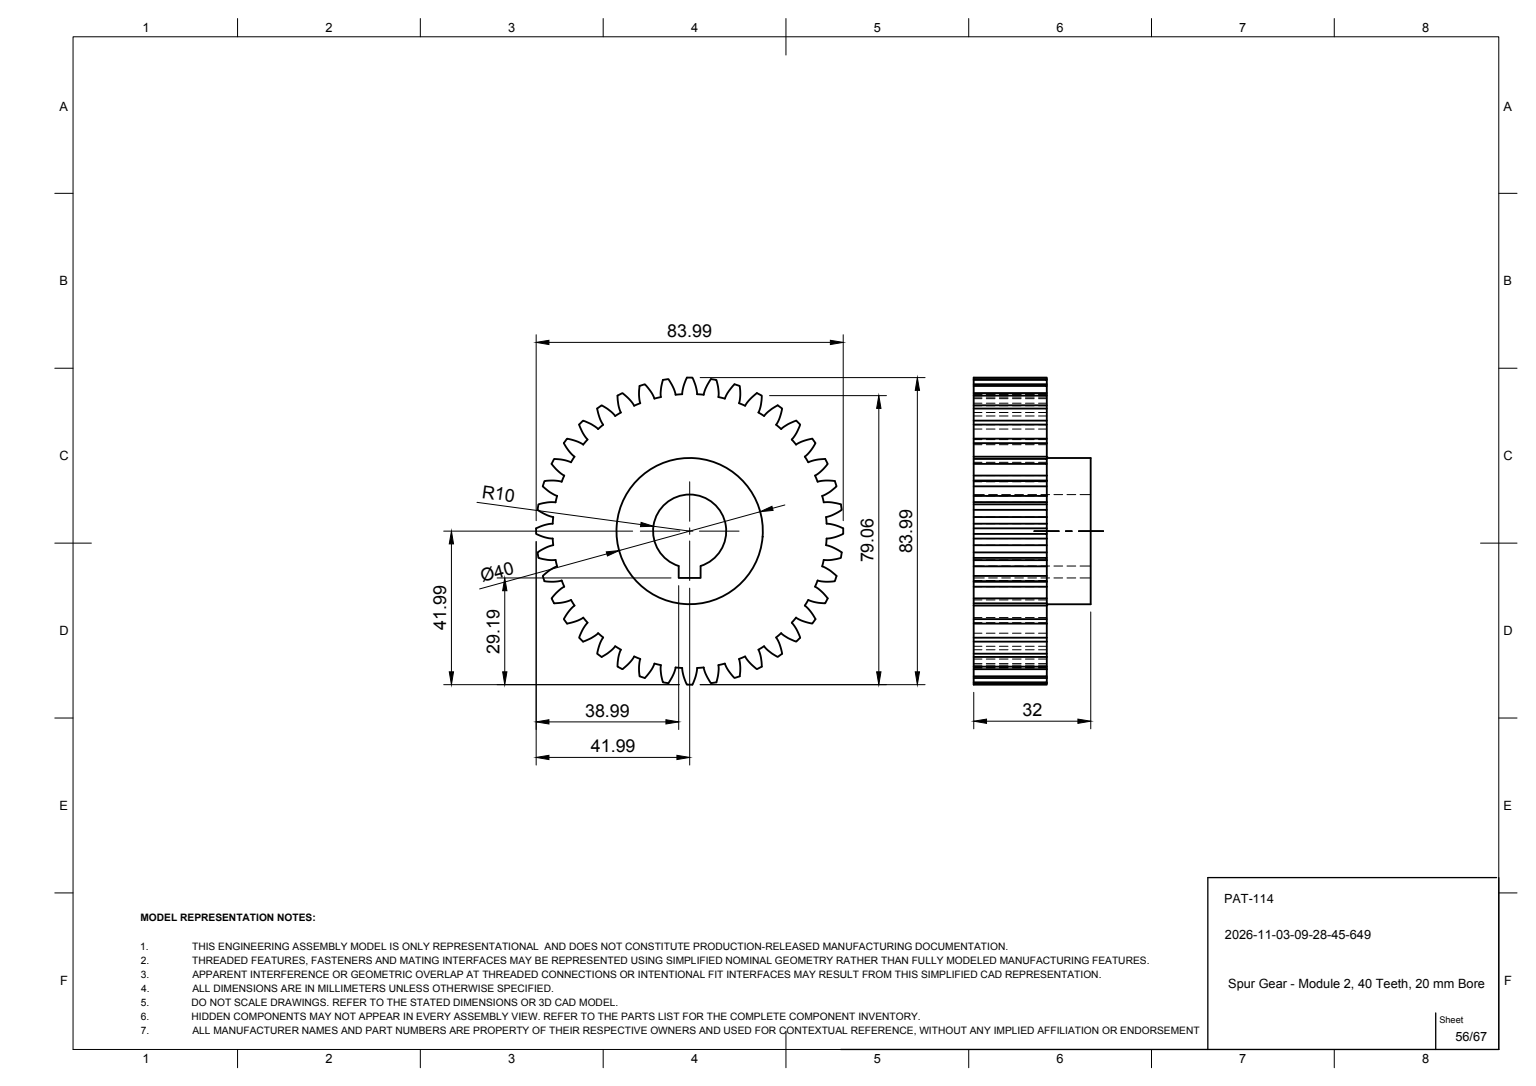
ISO-10303-21;
HEADER;
/* Generated by software containing ST-Developer
 * from STEP Tools, Inc. (www.steptools.com) 
 */

FILE_DESCRIPTION(
/* description */ ('Two-stage gear reducer in split housing'),
/* implementation_level */ '2;1');

FILE_NAME(
/* name */ 'Spur Gear - Module 2, 40 Teeth, 20 mm Bore.step',
/* time_stamp */ '2026-10-28T03:22:31-07:00',
/* author */ (''),
/* organization */ (''),
/* preprocessor_version */ 'ST-DEVELOPER v20.2',
/* originating_system */ 'Autodesk Translation Framework v15.17.0.0',
/* authorisation */ '');

FILE_SCHEMA (('AUTOMOTIVE_DESIGN { 1 0 10303 214 3 1 1 }'));
ENDSEC;

DATA;
#10=MECHANICAL_DESIGN_GEOMETRIC_PRESENTATION_REPRESENTATION('',(#1303),#73366);
#91=(
BOUNDED_SURFACE()
B_SPLINE_SURFACE(5,1,((#55478,#55479),(#55480,#55481),(#55482,#55483),(#55484,
#55485),(#55486,#55487),(#55488,#55489),(#55490,#55491),(#55492,#55493),
(#55494,#55495),(#55496,#55497),(#55498,#55499),(#55500,#55501),(#55502,
#55503),(#55504,#55505),(#55506,#55507),(#55508,#55509),(#55510,#55511),
(#55512,#55513),(#55514,#55515),(#55516,#55517),(#55518,#55519),(#55520,
#55521),(#55522,#55523),(#55524,#55525),(#55526,#55527),(#55528,#55529),
(#55530,#55531),(#55532,#55533),(#55534,#55535),(#55536,#55537),(#55538,
#55539),(#55540,#55541),(#55542,#55543),(#55544,#55545),(#55546,#55547),
(#55548,#55549),(#55550,#55551),(#55552,#55553),(#55554,#55555),(#55556,
#55557),(#55558,#55559),(#55560,#55561),(#55562,#55563),(#55564,#55565),
(#55566,#55567),(#55568,#55569),(#55570,#55571),(#55572,#55573),(#55574,
#55575),(#55576,#55577),(#55578,#55579),(#55580,#55581),(#55582,#55583),
(#55584,#55585),(#55586,#55587),(#55588,#55589),(#55590,#55591),(#55592,
#55593),(#55594,#55595),(#55596,#55597),(#55598,#55599),(#55600,#55601),
(#55602,#55603),(#55604,#55605),(#55606,#55607),(#55608,#55609),(#55610,
#55611),(#55612,#55613),(#55614,#55615),(#55616,#55617)),.UNSPECIFIED.,
 .F.,.F.,.F.)
B_SPLINE_SURFACE_WITH_KNOTS((6,1,1,1,1,1,1,1,1,1,1,1,1,1,1,1,1,1,1,1,1,
1,1,1,1,1,1,1,1,1,1,1,1,1,1,1,1,1,1,1,1,1,1,1,1,1,1,1,1,1,1,1,1,1,1,1,1,
1,1,1,1,1,1,1,1,6),(2,2),(-1.,-0.984615384615383,-0.969230769230768,-0.953846153846152,
-0.938461538461537,-0.923076923076922,-0.907692307692306,-0.892307692307691,
-0.876923076923076,-0.86153846153846,-0.846153846153845,-0.83076923076923,
-0.815384615384614,-0.799999999999999,-0.784615384615384,-0.769230769230768,
-0.753846153846153,-0.738461538461538,-0.723076923076922,-0.707692307692307,
-0.692307692307692,-0.676923076923076,-0.661538461538461,-0.646153846153846,
-0.63076923076923,-0.615384615384615,-0.6,-0.584615384615384,-0.569230769230769,
-0.553846153846154,-0.538461538461538,-0.523076923076923,-0.507692307692308,
-0.492307692307692,-0.476923076923077,-0.461538461538462,-0.446153846153846,
-0.430769230769231,-0.415384615384615,-0.4,-0.384615384615385,-0.369230769230769,
-0.353846153846154,-0.338461538461538,-0.323076923076923,-0.307692307692308,
-0.292307692307692,-0.276923076923077,-0.261538461538462,-0.246153846153846,
-0.230769230769231,-0.215384615384615,-0.2,-0.184615384615385,-0.169230769230769,
-0.153846153846154,-0.138461538461538,-0.123076923076923,-0.107692307692308,
-0.0923076923076923,-0.0769230769230769,-0.0615384615384615,-0.0461538461538462,
-0.0307692307692308,-0.0153846153846154,0.),(-1.,1.),.UNSPECIFIED.)
GEOMETRIC_REPRESENTATION_ITEM()
RATIONAL_B_SPLINE_SURFACE(((1.,1.),(1.,1.),(1.,1.),(1.,1.),(1.,1.),(1.,
1.),(1.,1.),(1.,1.),(1.,1.),(1.,1.),(1.,1.),(1.,1.),(1.,1.),(1.,1.),(1.,
1.),(1.,1.),(1.,1.),(1.,1.),(1.,1.),(1.,1.),(1.,1.),(1.,1.),(1.,1.),(1.,
1.),(1.,1.),(1.,1.),(1.,1.),(1.,1.),(1.,1.),(1.,1.),(1.,1.),(1.,1.),(1.,
1.),(1.,1.),(1.,1.),(1.,1.),(1.,1.),(1.,1.),(1.,1.),(1.,1.),(1.,1.),(1.,
1.),(1.,1.),(1.,1.),(1.,1.),(1.,1.),(1.,1.),(1.,1.),(1.,1.),(1.,1.),(1.,
1.),(1.,1.),(1.,1.),(1.,1.),(1.,1.),(1.,1.),(1.,1.),(1.,1.),(1.,1.),(1.,
1.),(1.,1.),(1.,1.),(1.,1.),(1.,1.),(1.,1.),(1.,1.),(1.,1.),(1.,1.),(1.,
1.),(1.,1.)))
REPRESENTATION_ITEM('')
SURFACE()
);
#92=(
BOUNDED_SURFACE()
B_SPLINE_SURFACE(5,1,((#55697,#55698),(#55699,#55700),(#55701,#55702),(#55703,
#55704),(#55705,#55706),(#55707,#55708),(#55709,#55710),(#55711,#55712),
(#55713,#55714),(#55715,#55716),(#55717,#55718),(#55719,#55720),(#55721,
#55722),(#55723,#55724),(#55725,#55726),(#55727,#55728),(#55729,#55730),
(#55731,#55732),(#55733,#55734),(#55735,#55736),(#55737,#55738),(#55739,
#55740),(#55741,#55742),(#55743,#55744),(#55745,#55746),(#55747,#55748),
(#55749,#55750),(#55751,#55752),(#55753,#55754),(#55755,#55756),(#55757,
#55758),(#55759,#55760),(#55761,#55762),(#55763,#55764),(#55765,#55766),
(#55767,#55768),(#55769,#55770),(#55771,#55772),(#55773,#55774),(#55775,
#55776),(#55777,#55778),(#55779,#55780),(#55781,#55782),(#55783,#55784),
(#55785,#55786),(#55787,#55788),(#55789,#55790),(#55791,#55792),(#55793,
#55794),(#55795,#55796),(#55797,#55798),(#55799,#55800),(#55801,#55802),
(#55803,#55804),(#55805,#55806),(#55807,#55808),(#55809,#55810),(#55811,
#55812),(#55813,#55814),(#55815,#55816),(#55817,#55818),(#55819,#55820),
(#55821,#55822),(#55823,#55824),(#55825,#55826),(#55827,#55828),(#55829,
#55830),(#55831,#55832),(#55833,#55834),(#55835,#55836)),.UNSPECIFIED.,
 .F.,.F.,.F.)
B_SPLINE_SURFACE_WITH_KNOTS((6,1,1,1,1,1,1,1,1,1,1,1,1,1,1,1,1,1,1,1,1,
1,1,1,1,1,1,1,1,1,1,1,1,1,1,1,1,1,1,1,1,1,1,1,1,1,1,1,1,1,1,1,1,1,1,1,1,
1,1,1,1,1,1,1,1,6),(2,2),(-1.,-0.984615384615383,-0.969230769230768,-0.953846153846152,
-0.938461538461537,-0.923076923076922,-0.907692307692306,-0.892307692307691,
-0.876923076923076,-0.86153846153846,-0.846153846153845,-0.83076923076923,
-0.815384615384614,-0.799999999999999,-0.784615384615384,-0.769230769230768,
-0.753846153846153,-0.738461538461538,-0.723076923076922,-0.707692307692307,
-0.692307692307692,-0.676923076923076,-0.661538461538461,-0.646153846153846,
-0.63076923076923,-0.615384615384615,-0.6,-0.584615384615384,-0.569230769230769,
-0.553846153846154,-0.538461538461538,-0.523076923076923,-0.507692307692308,
-0.492307692307692,-0.476923076923077,-0.461538461538462,-0.446153846153846,
-0.430769230769231,-0.415384615384615,-0.4,-0.384615384615385,-0.369230769230769,
-0.353846153846154,-0.338461538461538,-0.323076923076923,-0.307692307692308,
-0.292307692307692,-0.276923076923077,-0.261538461538462,-0.246153846153846,
-0.230769230769231,-0.215384615384615,-0.2,-0.184615384615385,-0.169230769230769,
-0.153846153846154,-0.138461538461538,-0.123076923076923,-0.107692307692308,
-0.0923076923076923,-0.0769230769230769,-0.0615384615384615,-0.0461538461538462,
-0.0307692307692308,-0.0153846153846154,0.),(-1.,1.),.UNSPECIFIED.)
GEOMETRIC_REPRESENTATION_ITEM()
RATIONAL_B_SPLINE_SURFACE(((1.,1.),(1.,1.),(1.,1.),(1.,1.),(1.,1.),(1.,
1.),(1.,1.),(1.,1.),(1.,1.),(1.,1.),(1.,1.),(1.,1.),(1.,1.),(1.,1.),(1.,
1.),(1.,1.),(1.,1.),(1.,1.),(1.,1.),(1.,1.),(1.,1.),(1.,1.),(1.,1.),(1.,
1.),(1.,1.),(1.,1.),(1.,1.),(1.,1.),(1.,1.),(1.,1.),(1.,1.),(1.,1.),(1.,
1.),(1.,1.),(1.,1.),(1.,1.),(1.,1.),(1.,1.),(1.,1.),(1.,1.),(1.,1.),(1.,
1.),(1.,1.),(1.,1.),(1.,1.),(1.,1.),(1.,1.),(1.,1.),(1.,1.),(1.,1.),(1.,
1.),(1.,1.),(1.,1.),(1.,1.),(1.,1.),(1.,1.),(1.,1.),(1.,1.),(1.,1.),(1.,
1.),(1.,1.),(1.,1.),(1.,1.),(1.,1.),(1.,1.),(1.,1.),(1.,1.),(1.,1.),(1.,
1.),(1.,1.)))
REPRESENTATION_ITEM('')
SURFACE()
);
#93=(
BOUNDED_SURFACE()
B_SPLINE_SURFACE(5,1,((#55927,#55928),(#55929,#55930),(#55931,#55932),(#55933,
#55934),(#55935,#55936),(#55937,#55938),(#55939,#55940),(#55941,#55942),
(#55943,#55944),(#55945,#55946),(#55947,#55948),(#55949,#55950),(#55951,
#55952),(#55953,#55954),(#55955,#55956),(#55957,#55958),(#55959,#55960),
(#55961,#55962),(#55963,#55964),(#55965,#55966),(#55967,#55968),(#55969,
#55970),(#55971,#55972),(#55973,#55974),(#55975,#55976),(#55977,#55978),
(#55979,#55980),(#55981,#55982),(#55983,#55984),(#55985,#55986),(#55987,
#55988),(#55989,#55990),(#55991,#55992),(#55993,#55994),(#55995,#55996),
(#55997,#55998),(#55999,#56000),(#56001,#56002),(#56003,#56004),(#56005,
#56006),(#56007,#56008),(#56009,#56010),(#56011,#56012),(#56013,#56014),
(#56015,#56016),(#56017,#56018),(#56019,#56020),(#56021,#56022),(#56023,
#56024),(#56025,#56026),(#56027,#56028),(#56029,#56030),(#56031,#56032),
(#56033,#56034),(#56035,#56036),(#56037,#56038),(#56039,#56040),(#56041,
#56042),(#56043,#56044),(#56045,#56046),(#56047,#56048),(#56049,#56050),
(#56051,#56052),(#56053,#56054),(#56055,#56056),(#56057,#56058),(#56059,
#56060),(#56061,#56062),(#56063,#56064),(#56065,#56066)),.UNSPECIFIED.,
 .F.,.F.,.F.)
B_SPLINE_SURFACE_WITH_KNOTS((6,1,1,1,1,1,1,1,1,1,1,1,1,1,1,1,1,1,1,1,1,
1,1,1,1,1,1,1,1,1,1,1,1,1,1,1,1,1,1,1,1,1,1,1,1,1,1,1,1,1,1,1,1,1,1,1,1,
1,1,1,1,1,1,1,1,6),(2,2),(-1.,-0.984615384615383,-0.969230769230768,-0.953846153846152,
-0.938461538461537,-0.923076923076922,-0.907692307692306,-0.892307692307691,
-0.876923076923076,-0.86153846153846,-0.846153846153845,-0.83076923076923,
-0.815384615384614,-0.799999999999999,-0.784615384615384,-0.769230769230768,
-0.753846153846153,-0.738461538461538,-0.723076923076922,-0.707692307692307,
-0.692307692307692,-0.676923076923076,-0.661538461538461,-0.646153846153846,
-0.63076923076923,-0.615384615384615,-0.6,-0.584615384615384,-0.569230769230769,
-0.553846153846154,-0.538461538461538,-0.523076923076923,-0.507692307692308,
-0.492307692307692,-0.476923076923077,-0.461538461538462,-0.446153846153846,
-0.430769230769231,-0.415384615384615,-0.4,-0.384615384615385,-0.369230769230769,
-0.353846153846154,-0.338461538461538,-0.323076923076923,-0.307692307692308,
-0.292307692307692,-0.276923076923077,-0.261538461538462,-0.246153846153846,
-0.230769230769231,-0.215384615384615,-0.2,-0.184615384615385,-0.169230769230769,
-0.153846153846154,-0.138461538461538,-0.123076923076923,-0.107692307692308,
-0.0923076923076923,-0.0769230769230769,-0.0615384615384615,-0.0461538461538462,
-0.0307692307692308,-0.0153846153846154,0.),(-1.,1.),.UNSPECIFIED.)
GEOMETRIC_REPRESENTATION_ITEM()
RATIONAL_B_SPLINE_SURFACE(((1.,1.),(1.,1.),(1.,1.),(1.,1.),(1.,1.),(1.,
1.),(1.,1.),(1.,1.),(1.,1.),(1.,1.),(1.,1.),(1.,1.),(1.,1.),(1.,1.),(1.,
1.),(1.,1.),(1.,1.),(1.,1.),(1.,1.),(1.,1.),(1.,1.),(1.,1.),(1.,1.),(1.,
1.),(1.,1.),(1.,1.),(1.,1.),(1.,1.),(1.,1.),(1.,1.),(1.,1.),(1.,1.),(1.,
1.),(1.,1.),(1.,1.),(1.,1.),(1.,1.),(1.,1.),(1.,1.),(1.,1.),(1.,1.),(1.,
1.),(1.,1.),(1.,1.),(1.,1.),(1.,1.),(1.,1.),(1.,1.),(1.,1.),(1.,1.),(1.,
1.),(1.,1.),(1.,1.),(1.,1.),(1.,1.),(1.,1.),(1.,1.),(1.,1.),(1.,1.),(1.,
1.),(1.,1.),(1.,1.),(1.,1.),(1.,1.),(1.,1.),(1.,1.),(1.,1.),(1.,1.),(1.,
1.),(1.,1.)))
REPRESENTATION_ITEM('')
SURFACE()
);
#94=(
BOUNDED_SURFACE()
B_SPLINE_SURFACE(5,1,((#56139,#56140),(#56141,#56142),(#56143,#56144),(#56145,
#56146),(#56147,#56148),(#56149,#56150),(#56151,#56152),(#56153,#56154),
(#56155,#56156),(#56157,#56158),(#56159,#56160),(#56161,#56162),(#56163,
#56164),(#56165,#56166),(#56167,#56168),(#56169,#56170),(#56171,#56172),
(#56173,#56174),(#56175,#56176),(#56177,#56178),(#56179,#56180),(#56181,
#56182),(#56183,#56184),(#56185,#56186),(#56187,#56188),(#56189,#56190),
(#56191,#56192),(#56193,#56194),(#56195,#56196),(#56197,#56198),(#56199,
#56200),(#56201,#56202),(#56203,#56204),(#56205,#56206),(#56207,#56208),
(#56209,#56210),(#56211,#56212),(#56213,#56214),(#56215,#56216),(#56217,
#56218),(#56219,#56220),(#56221,#56222),(#56223,#56224),(#56225,#56226),
(#56227,#56228),(#56229,#56230),(#56231,#56232),(#56233,#56234),(#56235,
#56236),(#56237,#56238),(#56239,#56240),(#56241,#56242),(#56243,#56244),
(#56245,#56246),(#56247,#56248),(#56249,#56250),(#56251,#56252),(#56253,
#56254),(#56255,#56256),(#56257,#56258),(#56259,#56260),(#56261,#56262),
(#56263,#56264),(#56265,#56266),(#56267,#56268),(#56269,#56270),(#56271,
#56272),(#56273,#56274),(#56275,#56276),(#56277,#56278)),.UNSPECIFIED.,
 .F.,.F.,.F.)
B_SPLINE_SURFACE_WITH_KNOTS((6,1,1,1,1,1,1,1,1,1,1,1,1,1,1,1,1,1,1,1,1,
1,1,1,1,1,1,1,1,1,1,1,1,1,1,1,1,1,1,1,1,1,1,1,1,1,1,1,1,1,1,1,1,1,1,1,1,
1,1,1,1,1,1,1,1,6),(2,2),(-1.,-0.984615384615383,-0.969230769230768,-0.953846153846152,
-0.938461538461537,-0.923076923076922,-0.907692307692306,-0.892307692307691,
-0.876923076923076,-0.86153846153846,-0.846153846153845,-0.83076923076923,
-0.815384615384614,-0.799999999999999,-0.784615384615384,-0.769230769230768,
-0.753846153846153,-0.738461538461538,-0.723076923076922,-0.707692307692307,
-0.692307692307692,-0.676923076923076,-0.661538461538461,-0.646153846153846,
-0.63076923076923,-0.615384615384615,-0.6,-0.584615384615384,-0.569230769230769,
-0.553846153846154,-0.538461538461538,-0.523076923076923,-0.507692307692308,
-0.492307692307692,-0.476923076923077,-0.461538461538462,-0.446153846153846,
-0.430769230769231,-0.415384615384615,-0.4,-0.384615384615385,-0.369230769230769,
-0.353846153846154,-0.338461538461538,-0.323076923076923,-0.307692307692308,
-0.292307692307692,-0.276923076923077,-0.261538461538462,-0.246153846153846,
-0.230769230769231,-0.215384615384615,-0.2,-0.184615384615385,-0.169230769230769,
-0.153846153846154,-0.138461538461538,-0.123076923076923,-0.107692307692308,
-0.0923076923076923,-0.0769230769230769,-0.0615384615384615,-0.0461538461538462,
-0.0307692307692308,-0.0153846153846154,0.),(-1.,1.),.UNSPECIFIED.)
GEOMETRIC_REPRESENTATION_ITEM()
RATIONAL_B_SPLINE_SURFACE(((1.,1.),(1.,1.),(1.,1.),(1.,1.),(1.,1.),(1.,
1.),(1.,1.),(1.,1.),(1.,1.),(1.,1.),(1.,1.),(1.,1.),(1.,1.),(1.,1.),(1.,
1.),(1.,1.),(1.,1.),(1.,1.),(1.,1.),(1.,1.),(1.,1.),(1.,1.),(1.,1.),(1.,
1.),(1.,1.),(1.,1.),(1.,1.),(1.,1.),(1.,1.),(1.,1.),(1.,1.),(1.,1.),(1.,
1.),(1.,1.),(1.,1.),(1.,1.),(1.,1.),(1.,1.),(1.,1.),(1.,1.),(1.,1.),(1.,
1.),(1.,1.),(1.,1.),(1.,1.),(1.,1.),(1.,1.),(1.,1.),(1.,1.),(1.,1.),(1.,
1.),(1.,1.),(1.,1.),(1.,1.),(1.,1.),(1.,1.),(1.,1.),(1.,1.),(1.,1.),(1.,
1.),(1.,1.),(1.,1.),(1.,1.),(1.,1.),(1.,1.),(1.,1.),(1.,1.),(1.,1.),(1.,
1.),(1.,1.)))
REPRESENTATION_ITEM('')
SURFACE()
);
#95=(
BOUNDED_SURFACE()
B_SPLINE_SURFACE(5,1,((#56369,#56370),(#56371,#56372),(#56373,#56374),(#56375,
#56376),(#56377,#56378),(#56379,#56380),(#56381,#56382),(#56383,#56384),
(#56385,#56386),(#56387,#56388),(#56389,#56390),(#56391,#56392),(#56393,
#56394),(#56395,#56396),(#56397,#56398),(#56399,#56400),(#56401,#56402),
(#56403,#56404),(#56405,#56406),(#56407,#56408),(#56409,#56410),(#56411,
#56412),(#56413,#56414),(#56415,#56416),(#56417,#56418),(#56419,#56420),
(#56421,#56422),(#56423,#56424),(#56425,#56426),(#56427,#56428),(#56429,
#56430),(#56431,#56432),(#56433,#56434),(#56435,#56436),(#56437,#56438),
(#56439,#56440),(#56441,#56442),(#56443,#56444),(#56445,#56446),(#56447,
#56448),(#56449,#56450),(#56451,#56452),(#56453,#56454),(#56455,#56456),
(#56457,#56458),(#56459,#56460),(#56461,#56462),(#56463,#56464),(#56465,
#56466),(#56467,#56468),(#56469,#56470),(#56471,#56472),(#56473,#56474),
(#56475,#56476),(#56477,#56478),(#56479,#56480),(#56481,#56482),(#56483,
#56484),(#56485,#56486),(#56487,#56488),(#56489,#56490),(#56491,#56492),
(#56493,#56494),(#56495,#56496),(#56497,#56498),(#56499,#56500),(#56501,
#56502),(#56503,#56504),(#56505,#56506),(#56507,#56508)),.UNSPECIFIED.,
 .F.,.F.,.F.)
B_SPLINE_SURFACE_WITH_KNOTS((6,1,1,1,1,1,1,1,1,1,1,1,1,1,1,1,1,1,1,1,1,
1,1,1,1,1,1,1,1,1,1,1,1,1,1,1,1,1,1,1,1,1,1,1,1,1,1,1,1,1,1,1,1,1,1,1,1,
1,1,1,1,1,1,1,1,6),(2,2),(-1.,-0.984615384615383,-0.969230769230768,-0.953846153846152,
-0.938461538461537,-0.923076923076922,-0.907692307692306,-0.892307692307691,
-0.876923076923076,-0.86153846153846,-0.846153846153845,-0.83076923076923,
-0.815384615384614,-0.799999999999999,-0.784615384615384,-0.769230769230768,
-0.753846153846153,-0.738461538461538,-0.723076923076922,-0.707692307692307,
-0.692307692307692,-0.676923076923076,-0.661538461538461,-0.646153846153846,
-0.63076923076923,-0.615384615384615,-0.6,-0.584615384615384,-0.569230769230769,
-0.553846153846154,-0.538461538461538,-0.523076923076923,-0.507692307692308,
-0.492307692307692,-0.476923076923077,-0.461538461538462,-0.446153846153846,
-0.430769230769231,-0.415384615384615,-0.4,-0.384615384615385,-0.369230769230769,
-0.353846153846154,-0.338461538461538,-0.323076923076923,-0.307692307692308,
-0.292307692307692,-0.276923076923077,-0.261538461538462,-0.246153846153846,
-0.230769230769231,-0.215384615384615,-0.2,-0.184615384615385,-0.169230769230769,
-0.153846153846154,-0.138461538461538,-0.123076923076923,-0.107692307692308,
-0.0923076923076923,-0.0769230769230769,-0.0615384615384615,-0.0461538461538462,
-0.0307692307692308,-0.0153846153846154,0.),(-1.,1.),.UNSPECIFIED.)
GEOMETRIC_REPRESENTATION_ITEM()
RATIONAL_B_SPLINE_SURFACE(((1.,1.),(1.,1.),(1.,1.),(1.,1.),(1.,1.),(1.,
1.),(1.,1.),(1.,1.),(1.,1.),(1.,1.),(1.,1.),(1.,1.),(1.,1.),(1.,1.),(1.,
1.),(1.,1.),(1.,1.),(1.,1.),(1.,1.),(1.,1.),(1.,1.),(1.,1.),(1.,1.),(1.,
1.),(1.,1.),(1.,1.),(1.,1.),(1.,1.),(1.,1.),(1.,1.),(1.,1.),(1.,1.),(1.,
1.),(1.,1.),(1.,1.),(1.,1.),(1.,1.),(1.,1.),(1.,1.),(1.,1.),(1.,1.),(1.,
1.),(1.,1.),(1.,1.),(1.,1.),(1.,1.),(1.,1.),(1.,1.),(1.,1.),(1.,1.),(1.,
1.),(1.,1.),(1.,1.),(1.,1.),(1.,1.),(1.,1.),(1.,1.),(1.,1.),(1.,1.),(1.,
1.),(1.,1.),(1.,1.),(1.,1.),(1.,1.),(1.,1.),(1.,1.),(1.,1.),(1.,1.),(1.,
1.),(1.,1.)))
REPRESENTATION_ITEM('')
SURFACE()
);
#96=(
BOUNDED_SURFACE()
B_SPLINE_SURFACE(5,1,((#56581,#56582),(#56583,#56584),(#56585,#56586),(#56587,
#56588),(#56589,#56590),(#56591,#56592),(#56593,#56594),(#56595,#56596),
(#56597,#56598),(#56599,#56600),(#56601,#56602),(#56603,#56604),(#56605,
#56606),(#56607,#56608),(#56609,#56610),(#56611,#56612),(#56613,#56614),
(#56615,#56616),(#56617,#56618),(#56619,#56620),(#56621,#56622),(#56623,
#56624),(#56625,#56626),(#56627,#56628),(#56629,#56630),(#56631,#56632),
(#56633,#56634),(#56635,#56636),(#56637,#56638),(#56639,#56640),(#56641,
#56642),(#56643,#56644),(#56645,#56646),(#56647,#56648),(#56649,#56650),
(#56651,#56652),(#56653,#56654),(#56655,#56656),(#56657,#56658),(#56659,
#56660),(#56661,#56662),(#56663,#56664),(#56665,#56666),(#56667,#56668),
(#56669,#56670),(#56671,#56672),(#56673,#56674),(#56675,#56676),(#56677,
#56678),(#56679,#56680),(#56681,#56682),(#56683,#56684),(#56685,#56686),
(#56687,#56688),(#56689,#56690),(#56691,#56692),(#56693,#56694),(#56695,
#56696),(#56697,#56698),(#56699,#56700),(#56701,#56702),(#56703,#56704),
(#56705,#56706),(#56707,#56708),(#56709,#56710),(#56711,#56712),(#56713,
#56714),(#56715,#56716),(#56717,#56718),(#56719,#56720)),.UNSPECIFIED.,
 .F.,.F.,.F.)
B_SPLINE_SURFACE_WITH_KNOTS((6,1,1,1,1,1,1,1,1,1,1,1,1,1,1,1,1,1,1,1,1,
1,1,1,1,1,1,1,1,1,1,1,1,1,1,1,1,1,1,1,1,1,1,1,1,1,1,1,1,1,1,1,1,1,1,1,1,
1,1,1,1,1,1,1,1,6),(2,2),(-1.,-0.984615384615383,-0.969230769230768,-0.953846153846152,
-0.938461538461537,-0.923076923076922,-0.907692307692306,-0.892307692307691,
-0.876923076923076,-0.86153846153846,-0.846153846153845,-0.83076923076923,
-0.815384615384614,-0.799999999999999,-0.784615384615384,-0.769230769230768,
-0.753846153846153,-0.738461538461538,-0.723076923076922,-0.707692307692307,
-0.692307692307692,-0.676923076923076,-0.661538461538461,-0.646153846153846,
-0.63076923076923,-0.615384615384615,-0.6,-0.584615384615384,-0.569230769230769,
-0.553846153846154,-0.538461538461538,-0.523076923076923,-0.507692307692308,
-0.492307692307692,-0.476923076923077,-0.461538461538462,-0.446153846153846,
-0.430769230769231,-0.415384615384615,-0.4,-0.384615384615385,-0.369230769230769,
-0.353846153846154,-0.338461538461538,-0.323076923076923,-0.307692307692308,
-0.292307692307692,-0.276923076923077,-0.261538461538462,-0.246153846153846,
-0.230769230769231,-0.215384615384615,-0.2,-0.184615384615385,-0.169230769230769,
-0.153846153846154,-0.138461538461538,-0.123076923076923,-0.107692307692308,
-0.0923076923076923,-0.0769230769230769,-0.0615384615384615,-0.0461538461538462,
-0.0307692307692308,-0.0153846153846154,0.),(-1.,1.),.UNSPECIFIED.)
GEOMETRIC_REPRESENTATION_ITEM()
RATIONAL_B_SPLINE_SURFACE(((1.,1.),(1.,1.),(1.,1.),(1.,1.),(1.,1.),(1.,
1.),(1.,1.),(1.,1.),(1.,1.),(1.,1.),(1.,1.),(1.,1.),(1.,1.),(1.,1.),(1.,
1.),(1.,1.),(1.,1.),(1.,1.),(1.,1.),(1.,1.),(1.,1.),(1.,1.),(1.,1.),(1.,
1.),(1.,1.),(1.,1.),(1.,1.),(1.,1.),(1.,1.),(1.,1.),(1.,1.),(1.,1.),(1.,
1.),(1.,1.),(1.,1.),(1.,1.),(1.,1.),(1.,1.),(1.,1.),(1.,1.),(1.,1.),(1.,
1.),(1.,1.),(1.,1.),(1.,1.),(1.,1.),(1.,1.),(1.,1.),(1.,1.),(1.,1.),(1.,
1.),(1.,1.),(1.,1.),(1.,1.),(1.,1.),(1.,1.),(1.,1.),(1.,1.),(1.,1.),(1.,
1.),(1.,1.),(1.,1.),(1.,1.),(1.,1.),(1.,1.),(1.,1.),(1.,1.),(1.,1.),(1.,
1.),(1.,1.)))
REPRESENTATION_ITEM('')
SURFACE()
);
#97=(
BOUNDED_SURFACE()
B_SPLINE_SURFACE(5,1,((#56811,#56812),(#56813,#56814),(#56815,#56816),(#56817,
#56818),(#56819,#56820),(#56821,#56822),(#56823,#56824),(#56825,#56826),
(#56827,#56828),(#56829,#56830),(#56831,#56832),(#56833,#56834),(#56835,
#56836),(#56837,#56838),(#56839,#56840),(#56841,#56842),(#56843,#56844),
(#56845,#56846),(#56847,#56848),(#56849,#56850),(#56851,#56852),(#56853,
#56854),(#56855,#56856),(#56857,#56858),(#56859,#56860),(#56861,#56862),
(#56863,#56864),(#56865,#56866),(#56867,#56868),(#56869,#56870),(#56871,
#56872),(#56873,#56874),(#56875,#56876),(#56877,#56878),(#56879,#56880),
(#56881,#56882),(#56883,#56884),(#56885,#56886),(#56887,#56888),(#56889,
#56890),(#56891,#56892),(#56893,#56894),(#56895,#56896),(#56897,#56898),
(#56899,#56900),(#56901,#56902),(#56903,#56904),(#56905,#56906),(#56907,
#56908),(#56909,#56910),(#56911,#56912),(#56913,#56914),(#56915,#56916),
(#56917,#56918),(#56919,#56920),(#56921,#56922),(#56923,#56924),(#56925,
#56926),(#56927,#56928),(#56929,#56930),(#56931,#56932),(#56933,#56934),
(#56935,#56936),(#56937,#56938),(#56939,#56940),(#56941,#56942),(#56943,
#56944),(#56945,#56946),(#56947,#56948),(#56949,#56950)),.UNSPECIFIED.,
 .F.,.F.,.F.)
B_SPLINE_SURFACE_WITH_KNOTS((6,1,1,1,1,1,1,1,1,1,1,1,1,1,1,1,1,1,1,1,1,
1,1,1,1,1,1,1,1,1,1,1,1,1,1,1,1,1,1,1,1,1,1,1,1,1,1,1,1,1,1,1,1,1,1,1,1,
1,1,1,1,1,1,1,1,6),(2,2),(-1.,-0.984615384615383,-0.969230769230768,-0.953846153846152,
-0.938461538461537,-0.923076923076922,-0.907692307692306,-0.892307692307691,
-0.876923076923076,-0.86153846153846,-0.846153846153845,-0.83076923076923,
-0.815384615384614,-0.799999999999999,-0.784615384615384,-0.769230769230768,
-0.753846153846153,-0.738461538461538,-0.723076923076922,-0.707692307692307,
-0.692307692307692,-0.676923076923076,-0.661538461538461,-0.646153846153846,
-0.63076923076923,-0.615384615384615,-0.6,-0.584615384615384,-0.569230769230769,
-0.553846153846154,-0.538461538461538,-0.523076923076923,-0.507692307692308,
-0.492307692307692,-0.476923076923077,-0.461538461538462,-0.446153846153846,
-0.430769230769231,-0.415384615384615,-0.4,-0.384615384615385,-0.369230769230769,
-0.353846153846154,-0.338461538461538,-0.323076923076923,-0.307692307692308,
-0.292307692307692,-0.276923076923077,-0.261538461538462,-0.246153846153846,
-0.230769230769231,-0.215384615384615,-0.2,-0.184615384615385,-0.169230769230769,
-0.153846153846154,-0.138461538461538,-0.123076923076923,-0.107692307692308,
-0.0923076923076923,-0.0769230769230769,-0.0615384615384615,-0.0461538461538462,
-0.0307692307692308,-0.0153846153846154,0.),(-1.,1.),.UNSPECIFIED.)
GEOMETRIC_REPRESENTATION_ITEM()
RATIONAL_B_SPLINE_SURFACE(((1.,1.),(1.,1.),(1.,1.),(1.,1.),(1.,1.),(1.,
1.),(1.,1.),(1.,1.),(1.,1.),(1.,1.),(1.,1.),(1.,1.),(1.,1.),(1.,1.),(1.,
1.),(1.,1.),(1.,1.),(1.,1.),(1.,1.),(1.,1.),(1.,1.),(1.,1.),(1.,1.),(1.,
1.),(1.,1.),(1.,1.),(1.,1.),(1.,1.),(1.,1.),(1.,1.),(1.,1.),(1.,1.),(1.,
1.),(1.,1.),(1.,1.),(1.,1.),(1.,1.),(1.,1.),(1.,1.),(1.,1.),(1.,1.),(1.,
1.),(1.,1.),(1.,1.),(1.,1.),(1.,1.),(1.,1.),(1.,1.),(1.,1.),(1.,1.),(1.,
1.),(1.,1.),(1.,1.),(1.,1.),(1.,1.),(1.,1.),(1.,1.),(1.,1.),(1.,1.),(1.,
1.),(1.,1.),(1.,1.),(1.,1.),(1.,1.),(1.,1.),(1.,1.),(1.,1.),(1.,1.),(1.,
1.),(1.,1.)))
REPRESENTATION_ITEM('')
SURFACE()
);
#98=(
BOUNDED_SURFACE()
B_SPLINE_SURFACE(5,1,((#57023,#57024),(#57025,#57026),(#57027,#57028),(#57029,
#57030),(#57031,#57032),(#57033,#57034),(#57035,#57036),(#57037,#57038),
(#57039,#57040),(#57041,#57042),(#57043,#57044),(#57045,#57046),(#57047,
#57048),(#57049,#57050),(#57051,#57052),(#57053,#57054),(#57055,#57056),
(#57057,#57058),(#57059,#57060),(#57061,#57062),(#57063,#57064),(#57065,
#57066),(#57067,#57068),(#57069,#57070),(#57071,#57072),(#57073,#57074),
(#57075,#57076),(#57077,#57078),(#57079,#57080),(#57081,#57082),(#57083,
#57084),(#57085,#57086),(#57087,#57088),(#57089,#57090),(#57091,#57092),
(#57093,#57094),(#57095,#57096),(#57097,#57098),(#57099,#57100),(#57101,
#57102),(#57103,#57104),(#57105,#57106),(#57107,#57108),(#57109,#57110),
(#57111,#57112),(#57113,#57114),(#57115,#57116),(#57117,#57118),(#57119,
#57120),(#57121,#57122),(#57123,#57124),(#57125,#57126),(#57127,#57128),
(#57129,#57130),(#57131,#57132),(#57133,#57134),(#57135,#57136),(#57137,
#57138),(#57139,#57140),(#57141,#57142),(#57143,#57144),(#57145,#57146),
(#57147,#57148),(#57149,#57150),(#57151,#57152),(#57153,#57154),(#57155,
#57156),(#57157,#57158),(#57159,#57160),(#57161,#57162)),.UNSPECIFIED.,
 .F.,.F.,.F.)
B_SPLINE_SURFACE_WITH_KNOTS((6,1,1,1,1,1,1,1,1,1,1,1,1,1,1,1,1,1,1,1,1,
1,1,1,1,1,1,1,1,1,1,1,1,1,1,1,1,1,1,1,1,1,1,1,1,1,1,1,1,1,1,1,1,1,1,1,1,
1,1,1,1,1,1,1,1,6),(2,2),(-1.,-0.984615384615383,-0.969230769230768,-0.953846153846152,
-0.938461538461537,-0.923076923076922,-0.907692307692306,-0.892307692307691,
-0.876923076923076,-0.86153846153846,-0.846153846153845,-0.83076923076923,
-0.815384615384614,-0.799999999999999,-0.784615384615384,-0.769230769230768,
-0.753846153846153,-0.738461538461538,-0.723076923076922,-0.707692307692307,
-0.692307692307692,-0.676923076923076,-0.661538461538461,-0.646153846153846,
-0.63076923076923,-0.615384615384615,-0.6,-0.584615384615384,-0.569230769230769,
-0.553846153846154,-0.538461538461538,-0.523076923076923,-0.507692307692308,
-0.492307692307692,-0.476923076923077,-0.461538461538462,-0.446153846153846,
-0.430769230769231,-0.415384615384615,-0.4,-0.384615384615385,-0.369230769230769,
-0.353846153846154,-0.338461538461538,-0.323076923076923,-0.307692307692308,
-0.292307692307692,-0.276923076923077,-0.261538461538462,-0.246153846153846,
-0.230769230769231,-0.215384615384615,-0.2,-0.184615384615385,-0.169230769230769,
-0.153846153846154,-0.138461538461538,-0.123076923076923,-0.107692307692308,
-0.0923076923076923,-0.0769230769230769,-0.0615384615384615,-0.0461538461538462,
-0.0307692307692308,-0.0153846153846154,0.),(-1.,1.),.UNSPECIFIED.)
GEOMETRIC_REPRESENTATION_ITEM()
RATIONAL_B_SPLINE_SURFACE(((1.,1.),(1.,1.),(1.,1.),(1.,1.),(1.,1.),(1.,
1.),(1.,1.),(1.,1.),(1.,1.),(1.,1.),(1.,1.),(1.,1.),(1.,1.),(1.,1.),(1.,
1.),(1.,1.),(1.,1.),(1.,1.),(1.,1.),(1.,1.),(1.,1.),(1.,1.),(1.,1.),(1.,
1.),(1.,1.),(1.,1.),(1.,1.),(1.,1.),(1.,1.),(1.,1.),(1.,1.),(1.,1.),(1.,
1.),(1.,1.),(1.,1.),(1.,1.),(1.,1.),(1.,1.),(1.,1.),(1.,1.),(1.,1.),(1.,
1.),(1.,1.),(1.,1.),(1.,1.),(1.,1.),(1.,1.),(1.,1.),(1.,1.),(1.,1.),(1.,
1.),(1.,1.),(1.,1.),(1.,1.),(1.,1.),(1.,1.),(1.,1.),(1.,1.),(1.,1.),(1.,
1.),(1.,1.),(1.,1.),(1.,1.),(1.,1.),(1.,1.),(1.,1.),(1.,1.),(1.,1.),(1.,
1.),(1.,1.)))
REPRESENTATION_ITEM('')
SURFACE()
);
#99=(
BOUNDED_SURFACE()
B_SPLINE_SURFACE(5,1,((#57253,#57254),(#57255,#57256),(#57257,#57258),(#57259,
#57260),(#57261,#57262),(#57263,#57264),(#57265,#57266),(#57267,#57268),
(#57269,#57270),(#57271,#57272),(#57273,#57274),(#57275,#57276),(#57277,
#57278),(#57279,#57280),(#57281,#57282),(#57283,#57284),(#57285,#57286),
(#57287,#57288),(#57289,#57290),(#57291,#57292),(#57293,#57294),(#57295,
#57296),(#57297,#57298),(#57299,#57300),(#57301,#57302),(#57303,#57304),
(#57305,#57306),(#57307,#57308),(#57309,#57310),(#57311,#57312),(#57313,
#57314),(#57315,#57316),(#57317,#57318),(#57319,#57320),(#57321,#57322),
(#57323,#57324),(#57325,#57326),(#57327,#57328),(#57329,#57330),(#57331,
#57332),(#57333,#57334),(#57335,#57336),(#57337,#57338),(#57339,#57340),
(#57341,#57342),(#57343,#57344),(#57345,#57346),(#57347,#57348),(#57349,
#57350),(#57351,#57352),(#57353,#57354),(#57355,#57356),(#57357,#57358),
(#57359,#57360),(#57361,#57362),(#57363,#57364),(#57365,#57366),(#57367,
#57368),(#57369,#57370),(#57371,#57372),(#57373,#57374),(#57375,#57376),
(#57377,#57378),(#57379,#57380),(#57381,#57382),(#57383,#57384),(#57385,
#57386),(#57387,#57388),(#57389,#57390),(#57391,#57392)),.UNSPECIFIED.,
 .F.,.F.,.F.)
B_SPLINE_SURFACE_WITH_KNOTS((6,1,1,1,1,1,1,1,1,1,1,1,1,1,1,1,1,1,1,1,1,
1,1,1,1,1,1,1,1,1,1,1,1,1,1,1,1,1,1,1,1,1,1,1,1,1,1,1,1,1,1,1,1,1,1,1,1,
1,1,1,1,1,1,1,1,6),(2,2),(-1.,-0.984615384615383,-0.969230769230768,-0.953846153846152,
-0.938461538461537,-0.923076923076922,-0.907692307692306,-0.892307692307691,
-0.876923076923076,-0.86153846153846,-0.846153846153845,-0.83076923076923,
-0.815384615384614,-0.799999999999999,-0.784615384615384,-0.769230769230768,
-0.753846153846153,-0.738461538461538,-0.723076923076922,-0.707692307692307,
-0.692307692307692,-0.676923076923076,-0.661538461538461,-0.646153846153846,
-0.63076923076923,-0.615384615384615,-0.6,-0.584615384615384,-0.569230769230769,
-0.553846153846154,-0.538461538461538,-0.523076923076923,-0.507692307692308,
-0.492307692307692,-0.476923076923077,-0.461538461538462,-0.446153846153846,
-0.430769230769231,-0.415384615384615,-0.4,-0.384615384615385,-0.369230769230769,
-0.353846153846154,-0.338461538461538,-0.323076923076923,-0.307692307692308,
-0.292307692307692,-0.276923076923077,-0.261538461538462,-0.246153846153846,
-0.230769230769231,-0.215384615384615,-0.2,-0.184615384615385,-0.169230769230769,
-0.153846153846154,-0.138461538461538,-0.123076923076923,-0.107692307692308,
-0.0923076923076923,-0.0769230769230769,-0.0615384615384615,-0.0461538461538462,
-0.0307692307692308,-0.0153846153846154,0.),(-1.,1.),.UNSPECIFIED.)
GEOMETRIC_REPRESENTATION_ITEM()
RATIONAL_B_SPLINE_SURFACE(((1.,1.),(1.,1.),(1.,1.),(1.,1.),(1.,1.),(1.,
1.),(1.,1.),(1.,1.),(1.,1.),(1.,1.),(1.,1.),(1.,1.),(1.,1.),(1.,1.),(1.,
1.),(1.,1.),(1.,1.),(1.,1.),(1.,1.),(1.,1.),(1.,1.),(1.,1.),(1.,1.),(1.,
1.),(1.,1.),(1.,1.),(1.,1.),(1.,1.),(1.,1.),(1.,1.),(1.,1.),(1.,1.),(1.,
1.),(1.,1.),(1.,1.),(1.,1.),(1.,1.),(1.,1.),(1.,1.),(1.,1.),(1.,1.),(1.,
1.),(1.,1.),(1.,1.),(1.,1.),(1.,1.),(1.,1.),(1.,1.),(1.,1.),(1.,1.),(1.,
1.),(1.,1.),(1.,1.),(1.,1.),(1.,1.),(1.,1.),(1.,1.),(1.,1.),(1.,1.),(1.,
1.),(1.,1.),(1.,1.),(1.,1.),(1.,1.),(1.,1.),(1.,1.),(1.,1.),(1.,1.),(1.,
1.),(1.,1.)))
REPRESENTATION_ITEM('')
SURFACE()
);
#100=(
BOUNDED_SURFACE()
B_SPLINE_SURFACE(5,1,((#57465,#57466),(#57467,#57468),(#57469,#57470),(#57471,
#57472),(#57473,#57474),(#57475,#57476),(#57477,#57478),(#57479,#57480),
(#57481,#57482),(#57483,#57484),(#57485,#57486),(#57487,#57488),(#57489,
#57490),(#57491,#57492),(#57493,#57494),(#57495,#57496),(#57497,#57498),
(#57499,#57500),(#57501,#57502),(#57503,#57504),(#57505,#57506),(#57507,
#57508),(#57509,#57510),(#57511,#57512),(#57513,#57514),(#57515,#57516),
(#57517,#57518),(#57519,#57520),(#57521,#57522),(#57523,#57524),(#57525,
#57526),(#57527,#57528),(#57529,#57530),(#57531,#57532),(#57533,#57534),
(#57535,#57536),(#57537,#57538),(#57539,#57540),(#57541,#57542),(#57543,
#57544),(#57545,#57546),(#57547,#57548),(#57549,#57550),(#57551,#57552),
(#57553,#57554),(#57555,#57556),(#57557,#57558),(#57559,#57560),(#57561,
#57562),(#57563,#57564),(#57565,#57566),(#57567,#57568),(#57569,#57570),
(#57571,#57572),(#57573,#57574),(#57575,#57576),(#57577,#57578),(#57579,
#57580),(#57581,#57582),(#57583,#57584),(#57585,#57586),(#57587,#57588),
(#57589,#57590),(#57591,#57592),(#57593,#57594),(#57595,#57596),(#57597,
#57598),(#57599,#57600),(#57601,#57602),(#57603,#57604)),.UNSPECIFIED.,
 .F.,.F.,.F.)
B_SPLINE_SURFACE_WITH_KNOTS((6,1,1,1,1,1,1,1,1,1,1,1,1,1,1,1,1,1,1,1,1,
1,1,1,1,1,1,1,1,1,1,1,1,1,1,1,1,1,1,1,1,1,1,1,1,1,1,1,1,1,1,1,1,1,1,1,1,
1,1,1,1,1,1,1,1,6),(2,2),(-1.,-0.984615384615383,-0.969230769230768,-0.953846153846152,
-0.938461538461537,-0.923076923076922,-0.907692307692306,-0.892307692307691,
-0.876923076923076,-0.86153846153846,-0.846153846153845,-0.83076923076923,
-0.815384615384614,-0.799999999999999,-0.784615384615384,-0.769230769230768,
-0.753846153846153,-0.738461538461538,-0.723076923076922,-0.707692307692307,
-0.692307692307692,-0.676923076923076,-0.661538461538461,-0.646153846153846,
-0.63076923076923,-0.615384615384615,-0.6,-0.584615384615384,-0.569230769230769,
-0.553846153846154,-0.538461538461538,-0.523076923076923,-0.507692307692308,
-0.492307692307692,-0.476923076923077,-0.461538461538462,-0.446153846153846,
-0.430769230769231,-0.415384615384615,-0.4,-0.384615384615385,-0.369230769230769,
-0.353846153846154,-0.338461538461538,-0.323076923076923,-0.307692307692308,
-0.292307692307692,-0.276923076923077,-0.261538461538462,-0.246153846153846,
-0.230769230769231,-0.215384615384615,-0.2,-0.184615384615385,-0.169230769230769,
-0.153846153846154,-0.138461538461538,-0.123076923076923,-0.107692307692308,
-0.0923076923076923,-0.0769230769230769,-0.0615384615384615,-0.0461538461538462,
-0.0307692307692308,-0.0153846153846154,0.),(-1.,1.),.UNSPECIFIED.)
GEOMETRIC_REPRESENTATION_ITEM()
RATIONAL_B_SPLINE_SURFACE(((1.,1.),(1.,1.),(1.,1.),(1.,1.),(1.,1.),(1.,
1.),(1.,1.),(1.,1.),(1.,1.),(1.,1.),(1.,1.),(1.,1.),(1.,1.),(1.,1.),(1.,
1.),(1.,1.),(1.,1.),(1.,1.),(1.,1.),(1.,1.),(1.,1.),(1.,1.),(1.,1.),(1.,
1.),(1.,1.),(1.,1.),(1.,1.),(1.,1.),(1.,1.),(1.,1.),(1.,1.),(1.,1.),(1.,
1.),(1.,1.),(1.,1.),(1.,1.),(1.,1.),(1.,1.),(1.,1.),(1.,1.),(1.,1.),(1.,
1.),(1.,1.),(1.,1.),(1.,1.),(1.,1.),(1.,1.),(1.,1.),(1.,1.),(1.,1.),(1.,
1.),(1.,1.),(1.,1.),(1.,1.),(1.,1.),(1.,1.),(1.,1.),(1.,1.),(1.,1.),(1.,
1.),(1.,1.),(1.,1.),(1.,1.),(1.,1.),(1.,1.),(1.,1.),(1.,1.),(1.,1.),(1.,
1.),(1.,1.)))
REPRESENTATION_ITEM('')
SURFACE()
);
#101=(
BOUNDED_SURFACE()
B_SPLINE_SURFACE(5,1,((#57695,#57696),(#57697,#57698),(#57699,#57700),(#57701,
#57702),(#57703,#57704),(#57705,#57706),(#57707,#57708),(#57709,#57710),
(#57711,#57712),(#57713,#57714),(#57715,#57716),(#57717,#57718),(#57719,
#57720),(#57721,#57722),(#57723,#57724),(#57725,#57726),(#57727,#57728),
(#57729,#57730),(#57731,#57732),(#57733,#57734),(#57735,#57736),(#57737,
#57738),(#57739,#57740),(#57741,#57742),(#57743,#57744),(#57745,#57746),
(#57747,#57748),(#57749,#57750),(#57751,#57752),(#57753,#57754),(#57755,
#57756),(#57757,#57758),(#57759,#57760),(#57761,#57762),(#57763,#57764),
(#57765,#57766),(#57767,#57768),(#57769,#57770),(#57771,#57772),(#57773,
#57774),(#57775,#57776),(#57777,#57778),(#57779,#57780),(#57781,#57782),
(#57783,#57784),(#57785,#57786),(#57787,#57788),(#57789,#57790),(#57791,
#57792),(#57793,#57794),(#57795,#57796),(#57797,#57798),(#57799,#57800),
(#57801,#57802),(#57803,#57804),(#57805,#57806),(#57807,#57808),(#57809,
#57810),(#57811,#57812),(#57813,#57814),(#57815,#57816),(#57817,#57818),
(#57819,#57820),(#57821,#57822),(#57823,#57824),(#57825,#57826),(#57827,
#57828),(#57829,#57830),(#57831,#57832),(#57833,#57834)),.UNSPECIFIED.,
 .F.,.F.,.F.)
B_SPLINE_SURFACE_WITH_KNOTS((6,1,1,1,1,1,1,1,1,1,1,1,1,1,1,1,1,1,1,1,1,
1,1,1,1,1,1,1,1,1,1,1,1,1,1,1,1,1,1,1,1,1,1,1,1,1,1,1,1,1,1,1,1,1,1,1,1,
1,1,1,1,1,1,1,1,6),(2,2),(-1.,-0.984615384615383,-0.969230769230768,-0.953846153846152,
-0.938461538461537,-0.923076923076922,-0.907692307692306,-0.892307692307691,
-0.876923076923076,-0.86153846153846,-0.846153846153845,-0.83076923076923,
-0.815384615384614,-0.799999999999999,-0.784615384615384,-0.769230769230768,
-0.753846153846153,-0.738461538461538,-0.723076923076922,-0.707692307692307,
-0.692307692307692,-0.676923076923076,-0.661538461538461,-0.646153846153846,
-0.63076923076923,-0.615384615384615,-0.6,-0.584615384615384,-0.569230769230769,
-0.553846153846154,-0.538461538461538,-0.523076923076923,-0.507692307692308,
-0.492307692307692,-0.476923076923077,-0.461538461538462,-0.446153846153846,
-0.430769230769231,-0.415384615384615,-0.4,-0.384615384615385,-0.369230769230769,
-0.353846153846154,-0.338461538461538,-0.323076923076923,-0.307692307692308,
-0.292307692307692,-0.276923076923077,-0.261538461538462,-0.246153846153846,
-0.230769230769231,-0.215384615384615,-0.2,-0.184615384615385,-0.169230769230769,
-0.153846153846154,-0.138461538461538,-0.123076923076923,-0.107692307692308,
-0.0923076923076923,-0.0769230769230769,-0.0615384615384615,-0.0461538461538462,
-0.0307692307692308,-0.0153846153846154,0.),(-1.,1.),.UNSPECIFIED.)
GEOMETRIC_REPRESENTATION_ITEM()
RATIONAL_B_SPLINE_SURFACE(((1.,1.),(1.,1.),(1.,1.),(1.,1.),(1.,1.),(1.,
1.),(1.,1.),(1.,1.),(1.,1.),(1.,1.),(1.,1.),(1.,1.),(1.,1.),(1.,1.),(1.,
1.),(1.,1.),(1.,1.),(1.,1.),(1.,1.),(1.,1.),(1.,1.),(1.,1.),(1.,1.),(1.,
1.),(1.,1.),(1.,1.),(1.,1.),(1.,1.),(1.,1.),(1.,1.),(1.,1.),(1.,1.),(1.,
1.),(1.,1.),(1.,1.),(1.,1.),(1.,1.),(1.,1.),(1.,1.),(1.,1.),(1.,1.),(1.,
1.),(1.,1.),(1.,1.),(1.,1.),(1.,1.),(1.,1.),(1.,1.),(1.,1.),(1.,1.),(1.,
1.),(1.,1.),(1.,1.),(1.,1.),(1.,1.),(1.,1.),(1.,1.),(1.,1.),(1.,1.),(1.,
1.),(1.,1.),(1.,1.),(1.,1.),(1.,1.),(1.,1.),(1.,1.),(1.,1.),(1.,1.),(1.,
1.),(1.,1.)))
REPRESENTATION_ITEM('')
SURFACE()
);
#102=(
BOUNDED_SURFACE()
B_SPLINE_SURFACE(5,1,((#57907,#57908),(#57909,#57910),(#57911,#57912),(#57913,
#57914),(#57915,#57916),(#57917,#57918),(#57919,#57920),(#57921,#57922),
(#57923,#57924),(#57925,#57926),(#57927,#57928),(#57929,#57930),(#57931,
#57932),(#57933,#57934),(#57935,#57936),(#57937,#57938),(#57939,#57940),
(#57941,#57942),(#57943,#57944),(#57945,#57946),(#57947,#57948),(#57949,
#57950),(#57951,#57952),(#57953,#57954),(#57955,#57956),(#57957,#57958),
(#57959,#57960),(#57961,#57962),(#57963,#57964),(#57965,#57966),(#57967,
#57968),(#57969,#57970),(#57971,#57972),(#57973,#57974),(#57975,#57976),
(#57977,#57978),(#57979,#57980),(#57981,#57982),(#57983,#57984),(#57985,
#57986),(#57987,#57988),(#57989,#57990),(#57991,#57992),(#57993,#57994),
(#57995,#57996),(#57997,#57998),(#57999,#58000),(#58001,#58002),(#58003,
#58004),(#58005,#58006),(#58007,#58008),(#58009,#58010),(#58011,#58012),
(#58013,#58014),(#58015,#58016),(#58017,#58018),(#58019,#58020),(#58021,
#58022),(#58023,#58024),(#58025,#58026),(#58027,#58028),(#58029,#58030),
(#58031,#58032),(#58033,#58034),(#58035,#58036),(#58037,#58038),(#58039,
#58040),(#58041,#58042),(#58043,#58044),(#58045,#58046)),.UNSPECIFIED.,
 .F.,.F.,.F.)
B_SPLINE_SURFACE_WITH_KNOTS((6,1,1,1,1,1,1,1,1,1,1,1,1,1,1,1,1,1,1,1,1,
1,1,1,1,1,1,1,1,1,1,1,1,1,1,1,1,1,1,1,1,1,1,1,1,1,1,1,1,1,1,1,1,1,1,1,1,
1,1,1,1,1,1,1,1,6),(2,2),(-1.,-0.984615384615383,-0.969230769230768,-0.953846153846152,
-0.938461538461537,-0.923076923076922,-0.907692307692306,-0.892307692307691,
-0.876923076923076,-0.86153846153846,-0.846153846153845,-0.83076923076923,
-0.815384615384614,-0.799999999999999,-0.784615384615384,-0.769230769230768,
-0.753846153846153,-0.738461538461538,-0.723076923076922,-0.707692307692307,
-0.692307692307692,-0.676923076923076,-0.661538461538461,-0.646153846153846,
-0.63076923076923,-0.615384615384615,-0.6,-0.584615384615384,-0.569230769230769,
-0.553846153846154,-0.538461538461538,-0.523076923076923,-0.507692307692308,
-0.492307692307692,-0.476923076923077,-0.461538461538462,-0.446153846153846,
-0.430769230769231,-0.415384615384615,-0.4,-0.384615384615385,-0.369230769230769,
-0.353846153846154,-0.338461538461538,-0.323076923076923,-0.307692307692308,
-0.292307692307692,-0.276923076923077,-0.261538461538462,-0.246153846153846,
-0.230769230769231,-0.215384615384615,-0.2,-0.184615384615385,-0.169230769230769,
-0.153846153846154,-0.138461538461538,-0.123076923076923,-0.107692307692308,
-0.0923076923076923,-0.0769230769230769,-0.0615384615384615,-0.0461538461538462,
-0.0307692307692308,-0.0153846153846154,0.),(-1.,1.),.UNSPECIFIED.)
GEOMETRIC_REPRESENTATION_ITEM()
RATIONAL_B_SPLINE_SURFACE(((1.,1.),(1.,1.),(1.,1.),(1.,1.),(1.,1.),(1.,
1.),(1.,1.),(1.,1.),(1.,1.),(1.,1.),(1.,1.),(1.,1.),(1.,1.),(1.,1.),(1.,
1.),(1.,1.),(1.,1.),(1.,1.),(1.,1.),(1.,1.),(1.,1.),(1.,1.),(1.,1.),(1.,
1.),(1.,1.),(1.,1.),(1.,1.),(1.,1.),(1.,1.),(1.,1.),(1.,1.),(1.,1.),(1.,
1.),(1.,1.),(1.,1.),(1.,1.),(1.,1.),(1.,1.),(1.,1.),(1.,1.),(1.,1.),(1.,
1.),(1.,1.),(1.,1.),(1.,1.),(1.,1.),(1.,1.),(1.,1.),(1.,1.),(1.,1.),(1.,
1.),(1.,1.),(1.,1.),(1.,1.),(1.,1.),(1.,1.),(1.,1.),(1.,1.),(1.,1.),(1.,
1.),(1.,1.),(1.,1.),(1.,1.),(1.,1.),(1.,1.),(1.,1.),(1.,1.),(1.,1.),(1.,
1.),(1.,1.)))
REPRESENTATION_ITEM('')
SURFACE()
);
#103=(
BOUNDED_SURFACE()
B_SPLINE_SURFACE(5,1,((#58137,#58138),(#58139,#58140),(#58141,#58142),(#58143,
#58144),(#58145,#58146),(#58147,#58148),(#58149,#58150),(#58151,#58152),
(#58153,#58154),(#58155,#58156),(#58157,#58158),(#58159,#58160),(#58161,
#58162),(#58163,#58164),(#58165,#58166),(#58167,#58168),(#58169,#58170),
(#58171,#58172),(#58173,#58174),(#58175,#58176),(#58177,#58178),(#58179,
#58180),(#58181,#58182),(#58183,#58184),(#58185,#58186),(#58187,#58188),
(#58189,#58190),(#58191,#58192),(#58193,#58194),(#58195,#58196),(#58197,
#58198),(#58199,#58200),(#58201,#58202),(#58203,#58204),(#58205,#58206),
(#58207,#58208),(#58209,#58210),(#58211,#58212),(#58213,#58214),(#58215,
#58216),(#58217,#58218),(#58219,#58220),(#58221,#58222),(#58223,#58224),
(#58225,#58226),(#58227,#58228),(#58229,#58230),(#58231,#58232),(#58233,
#58234),(#58235,#58236),(#58237,#58238),(#58239,#58240),(#58241,#58242),
(#58243,#58244),(#58245,#58246),(#58247,#58248),(#58249,#58250),(#58251,
#58252),(#58253,#58254),(#58255,#58256),(#58257,#58258),(#58259,#58260),
(#58261,#58262),(#58263,#58264),(#58265,#58266),(#58267,#58268),(#58269,
#58270),(#58271,#58272),(#58273,#58274),(#58275,#58276)),.UNSPECIFIED.,
 .F.,.F.,.F.)
B_SPLINE_SURFACE_WITH_KNOTS((6,1,1,1,1,1,1,1,1,1,1,1,1,1,1,1,1,1,1,1,1,
1,1,1,1,1,1,1,1,1,1,1,1,1,1,1,1,1,1,1,1,1,1,1,1,1,1,1,1,1,1,1,1,1,1,1,1,
1,1,1,1,1,1,1,1,6),(2,2),(-1.,-0.984615384615383,-0.969230769230768,-0.953846153846152,
-0.938461538461537,-0.923076923076922,-0.907692307692306,-0.892307692307691,
-0.876923076923076,-0.86153846153846,-0.846153846153845,-0.83076923076923,
-0.815384615384614,-0.799999999999999,-0.784615384615384,-0.769230769230768,
-0.753846153846153,-0.738461538461538,-0.723076923076922,-0.707692307692307,
-0.692307692307692,-0.676923076923076,-0.661538461538461,-0.646153846153846,
-0.63076923076923,-0.615384615384615,-0.6,-0.584615384615384,-0.569230769230769,
-0.553846153846154,-0.538461538461538,-0.523076923076923,-0.507692307692308,
-0.492307692307692,-0.476923076923077,-0.461538461538462,-0.446153846153846,
-0.430769230769231,-0.415384615384615,-0.4,-0.384615384615385,-0.369230769230769,
-0.353846153846154,-0.338461538461538,-0.323076923076923,-0.307692307692308,
-0.292307692307692,-0.276923076923077,-0.261538461538462,-0.246153846153846,
-0.230769230769231,-0.215384615384615,-0.2,-0.184615384615385,-0.169230769230769,
-0.153846153846154,-0.138461538461538,-0.123076923076923,-0.107692307692308,
-0.0923076923076923,-0.0769230769230769,-0.0615384615384615,-0.0461538461538462,
-0.0307692307692308,-0.0153846153846154,0.),(-1.,1.),.UNSPECIFIED.)
GEOMETRIC_REPRESENTATION_ITEM()
RATIONAL_B_SPLINE_SURFACE(((1.,1.),(1.,1.),(1.,1.),(1.,1.),(1.,1.),(1.,
1.),(1.,1.),(1.,1.),(1.,1.),(1.,1.),(1.,1.),(1.,1.),(1.,1.),(1.,1.),(1.,
1.),(1.,1.),(1.,1.),(1.,1.),(1.,1.),(1.,1.),(1.,1.),(1.,1.),(1.,1.),(1.,
1.),(1.,1.),(1.,1.),(1.,1.),(1.,1.),(1.,1.),(1.,1.),(1.,1.),(1.,1.),(1.,
1.),(1.,1.),(1.,1.),(1.,1.),(1.,1.),(1.,1.),(1.,1.),(1.,1.),(1.,1.),(1.,
1.),(1.,1.),(1.,1.),(1.,1.),(1.,1.),(1.,1.),(1.,1.),(1.,1.),(1.,1.),(1.,
1.),(1.,1.),(1.,1.),(1.,1.),(1.,1.),(1.,1.),(1.,1.),(1.,1.),(1.,1.),(1.,
1.),(1.,1.),(1.,1.),(1.,1.),(1.,1.),(1.,1.),(1.,1.),(1.,1.),(1.,1.),(1.,
1.),(1.,1.)))
REPRESENTATION_ITEM('')
SURFACE()
);
#104=(
BOUNDED_SURFACE()
B_SPLINE_SURFACE(5,1,((#58349,#58350),(#58351,#58352),(#58353,#58354),(#58355,
#58356),(#58357,#58358),(#58359,#58360),(#58361,#58362),(#58363,#58364),
(#58365,#58366),(#58367,#58368),(#58369,#58370),(#58371,#58372),(#58373,
#58374),(#58375,#58376),(#58377,#58378),(#58379,#58380),(#58381,#58382),
(#58383,#58384),(#58385,#58386),(#58387,#58388),(#58389,#58390),(#58391,
#58392),(#58393,#58394),(#58395,#58396),(#58397,#58398),(#58399,#58400),
(#58401,#58402),(#58403,#58404),(#58405,#58406),(#58407,#58408),(#58409,
#58410),(#58411,#58412),(#58413,#58414),(#58415,#58416),(#58417,#58418),
(#58419,#58420),(#58421,#58422),(#58423,#58424),(#58425,#58426),(#58427,
#58428),(#58429,#58430),(#58431,#58432),(#58433,#58434),(#58435,#58436),
(#58437,#58438),(#58439,#58440),(#58441,#58442),(#58443,#58444),(#58445,
#58446),(#58447,#58448),(#58449,#58450),(#58451,#58452),(#58453,#58454),
(#58455,#58456),(#58457,#58458),(#58459,#58460),(#58461,#58462),(#58463,
#58464),(#58465,#58466),(#58467,#58468),(#58469,#58470),(#58471,#58472),
(#58473,#58474),(#58475,#58476),(#58477,#58478),(#58479,#58480),(#58481,
#58482),(#58483,#58484),(#58485,#58486),(#58487,#58488)),.UNSPECIFIED.,
 .F.,.F.,.F.)
B_SPLINE_SURFACE_WITH_KNOTS((6,1,1,1,1,1,1,1,1,1,1,1,1,1,1,1,1,1,1,1,1,
1,1,1,1,1,1,1,1,1,1,1,1,1,1,1,1,1,1,1,1,1,1,1,1,1,1,1,1,1,1,1,1,1,1,1,1,
1,1,1,1,1,1,1,1,6),(2,2),(-1.,-0.984615384615383,-0.969230769230768,-0.953846153846152,
-0.938461538461537,-0.923076923076922,-0.907692307692306,-0.892307692307691,
-0.876923076923076,-0.86153846153846,-0.846153846153845,-0.83076923076923,
-0.815384615384614,-0.799999999999999,-0.784615384615384,-0.769230769230768,
-0.753846153846153,-0.738461538461538,-0.723076923076922,-0.707692307692307,
-0.692307692307692,-0.676923076923076,-0.661538461538461,-0.646153846153846,
-0.63076923076923,-0.615384615384615,-0.6,-0.584615384615384,-0.569230769230769,
-0.553846153846154,-0.538461538461538,-0.523076923076923,-0.507692307692308,
-0.492307692307692,-0.476923076923077,-0.461538461538462,-0.446153846153846,
-0.430769230769231,-0.415384615384615,-0.4,-0.384615384615385,-0.369230769230769,
-0.353846153846154,-0.338461538461538,-0.323076923076923,-0.307692307692308,
-0.292307692307692,-0.276923076923077,-0.261538461538462,-0.246153846153846,
-0.230769230769231,-0.215384615384615,-0.2,-0.184615384615385,-0.169230769230769,
-0.153846153846154,-0.138461538461538,-0.123076923076923,-0.107692307692308,
-0.0923076923076923,-0.0769230769230769,-0.0615384615384615,-0.0461538461538462,
-0.0307692307692308,-0.0153846153846154,0.),(-1.,1.),.UNSPECIFIED.)
GEOMETRIC_REPRESENTATION_ITEM()
RATIONAL_B_SPLINE_SURFACE(((1.,1.),(1.,1.),(1.,1.),(1.,1.),(1.,1.),(1.,
1.),(1.,1.),(1.,1.),(1.,1.),(1.,1.),(1.,1.),(1.,1.),(1.,1.),(1.,1.),(1.,
1.),(1.,1.),(1.,1.),(1.,1.),(1.,1.),(1.,1.),(1.,1.),(1.,1.),(1.,1.),(1.,
1.),(1.,1.),(1.,1.),(1.,1.),(1.,1.),(1.,1.),(1.,1.),(1.,1.),(1.,1.),(1.,
1.),(1.,1.),(1.,1.),(1.,1.),(1.,1.),(1.,1.),(1.,1.),(1.,1.),(1.,1.),(1.,
1.),(1.,1.),(1.,1.),(1.,1.),(1.,1.),(1.,1.),(1.,1.),(1.,1.),(1.,1.),(1.,
1.),(1.,1.),(1.,1.),(1.,1.),(1.,1.),(1.,1.),(1.,1.),(1.,1.),(1.,1.),(1.,
1.),(1.,1.),(1.,1.),(1.,1.),(1.,1.),(1.,1.),(1.,1.),(1.,1.),(1.,1.),(1.,
1.),(1.,1.)))
REPRESENTATION_ITEM('')
SURFACE()
);
#105=(
BOUNDED_SURFACE()
B_SPLINE_SURFACE(5,1,((#58579,#58580),(#58581,#58582),(#58583,#58584),(#58585,
#58586),(#58587,#58588),(#58589,#58590),(#58591,#58592),(#58593,#58594),
(#58595,#58596),(#58597,#58598),(#58599,#58600),(#58601,#58602),(#58603,
#58604),(#58605,#58606),(#58607,#58608),(#58609,#58610),(#58611,#58612),
(#58613,#58614),(#58615,#58616),(#58617,#58618),(#58619,#58620),(#58621,
#58622),(#58623,#58624),(#58625,#58626),(#58627,#58628),(#58629,#58630),
(#58631,#58632),(#58633,#58634),(#58635,#58636),(#58637,#58638),(#58639,
#58640),(#58641,#58642),(#58643,#58644),(#58645,#58646),(#58647,#58648),
(#58649,#58650),(#58651,#58652),(#58653,#58654),(#58655,#58656),(#58657,
#58658),(#58659,#58660),(#58661,#58662),(#58663,#58664),(#58665,#58666),
(#58667,#58668),(#58669,#58670),(#58671,#58672),(#58673,#58674),(#58675,
#58676),(#58677,#58678),(#58679,#58680),(#58681,#58682),(#58683,#58684),
(#58685,#58686),(#58687,#58688),(#58689,#58690),(#58691,#58692),(#58693,
#58694),(#58695,#58696),(#58697,#58698),(#58699,#58700),(#58701,#58702),
(#58703,#58704),(#58705,#58706),(#58707,#58708),(#58709,#58710),(#58711,
#58712),(#58713,#58714),(#58715,#58716),(#58717,#58718)),.UNSPECIFIED.,
 .F.,.F.,.F.)
B_SPLINE_SURFACE_WITH_KNOTS((6,1,1,1,1,1,1,1,1,1,1,1,1,1,1,1,1,1,1,1,1,
1,1,1,1,1,1,1,1,1,1,1,1,1,1,1,1,1,1,1,1,1,1,1,1,1,1,1,1,1,1,1,1,1,1,1,1,
1,1,1,1,1,1,1,1,6),(2,2),(-1.,-0.984615384615383,-0.969230769230768,-0.953846153846152,
-0.938461538461537,-0.923076923076922,-0.907692307692306,-0.892307692307691,
-0.876923076923076,-0.86153846153846,-0.846153846153845,-0.83076923076923,
-0.815384615384614,-0.799999999999999,-0.784615384615384,-0.769230769230768,
-0.753846153846153,-0.738461538461538,-0.723076923076922,-0.707692307692307,
-0.692307692307692,-0.676923076923076,-0.661538461538461,-0.646153846153846,
-0.63076923076923,-0.615384615384615,-0.6,-0.584615384615384,-0.569230769230769,
-0.553846153846154,-0.538461538461538,-0.523076923076923,-0.507692307692308,
-0.492307692307692,-0.476923076923077,-0.461538461538462,-0.446153846153846,
-0.430769230769231,-0.415384615384615,-0.4,-0.384615384615385,-0.369230769230769,
-0.353846153846154,-0.338461538461538,-0.323076923076923,-0.307692307692308,
-0.292307692307692,-0.276923076923077,-0.261538461538462,-0.246153846153846,
-0.230769230769231,-0.215384615384615,-0.2,-0.184615384615385,-0.169230769230769,
-0.153846153846154,-0.138461538461538,-0.123076923076923,-0.107692307692308,
-0.0923076923076923,-0.0769230769230769,-0.0615384615384615,-0.0461538461538462,
-0.0307692307692308,-0.0153846153846154,0.),(-1.,1.),.UNSPECIFIED.)
GEOMETRIC_REPRESENTATION_ITEM()
RATIONAL_B_SPLINE_SURFACE(((1.,1.),(1.,1.),(1.,1.),(1.,1.),(1.,1.),(1.,
1.),(1.,1.),(1.,1.),(1.,1.),(1.,1.),(1.,1.),(1.,1.),(1.,1.),(1.,1.),(1.,
1.),(1.,1.),(1.,1.),(1.,1.),(1.,1.),(1.,1.),(1.,1.),(1.,1.),(1.,1.),(1.,
1.),(1.,1.),(1.,1.),(1.,1.),(1.,1.),(1.,1.),(1.,1.),(1.,1.),(1.,1.),(1.,
1.),(1.,1.),(1.,1.),(1.,1.),(1.,1.),(1.,1.),(1.,1.),(1.,1.),(1.,1.),(1.,
1.),(1.,1.),(1.,1.),(1.,1.),(1.,1.),(1.,1.),(1.,1.),(1.,1.),(1.,1.),(1.,
1.),(1.,1.),(1.,1.),(1.,1.),(1.,1.),(1.,1.),(1.,1.),(1.,1.),(1.,1.),(1.,
1.),(1.,1.),(1.,1.),(1.,1.),(1.,1.),(1.,1.),(1.,1.),(1.,1.),(1.,1.),(1.,
1.),(1.,1.)))
REPRESENTATION_ITEM('')
SURFACE()
);
#106=(
BOUNDED_SURFACE()
B_SPLINE_SURFACE(5,1,((#58791,#58792),(#58793,#58794),(#58795,#58796),(#58797,
#58798),(#58799,#58800),(#58801,#58802),(#58803,#58804),(#58805,#58806),
(#58807,#58808),(#58809,#58810),(#58811,#58812),(#58813,#58814),(#58815,
#58816),(#58817,#58818),(#58819,#58820),(#58821,#58822),(#58823,#58824),
(#58825,#58826),(#58827,#58828),(#58829,#58830),(#58831,#58832),(#58833,
#58834),(#58835,#58836),(#58837,#58838),(#58839,#58840),(#58841,#58842),
(#58843,#58844),(#58845,#58846),(#58847,#58848),(#58849,#58850),(#58851,
#58852),(#58853,#58854),(#58855,#58856),(#58857,#58858),(#58859,#58860),
(#58861,#58862),(#58863,#58864),(#58865,#58866),(#58867,#58868),(#58869,
#58870),(#58871,#58872),(#58873,#58874),(#58875,#58876),(#58877,#58878),
(#58879,#58880),(#58881,#58882),(#58883,#58884),(#58885,#58886),(#58887,
#58888),(#58889,#58890),(#58891,#58892),(#58893,#58894),(#58895,#58896),
(#58897,#58898),(#58899,#58900),(#58901,#58902),(#58903,#58904),(#58905,
#58906),(#58907,#58908),(#58909,#58910),(#58911,#58912),(#58913,#58914),
(#58915,#58916),(#58917,#58918),(#58919,#58920),(#58921,#58922),(#58923,
#58924),(#58925,#58926),(#58927,#58928),(#58929,#58930)),.UNSPECIFIED.,
 .F.,.F.,.F.)
B_SPLINE_SURFACE_WITH_KNOTS((6,1,1,1,1,1,1,1,1,1,1,1,1,1,1,1,1,1,1,1,1,
1,1,1,1,1,1,1,1,1,1,1,1,1,1,1,1,1,1,1,1,1,1,1,1,1,1,1,1,1,1,1,1,1,1,1,1,
1,1,1,1,1,1,1,1,6),(2,2),(-1.,-0.984615384615383,-0.969230769230768,-0.953846153846152,
-0.938461538461537,-0.923076923076922,-0.907692307692306,-0.892307692307691,
-0.876923076923076,-0.86153846153846,-0.846153846153845,-0.83076923076923,
-0.815384615384614,-0.799999999999999,-0.784615384615384,-0.769230769230768,
-0.753846153846153,-0.738461538461538,-0.723076923076922,-0.707692307692307,
-0.692307692307692,-0.676923076923076,-0.661538461538461,-0.646153846153846,
-0.63076923076923,-0.615384615384615,-0.6,-0.584615384615384,-0.569230769230769,
-0.553846153846154,-0.538461538461538,-0.523076923076923,-0.507692307692308,
-0.492307692307692,-0.476923076923077,-0.461538461538462,-0.446153846153846,
-0.430769230769231,-0.415384615384615,-0.4,-0.384615384615385,-0.369230769230769,
-0.353846153846154,-0.338461538461538,-0.323076923076923,-0.307692307692308,
-0.292307692307692,-0.276923076923077,-0.261538461538462,-0.246153846153846,
-0.230769230769231,-0.215384615384615,-0.2,-0.184615384615385,-0.169230769230769,
-0.153846153846154,-0.138461538461538,-0.123076923076923,-0.107692307692308,
-0.0923076923076923,-0.0769230769230769,-0.0615384615384615,-0.0461538461538462,
-0.0307692307692308,-0.0153846153846154,0.),(-1.,1.),.UNSPECIFIED.)
GEOMETRIC_REPRESENTATION_ITEM()
RATIONAL_B_SPLINE_SURFACE(((1.,1.),(1.,1.),(1.,1.),(1.,1.),(1.,1.),(1.,
1.),(1.,1.),(1.,1.),(1.,1.),(1.,1.),(1.,1.),(1.,1.),(1.,1.),(1.,1.),(1.,
1.),(1.,1.),(1.,1.),(1.,1.),(1.,1.),(1.,1.),(1.,1.),(1.,1.),(1.,1.),(1.,
1.),(1.,1.),(1.,1.),(1.,1.),(1.,1.),(1.,1.),(1.,1.),(1.,1.),(1.,1.),(1.,
1.),(1.,1.),(1.,1.),(1.,1.),(1.,1.),(1.,1.),(1.,1.),(1.,1.),(1.,1.),(1.,
1.),(1.,1.),(1.,1.),(1.,1.),(1.,1.),(1.,1.),(1.,1.),(1.,1.),(1.,1.),(1.,
1.),(1.,1.),(1.,1.),(1.,1.),(1.,1.),(1.,1.),(1.,1.),(1.,1.),(1.,1.),(1.,
1.),(1.,1.),(1.,1.),(1.,1.),(1.,1.),(1.,1.),(1.,1.),(1.,1.),(1.,1.),(1.,
1.),(1.,1.)))
REPRESENTATION_ITEM('')
SURFACE()
);
#107=(
BOUNDED_SURFACE()
B_SPLINE_SURFACE(5,1,((#59021,#59022),(#59023,#59024),(#59025,#59026),(#59027,
#59028),(#59029,#59030),(#59031,#59032),(#59033,#59034),(#59035,#59036),
(#59037,#59038),(#59039,#59040),(#59041,#59042),(#59043,#59044),(#59045,
#59046),(#59047,#59048),(#59049,#59050),(#59051,#59052),(#59053,#59054),
(#59055,#59056),(#59057,#59058),(#59059,#59060),(#59061,#59062),(#59063,
#59064),(#59065,#59066),(#59067,#59068),(#59069,#59070),(#59071,#59072),
(#59073,#59074),(#59075,#59076),(#59077,#59078),(#59079,#59080),(#59081,
#59082),(#59083,#59084),(#59085,#59086),(#59087,#59088),(#59089,#59090),
(#59091,#59092),(#59093,#59094),(#59095,#59096),(#59097,#59098),(#59099,
#59100),(#59101,#59102),(#59103,#59104),(#59105,#59106),(#59107,#59108),
(#59109,#59110),(#59111,#59112),(#59113,#59114),(#59115,#59116),(#59117,
#59118),(#59119,#59120),(#59121,#59122),(#59123,#59124),(#59125,#59126),
(#59127,#59128),(#59129,#59130),(#59131,#59132),(#59133,#59134),(#59135,
#59136),(#59137,#59138),(#59139,#59140),(#59141,#59142),(#59143,#59144),
(#59145,#59146),(#59147,#59148),(#59149,#59150),(#59151,#59152),(#59153,
#59154),(#59155,#59156),(#59157,#59158),(#59159,#59160)),.UNSPECIFIED.,
 .F.,.F.,.F.)
B_SPLINE_SURFACE_WITH_KNOTS((6,1,1,1,1,1,1,1,1,1,1,1,1,1,1,1,1,1,1,1,1,
1,1,1,1,1,1,1,1,1,1,1,1,1,1,1,1,1,1,1,1,1,1,1,1,1,1,1,1,1,1,1,1,1,1,1,1,
1,1,1,1,1,1,1,1,6),(2,2),(-1.,-0.984615384615383,-0.969230769230768,-0.953846153846152,
-0.938461538461537,-0.923076923076922,-0.907692307692306,-0.892307692307691,
-0.876923076923076,-0.86153846153846,-0.846153846153845,-0.83076923076923,
-0.815384615384614,-0.799999999999999,-0.784615384615384,-0.769230769230768,
-0.753846153846153,-0.738461538461538,-0.723076923076922,-0.707692307692307,
-0.692307692307692,-0.676923076923076,-0.661538461538461,-0.646153846153846,
-0.63076923076923,-0.615384615384615,-0.6,-0.584615384615384,-0.569230769230769,
-0.553846153846154,-0.538461538461538,-0.523076923076923,-0.507692307692308,
-0.492307692307692,-0.476923076923077,-0.461538461538462,-0.446153846153846,
-0.430769230769231,-0.415384615384615,-0.4,-0.384615384615385,-0.369230769230769,
-0.353846153846154,-0.338461538461538,-0.323076923076923,-0.307692307692308,
-0.292307692307692,-0.276923076923077,-0.261538461538462,-0.246153846153846,
-0.230769230769231,-0.215384615384615,-0.2,-0.184615384615385,-0.169230769230769,
-0.153846153846154,-0.138461538461538,-0.123076923076923,-0.107692307692308,
-0.0923076923076923,-0.0769230769230769,-0.0615384615384615,-0.0461538461538462,
-0.0307692307692308,-0.0153846153846154,0.),(-1.,1.),.UNSPECIFIED.)
GEOMETRIC_REPRESENTATION_ITEM()
RATIONAL_B_SPLINE_SURFACE(((1.,1.),(1.,1.),(1.,1.),(1.,1.),(1.,1.),(1.,
1.),(1.,1.),(1.,1.),(1.,1.),(1.,1.),(1.,1.),(1.,1.),(1.,1.),(1.,1.),(1.,
1.),(1.,1.),(1.,1.),(1.,1.),(1.,1.),(1.,1.),(1.,1.),(1.,1.),(1.,1.),(1.,
1.),(1.,1.),(1.,1.),(1.,1.),(1.,1.),(1.,1.),(1.,1.),(1.,1.),(1.,1.),(1.,
1.),(1.,1.),(1.,1.),(1.,1.),(1.,1.),(1.,1.),(1.,1.),(1.,1.),(1.,1.),(1.,
1.),(1.,1.),(1.,1.),(1.,1.),(1.,1.),(1.,1.),(1.,1.),(1.,1.),(1.,1.),(1.,
1.),(1.,1.),(1.,1.),(1.,1.),(1.,1.),(1.,1.),(1.,1.),(1.,1.),(1.,1.),(1.,
1.),(1.,1.),(1.,1.),(1.,1.),(1.,1.),(1.,1.),(1.,1.),(1.,1.),(1.,1.),(1.,
1.),(1.,1.)))
REPRESENTATION_ITEM('')
SURFACE()
);
#108=(
BOUNDED_SURFACE()
B_SPLINE_SURFACE(5,1,((#59233,#59234),(#59235,#59236),(#59237,#59238),(#59239,
#59240),(#59241,#59242),(#59243,#59244),(#59245,#59246),(#59247,#59248),
(#59249,#59250),(#59251,#59252),(#59253,#59254),(#59255,#59256),(#59257,
#59258),(#59259,#59260),(#59261,#59262),(#59263,#59264),(#59265,#59266),
(#59267,#59268),(#59269,#59270),(#59271,#59272),(#59273,#59274),(#59275,
#59276),(#59277,#59278),(#59279,#59280),(#59281,#59282),(#59283,#59284),
(#59285,#59286),(#59287,#59288),(#59289,#59290),(#59291,#59292),(#59293,
#59294),(#59295,#59296),(#59297,#59298),(#59299,#59300),(#59301,#59302),
(#59303,#59304),(#59305,#59306),(#59307,#59308),(#59309,#59310),(#59311,
#59312),(#59313,#59314),(#59315,#59316),(#59317,#59318),(#59319,#59320),
(#59321,#59322),(#59323,#59324),(#59325,#59326),(#59327,#59328),(#59329,
#59330),(#59331,#59332),(#59333,#59334),(#59335,#59336),(#59337,#59338),
(#59339,#59340),(#59341,#59342),(#59343,#59344),(#59345,#59346),(#59347,
#59348),(#59349,#59350),(#59351,#59352),(#59353,#59354),(#59355,#59356),
(#59357,#59358),(#59359,#59360),(#59361,#59362),(#59363,#59364),(#59365,
#59366),(#59367,#59368),(#59369,#59370),(#59371,#59372)),.UNSPECIFIED.,
 .F.,.F.,.F.)
B_SPLINE_SURFACE_WITH_KNOTS((6,1,1,1,1,1,1,1,1,1,1,1,1,1,1,1,1,1,1,1,1,
1,1,1,1,1,1,1,1,1,1,1,1,1,1,1,1,1,1,1,1,1,1,1,1,1,1,1,1,1,1,1,1,1,1,1,1,
1,1,1,1,1,1,1,1,6),(2,2),(-1.,-0.984615384615383,-0.969230769230768,-0.953846153846152,
-0.938461538461537,-0.923076923076922,-0.907692307692306,-0.892307692307691,
-0.876923076923076,-0.86153846153846,-0.846153846153845,-0.83076923076923,
-0.815384615384614,-0.799999999999999,-0.784615384615384,-0.769230769230768,
-0.753846153846153,-0.738461538461538,-0.723076923076922,-0.707692307692307,
-0.692307692307692,-0.676923076923076,-0.661538461538461,-0.646153846153846,
-0.63076923076923,-0.615384615384615,-0.6,-0.584615384615384,-0.569230769230769,
-0.553846153846154,-0.538461538461538,-0.523076923076923,-0.507692307692308,
-0.492307692307692,-0.476923076923077,-0.461538461538462,-0.446153846153846,
-0.430769230769231,-0.415384615384615,-0.4,-0.384615384615385,-0.369230769230769,
-0.353846153846154,-0.338461538461538,-0.323076923076923,-0.307692307692308,
-0.292307692307692,-0.276923076923077,-0.261538461538462,-0.246153846153846,
-0.230769230769231,-0.215384615384615,-0.2,-0.184615384615385,-0.169230769230769,
-0.153846153846154,-0.138461538461538,-0.123076923076923,-0.107692307692308,
-0.0923076923076923,-0.0769230769230769,-0.0615384615384615,-0.0461538461538462,
-0.0307692307692308,-0.0153846153846154,0.),(-1.,1.),.UNSPECIFIED.)
GEOMETRIC_REPRESENTATION_ITEM()
RATIONAL_B_SPLINE_SURFACE(((1.,1.),(1.,1.),(1.,1.),(1.,1.),(1.,1.),(1.,
1.),(1.,1.),(1.,1.),(1.,1.),(1.,1.),(1.,1.),(1.,1.),(1.,1.),(1.,1.),(1.,
1.),(1.,1.),(1.,1.),(1.,1.),(1.,1.),(1.,1.),(1.,1.),(1.,1.),(1.,1.),(1.,
1.),(1.,1.),(1.,1.),(1.,1.),(1.,1.),(1.,1.),(1.,1.),(1.,1.),(1.,1.),(1.,
1.),(1.,1.),(1.,1.),(1.,1.),(1.,1.),(1.,1.),(1.,1.),(1.,1.),(1.,1.),(1.,
1.),(1.,1.),(1.,1.),(1.,1.),(1.,1.),(1.,1.),(1.,1.),(1.,1.),(1.,1.),(1.,
1.),(1.,1.),(1.,1.),(1.,1.),(1.,1.),(1.,1.),(1.,1.),(1.,1.),(1.,1.),(1.,
1.),(1.,1.),(1.,1.),(1.,1.),(1.,1.),(1.,1.),(1.,1.),(1.,1.),(1.,1.),(1.,
1.),(1.,1.)))
REPRESENTATION_ITEM('')
SURFACE()
);
#109=(
BOUNDED_SURFACE()
B_SPLINE_SURFACE(5,1,((#59463,#59464),(#59465,#59466),(#59467,#59468),(#59469,
#59470),(#59471,#59472),(#59473,#59474),(#59475,#59476),(#59477,#59478),
(#59479,#59480),(#59481,#59482),(#59483,#59484),(#59485,#59486),(#59487,
#59488),(#59489,#59490),(#59491,#59492),(#59493,#59494),(#59495,#59496),
(#59497,#59498),(#59499,#59500),(#59501,#59502),(#59503,#59504),(#59505,
#59506),(#59507,#59508),(#59509,#59510),(#59511,#59512),(#59513,#59514),
(#59515,#59516),(#59517,#59518),(#59519,#59520),(#59521,#59522),(#59523,
#59524),(#59525,#59526),(#59527,#59528),(#59529,#59530),(#59531,#59532),
(#59533,#59534),(#59535,#59536),(#59537,#59538),(#59539,#59540),(#59541,
#59542),(#59543,#59544),(#59545,#59546),(#59547,#59548),(#59549,#59550),
(#59551,#59552),(#59553,#59554),(#59555,#59556),(#59557,#59558),(#59559,
#59560),(#59561,#59562),(#59563,#59564),(#59565,#59566),(#59567,#59568),
(#59569,#59570),(#59571,#59572),(#59573,#59574),(#59575,#59576),(#59577,
#59578),(#59579,#59580),(#59581,#59582),(#59583,#59584),(#59585,#59586),
(#59587,#59588),(#59589,#59590),(#59591,#59592),(#59593,#59594),(#59595,
#59596),(#59597,#59598),(#59599,#59600),(#59601,#59602)),.UNSPECIFIED.,
 .F.,.F.,.F.)
B_SPLINE_SURFACE_WITH_KNOTS((6,1,1,1,1,1,1,1,1,1,1,1,1,1,1,1,1,1,1,1,1,
1,1,1,1,1,1,1,1,1,1,1,1,1,1,1,1,1,1,1,1,1,1,1,1,1,1,1,1,1,1,1,1,1,1,1,1,
1,1,1,1,1,1,1,1,6),(2,2),(-1.,-0.984615384615383,-0.969230769230768,-0.953846153846152,
-0.938461538461537,-0.923076923076922,-0.907692307692306,-0.892307692307691,
-0.876923076923076,-0.86153846153846,-0.846153846153845,-0.83076923076923,
-0.815384615384614,-0.799999999999999,-0.784615384615384,-0.769230769230768,
-0.753846153846153,-0.738461538461538,-0.723076923076922,-0.707692307692307,
-0.692307692307692,-0.676923076923076,-0.661538461538461,-0.646153846153846,
-0.63076923076923,-0.615384615384615,-0.6,-0.584615384615384,-0.569230769230769,
-0.553846153846154,-0.538461538461538,-0.523076923076923,-0.507692307692308,
-0.492307692307692,-0.476923076923077,-0.461538461538462,-0.446153846153846,
-0.430769230769231,-0.415384615384615,-0.4,-0.384615384615385,-0.369230769230769,
-0.353846153846154,-0.338461538461538,-0.323076923076923,-0.307692307692308,
-0.292307692307692,-0.276923076923077,-0.261538461538462,-0.246153846153846,
-0.230769230769231,-0.215384615384615,-0.2,-0.184615384615385,-0.169230769230769,
-0.153846153846154,-0.138461538461538,-0.123076923076923,-0.107692307692308,
-0.0923076923076923,-0.0769230769230769,-0.0615384615384615,-0.0461538461538462,
-0.0307692307692308,-0.0153846153846154,0.),(-1.,1.),.UNSPECIFIED.)
GEOMETRIC_REPRESENTATION_ITEM()
RATIONAL_B_SPLINE_SURFACE(((1.,1.),(1.,1.),(1.,1.),(1.,1.),(1.,1.),(1.,
1.),(1.,1.),(1.,1.),(1.,1.),(1.,1.),(1.,1.),(1.,1.),(1.,1.),(1.,1.),(1.,
1.),(1.,1.),(1.,1.),(1.,1.),(1.,1.),(1.,1.),(1.,1.),(1.,1.),(1.,1.),(1.,
1.),(1.,1.),(1.,1.),(1.,1.),(1.,1.),(1.,1.),(1.,1.),(1.,1.),(1.,1.),(1.,
1.),(1.,1.),(1.,1.),(1.,1.),(1.,1.),(1.,1.),(1.,1.),(1.,1.),(1.,1.),(1.,
1.),(1.,1.),(1.,1.),(1.,1.),(1.,1.),(1.,1.),(1.,1.),(1.,1.),(1.,1.),(1.,
1.),(1.,1.),(1.,1.),(1.,1.),(1.,1.),(1.,1.),(1.,1.),(1.,1.),(1.,1.),(1.,
1.),(1.,1.),(1.,1.),(1.,1.),(1.,1.),(1.,1.),(1.,1.),(1.,1.),(1.,1.),(1.,
1.),(1.,1.)))
REPRESENTATION_ITEM('')
SURFACE()
);
#110=(
BOUNDED_SURFACE()
B_SPLINE_SURFACE(5,1,((#59675,#59676),(#59677,#59678),(#59679,#59680),(#59681,
#59682),(#59683,#59684),(#59685,#59686),(#59687,#59688),(#59689,#59690),
(#59691,#59692),(#59693,#59694),(#59695,#59696),(#59697,#59698),(#59699,
#59700),(#59701,#59702),(#59703,#59704),(#59705,#59706),(#59707,#59708),
(#59709,#59710),(#59711,#59712),(#59713,#59714),(#59715,#59716),(#59717,
#59718),(#59719,#59720),(#59721,#59722),(#59723,#59724),(#59725,#59726),
(#59727,#59728),(#59729,#59730),(#59731,#59732),(#59733,#59734),(#59735,
#59736),(#59737,#59738),(#59739,#59740),(#59741,#59742),(#59743,#59744),
(#59745,#59746),(#59747,#59748),(#59749,#59750),(#59751,#59752),(#59753,
#59754),(#59755,#59756),(#59757,#59758),(#59759,#59760),(#59761,#59762),
(#59763,#59764),(#59765,#59766),(#59767,#59768),(#59769,#59770),(#59771,
#59772),(#59773,#59774),(#59775,#59776),(#59777,#59778),(#59779,#59780),
(#59781,#59782),(#59783,#59784),(#59785,#59786),(#59787,#59788),(#59789,
#59790),(#59791,#59792),(#59793,#59794),(#59795,#59796),(#59797,#59798),
(#59799,#59800),(#59801,#59802),(#59803,#59804),(#59805,#59806),(#59807,
#59808),(#59809,#59810),(#59811,#59812),(#59813,#59814)),.UNSPECIFIED.,
 .F.,.F.,.F.)
B_SPLINE_SURFACE_WITH_KNOTS((6,1,1,1,1,1,1,1,1,1,1,1,1,1,1,1,1,1,1,1,1,
1,1,1,1,1,1,1,1,1,1,1,1,1,1,1,1,1,1,1,1,1,1,1,1,1,1,1,1,1,1,1,1,1,1,1,1,
1,1,1,1,1,1,1,1,6),(2,2),(-1.,-0.984615384615383,-0.969230769230768,-0.953846153846152,
-0.938461538461537,-0.923076923076922,-0.907692307692306,-0.892307692307691,
-0.876923076923076,-0.86153846153846,-0.846153846153845,-0.83076923076923,
-0.815384615384614,-0.799999999999999,-0.784615384615384,-0.769230769230768,
-0.753846153846153,-0.738461538461538,-0.723076923076922,-0.707692307692307,
-0.692307692307692,-0.676923076923076,-0.661538461538461,-0.646153846153846,
-0.63076923076923,-0.615384615384615,-0.6,-0.584615384615384,-0.569230769230769,
-0.553846153846154,-0.538461538461538,-0.523076923076923,-0.507692307692308,
-0.492307692307692,-0.476923076923077,-0.461538461538462,-0.446153846153846,
-0.430769230769231,-0.415384615384615,-0.4,-0.384615384615385,-0.369230769230769,
-0.353846153846154,-0.338461538461538,-0.323076923076923,-0.307692307692308,
-0.292307692307692,-0.276923076923077,-0.261538461538462,-0.246153846153846,
-0.230769230769231,-0.215384615384615,-0.2,-0.184615384615385,-0.169230769230769,
-0.153846153846154,-0.138461538461538,-0.123076923076923,-0.107692307692308,
-0.0923076923076923,-0.0769230769230769,-0.0615384615384615,-0.0461538461538462,
-0.0307692307692308,-0.0153846153846154,0.),(-1.,1.),.UNSPECIFIED.)
GEOMETRIC_REPRESENTATION_ITEM()
RATIONAL_B_SPLINE_SURFACE(((1.,1.),(1.,1.),(1.,1.),(1.,1.),(1.,1.),(1.,
1.),(1.,1.),(1.,1.),(1.,1.),(1.,1.),(1.,1.),(1.,1.),(1.,1.),(1.,1.),(1.,
1.),(1.,1.),(1.,1.),(1.,1.),(1.,1.),(1.,1.),(1.,1.),(1.,1.),(1.,1.),(1.,
1.),(1.,1.),(1.,1.),(1.,1.),(1.,1.),(1.,1.),(1.,1.),(1.,1.),(1.,1.),(1.,
1.),(1.,1.),(1.,1.),(1.,1.),(1.,1.),(1.,1.),(1.,1.),(1.,1.),(1.,1.),(1.,
1.),(1.,1.),(1.,1.),(1.,1.),(1.,1.),(1.,1.),(1.,1.),(1.,1.),(1.,1.),(1.,
1.),(1.,1.),(1.,1.),(1.,1.),(1.,1.),(1.,1.),(1.,1.),(1.,1.),(1.,1.),(1.,
1.),(1.,1.),(1.,1.),(1.,1.),(1.,1.),(1.,1.),(1.,1.),(1.,1.),(1.,1.),(1.,
1.),(1.,1.)))
REPRESENTATION_ITEM('')
SURFACE()
);
#111=(
BOUNDED_SURFACE()
B_SPLINE_SURFACE(5,1,((#59905,#59906),(#59907,#59908),(#59909,#59910),(#59911,
#59912),(#59913,#59914),(#59915,#59916),(#59917,#59918),(#59919,#59920),
(#59921,#59922),(#59923,#59924),(#59925,#59926),(#59927,#59928),(#59929,
#59930),(#59931,#59932),(#59933,#59934),(#59935,#59936),(#59937,#59938),
(#59939,#59940),(#59941,#59942),(#59943,#59944),(#59945,#59946),(#59947,
#59948),(#59949,#59950),(#59951,#59952),(#59953,#59954),(#59955,#59956),
(#59957,#59958),(#59959,#59960),(#59961,#59962),(#59963,#59964),(#59965,
#59966),(#59967,#59968),(#59969,#59970),(#59971,#59972),(#59973,#59974),
(#59975,#59976),(#59977,#59978),(#59979,#59980),(#59981,#59982),(#59983,
#59984),(#59985,#59986),(#59987,#59988),(#59989,#59990),(#59991,#59992),
(#59993,#59994),(#59995,#59996),(#59997,#59998),(#59999,#60000),(#60001,
#60002),(#60003,#60004),(#60005,#60006),(#60007,#60008),(#60009,#60010),
(#60011,#60012),(#60013,#60014),(#60015,#60016),(#60017,#60018),(#60019,
#60020),(#60021,#60022),(#60023,#60024),(#60025,#60026),(#60027,#60028),
(#60029,#60030),(#60031,#60032),(#60033,#60034),(#60035,#60036),(#60037,
#60038),(#60039,#60040),(#60041,#60042),(#60043,#60044)),.UNSPECIFIED.,
 .F.,.F.,.F.)
B_SPLINE_SURFACE_WITH_KNOTS((6,1,1,1,1,1,1,1,1,1,1,1,1,1,1,1,1,1,1,1,1,
1,1,1,1,1,1,1,1,1,1,1,1,1,1,1,1,1,1,1,1,1,1,1,1,1,1,1,1,1,1,1,1,1,1,1,1,
1,1,1,1,1,1,1,1,6),(2,2),(-1.,-0.984615384615383,-0.969230769230768,-0.953846153846152,
-0.938461538461537,-0.923076923076922,-0.907692307692306,-0.892307692307691,
-0.876923076923076,-0.86153846153846,-0.846153846153845,-0.83076923076923,
-0.815384615384614,-0.799999999999999,-0.784615384615384,-0.769230769230768,
-0.753846153846153,-0.738461538461538,-0.723076923076922,-0.707692307692307,
-0.692307692307692,-0.676923076923076,-0.661538461538461,-0.646153846153846,
-0.63076923076923,-0.615384615384615,-0.6,-0.584615384615384,-0.569230769230769,
-0.553846153846154,-0.538461538461538,-0.523076923076923,-0.507692307692308,
-0.492307692307692,-0.476923076923077,-0.461538461538462,-0.446153846153846,
-0.430769230769231,-0.415384615384615,-0.4,-0.384615384615385,-0.369230769230769,
-0.353846153846154,-0.338461538461538,-0.323076923076923,-0.307692307692308,
-0.292307692307692,-0.276923076923077,-0.261538461538462,-0.246153846153846,
-0.230769230769231,-0.215384615384615,-0.2,-0.184615384615385,-0.169230769230769,
-0.153846153846154,-0.138461538461538,-0.123076923076923,-0.107692307692308,
-0.0923076923076923,-0.0769230769230769,-0.0615384615384615,-0.0461538461538462,
-0.0307692307692308,-0.0153846153846154,0.),(-1.,1.),.UNSPECIFIED.)
GEOMETRIC_REPRESENTATION_ITEM()
RATIONAL_B_SPLINE_SURFACE(((1.,1.),(1.,1.),(1.,1.),(1.,1.),(1.,1.),(1.,
1.),(1.,1.),(1.,1.),(1.,1.),(1.,1.),(1.,1.),(1.,1.),(1.,1.),(1.,1.),(1.,
1.),(1.,1.),(1.,1.),(1.,1.),(1.,1.),(1.,1.),(1.,1.),(1.,1.),(1.,1.),(1.,
1.),(1.,1.),(1.,1.),(1.,1.),(1.,1.),(1.,1.),(1.,1.),(1.,1.),(1.,1.),(1.,
1.),(1.,1.),(1.,1.),(1.,1.),(1.,1.),(1.,1.),(1.,1.),(1.,1.),(1.,1.),(1.,
1.),(1.,1.),(1.,1.),(1.,1.),(1.,1.),(1.,1.),(1.,1.),(1.,1.),(1.,1.),(1.,
1.),(1.,1.),(1.,1.),(1.,1.),(1.,1.),(1.,1.),(1.,1.),(1.,1.),(1.,1.),(1.,
1.),(1.,1.),(1.,1.),(1.,1.),(1.,1.),(1.,1.),(1.,1.),(1.,1.),(1.,1.),(1.,
1.),(1.,1.)))
REPRESENTATION_ITEM('')
SURFACE()
);
#112=(
BOUNDED_SURFACE()
B_SPLINE_SURFACE(5,1,((#60117,#60118),(#60119,#60120),(#60121,#60122),(#60123,
#60124),(#60125,#60126),(#60127,#60128),(#60129,#60130),(#60131,#60132),
(#60133,#60134),(#60135,#60136),(#60137,#60138),(#60139,#60140),(#60141,
#60142),(#60143,#60144),(#60145,#60146),(#60147,#60148),(#60149,#60150),
(#60151,#60152),(#60153,#60154),(#60155,#60156),(#60157,#60158),(#60159,
#60160),(#60161,#60162),(#60163,#60164),(#60165,#60166),(#60167,#60168),
(#60169,#60170),(#60171,#60172),(#60173,#60174),(#60175,#60176),(#60177,
#60178),(#60179,#60180),(#60181,#60182),(#60183,#60184),(#60185,#60186),
(#60187,#60188),(#60189,#60190),(#60191,#60192),(#60193,#60194),(#60195,
#60196),(#60197,#60198),(#60199,#60200),(#60201,#60202),(#60203,#60204),
(#60205,#60206),(#60207,#60208),(#60209,#60210),(#60211,#60212),(#60213,
#60214),(#60215,#60216),(#60217,#60218),(#60219,#60220),(#60221,#60222),
(#60223,#60224),(#60225,#60226),(#60227,#60228),(#60229,#60230),(#60231,
#60232),(#60233,#60234),(#60235,#60236),(#60237,#60238),(#60239,#60240),
(#60241,#60242),(#60243,#60244),(#60245,#60246),(#60247,#60248),(#60249,
#60250),(#60251,#60252),(#60253,#60254),(#60255,#60256)),.UNSPECIFIED.,
 .F.,.F.,.F.)
B_SPLINE_SURFACE_WITH_KNOTS((6,1,1,1,1,1,1,1,1,1,1,1,1,1,1,1,1,1,1,1,1,
1,1,1,1,1,1,1,1,1,1,1,1,1,1,1,1,1,1,1,1,1,1,1,1,1,1,1,1,1,1,1,1,1,1,1,1,
1,1,1,1,1,1,1,1,6),(2,2),(-1.,-0.984615384615383,-0.969230769230768,-0.953846153846152,
-0.938461538461537,-0.923076923076922,-0.907692307692306,-0.892307692307691,
-0.876923076923076,-0.86153846153846,-0.846153846153845,-0.83076923076923,
-0.815384615384614,-0.799999999999999,-0.784615384615384,-0.769230769230768,
-0.753846153846153,-0.738461538461538,-0.723076923076922,-0.707692307692307,
-0.692307692307692,-0.676923076923076,-0.661538461538461,-0.646153846153846,
-0.63076923076923,-0.615384615384615,-0.6,-0.584615384615384,-0.569230769230769,
-0.553846153846154,-0.538461538461538,-0.523076923076923,-0.507692307692308,
-0.492307692307692,-0.476923076923077,-0.461538461538462,-0.446153846153846,
-0.430769230769231,-0.415384615384615,-0.4,-0.384615384615385,-0.369230769230769,
-0.353846153846154,-0.338461538461538,-0.323076923076923,-0.307692307692308,
-0.292307692307692,-0.276923076923077,-0.261538461538462,-0.246153846153846,
-0.230769230769231,-0.215384615384615,-0.2,-0.184615384615385,-0.169230769230769,
-0.153846153846154,-0.138461538461538,-0.123076923076923,-0.107692307692308,
-0.0923076923076923,-0.0769230769230769,-0.0615384615384615,-0.0461538461538462,
-0.0307692307692308,-0.0153846153846154,0.),(-1.,1.),.UNSPECIFIED.)
GEOMETRIC_REPRESENTATION_ITEM()
RATIONAL_B_SPLINE_SURFACE(((1.,1.),(1.,1.),(1.,1.),(1.,1.),(1.,1.),(1.,
1.),(1.,1.),(1.,1.),(1.,1.),(1.,1.),(1.,1.),(1.,1.),(1.,1.),(1.,1.),(1.,
1.),(1.,1.),(1.,1.),(1.,1.),(1.,1.),(1.,1.),(1.,1.),(1.,1.),(1.,1.),(1.,
1.),(1.,1.),(1.,1.),(1.,1.),(1.,1.),(1.,1.),(1.,1.),(1.,1.),(1.,1.),(1.,
1.),(1.,1.),(1.,1.),(1.,1.),(1.,1.),(1.,1.),(1.,1.),(1.,1.),(1.,1.),(1.,
1.),(1.,1.),(1.,1.),(1.,1.),(1.,1.),(1.,1.),(1.,1.),(1.,1.),(1.,1.),(1.,
1.),(1.,1.),(1.,1.),(1.,1.),(1.,1.),(1.,1.),(1.,1.),(1.,1.),(1.,1.),(1.,
1.),(1.,1.),(1.,1.),(1.,1.),(1.,1.),(1.,1.),(1.,1.),(1.,1.),(1.,1.),(1.,
1.),(1.,1.)))
REPRESENTATION_ITEM('')
SURFACE()
);
#113=(
BOUNDED_SURFACE()
B_SPLINE_SURFACE(5,1,((#60347,#60348),(#60349,#60350),(#60351,#60352),(#60353,
#60354),(#60355,#60356),(#60357,#60358),(#60359,#60360),(#60361,#60362),
(#60363,#60364),(#60365,#60366),(#60367,#60368),(#60369,#60370),(#60371,
#60372),(#60373,#60374),(#60375,#60376),(#60377,#60378),(#60379,#60380),
(#60381,#60382),(#60383,#60384),(#60385,#60386),(#60387,#60388),(#60389,
#60390),(#60391,#60392),(#60393,#60394),(#60395,#60396),(#60397,#60398),
(#60399,#60400),(#60401,#60402),(#60403,#60404),(#60405,#60406),(#60407,
#60408),(#60409,#60410),(#60411,#60412),(#60413,#60414),(#60415,#60416),
(#60417,#60418),(#60419,#60420),(#60421,#60422),(#60423,#60424),(#60425,
#60426),(#60427,#60428),(#60429,#60430),(#60431,#60432),(#60433,#60434),
(#60435,#60436),(#60437,#60438),(#60439,#60440),(#60441,#60442),(#60443,
#60444),(#60445,#60446),(#60447,#60448),(#60449,#60450),(#60451,#60452),
(#60453,#60454),(#60455,#60456),(#60457,#60458),(#60459,#60460),(#60461,
#60462),(#60463,#60464),(#60465,#60466),(#60467,#60468),(#60469,#60470),
(#60471,#60472),(#60473,#60474),(#60475,#60476),(#60477,#60478),(#60479,
#60480),(#60481,#60482),(#60483,#60484),(#60485,#60486)),.UNSPECIFIED.,
 .F.,.F.,.F.)
B_SPLINE_SURFACE_WITH_KNOTS((6,1,1,1,1,1,1,1,1,1,1,1,1,1,1,1,1,1,1,1,1,
1,1,1,1,1,1,1,1,1,1,1,1,1,1,1,1,1,1,1,1,1,1,1,1,1,1,1,1,1,1,1,1,1,1,1,1,
1,1,1,1,1,1,1,1,6),(2,2),(-1.,-0.984615384615383,-0.969230769230768,-0.953846153846152,
-0.938461538461537,-0.923076923076922,-0.907692307692306,-0.892307692307691,
-0.876923076923076,-0.86153846153846,-0.846153846153845,-0.83076923076923,
-0.815384615384614,-0.799999999999999,-0.784615384615384,-0.769230769230768,
-0.753846153846153,-0.738461538461538,-0.723076923076922,-0.707692307692307,
-0.692307692307692,-0.676923076923076,-0.661538461538461,-0.646153846153846,
-0.63076923076923,-0.615384615384615,-0.6,-0.584615384615384,-0.569230769230769,
-0.553846153846154,-0.538461538461538,-0.523076923076923,-0.507692307692308,
-0.492307692307692,-0.476923076923077,-0.461538461538462,-0.446153846153846,
-0.430769230769231,-0.415384615384615,-0.4,-0.384615384615385,-0.369230769230769,
-0.353846153846154,-0.338461538461538,-0.323076923076923,-0.307692307692308,
-0.292307692307692,-0.276923076923077,-0.261538461538462,-0.246153846153846,
-0.230769230769231,-0.215384615384615,-0.2,-0.184615384615385,-0.169230769230769,
-0.153846153846154,-0.138461538461538,-0.123076923076923,-0.107692307692308,
-0.0923076923076923,-0.0769230769230769,-0.0615384615384615,-0.0461538461538462,
-0.0307692307692308,-0.0153846153846154,0.),(-1.,1.),.UNSPECIFIED.)
GEOMETRIC_REPRESENTATION_ITEM()
RATIONAL_B_SPLINE_SURFACE(((1.,1.),(1.,1.),(1.,1.),(1.,1.),(1.,1.),(1.,
1.),(1.,1.),(1.,1.),(1.,1.),(1.,1.),(1.,1.),(1.,1.),(1.,1.),(1.,1.),(1.,
1.),(1.,1.),(1.,1.),(1.,1.),(1.,1.),(1.,1.),(1.,1.),(1.,1.),(1.,1.),(1.,
1.),(1.,1.),(1.,1.),(1.,1.),(1.,1.),(1.,1.),(1.,1.),(1.,1.),(1.,1.),(1.,
1.),(1.,1.),(1.,1.),(1.,1.),(1.,1.),(1.,1.),(1.,1.),(1.,1.),(1.,1.),(1.,
1.),(1.,1.),(1.,1.),(1.,1.),(1.,1.),(1.,1.),(1.,1.),(1.,1.),(1.,1.),(1.,
1.),(1.,1.),(1.,1.),(1.,1.),(1.,1.),(1.,1.),(1.,1.),(1.,1.),(1.,1.),(1.,
1.),(1.,1.),(1.,1.),(1.,1.),(1.,1.),(1.,1.),(1.,1.),(1.,1.),(1.,1.),(1.,
1.),(1.,1.)))
REPRESENTATION_ITEM('')
SURFACE()
);
#114=(
BOUNDED_SURFACE()
B_SPLINE_SURFACE(5,1,((#60559,#60560),(#60561,#60562),(#60563,#60564),(#60565,
#60566),(#60567,#60568),(#60569,#60570),(#60571,#60572),(#60573,#60574),
(#60575,#60576),(#60577,#60578),(#60579,#60580),(#60581,#60582),(#60583,
#60584),(#60585,#60586),(#60587,#60588),(#60589,#60590),(#60591,#60592),
(#60593,#60594),(#60595,#60596),(#60597,#60598),(#60599,#60600),(#60601,
#60602),(#60603,#60604),(#60605,#60606),(#60607,#60608),(#60609,#60610),
(#60611,#60612),(#60613,#60614),(#60615,#60616),(#60617,#60618),(#60619,
#60620),(#60621,#60622),(#60623,#60624),(#60625,#60626),(#60627,#60628),
(#60629,#60630),(#60631,#60632),(#60633,#60634),(#60635,#60636),(#60637,
#60638),(#60639,#60640),(#60641,#60642),(#60643,#60644),(#60645,#60646),
(#60647,#60648),(#60649,#60650),(#60651,#60652),(#60653,#60654),(#60655,
#60656),(#60657,#60658),(#60659,#60660),(#60661,#60662),(#60663,#60664),
(#60665,#60666),(#60667,#60668),(#60669,#60670),(#60671,#60672),(#60673,
#60674),(#60675,#60676),(#60677,#60678),(#60679,#60680),(#60681,#60682),
(#60683,#60684),(#60685,#60686),(#60687,#60688),(#60689,#60690),(#60691,
#60692),(#60693,#60694),(#60695,#60696),(#60697,#60698)),.UNSPECIFIED.,
 .F.,.F.,.F.)
B_SPLINE_SURFACE_WITH_KNOTS((6,1,1,1,1,1,1,1,1,1,1,1,1,1,1,1,1,1,1,1,1,
1,1,1,1,1,1,1,1,1,1,1,1,1,1,1,1,1,1,1,1,1,1,1,1,1,1,1,1,1,1,1,1,1,1,1,1,
1,1,1,1,1,1,1,1,6),(2,2),(-1.,-0.984615384615383,-0.969230769230768,-0.953846153846152,
-0.938461538461537,-0.923076923076922,-0.907692307692306,-0.892307692307691,
-0.876923076923076,-0.86153846153846,-0.846153846153845,-0.83076923076923,
-0.815384615384614,-0.799999999999999,-0.784615384615384,-0.769230769230768,
-0.753846153846153,-0.738461538461538,-0.723076923076922,-0.707692307692307,
-0.692307692307692,-0.676923076923076,-0.661538461538461,-0.646153846153846,
-0.63076923076923,-0.615384615384615,-0.6,-0.584615384615384,-0.569230769230769,
-0.553846153846154,-0.538461538461538,-0.523076923076923,-0.507692307692308,
-0.492307692307692,-0.476923076923077,-0.461538461538462,-0.446153846153846,
-0.430769230769231,-0.415384615384615,-0.4,-0.384615384615385,-0.369230769230769,
-0.353846153846154,-0.338461538461538,-0.323076923076923,-0.307692307692308,
-0.292307692307692,-0.276923076923077,-0.261538461538462,-0.246153846153846,
-0.230769230769231,-0.215384615384615,-0.2,-0.184615384615385,-0.169230769230769,
-0.153846153846154,-0.138461538461538,-0.123076923076923,-0.107692307692308,
-0.0923076923076923,-0.0769230769230769,-0.0615384615384615,-0.0461538461538462,
-0.0307692307692308,-0.0153846153846154,0.),(-1.,1.),.UNSPECIFIED.)
GEOMETRIC_REPRESENTATION_ITEM()
RATIONAL_B_SPLINE_SURFACE(((1.,1.),(1.,1.),(1.,1.),(1.,1.),(1.,1.),(1.,
1.),(1.,1.),(1.,1.),(1.,1.),(1.,1.),(1.,1.),(1.,1.),(1.,1.),(1.,1.),(1.,
1.),(1.,1.),(1.,1.),(1.,1.),(1.,1.),(1.,1.),(1.,1.),(1.,1.),(1.,1.),(1.,
1.),(1.,1.),(1.,1.),(1.,1.),(1.,1.),(1.,1.),(1.,1.),(1.,1.),(1.,1.),(1.,
1.),(1.,1.),(1.,1.),(1.,1.),(1.,1.),(1.,1.),(1.,1.),(1.,1.),(1.,1.),(1.,
1.),(1.,1.),(1.,1.),(1.,1.),(1.,1.),(1.,1.),(1.,1.),(1.,1.),(1.,1.),(1.,
1.),(1.,1.),(1.,1.),(1.,1.),(1.,1.),(1.,1.),(1.,1.),(1.,1.),(1.,1.),(1.,
1.),(1.,1.),(1.,1.),(1.,1.),(1.,1.),(1.,1.),(1.,1.),(1.,1.),(1.,1.),(1.,
1.),(1.,1.)))
REPRESENTATION_ITEM('')
SURFACE()
);
#115=(
BOUNDED_SURFACE()
B_SPLINE_SURFACE(5,1,((#60789,#60790),(#60791,#60792),(#60793,#60794),(#60795,
#60796),(#60797,#60798),(#60799,#60800),(#60801,#60802),(#60803,#60804),
(#60805,#60806),(#60807,#60808),(#60809,#60810),(#60811,#60812),(#60813,
#60814),(#60815,#60816),(#60817,#60818),(#60819,#60820),(#60821,#60822),
(#60823,#60824),(#60825,#60826),(#60827,#60828),(#60829,#60830),(#60831,
#60832),(#60833,#60834),(#60835,#60836),(#60837,#60838),(#60839,#60840),
(#60841,#60842),(#60843,#60844),(#60845,#60846),(#60847,#60848),(#60849,
#60850),(#60851,#60852),(#60853,#60854),(#60855,#60856),(#60857,#60858),
(#60859,#60860),(#60861,#60862),(#60863,#60864),(#60865,#60866),(#60867,
#60868),(#60869,#60870),(#60871,#60872),(#60873,#60874),(#60875,#60876),
(#60877,#60878),(#60879,#60880),(#60881,#60882),(#60883,#60884),(#60885,
#60886),(#60887,#60888),(#60889,#60890),(#60891,#60892),(#60893,#60894),
(#60895,#60896),(#60897,#60898),(#60899,#60900),(#60901,#60902),(#60903,
#60904),(#60905,#60906),(#60907,#60908),(#60909,#60910),(#60911,#60912),
(#60913,#60914),(#60915,#60916),(#60917,#60918),(#60919,#60920),(#60921,
#60922),(#60923,#60924),(#60925,#60926),(#60927,#60928)),.UNSPECIFIED.,
 .F.,.F.,.F.)
B_SPLINE_SURFACE_WITH_KNOTS((6,1,1,1,1,1,1,1,1,1,1,1,1,1,1,1,1,1,1,1,1,
1,1,1,1,1,1,1,1,1,1,1,1,1,1,1,1,1,1,1,1,1,1,1,1,1,1,1,1,1,1,1,1,1,1,1,1,
1,1,1,1,1,1,1,1,6),(2,2),(-1.,-0.984615384615383,-0.969230769230768,-0.953846153846152,
-0.938461538461537,-0.923076923076922,-0.907692307692306,-0.892307692307691,
-0.876923076923076,-0.86153846153846,-0.846153846153845,-0.83076923076923,
-0.815384615384614,-0.799999999999999,-0.784615384615384,-0.769230769230768,
-0.753846153846153,-0.738461538461538,-0.723076923076922,-0.707692307692307,
-0.692307692307692,-0.676923076923076,-0.661538461538461,-0.646153846153846,
-0.63076923076923,-0.615384615384615,-0.6,-0.584615384615384,-0.569230769230769,
-0.553846153846154,-0.538461538461538,-0.523076923076923,-0.507692307692308,
-0.492307692307692,-0.476923076923077,-0.461538461538462,-0.446153846153846,
-0.430769230769231,-0.415384615384615,-0.4,-0.384615384615385,-0.369230769230769,
-0.353846153846154,-0.338461538461538,-0.323076923076923,-0.307692307692308,
-0.292307692307692,-0.276923076923077,-0.261538461538462,-0.246153846153846,
-0.230769230769231,-0.215384615384615,-0.2,-0.184615384615385,-0.169230769230769,
-0.153846153846154,-0.138461538461538,-0.123076923076923,-0.107692307692308,
-0.0923076923076923,-0.0769230769230769,-0.0615384615384615,-0.0461538461538462,
-0.0307692307692308,-0.0153846153846154,0.),(-1.,1.),.UNSPECIFIED.)
GEOMETRIC_REPRESENTATION_ITEM()
RATIONAL_B_SPLINE_SURFACE(((1.,1.),(1.,1.),(1.,1.),(1.,1.),(1.,1.),(1.,
1.),(1.,1.),(1.,1.),(1.,1.),(1.,1.),(1.,1.),(1.,1.),(1.,1.),(1.,1.),(1.,
1.),(1.,1.),(1.,1.),(1.,1.),(1.,1.),(1.,1.),(1.,1.),(1.,1.),(1.,1.),(1.,
1.),(1.,1.),(1.,1.),(1.,1.),(1.,1.),(1.,1.),(1.,1.),(1.,1.),(1.,1.),(1.,
1.),(1.,1.),(1.,1.),(1.,1.),(1.,1.),(1.,1.),(1.,1.),(1.,1.),(1.,1.),(1.,
1.),(1.,1.),(1.,1.),(1.,1.),(1.,1.),(1.,1.),(1.,1.),(1.,1.),(1.,1.),(1.,
1.),(1.,1.),(1.,1.),(1.,1.),(1.,1.),(1.,1.),(1.,1.),(1.,1.),(1.,1.),(1.,
1.),(1.,1.),(1.,1.),(1.,1.),(1.,1.),(1.,1.),(1.,1.),(1.,1.),(1.,1.),(1.,
1.),(1.,1.)))
REPRESENTATION_ITEM('')
SURFACE()
);
#116=(
BOUNDED_SURFACE()
B_SPLINE_SURFACE(5,1,((#61001,#61002),(#61003,#61004),(#61005,#61006),(#61007,
#61008),(#61009,#61010),(#61011,#61012),(#61013,#61014),(#61015,#61016),
(#61017,#61018),(#61019,#61020),(#61021,#61022),(#61023,#61024),(#61025,
#61026),(#61027,#61028),(#61029,#61030),(#61031,#61032),(#61033,#61034),
(#61035,#61036),(#61037,#61038),(#61039,#61040),(#61041,#61042),(#61043,
#61044),(#61045,#61046),(#61047,#61048),(#61049,#61050),(#61051,#61052),
(#61053,#61054),(#61055,#61056),(#61057,#61058),(#61059,#61060),(#61061,
#61062),(#61063,#61064),(#61065,#61066),(#61067,#61068),(#61069,#61070),
(#61071,#61072),(#61073,#61074),(#61075,#61076),(#61077,#61078),(#61079,
#61080),(#61081,#61082),(#61083,#61084),(#61085,#61086),(#61087,#61088),
(#61089,#61090),(#61091,#61092),(#61093,#61094),(#61095,#61096),(#61097,
#61098),(#61099,#61100),(#61101,#61102),(#61103,#61104),(#61105,#61106),
(#61107,#61108),(#61109,#61110),(#61111,#61112),(#61113,#61114),(#61115,
#61116),(#61117,#61118),(#61119,#61120),(#61121,#61122),(#61123,#61124),
(#61125,#61126),(#61127,#61128),(#61129,#61130),(#61131,#61132),(#61133,
#61134),(#61135,#61136),(#61137,#61138),(#61139,#61140)),.UNSPECIFIED.,
 .F.,.F.,.F.)
B_SPLINE_SURFACE_WITH_KNOTS((6,1,1,1,1,1,1,1,1,1,1,1,1,1,1,1,1,1,1,1,1,
1,1,1,1,1,1,1,1,1,1,1,1,1,1,1,1,1,1,1,1,1,1,1,1,1,1,1,1,1,1,1,1,1,1,1,1,
1,1,1,1,1,1,1,1,6),(2,2),(-1.,-0.984615384615383,-0.969230769230768,-0.953846153846152,
-0.938461538461537,-0.923076923076922,-0.907692307692306,-0.892307692307691,
-0.876923076923076,-0.86153846153846,-0.846153846153845,-0.83076923076923,
-0.815384615384614,-0.799999999999999,-0.784615384615384,-0.769230769230768,
-0.753846153846153,-0.738461538461538,-0.723076923076922,-0.707692307692307,
-0.692307692307692,-0.676923076923076,-0.661538461538461,-0.646153846153846,
-0.63076923076923,-0.615384615384615,-0.6,-0.584615384615384,-0.569230769230769,
-0.553846153846154,-0.538461538461538,-0.523076923076923,-0.507692307692308,
-0.492307692307692,-0.476923076923077,-0.461538461538462,-0.446153846153846,
-0.430769230769231,-0.415384615384615,-0.4,-0.384615384615385,-0.369230769230769,
-0.353846153846154,-0.338461538461538,-0.323076923076923,-0.307692307692308,
-0.292307692307692,-0.276923076923077,-0.261538461538462,-0.246153846153846,
-0.230769230769231,-0.215384615384615,-0.2,-0.184615384615385,-0.169230769230769,
-0.153846153846154,-0.138461538461538,-0.123076923076923,-0.107692307692308,
-0.0923076923076923,-0.0769230769230769,-0.0615384615384615,-0.0461538461538462,
-0.0307692307692308,-0.0153846153846154,0.),(-1.,1.),.UNSPECIFIED.)
GEOMETRIC_REPRESENTATION_ITEM()
RATIONAL_B_SPLINE_SURFACE(((1.,1.),(1.,1.),(1.,1.),(1.,1.),(1.,1.),(1.,
1.),(1.,1.),(1.,1.),(1.,1.),(1.,1.),(1.,1.),(1.,1.),(1.,1.),(1.,1.),(1.,
1.),(1.,1.),(1.,1.),(1.,1.),(1.,1.),(1.,1.),(1.,1.),(1.,1.),(1.,1.),(1.,
1.),(1.,1.),(1.,1.),(1.,1.),(1.,1.),(1.,1.),(1.,1.),(1.,1.),(1.,1.),(1.,
1.),(1.,1.),(1.,1.),(1.,1.),(1.,1.),(1.,1.),(1.,1.),(1.,1.),(1.,1.),(1.,
1.),(1.,1.),(1.,1.),(1.,1.),(1.,1.),(1.,1.),(1.,1.),(1.,1.),(1.,1.),(1.,
1.),(1.,1.),(1.,1.),(1.,1.),(1.,1.),(1.,1.),(1.,1.),(1.,1.),(1.,1.),(1.,
1.),(1.,1.),(1.,1.),(1.,1.),(1.,1.),(1.,1.),(1.,1.),(1.,1.),(1.,1.),(1.,
1.),(1.,1.)))
REPRESENTATION_ITEM('')
SURFACE()
);
#117=(
BOUNDED_SURFACE()
B_SPLINE_SURFACE(5,1,((#61231,#61232),(#61233,#61234),(#61235,#61236),(#61237,
#61238),(#61239,#61240),(#61241,#61242),(#61243,#61244),(#61245,#61246),
(#61247,#61248),(#61249,#61250),(#61251,#61252),(#61253,#61254),(#61255,
#61256),(#61257,#61258),(#61259,#61260),(#61261,#61262),(#61263,#61264),
(#61265,#61266),(#61267,#61268),(#61269,#61270),(#61271,#61272),(#61273,
#61274),(#61275,#61276),(#61277,#61278),(#61279,#61280),(#61281,#61282),
(#61283,#61284),(#61285,#61286),(#61287,#61288),(#61289,#61290),(#61291,
#61292),(#61293,#61294),(#61295,#61296),(#61297,#61298),(#61299,#61300),
(#61301,#61302),(#61303,#61304),(#61305,#61306),(#61307,#61308),(#61309,
#61310),(#61311,#61312),(#61313,#61314),(#61315,#61316),(#61317,#61318),
(#61319,#61320),(#61321,#61322),(#61323,#61324),(#61325,#61326),(#61327,
#61328),(#61329,#61330),(#61331,#61332),(#61333,#61334),(#61335,#61336),
(#61337,#61338),(#61339,#61340),(#61341,#61342),(#61343,#61344),(#61345,
#61346),(#61347,#61348),(#61349,#61350),(#61351,#61352),(#61353,#61354),
(#61355,#61356),(#61357,#61358),(#61359,#61360),(#61361,#61362),(#61363,
#61364),(#61365,#61366),(#61367,#61368),(#61369,#61370)),.UNSPECIFIED.,
 .F.,.F.,.F.)
B_SPLINE_SURFACE_WITH_KNOTS((6,1,1,1,1,1,1,1,1,1,1,1,1,1,1,1,1,1,1,1,1,
1,1,1,1,1,1,1,1,1,1,1,1,1,1,1,1,1,1,1,1,1,1,1,1,1,1,1,1,1,1,1,1,1,1,1,1,
1,1,1,1,1,1,1,1,6),(2,2),(-1.,-0.984615384615383,-0.969230769230768,-0.953846153846152,
-0.938461538461537,-0.923076923076922,-0.907692307692306,-0.892307692307691,
-0.876923076923076,-0.86153846153846,-0.846153846153845,-0.83076923076923,
-0.815384615384614,-0.799999999999999,-0.784615384615384,-0.769230769230768,
-0.753846153846153,-0.738461538461538,-0.723076923076922,-0.707692307692307,
-0.692307692307692,-0.676923076923076,-0.661538461538461,-0.646153846153846,
-0.63076923076923,-0.615384615384615,-0.6,-0.584615384615384,-0.569230769230769,
-0.553846153846154,-0.538461538461538,-0.523076923076923,-0.507692307692308,
-0.492307692307692,-0.476923076923077,-0.461538461538462,-0.446153846153846,
-0.430769230769231,-0.415384615384615,-0.4,-0.384615384615385,-0.369230769230769,
-0.353846153846154,-0.338461538461538,-0.323076923076923,-0.307692307692308,
-0.292307692307692,-0.276923076923077,-0.261538461538462,-0.246153846153846,
-0.230769230769231,-0.215384615384615,-0.2,-0.184615384615385,-0.169230769230769,
-0.153846153846154,-0.138461538461538,-0.123076923076923,-0.107692307692308,
-0.0923076923076923,-0.0769230769230769,-0.0615384615384615,-0.0461538461538462,
-0.0307692307692308,-0.0153846153846154,0.),(-1.,1.),.UNSPECIFIED.)
GEOMETRIC_REPRESENTATION_ITEM()
RATIONAL_B_SPLINE_SURFACE(((1.,1.),(1.,1.),(1.,1.),(1.,1.),(1.,1.),(1.,
1.),(1.,1.),(1.,1.),(1.,1.),(1.,1.),(1.,1.),(1.,1.),(1.,1.),(1.,1.),(1.,
1.),(1.,1.),(1.,1.),(1.,1.),(1.,1.),(1.,1.),(1.,1.),(1.,1.),(1.,1.),(1.,
1.),(1.,1.),(1.,1.),(1.,1.),(1.,1.),(1.,1.),(1.,1.),(1.,1.),(1.,1.),(1.,
1.),(1.,1.),(1.,1.),(1.,1.),(1.,1.),(1.,1.),(1.,1.),(1.,1.),(1.,1.),(1.,
1.),(1.,1.),(1.,1.),(1.,1.),(1.,1.),(1.,1.),(1.,1.),(1.,1.),(1.,1.),(1.,
1.),(1.,1.),(1.,1.),(1.,1.),(1.,1.),(1.,1.),(1.,1.),(1.,1.),(1.,1.),(1.,
1.),(1.,1.),(1.,1.),(1.,1.),(1.,1.),(1.,1.),(1.,1.),(1.,1.),(1.,1.),(1.,
1.),(1.,1.)))
REPRESENTATION_ITEM('')
SURFACE()
);
#118=(
BOUNDED_SURFACE()
B_SPLINE_SURFACE(5,1,((#61443,#61444),(#61445,#61446),(#61447,#61448),(#61449,
#61450),(#61451,#61452),(#61453,#61454),(#61455,#61456),(#61457,#61458),
(#61459,#61460),(#61461,#61462),(#61463,#61464),(#61465,#61466),(#61467,
#61468),(#61469,#61470),(#61471,#61472),(#61473,#61474),(#61475,#61476),
(#61477,#61478),(#61479,#61480),(#61481,#61482),(#61483,#61484),(#61485,
#61486),(#61487,#61488),(#61489,#61490),(#61491,#61492),(#61493,#61494),
(#61495,#61496),(#61497,#61498),(#61499,#61500),(#61501,#61502),(#61503,
#61504),(#61505,#61506),(#61507,#61508),(#61509,#61510),(#61511,#61512),
(#61513,#61514),(#61515,#61516),(#61517,#61518),(#61519,#61520),(#61521,
#61522),(#61523,#61524),(#61525,#61526),(#61527,#61528),(#61529,#61530),
(#61531,#61532),(#61533,#61534),(#61535,#61536),(#61537,#61538),(#61539,
#61540),(#61541,#61542),(#61543,#61544),(#61545,#61546),(#61547,#61548),
(#61549,#61550),(#61551,#61552),(#61553,#61554),(#61555,#61556),(#61557,
#61558),(#61559,#61560),(#61561,#61562),(#61563,#61564),(#61565,#61566),
(#61567,#61568),(#61569,#61570),(#61571,#61572),(#61573,#61574),(#61575,
#61576),(#61577,#61578),(#61579,#61580),(#61581,#61582)),.UNSPECIFIED.,
 .F.,.F.,.F.)
B_SPLINE_SURFACE_WITH_KNOTS((6,1,1,1,1,1,1,1,1,1,1,1,1,1,1,1,1,1,1,1,1,
1,1,1,1,1,1,1,1,1,1,1,1,1,1,1,1,1,1,1,1,1,1,1,1,1,1,1,1,1,1,1,1,1,1,1,1,
1,1,1,1,1,1,1,1,6),(2,2),(-1.,-0.984615384615383,-0.969230769230768,-0.953846153846152,
-0.938461538461537,-0.923076923076922,-0.907692307692306,-0.892307692307691,
-0.876923076923076,-0.86153846153846,-0.846153846153845,-0.83076923076923,
-0.815384615384614,-0.799999999999999,-0.784615384615384,-0.769230769230768,
-0.753846153846153,-0.738461538461538,-0.723076923076922,-0.707692307692307,
-0.692307692307692,-0.676923076923076,-0.661538461538461,-0.646153846153846,
-0.63076923076923,-0.615384615384615,-0.6,-0.584615384615384,-0.569230769230769,
-0.553846153846154,-0.538461538461538,-0.523076923076923,-0.507692307692308,
-0.492307692307692,-0.476923076923077,-0.461538461538462,-0.446153846153846,
-0.430769230769231,-0.415384615384615,-0.4,-0.384615384615385,-0.369230769230769,
-0.353846153846154,-0.338461538461538,-0.323076923076923,-0.307692307692308,
-0.292307692307692,-0.276923076923077,-0.261538461538462,-0.246153846153846,
-0.230769230769231,-0.215384615384615,-0.2,-0.184615384615385,-0.169230769230769,
-0.153846153846154,-0.138461538461538,-0.123076923076923,-0.107692307692308,
-0.0923076923076923,-0.0769230769230769,-0.0615384615384615,-0.0461538461538462,
-0.0307692307692308,-0.0153846153846154,0.),(-1.,1.),.UNSPECIFIED.)
GEOMETRIC_REPRESENTATION_ITEM()
RATIONAL_B_SPLINE_SURFACE(((1.,1.),(1.,1.),(1.,1.),(1.,1.),(1.,1.),(1.,
1.),(1.,1.),(1.,1.),(1.,1.),(1.,1.),(1.,1.),(1.,1.),(1.,1.),(1.,1.),(1.,
1.),(1.,1.),(1.,1.),(1.,1.),(1.,1.),(1.,1.),(1.,1.),(1.,1.),(1.,1.),(1.,
1.),(1.,1.),(1.,1.),(1.,1.),(1.,1.),(1.,1.),(1.,1.),(1.,1.),(1.,1.),(1.,
1.),(1.,1.),(1.,1.),(1.,1.),(1.,1.),(1.,1.),(1.,1.),(1.,1.),(1.,1.),(1.,
1.),(1.,1.),(1.,1.),(1.,1.),(1.,1.),(1.,1.),(1.,1.),(1.,1.),(1.,1.),(1.,
1.),(1.,1.),(1.,1.),(1.,1.),(1.,1.),(1.,1.),(1.,1.),(1.,1.),(1.,1.),(1.,
1.),(1.,1.),(1.,1.),(1.,1.),(1.,1.),(1.,1.),(1.,1.),(1.,1.),(1.,1.),(1.,
1.),(1.,1.)))
REPRESENTATION_ITEM('')
SURFACE()
);
#119=(
BOUNDED_SURFACE()
B_SPLINE_SURFACE(5,1,((#61673,#61674),(#61675,#61676),(#61677,#61678),(#61679,
#61680),(#61681,#61682),(#61683,#61684),(#61685,#61686),(#61687,#61688),
(#61689,#61690),(#61691,#61692),(#61693,#61694),(#61695,#61696),(#61697,
#61698),(#61699,#61700),(#61701,#61702),(#61703,#61704),(#61705,#61706),
(#61707,#61708),(#61709,#61710),(#61711,#61712),(#61713,#61714),(#61715,
#61716),(#61717,#61718),(#61719,#61720),(#61721,#61722),(#61723,#61724),
(#61725,#61726),(#61727,#61728),(#61729,#61730),(#61731,#61732),(#61733,
#61734),(#61735,#61736),(#61737,#61738),(#61739,#61740),(#61741,#61742),
(#61743,#61744),(#61745,#61746),(#61747,#61748),(#61749,#61750),(#61751,
#61752),(#61753,#61754),(#61755,#61756),(#61757,#61758),(#61759,#61760),
(#61761,#61762),(#61763,#61764),(#61765,#61766),(#61767,#61768),(#61769,
#61770),(#61771,#61772),(#61773,#61774),(#61775,#61776),(#61777,#61778),
(#61779,#61780),(#61781,#61782),(#61783,#61784),(#61785,#61786),(#61787,
#61788),(#61789,#61790),(#61791,#61792),(#61793,#61794),(#61795,#61796),
(#61797,#61798),(#61799,#61800),(#61801,#61802),(#61803,#61804),(#61805,
#61806),(#61807,#61808),(#61809,#61810),(#61811,#61812)),.UNSPECIFIED.,
 .F.,.F.,.F.)
B_SPLINE_SURFACE_WITH_KNOTS((6,1,1,1,1,1,1,1,1,1,1,1,1,1,1,1,1,1,1,1,1,
1,1,1,1,1,1,1,1,1,1,1,1,1,1,1,1,1,1,1,1,1,1,1,1,1,1,1,1,1,1,1,1,1,1,1,1,
1,1,1,1,1,1,1,1,6),(2,2),(-1.,-0.984615384615383,-0.969230769230768,-0.953846153846152,
-0.938461538461537,-0.923076923076922,-0.907692307692306,-0.892307692307691,
-0.876923076923076,-0.86153846153846,-0.846153846153845,-0.83076923076923,
-0.815384615384614,-0.799999999999999,-0.784615384615384,-0.769230769230768,
-0.753846153846153,-0.738461538461538,-0.723076923076922,-0.707692307692307,
-0.692307692307692,-0.676923076923076,-0.661538461538461,-0.646153846153846,
-0.63076923076923,-0.615384615384615,-0.6,-0.584615384615384,-0.569230769230769,
-0.553846153846154,-0.538461538461538,-0.523076923076923,-0.507692307692308,
-0.492307692307692,-0.476923076923077,-0.461538461538462,-0.446153846153846,
-0.430769230769231,-0.415384615384615,-0.4,-0.384615384615385,-0.369230769230769,
-0.353846153846154,-0.338461538461538,-0.323076923076923,-0.307692307692308,
-0.292307692307692,-0.276923076923077,-0.261538461538462,-0.246153846153846,
-0.230769230769231,-0.215384615384615,-0.2,-0.184615384615385,-0.169230769230769,
-0.153846153846154,-0.138461538461538,-0.123076923076923,-0.107692307692308,
-0.0923076923076923,-0.0769230769230769,-0.0615384615384615,-0.0461538461538462,
-0.0307692307692308,-0.0153846153846154,0.),(-1.,1.),.UNSPECIFIED.)
GEOMETRIC_REPRESENTATION_ITEM()
RATIONAL_B_SPLINE_SURFACE(((1.,1.),(1.,1.),(1.,1.),(1.,1.),(1.,1.),(1.,
1.),(1.,1.),(1.,1.),(1.,1.),(1.,1.),(1.,1.),(1.,1.),(1.,1.),(1.,1.),(1.,
1.),(1.,1.),(1.,1.),(1.,1.),(1.,1.),(1.,1.),(1.,1.),(1.,1.),(1.,1.),(1.,
1.),(1.,1.),(1.,1.),(1.,1.),(1.,1.),(1.,1.),(1.,1.),(1.,1.),(1.,1.),(1.,
1.),(1.,1.),(1.,1.),(1.,1.),(1.,1.),(1.,1.),(1.,1.),(1.,1.),(1.,1.),(1.,
1.),(1.,1.),(1.,1.),(1.,1.),(1.,1.),(1.,1.),(1.,1.),(1.,1.),(1.,1.),(1.,
1.),(1.,1.),(1.,1.),(1.,1.),(1.,1.),(1.,1.),(1.,1.),(1.,1.),(1.,1.),(1.,
1.),(1.,1.),(1.,1.),(1.,1.),(1.,1.),(1.,1.),(1.,1.),(1.,1.),(1.,1.),(1.,
1.),(1.,1.)))
REPRESENTATION_ITEM('')
SURFACE()
);
#120=(
BOUNDED_SURFACE()
B_SPLINE_SURFACE(5,1,((#61885,#61886),(#61887,#61888),(#61889,#61890),(#61891,
#61892),(#61893,#61894),(#61895,#61896),(#61897,#61898),(#61899,#61900),
(#61901,#61902),(#61903,#61904),(#61905,#61906),(#61907,#61908),(#61909,
#61910),(#61911,#61912),(#61913,#61914),(#61915,#61916),(#61917,#61918),
(#61919,#61920),(#61921,#61922),(#61923,#61924),(#61925,#61926),(#61927,
#61928),(#61929,#61930),(#61931,#61932),(#61933,#61934),(#61935,#61936),
(#61937,#61938),(#61939,#61940),(#61941,#61942),(#61943,#61944),(#61945,
#61946),(#61947,#61948),(#61949,#61950),(#61951,#61952),(#61953,#61954),
(#61955,#61956),(#61957,#61958),(#61959,#61960),(#61961,#61962),(#61963,
#61964),(#61965,#61966),(#61967,#61968),(#61969,#61970),(#61971,#61972),
(#61973,#61974),(#61975,#61976),(#61977,#61978),(#61979,#61980),(#61981,
#61982),(#61983,#61984),(#61985,#61986),(#61987,#61988),(#61989,#61990),
(#61991,#61992),(#61993,#61994),(#61995,#61996),(#61997,#61998),(#61999,
#62000),(#62001,#62002),(#62003,#62004),(#62005,#62006),(#62007,#62008),
(#62009,#62010),(#62011,#62012),(#62013,#62014),(#62015,#62016),(#62017,
#62018),(#62019,#62020),(#62021,#62022),(#62023,#62024)),.UNSPECIFIED.,
 .F.,.F.,.F.)
B_SPLINE_SURFACE_WITH_KNOTS((6,1,1,1,1,1,1,1,1,1,1,1,1,1,1,1,1,1,1,1,1,
1,1,1,1,1,1,1,1,1,1,1,1,1,1,1,1,1,1,1,1,1,1,1,1,1,1,1,1,1,1,1,1,1,1,1,1,
1,1,1,1,1,1,1,1,6),(2,2),(-1.,-0.984615384615383,-0.969230769230768,-0.953846153846152,
-0.938461538461537,-0.923076923076922,-0.907692307692306,-0.892307692307691,
-0.876923076923076,-0.86153846153846,-0.846153846153845,-0.83076923076923,
-0.815384615384614,-0.799999999999999,-0.784615384615384,-0.769230769230768,
-0.753846153846153,-0.738461538461538,-0.723076923076922,-0.707692307692307,
-0.692307692307692,-0.676923076923076,-0.661538461538461,-0.646153846153846,
-0.63076923076923,-0.615384615384615,-0.6,-0.584615384615384,-0.569230769230769,
-0.553846153846154,-0.538461538461538,-0.523076923076923,-0.507692307692308,
-0.492307692307692,-0.476923076923077,-0.461538461538462,-0.446153846153846,
-0.430769230769231,-0.415384615384615,-0.4,-0.384615384615385,-0.369230769230769,
-0.353846153846154,-0.338461538461538,-0.323076923076923,-0.307692307692308,
-0.292307692307692,-0.276923076923077,-0.261538461538462,-0.246153846153846,
-0.230769230769231,-0.215384615384615,-0.2,-0.184615384615385,-0.169230769230769,
-0.153846153846154,-0.138461538461538,-0.123076923076923,-0.107692307692308,
-0.0923076923076923,-0.0769230769230769,-0.0615384615384615,-0.0461538461538462,
-0.0307692307692308,-0.0153846153846154,0.),(-1.,1.),.UNSPECIFIED.)
GEOMETRIC_REPRESENTATION_ITEM()
RATIONAL_B_SPLINE_SURFACE(((1.,1.),(1.,1.),(1.,1.),(1.,1.),(1.,1.),(1.,
1.),(1.,1.),(1.,1.),(1.,1.),(1.,1.),(1.,1.),(1.,1.),(1.,1.),(1.,1.),(1.,
1.),(1.,1.),(1.,1.),(1.,1.),(1.,1.),(1.,1.),(1.,1.),(1.,1.),(1.,1.),(1.,
1.),(1.,1.),(1.,1.),(1.,1.),(1.,1.),(1.,1.),(1.,1.),(1.,1.),(1.,1.),(1.,
1.),(1.,1.),(1.,1.),(1.,1.),(1.,1.),(1.,1.),(1.,1.),(1.,1.),(1.,1.),(1.,
1.),(1.,1.),(1.,1.),(1.,1.),(1.,1.),(1.,1.),(1.,1.),(1.,1.),(1.,1.),(1.,
1.),(1.,1.),(1.,1.),(1.,1.),(1.,1.),(1.,1.),(1.,1.),(1.,1.),(1.,1.),(1.,
1.),(1.,1.),(1.,1.),(1.,1.),(1.,1.),(1.,1.),(1.,1.),(1.,1.),(1.,1.),(1.,
1.),(1.,1.)))
REPRESENTATION_ITEM('')
SURFACE()
);
#121=(
BOUNDED_SURFACE()
B_SPLINE_SURFACE(5,1,((#62115,#62116),(#62117,#62118),(#62119,#62120),(#62121,
#62122),(#62123,#62124),(#62125,#62126),(#62127,#62128),(#62129,#62130),
(#62131,#62132),(#62133,#62134),(#62135,#62136),(#62137,#62138),(#62139,
#62140),(#62141,#62142),(#62143,#62144),(#62145,#62146),(#62147,#62148),
(#62149,#62150),(#62151,#62152),(#62153,#62154),(#62155,#62156),(#62157,
#62158),(#62159,#62160),(#62161,#62162),(#62163,#62164),(#62165,#62166),
(#62167,#62168),(#62169,#62170),(#62171,#62172),(#62173,#62174),(#62175,
#62176),(#62177,#62178),(#62179,#62180),(#62181,#62182),(#62183,#62184),
(#62185,#62186),(#62187,#62188),(#62189,#62190),(#62191,#62192),(#62193,
#62194),(#62195,#62196),(#62197,#62198),(#62199,#62200),(#62201,#62202),
(#62203,#62204),(#62205,#62206),(#62207,#62208),(#62209,#62210),(#62211,
#62212),(#62213,#62214),(#62215,#62216),(#62217,#62218),(#62219,#62220),
(#62221,#62222),(#62223,#62224),(#62225,#62226),(#62227,#62228),(#62229,
#62230),(#62231,#62232),(#62233,#62234),(#62235,#62236),(#62237,#62238),
(#62239,#62240),(#62241,#62242),(#62243,#62244),(#62245,#62246),(#62247,
#62248),(#62249,#62250),(#62251,#62252),(#62253,#62254)),.UNSPECIFIED.,
 .F.,.F.,.F.)
B_SPLINE_SURFACE_WITH_KNOTS((6,1,1,1,1,1,1,1,1,1,1,1,1,1,1,1,1,1,1,1,1,
1,1,1,1,1,1,1,1,1,1,1,1,1,1,1,1,1,1,1,1,1,1,1,1,1,1,1,1,1,1,1,1,1,1,1,1,
1,1,1,1,1,1,1,1,6),(2,2),(-1.,-0.984615384615383,-0.969230769230768,-0.953846153846152,
-0.938461538461537,-0.923076923076922,-0.907692307692306,-0.892307692307691,
-0.876923076923076,-0.86153846153846,-0.846153846153845,-0.83076923076923,
-0.815384615384614,-0.799999999999999,-0.784615384615384,-0.769230769230768,
-0.753846153846153,-0.738461538461538,-0.723076923076922,-0.707692307692307,
-0.692307692307692,-0.676923076923076,-0.661538461538461,-0.646153846153846,
-0.63076923076923,-0.615384615384615,-0.6,-0.584615384615384,-0.569230769230769,
-0.553846153846154,-0.538461538461538,-0.523076923076923,-0.507692307692308,
-0.492307692307692,-0.476923076923077,-0.461538461538462,-0.446153846153846,
-0.430769230769231,-0.415384615384615,-0.4,-0.384615384615385,-0.369230769230769,
-0.353846153846154,-0.338461538461538,-0.323076923076923,-0.307692307692308,
-0.292307692307692,-0.276923076923077,-0.261538461538462,-0.246153846153846,
-0.230769230769231,-0.215384615384615,-0.2,-0.184615384615385,-0.169230769230769,
-0.153846153846154,-0.138461538461538,-0.123076923076923,-0.107692307692308,
-0.0923076923076923,-0.0769230769230769,-0.0615384615384615,-0.0461538461538462,
-0.0307692307692308,-0.0153846153846154,0.),(-1.,1.),.UNSPECIFIED.)
GEOMETRIC_REPRESENTATION_ITEM()
RATIONAL_B_SPLINE_SURFACE(((1.,1.),(1.,1.),(1.,1.),(1.,1.),(1.,1.),(1.,
1.),(1.,1.),(1.,1.),(1.,1.),(1.,1.),(1.,1.),(1.,1.),(1.,1.),(1.,1.),(1.,
1.),(1.,1.),(1.,1.),(1.,1.),(1.,1.),(1.,1.),(1.,1.),(1.,1.),(1.,1.),(1.,
1.),(1.,1.),(1.,1.),(1.,1.),(1.,1.),(1.,1.),(1.,1.),(1.,1.),(1.,1.),(1.,
1.),(1.,1.),(1.,1.),(1.,1.),(1.,1.),(1.,1.),(1.,1.),(1.,1.),(1.,1.),(1.,
1.),(1.,1.),(1.,1.),(1.,1.),(1.,1.),(1.,1.),(1.,1.),(1.,1.),(1.,1.),(1.,
1.),(1.,1.),(1.,1.),(1.,1.),(1.,1.),(1.,1.),(1.,1.),(1.,1.),(1.,1.),(1.,
1.),(1.,1.),(1.,1.),(1.,1.),(1.,1.),(1.,1.),(1.,1.),(1.,1.),(1.,1.),(1.,
1.),(1.,1.)))
REPRESENTATION_ITEM('')
SURFACE()
);
#122=(
BOUNDED_SURFACE()
B_SPLINE_SURFACE(5,1,((#62327,#62328),(#62329,#62330),(#62331,#62332),(#62333,
#62334),(#62335,#62336),(#62337,#62338),(#62339,#62340),(#62341,#62342),
(#62343,#62344),(#62345,#62346),(#62347,#62348),(#62349,#62350),(#62351,
#62352),(#62353,#62354),(#62355,#62356),(#62357,#62358),(#62359,#62360),
(#62361,#62362),(#62363,#62364),(#62365,#62366),(#62367,#62368),(#62369,
#62370),(#62371,#62372),(#62373,#62374),(#62375,#62376),(#62377,#62378),
(#62379,#62380),(#62381,#62382),(#62383,#62384),(#62385,#62386),(#62387,
#62388),(#62389,#62390),(#62391,#62392),(#62393,#62394),(#62395,#62396),
(#62397,#62398),(#62399,#62400),(#62401,#62402),(#62403,#62404),(#62405,
#62406),(#62407,#62408),(#62409,#62410),(#62411,#62412),(#62413,#62414),
(#62415,#62416),(#62417,#62418),(#62419,#62420),(#62421,#62422),(#62423,
#62424),(#62425,#62426),(#62427,#62428),(#62429,#62430),(#62431,#62432),
(#62433,#62434),(#62435,#62436),(#62437,#62438),(#62439,#62440),(#62441,
#62442),(#62443,#62444),(#62445,#62446),(#62447,#62448),(#62449,#62450),
(#62451,#62452),(#62453,#62454),(#62455,#62456),(#62457,#62458),(#62459,
#62460),(#62461,#62462),(#62463,#62464),(#62465,#62466)),.UNSPECIFIED.,
 .F.,.F.,.F.)
B_SPLINE_SURFACE_WITH_KNOTS((6,1,1,1,1,1,1,1,1,1,1,1,1,1,1,1,1,1,1,1,1,
1,1,1,1,1,1,1,1,1,1,1,1,1,1,1,1,1,1,1,1,1,1,1,1,1,1,1,1,1,1,1,1,1,1,1,1,
1,1,1,1,1,1,1,1,6),(2,2),(-1.,-0.984615384615383,-0.969230769230768,-0.953846153846152,
-0.938461538461537,-0.923076923076922,-0.907692307692306,-0.892307692307691,
-0.876923076923076,-0.86153846153846,-0.846153846153845,-0.83076923076923,
-0.815384615384614,-0.799999999999999,-0.784615384615384,-0.769230769230768,
-0.753846153846153,-0.738461538461538,-0.723076923076922,-0.707692307692307,
-0.692307692307692,-0.676923076923076,-0.661538461538461,-0.646153846153846,
-0.63076923076923,-0.615384615384615,-0.6,-0.584615384615384,-0.569230769230769,
-0.553846153846154,-0.538461538461538,-0.523076923076923,-0.507692307692308,
-0.492307692307692,-0.476923076923077,-0.461538461538462,-0.446153846153846,
-0.430769230769231,-0.415384615384615,-0.4,-0.384615384615385,-0.369230769230769,
-0.353846153846154,-0.338461538461538,-0.323076923076923,-0.307692307692308,
-0.292307692307692,-0.276923076923077,-0.261538461538462,-0.246153846153846,
-0.230769230769231,-0.215384615384615,-0.2,-0.184615384615385,-0.169230769230769,
-0.153846153846154,-0.138461538461538,-0.123076923076923,-0.107692307692308,
-0.0923076923076923,-0.0769230769230769,-0.0615384615384615,-0.0461538461538462,
-0.0307692307692308,-0.0153846153846154,0.),(-1.,1.),.UNSPECIFIED.)
GEOMETRIC_REPRESENTATION_ITEM()
RATIONAL_B_SPLINE_SURFACE(((1.,1.),(1.,1.),(1.,1.),(1.,1.),(1.,1.),(1.,
1.),(1.,1.),(1.,1.),(1.,1.),(1.,1.),(1.,1.),(1.,1.),(1.,1.),(1.,1.),(1.,
1.),(1.,1.),(1.,1.),(1.,1.),(1.,1.),(1.,1.),(1.,1.),(1.,1.),(1.,1.),(1.,
1.),(1.,1.),(1.,1.),(1.,1.),(1.,1.),(1.,1.),(1.,1.),(1.,1.),(1.,1.),(1.,
1.),(1.,1.),(1.,1.),(1.,1.),(1.,1.),(1.,1.),(1.,1.),(1.,1.),(1.,1.),(1.,
1.),(1.,1.),(1.,1.),(1.,1.),(1.,1.),(1.,1.),(1.,1.),(1.,1.),(1.,1.),(1.,
1.),(1.,1.),(1.,1.),(1.,1.),(1.,1.),(1.,1.),(1.,1.),(1.,1.),(1.,1.),(1.,
1.),(1.,1.),(1.,1.),(1.,1.),(1.,1.),(1.,1.),(1.,1.),(1.,1.),(1.,1.),(1.,
1.),(1.,1.)))
REPRESENTATION_ITEM('')
SURFACE()
);
#123=(
BOUNDED_SURFACE()
B_SPLINE_SURFACE(5,1,((#62557,#62558),(#62559,#62560),(#62561,#62562),(#62563,
#62564),(#62565,#62566),(#62567,#62568),(#62569,#62570),(#62571,#62572),
(#62573,#62574),(#62575,#62576),(#62577,#62578),(#62579,#62580),(#62581,
#62582),(#62583,#62584),(#62585,#62586),(#62587,#62588),(#62589,#62590),
(#62591,#62592),(#62593,#62594),(#62595,#62596),(#62597,#62598),(#62599,
#62600),(#62601,#62602),(#62603,#62604),(#62605,#62606),(#62607,#62608),
(#62609,#62610),(#62611,#62612),(#62613,#62614),(#62615,#62616),(#62617,
#62618),(#62619,#62620),(#62621,#62622),(#62623,#62624),(#62625,#62626),
(#62627,#62628),(#62629,#62630),(#62631,#62632),(#62633,#62634),(#62635,
#62636),(#62637,#62638),(#62639,#62640),(#62641,#62642),(#62643,#62644),
(#62645,#62646),(#62647,#62648),(#62649,#62650),(#62651,#62652),(#62653,
#62654),(#62655,#62656),(#62657,#62658),(#62659,#62660),(#62661,#62662),
(#62663,#62664),(#62665,#62666),(#62667,#62668),(#62669,#62670),(#62671,
#62672),(#62673,#62674),(#62675,#62676),(#62677,#62678),(#62679,#62680),
(#62681,#62682),(#62683,#62684),(#62685,#62686),(#62687,#62688),(#62689,
#62690),(#62691,#62692),(#62693,#62694),(#62695,#62696)),.UNSPECIFIED.,
 .F.,.F.,.F.)
B_SPLINE_SURFACE_WITH_KNOTS((6,1,1,1,1,1,1,1,1,1,1,1,1,1,1,1,1,1,1,1,1,
1,1,1,1,1,1,1,1,1,1,1,1,1,1,1,1,1,1,1,1,1,1,1,1,1,1,1,1,1,1,1,1,1,1,1,1,
1,1,1,1,1,1,1,1,6),(2,2),(-1.,-0.984615384615383,-0.969230769230768,-0.953846153846152,
-0.938461538461537,-0.923076923076922,-0.907692307692306,-0.892307692307691,
-0.876923076923076,-0.86153846153846,-0.846153846153845,-0.83076923076923,
-0.815384615384614,-0.799999999999999,-0.784615384615384,-0.769230769230768,
-0.753846153846153,-0.738461538461538,-0.723076923076922,-0.707692307692307,
-0.692307692307692,-0.676923076923076,-0.661538461538461,-0.646153846153846,
-0.63076923076923,-0.615384615384615,-0.6,-0.584615384615384,-0.569230769230769,
-0.553846153846154,-0.538461538461538,-0.523076923076923,-0.507692307692308,
-0.492307692307692,-0.476923076923077,-0.461538461538462,-0.446153846153846,
-0.430769230769231,-0.415384615384615,-0.4,-0.384615384615385,-0.369230769230769,
-0.353846153846154,-0.338461538461538,-0.323076923076923,-0.307692307692308,
-0.292307692307692,-0.276923076923077,-0.261538461538462,-0.246153846153846,
-0.230769230769231,-0.215384615384615,-0.2,-0.184615384615385,-0.169230769230769,
-0.153846153846154,-0.138461538461538,-0.123076923076923,-0.107692307692308,
-0.0923076923076923,-0.0769230769230769,-0.0615384615384615,-0.0461538461538462,
-0.0307692307692308,-0.0153846153846154,0.),(-1.,1.),.UNSPECIFIED.)
GEOMETRIC_REPRESENTATION_ITEM()
RATIONAL_B_SPLINE_SURFACE(((1.,1.),(1.,1.),(1.,1.),(1.,1.),(1.,1.),(1.,
1.),(1.,1.),(1.,1.),(1.,1.),(1.,1.),(1.,1.),(1.,1.),(1.,1.),(1.,1.),(1.,
1.),(1.,1.),(1.,1.),(1.,1.),(1.,1.),(1.,1.),(1.,1.),(1.,1.),(1.,1.),(1.,
1.),(1.,1.),(1.,1.),(1.,1.),(1.,1.),(1.,1.),(1.,1.),(1.,1.),(1.,1.),(1.,
1.),(1.,1.),(1.,1.),(1.,1.),(1.,1.),(1.,1.),(1.,1.),(1.,1.),(1.,1.),(1.,
1.),(1.,1.),(1.,1.),(1.,1.),(1.,1.),(1.,1.),(1.,1.),(1.,1.),(1.,1.),(1.,
1.),(1.,1.),(1.,1.),(1.,1.),(1.,1.),(1.,1.),(1.,1.),(1.,1.),(1.,1.),(1.,
1.),(1.,1.),(1.,1.),(1.,1.),(1.,1.),(1.,1.),(1.,1.),(1.,1.),(1.,1.),(1.,
1.),(1.,1.)))
REPRESENTATION_ITEM('')
SURFACE()
);
#124=(
BOUNDED_SURFACE()
B_SPLINE_SURFACE(5,1,((#62769,#62770),(#62771,#62772),(#62773,#62774),(#62775,
#62776),(#62777,#62778),(#62779,#62780),(#62781,#62782),(#62783,#62784),
(#62785,#62786),(#62787,#62788),(#62789,#62790),(#62791,#62792),(#62793,
#62794),(#62795,#62796),(#62797,#62798),(#62799,#62800),(#62801,#62802),
(#62803,#62804),(#62805,#62806),(#62807,#62808),(#62809,#62810),(#62811,
#62812),(#62813,#62814),(#62815,#62816),(#62817,#62818),(#62819,#62820),
(#62821,#62822),(#62823,#62824),(#62825,#62826),(#62827,#62828),(#62829,
#62830),(#62831,#62832),(#62833,#62834),(#62835,#62836),(#62837,#62838),
(#62839,#62840),(#62841,#62842),(#62843,#62844),(#62845,#62846),(#62847,
#62848),(#62849,#62850),(#62851,#62852),(#62853,#62854),(#62855,#62856),
(#62857,#62858),(#62859,#62860),(#62861,#62862),(#62863,#62864),(#62865,
#62866),(#62867,#62868),(#62869,#62870),(#62871,#62872),(#62873,#62874),
(#62875,#62876),(#62877,#62878),(#62879,#62880),(#62881,#62882),(#62883,
#62884),(#62885,#62886),(#62887,#62888),(#62889,#62890),(#62891,#62892),
(#62893,#62894),(#62895,#62896),(#62897,#62898),(#62899,#62900),(#62901,
#62902),(#62903,#62904),(#62905,#62906),(#62907,#62908)),.UNSPECIFIED.,
 .F.,.F.,.F.)
B_SPLINE_SURFACE_WITH_KNOTS((6,1,1,1,1,1,1,1,1,1,1,1,1,1,1,1,1,1,1,1,1,
1,1,1,1,1,1,1,1,1,1,1,1,1,1,1,1,1,1,1,1,1,1,1,1,1,1,1,1,1,1,1,1,1,1,1,1,
1,1,1,1,1,1,1,1,6),(2,2),(-1.,-0.984615384615383,-0.969230769230768,-0.953846153846152,
-0.938461538461537,-0.923076923076922,-0.907692307692306,-0.892307692307691,
-0.876923076923076,-0.86153846153846,-0.846153846153845,-0.83076923076923,
-0.815384615384614,-0.799999999999999,-0.784615384615384,-0.769230769230768,
-0.753846153846153,-0.738461538461538,-0.723076923076922,-0.707692307692307,
-0.692307692307692,-0.676923076923076,-0.661538461538461,-0.646153846153846,
-0.63076923076923,-0.615384615384615,-0.6,-0.584615384615384,-0.569230769230769,
-0.553846153846154,-0.538461538461538,-0.523076923076923,-0.507692307692308,
-0.492307692307692,-0.476923076923077,-0.461538461538462,-0.446153846153846,
-0.430769230769231,-0.415384615384615,-0.4,-0.384615384615385,-0.369230769230769,
-0.353846153846154,-0.338461538461538,-0.323076923076923,-0.307692307692308,
-0.292307692307692,-0.276923076923077,-0.261538461538462,-0.246153846153846,
-0.230769230769231,-0.215384615384615,-0.2,-0.184615384615385,-0.169230769230769,
-0.153846153846154,-0.138461538461538,-0.123076923076923,-0.107692307692308,
-0.0923076923076923,-0.0769230769230769,-0.0615384615384615,-0.0461538461538462,
-0.0307692307692308,-0.0153846153846154,0.),(-1.,1.),.UNSPECIFIED.)
GEOMETRIC_REPRESENTATION_ITEM()
RATIONAL_B_SPLINE_SURFACE(((1.,1.),(1.,1.),(1.,1.),(1.,1.),(1.,1.),(1.,
1.),(1.,1.),(1.,1.),(1.,1.),(1.,1.),(1.,1.),(1.,1.),(1.,1.),(1.,1.),(1.,
1.),(1.,1.),(1.,1.),(1.,1.),(1.,1.),(1.,1.),(1.,1.),(1.,1.),(1.,1.),(1.,
1.),(1.,1.),(1.,1.),(1.,1.),(1.,1.),(1.,1.),(1.,1.),(1.,1.),(1.,1.),(1.,
1.),(1.,1.),(1.,1.),(1.,1.),(1.,1.),(1.,1.),(1.,1.),(1.,1.),(1.,1.),(1.,
1.),(1.,1.),(1.,1.),(1.,1.),(1.,1.),(1.,1.),(1.,1.),(1.,1.),(1.,1.),(1.,
1.),(1.,1.),(1.,1.),(1.,1.),(1.,1.),(1.,1.),(1.,1.),(1.,1.),(1.,1.),(1.,
1.),(1.,1.),(1.,1.),(1.,1.),(1.,1.),(1.,1.),(1.,1.),(1.,1.),(1.,1.),(1.,
1.),(1.,1.)))
REPRESENTATION_ITEM('')
SURFACE()
);
#125=(
BOUNDED_SURFACE()
B_SPLINE_SURFACE(5,1,((#62999,#63000),(#63001,#63002),(#63003,#63004),(#63005,
#63006),(#63007,#63008),(#63009,#63010),(#63011,#63012),(#63013,#63014),
(#63015,#63016),(#63017,#63018),(#63019,#63020),(#63021,#63022),(#63023,
#63024),(#63025,#63026),(#63027,#63028),(#63029,#63030),(#63031,#63032),
(#63033,#63034),(#63035,#63036),(#63037,#63038),(#63039,#63040),(#63041,
#63042),(#63043,#63044),(#63045,#63046),(#63047,#63048),(#63049,#63050),
(#63051,#63052),(#63053,#63054),(#63055,#63056),(#63057,#63058),(#63059,
#63060),(#63061,#63062),(#63063,#63064),(#63065,#63066),(#63067,#63068),
(#63069,#63070),(#63071,#63072),(#63073,#63074),(#63075,#63076),(#63077,
#63078),(#63079,#63080),(#63081,#63082),(#63083,#63084),(#63085,#63086),
(#63087,#63088),(#63089,#63090),(#63091,#63092),(#63093,#63094),(#63095,
#63096),(#63097,#63098),(#63099,#63100),(#63101,#63102),(#63103,#63104),
(#63105,#63106),(#63107,#63108),(#63109,#63110),(#63111,#63112),(#63113,
#63114),(#63115,#63116),(#63117,#63118),(#63119,#63120),(#63121,#63122),
(#63123,#63124),(#63125,#63126),(#63127,#63128),(#63129,#63130),(#63131,
#63132),(#63133,#63134),(#63135,#63136),(#63137,#63138)),.UNSPECIFIED.,
 .F.,.F.,.F.)
B_SPLINE_SURFACE_WITH_KNOTS((6,1,1,1,1,1,1,1,1,1,1,1,1,1,1,1,1,1,1,1,1,
1,1,1,1,1,1,1,1,1,1,1,1,1,1,1,1,1,1,1,1,1,1,1,1,1,1,1,1,1,1,1,1,1,1,1,1,
1,1,1,1,1,1,1,1,6),(2,2),(-1.,-0.984615384615383,-0.969230769230768,-0.953846153846152,
-0.938461538461537,-0.923076923076922,-0.907692307692306,-0.892307692307691,
-0.876923076923076,-0.86153846153846,-0.846153846153845,-0.83076923076923,
-0.815384615384614,-0.799999999999999,-0.784615384615384,-0.769230769230768,
-0.753846153846153,-0.738461538461538,-0.723076923076922,-0.707692307692307,
-0.692307692307692,-0.676923076923076,-0.661538461538461,-0.646153846153846,
-0.63076923076923,-0.615384615384615,-0.6,-0.584615384615384,-0.569230769230769,
-0.553846153846154,-0.538461538461538,-0.523076923076923,-0.507692307692308,
-0.492307692307692,-0.476923076923077,-0.461538461538462,-0.446153846153846,
-0.430769230769231,-0.415384615384615,-0.4,-0.384615384615385,-0.369230769230769,
-0.353846153846154,-0.338461538461538,-0.323076923076923,-0.307692307692308,
-0.292307692307692,-0.276923076923077,-0.261538461538462,-0.246153846153846,
-0.230769230769231,-0.215384615384615,-0.2,-0.184615384615385,-0.169230769230769,
-0.153846153846154,-0.138461538461538,-0.123076923076923,-0.107692307692308,
-0.0923076923076923,-0.0769230769230769,-0.0615384615384615,-0.0461538461538462,
-0.0307692307692308,-0.0153846153846154,0.),(-1.,1.),.UNSPECIFIED.)
GEOMETRIC_REPRESENTATION_ITEM()
RATIONAL_B_SPLINE_SURFACE(((1.,1.),(1.,1.),(1.,1.),(1.,1.),(1.,1.),(1.,
1.),(1.,1.),(1.,1.),(1.,1.),(1.,1.),(1.,1.),(1.,1.),(1.,1.),(1.,1.),(1.,
1.),(1.,1.),(1.,1.),(1.,1.),(1.,1.),(1.,1.),(1.,1.),(1.,1.),(1.,1.),(1.,
1.),(1.,1.),(1.,1.),(1.,1.),(1.,1.),(1.,1.),(1.,1.),(1.,1.),(1.,1.),(1.,
1.),(1.,1.),(1.,1.),(1.,1.),(1.,1.),(1.,1.),(1.,1.),(1.,1.),(1.,1.),(1.,
1.),(1.,1.),(1.,1.),(1.,1.),(1.,1.),(1.,1.),(1.,1.),(1.,1.),(1.,1.),(1.,
1.),(1.,1.),(1.,1.),(1.,1.),(1.,1.),(1.,1.),(1.,1.),(1.,1.),(1.,1.),(1.,
1.),(1.,1.),(1.,1.),(1.,1.),(1.,1.),(1.,1.),(1.,1.),(1.,1.),(1.,1.),(1.,
1.),(1.,1.)))
REPRESENTATION_ITEM('')
SURFACE()
);
#126=(
BOUNDED_SURFACE()
B_SPLINE_SURFACE(5,1,((#63211,#63212),(#63213,#63214),(#63215,#63216),(#63217,
#63218),(#63219,#63220),(#63221,#63222),(#63223,#63224),(#63225,#63226),
(#63227,#63228),(#63229,#63230),(#63231,#63232),(#63233,#63234),(#63235,
#63236),(#63237,#63238),(#63239,#63240),(#63241,#63242),(#63243,#63244),
(#63245,#63246),(#63247,#63248),(#63249,#63250),(#63251,#63252),(#63253,
#63254),(#63255,#63256),(#63257,#63258),(#63259,#63260),(#63261,#63262),
(#63263,#63264),(#63265,#63266),(#63267,#63268),(#63269,#63270),(#63271,
#63272),(#63273,#63274),(#63275,#63276),(#63277,#63278),(#63279,#63280),
(#63281,#63282),(#63283,#63284),(#63285,#63286),(#63287,#63288),(#63289,
#63290),(#63291,#63292),(#63293,#63294),(#63295,#63296),(#63297,#63298),
(#63299,#63300),(#63301,#63302),(#63303,#63304),(#63305,#63306),(#63307,
#63308),(#63309,#63310),(#63311,#63312),(#63313,#63314),(#63315,#63316),
(#63317,#63318),(#63319,#63320),(#63321,#63322),(#63323,#63324),(#63325,
#63326),(#63327,#63328),(#63329,#63330),(#63331,#63332),(#63333,#63334),
(#63335,#63336),(#63337,#63338),(#63339,#63340),(#63341,#63342),(#63343,
#63344),(#63345,#63346),(#63347,#63348),(#63349,#63350)),.UNSPECIFIED.,
 .F.,.F.,.F.)
B_SPLINE_SURFACE_WITH_KNOTS((6,1,1,1,1,1,1,1,1,1,1,1,1,1,1,1,1,1,1,1,1,
1,1,1,1,1,1,1,1,1,1,1,1,1,1,1,1,1,1,1,1,1,1,1,1,1,1,1,1,1,1,1,1,1,1,1,1,
1,1,1,1,1,1,1,1,6),(2,2),(-1.,-0.984615384615383,-0.969230769230768,-0.953846153846152,
-0.938461538461537,-0.923076923076922,-0.907692307692306,-0.892307692307691,
-0.876923076923076,-0.86153846153846,-0.846153846153845,-0.83076923076923,
-0.815384615384614,-0.799999999999999,-0.784615384615384,-0.769230769230768,
-0.753846153846153,-0.738461538461538,-0.723076923076922,-0.707692307692307,
-0.692307692307692,-0.676923076923076,-0.661538461538461,-0.646153846153846,
-0.63076923076923,-0.615384615384615,-0.6,-0.584615384615384,-0.569230769230769,
-0.553846153846154,-0.538461538461538,-0.523076923076923,-0.507692307692308,
-0.492307692307692,-0.476923076923077,-0.461538461538462,-0.446153846153846,
-0.430769230769231,-0.415384615384615,-0.4,-0.384615384615385,-0.369230769230769,
-0.353846153846154,-0.338461538461538,-0.323076923076923,-0.307692307692308,
-0.292307692307692,-0.276923076923077,-0.261538461538462,-0.246153846153846,
-0.230769230769231,-0.215384615384615,-0.2,-0.184615384615385,-0.169230769230769,
-0.153846153846154,-0.138461538461538,-0.123076923076923,-0.107692307692308,
-0.0923076923076923,-0.0769230769230769,-0.0615384615384615,-0.0461538461538462,
-0.0307692307692308,-0.0153846153846154,0.),(-1.,1.),.UNSPECIFIED.)
GEOMETRIC_REPRESENTATION_ITEM()
RATIONAL_B_SPLINE_SURFACE(((1.,1.),(1.,1.),(1.,1.),(1.,1.),(1.,1.),(1.,
1.),(1.,1.),(1.,1.),(1.,1.),(1.,1.),(1.,1.),(1.,1.),(1.,1.),(1.,1.),(1.,
1.),(1.,1.),(1.,1.),(1.,1.),(1.,1.),(1.,1.),(1.,1.),(1.,1.),(1.,1.),(1.,
1.),(1.,1.),(1.,1.),(1.,1.),(1.,1.),(1.,1.),(1.,1.),(1.,1.),(1.,1.),(1.,
1.),(1.,1.),(1.,1.),(1.,1.),(1.,1.),(1.,1.),(1.,1.),(1.,1.),(1.,1.),(1.,
1.),(1.,1.),(1.,1.),(1.,1.),(1.,1.),(1.,1.),(1.,1.),(1.,1.),(1.,1.),(1.,
1.),(1.,1.),(1.,1.),(1.,1.),(1.,1.),(1.,1.),(1.,1.),(1.,1.),(1.,1.),(1.,
1.),(1.,1.),(1.,1.),(1.,1.),(1.,1.),(1.,1.),(1.,1.),(1.,1.),(1.,1.),(1.,
1.),(1.,1.)))
REPRESENTATION_ITEM('')
SURFACE()
);
#127=(
BOUNDED_SURFACE()
B_SPLINE_SURFACE(5,1,((#63441,#63442),(#63443,#63444),(#63445,#63446),(#63447,
#63448),(#63449,#63450),(#63451,#63452),(#63453,#63454),(#63455,#63456),
(#63457,#63458),(#63459,#63460),(#63461,#63462),(#63463,#63464),(#63465,
#63466),(#63467,#63468),(#63469,#63470),(#63471,#63472),(#63473,#63474),
(#63475,#63476),(#63477,#63478),(#63479,#63480),(#63481,#63482),(#63483,
#63484),(#63485,#63486),(#63487,#63488),(#63489,#63490),(#63491,#63492),
(#63493,#63494),(#63495,#63496),(#63497,#63498),(#63499,#63500),(#63501,
#63502),(#63503,#63504),(#63505,#63506),(#63507,#63508),(#63509,#63510),
(#63511,#63512),(#63513,#63514),(#63515,#63516),(#63517,#63518),(#63519,
#63520),(#63521,#63522),(#63523,#63524),(#63525,#63526),(#63527,#63528),
(#63529,#63530),(#63531,#63532),(#63533,#63534),(#63535,#63536),(#63537,
#63538),(#63539,#63540),(#63541,#63542),(#63543,#63544),(#63545,#63546),
(#63547,#63548),(#63549,#63550),(#63551,#63552),(#63553,#63554),(#63555,
#63556),(#63557,#63558),(#63559,#63560),(#63561,#63562),(#63563,#63564),
(#63565,#63566),(#63567,#63568),(#63569,#63570),(#63571,#63572),(#63573,
#63574),(#63575,#63576),(#63577,#63578),(#63579,#63580)),.UNSPECIFIED.,
 .F.,.F.,.F.)
B_SPLINE_SURFACE_WITH_KNOTS((6,1,1,1,1,1,1,1,1,1,1,1,1,1,1,1,1,1,1,1,1,
1,1,1,1,1,1,1,1,1,1,1,1,1,1,1,1,1,1,1,1,1,1,1,1,1,1,1,1,1,1,1,1,1,1,1,1,
1,1,1,1,1,1,1,1,6),(2,2),(-1.,-0.984615384615383,-0.969230769230768,-0.953846153846152,
-0.938461538461537,-0.923076923076922,-0.907692307692306,-0.892307692307691,
-0.876923076923076,-0.86153846153846,-0.846153846153845,-0.83076923076923,
-0.815384615384614,-0.799999999999999,-0.784615384615384,-0.769230769230768,
-0.753846153846153,-0.738461538461538,-0.723076923076922,-0.707692307692307,
-0.692307692307692,-0.676923076923076,-0.661538461538461,-0.646153846153846,
-0.63076923076923,-0.615384615384615,-0.6,-0.584615384615384,-0.569230769230769,
-0.553846153846154,-0.538461538461538,-0.523076923076923,-0.507692307692308,
-0.492307692307692,-0.476923076923077,-0.461538461538462,-0.446153846153846,
-0.430769230769231,-0.415384615384615,-0.4,-0.384615384615385,-0.369230769230769,
-0.353846153846154,-0.338461538461538,-0.323076923076923,-0.307692307692308,
-0.292307692307692,-0.276923076923077,-0.261538461538462,-0.246153846153846,
-0.230769230769231,-0.215384615384615,-0.2,-0.184615384615385,-0.169230769230769,
-0.153846153846154,-0.138461538461538,-0.123076923076923,-0.107692307692308,
-0.0923076923076923,-0.0769230769230769,-0.0615384615384615,-0.0461538461538462,
-0.0307692307692308,-0.0153846153846154,0.),(-1.,1.),.UNSPECIFIED.)
GEOMETRIC_REPRESENTATION_ITEM()
RATIONAL_B_SPLINE_SURFACE(((1.,1.),(1.,1.),(1.,1.),(1.,1.),(1.,1.),(1.,
1.),(1.,1.),(1.,1.),(1.,1.),(1.,1.),(1.,1.),(1.,1.),(1.,1.),(1.,1.),(1.,
1.),(1.,1.),(1.,1.),(1.,1.),(1.,1.),(1.,1.),(1.,1.),(1.,1.),(1.,1.),(1.,
1.),(1.,1.),(1.,1.),(1.,1.),(1.,1.),(1.,1.),(1.,1.),(1.,1.),(1.,1.),(1.,
1.),(1.,1.),(1.,1.),(1.,1.),(1.,1.),(1.,1.),(1.,1.),(1.,1.),(1.,1.),(1.,
1.),(1.,1.),(1.,1.),(1.,1.),(1.,1.),(1.,1.),(1.,1.),(1.,1.),(1.,1.),(1.,
1.),(1.,1.),(1.,1.),(1.,1.),(1.,1.),(1.,1.),(1.,1.),(1.,1.),(1.,1.),(1.,
1.),(1.,1.),(1.,1.),(1.,1.),(1.,1.),(1.,1.),(1.,1.),(1.,1.),(1.,1.),(1.,
1.),(1.,1.)))
REPRESENTATION_ITEM('')
SURFACE()
);
#128=(
BOUNDED_SURFACE()
B_SPLINE_SURFACE(5,1,((#63653,#63654),(#63655,#63656),(#63657,#63658),(#63659,
#63660),(#63661,#63662),(#63663,#63664),(#63665,#63666),(#63667,#63668),
(#63669,#63670),(#63671,#63672),(#63673,#63674),(#63675,#63676),(#63677,
#63678),(#63679,#63680),(#63681,#63682),(#63683,#63684),(#63685,#63686),
(#63687,#63688),(#63689,#63690),(#63691,#63692),(#63693,#63694),(#63695,
#63696),(#63697,#63698),(#63699,#63700),(#63701,#63702),(#63703,#63704),
(#63705,#63706),(#63707,#63708),(#63709,#63710),(#63711,#63712),(#63713,
#63714),(#63715,#63716),(#63717,#63718),(#63719,#63720),(#63721,#63722),
(#63723,#63724),(#63725,#63726),(#63727,#63728),(#63729,#63730),(#63731,
#63732),(#63733,#63734),(#63735,#63736),(#63737,#63738),(#63739,#63740),
(#63741,#63742),(#63743,#63744),(#63745,#63746),(#63747,#63748),(#63749,
#63750),(#63751,#63752),(#63753,#63754),(#63755,#63756),(#63757,#63758),
(#63759,#63760),(#63761,#63762),(#63763,#63764),(#63765,#63766),(#63767,
#63768),(#63769,#63770),(#63771,#63772),(#63773,#63774),(#63775,#63776),
(#63777,#63778),(#63779,#63780),(#63781,#63782),(#63783,#63784),(#63785,
#63786),(#63787,#63788),(#63789,#63790),(#63791,#63792)),.UNSPECIFIED.,
 .F.,.F.,.F.)
B_SPLINE_SURFACE_WITH_KNOTS((6,1,1,1,1,1,1,1,1,1,1,1,1,1,1,1,1,1,1,1,1,
1,1,1,1,1,1,1,1,1,1,1,1,1,1,1,1,1,1,1,1,1,1,1,1,1,1,1,1,1,1,1,1,1,1,1,1,
1,1,1,1,1,1,1,1,6),(2,2),(-1.,-0.984615384615383,-0.969230769230768,-0.953846153846152,
-0.938461538461537,-0.923076923076922,-0.907692307692306,-0.892307692307691,
-0.876923076923076,-0.86153846153846,-0.846153846153845,-0.83076923076923,
-0.815384615384614,-0.799999999999999,-0.784615384615384,-0.769230769230768,
-0.753846153846153,-0.738461538461538,-0.723076923076922,-0.707692307692307,
-0.692307692307692,-0.676923076923076,-0.661538461538461,-0.646153846153846,
-0.63076923076923,-0.615384615384615,-0.6,-0.584615384615384,-0.569230769230769,
-0.553846153846154,-0.538461538461538,-0.523076923076923,-0.507692307692308,
-0.492307692307692,-0.476923076923077,-0.461538461538462,-0.446153846153846,
-0.430769230769231,-0.415384615384615,-0.4,-0.384615384615385,-0.369230769230769,
-0.353846153846154,-0.338461538461538,-0.323076923076923,-0.307692307692308,
-0.292307692307692,-0.276923076923077,-0.261538461538462,-0.246153846153846,
-0.230769230769231,-0.215384615384615,-0.2,-0.184615384615385,-0.169230769230769,
-0.153846153846154,-0.138461538461538,-0.123076923076923,-0.107692307692308,
-0.0923076923076923,-0.0769230769230769,-0.0615384615384615,-0.0461538461538462,
-0.0307692307692308,-0.0153846153846154,0.),(-1.,1.),.UNSPECIFIED.)
GEOMETRIC_REPRESENTATION_ITEM()
RATIONAL_B_SPLINE_SURFACE(((1.,1.),(1.,1.),(1.,1.),(1.,1.),(1.,1.),(1.,
1.),(1.,1.),(1.,1.),(1.,1.),(1.,1.),(1.,1.),(1.,1.),(1.,1.),(1.,1.),(1.,
1.),(1.,1.),(1.,1.),(1.,1.),(1.,1.),(1.,1.),(1.,1.),(1.,1.),(1.,1.),(1.,
1.),(1.,1.),(1.,1.),(1.,1.),(1.,1.),(1.,1.),(1.,1.),(1.,1.),(1.,1.),(1.,
1.),(1.,1.),(1.,1.),(1.,1.),(1.,1.),(1.,1.),(1.,1.),(1.,1.),(1.,1.),(1.,
1.),(1.,1.),(1.,1.),(1.,1.),(1.,1.),(1.,1.),(1.,1.),(1.,1.),(1.,1.),(1.,
1.),(1.,1.),(1.,1.),(1.,1.),(1.,1.),(1.,1.),(1.,1.),(1.,1.),(1.,1.),(1.,
1.),(1.,1.),(1.,1.),(1.,1.),(1.,1.),(1.,1.),(1.,1.),(1.,1.),(1.,1.),(1.,
1.),(1.,1.)))
REPRESENTATION_ITEM('')
SURFACE()
);
#129=(
BOUNDED_SURFACE()
B_SPLINE_SURFACE(5,1,((#63883,#63884),(#63885,#63886),(#63887,#63888),(#63889,
#63890),(#63891,#63892),(#63893,#63894),(#63895,#63896),(#63897,#63898),
(#63899,#63900),(#63901,#63902),(#63903,#63904),(#63905,#63906),(#63907,
#63908),(#63909,#63910),(#63911,#63912),(#63913,#63914),(#63915,#63916),
(#63917,#63918),(#63919,#63920),(#63921,#63922),(#63923,#63924),(#63925,
#63926),(#63927,#63928),(#63929,#63930),(#63931,#63932),(#63933,#63934),
(#63935,#63936),(#63937,#63938),(#63939,#63940),(#63941,#63942),(#63943,
#63944),(#63945,#63946),(#63947,#63948),(#63949,#63950),(#63951,#63952),
(#63953,#63954),(#63955,#63956),(#63957,#63958),(#63959,#63960),(#63961,
#63962),(#63963,#63964),(#63965,#63966),(#63967,#63968),(#63969,#63970),
(#63971,#63972),(#63973,#63974),(#63975,#63976),(#63977,#63978),(#63979,
#63980),(#63981,#63982),(#63983,#63984),(#63985,#63986),(#63987,#63988),
(#63989,#63990),(#63991,#63992),(#63993,#63994),(#63995,#63996),(#63997,
#63998),(#63999,#64000),(#64001,#64002),(#64003,#64004),(#64005,#64006),
(#64007,#64008),(#64009,#64010),(#64011,#64012),(#64013,#64014),(#64015,
#64016),(#64017,#64018),(#64019,#64020),(#64021,#64022)),.UNSPECIFIED.,
 .F.,.F.,.F.)
B_SPLINE_SURFACE_WITH_KNOTS((6,1,1,1,1,1,1,1,1,1,1,1,1,1,1,1,1,1,1,1,1,
1,1,1,1,1,1,1,1,1,1,1,1,1,1,1,1,1,1,1,1,1,1,1,1,1,1,1,1,1,1,1,1,1,1,1,1,
1,1,1,1,1,1,1,1,6),(2,2),(-1.,-0.984615384615383,-0.969230769230768,-0.953846153846152,
-0.938461538461537,-0.923076923076922,-0.907692307692306,-0.892307692307691,
-0.876923076923076,-0.86153846153846,-0.846153846153845,-0.83076923076923,
-0.815384615384614,-0.799999999999999,-0.784615384615384,-0.769230769230768,
-0.753846153846153,-0.738461538461538,-0.723076923076922,-0.707692307692307,
-0.692307692307692,-0.676923076923076,-0.661538461538461,-0.646153846153846,
-0.63076923076923,-0.615384615384615,-0.6,-0.584615384615384,-0.569230769230769,
-0.553846153846154,-0.538461538461538,-0.523076923076923,-0.507692307692308,
-0.492307692307692,-0.476923076923077,-0.461538461538462,-0.446153846153846,
-0.430769230769231,-0.415384615384615,-0.4,-0.384615384615385,-0.369230769230769,
-0.353846153846154,-0.338461538461538,-0.323076923076923,-0.307692307692308,
-0.292307692307692,-0.276923076923077,-0.261538461538462,-0.246153846153846,
-0.230769230769231,-0.215384615384615,-0.2,-0.184615384615385,-0.169230769230769,
-0.153846153846154,-0.138461538461538,-0.123076923076923,-0.107692307692308,
-0.0923076923076923,-0.0769230769230769,-0.0615384615384615,-0.0461538461538462,
-0.0307692307692308,-0.0153846153846154,0.),(-1.,1.),.UNSPECIFIED.)
GEOMETRIC_REPRESENTATION_ITEM()
RATIONAL_B_SPLINE_SURFACE(((1.,1.),(1.,1.),(1.,1.),(1.,1.),(1.,1.),(1.,
1.),(1.,1.),(1.,1.),(1.,1.),(1.,1.),(1.,1.),(1.,1.),(1.,1.),(1.,1.),(1.,
1.),(1.,1.),(1.,1.),(1.,1.),(1.,1.),(1.,1.),(1.,1.),(1.,1.),(1.,1.),(1.,
1.),(1.,1.),(1.,1.),(1.,1.),(1.,1.),(1.,1.),(1.,1.),(1.,1.),(1.,1.),(1.,
1.),(1.,1.),(1.,1.),(1.,1.),(1.,1.),(1.,1.),(1.,1.),(1.,1.),(1.,1.),(1.,
1.),(1.,1.),(1.,1.),(1.,1.),(1.,1.),(1.,1.),(1.,1.),(1.,1.),(1.,1.),(1.,
1.),(1.,1.),(1.,1.),(1.,1.),(1.,1.),(1.,1.),(1.,1.),(1.,1.),(1.,1.),(1.,
1.),(1.,1.),(1.,1.),(1.,1.),(1.,1.),(1.,1.),(1.,1.),(1.,1.),(1.,1.),(1.,
1.),(1.,1.)))
REPRESENTATION_ITEM('')
SURFACE()
);
#130=(
BOUNDED_SURFACE()
B_SPLINE_SURFACE(5,1,((#64095,#64096),(#64097,#64098),(#64099,#64100),(#64101,
#64102),(#64103,#64104),(#64105,#64106),(#64107,#64108),(#64109,#64110),
(#64111,#64112),(#64113,#64114),(#64115,#64116),(#64117,#64118),(#64119,
#64120),(#64121,#64122),(#64123,#64124),(#64125,#64126),(#64127,#64128),
(#64129,#64130),(#64131,#64132),(#64133,#64134),(#64135,#64136),(#64137,
#64138),(#64139,#64140),(#64141,#64142),(#64143,#64144),(#64145,#64146),
(#64147,#64148),(#64149,#64150),(#64151,#64152),(#64153,#64154),(#64155,
#64156),(#64157,#64158),(#64159,#64160),(#64161,#64162),(#64163,#64164),
(#64165,#64166),(#64167,#64168),(#64169,#64170),(#64171,#64172),(#64173,
#64174),(#64175,#64176),(#64177,#64178),(#64179,#64180),(#64181,#64182),
(#64183,#64184),(#64185,#64186),(#64187,#64188),(#64189,#64190),(#64191,
#64192),(#64193,#64194),(#64195,#64196),(#64197,#64198),(#64199,#64200),
(#64201,#64202),(#64203,#64204),(#64205,#64206),(#64207,#64208),(#64209,
#64210),(#64211,#64212),(#64213,#64214),(#64215,#64216),(#64217,#64218),
(#64219,#64220),(#64221,#64222),(#64223,#64224),(#64225,#64226),(#64227,
#64228),(#64229,#64230),(#64231,#64232),(#64233,#64234)),.UNSPECIFIED.,
 .F.,.F.,.F.)
B_SPLINE_SURFACE_WITH_KNOTS((6,1,1,1,1,1,1,1,1,1,1,1,1,1,1,1,1,1,1,1,1,
1,1,1,1,1,1,1,1,1,1,1,1,1,1,1,1,1,1,1,1,1,1,1,1,1,1,1,1,1,1,1,1,1,1,1,1,
1,1,1,1,1,1,1,1,6),(2,2),(-1.,-0.984615384615383,-0.969230769230768,-0.953846153846152,
-0.938461538461537,-0.923076923076922,-0.907692307692306,-0.892307692307691,
-0.876923076923076,-0.86153846153846,-0.846153846153845,-0.83076923076923,
-0.815384615384614,-0.799999999999999,-0.784615384615384,-0.769230769230768,
-0.753846153846153,-0.738461538461538,-0.723076923076922,-0.707692307692307,
-0.692307692307692,-0.676923076923076,-0.661538461538461,-0.646153846153846,
-0.63076923076923,-0.615384615384615,-0.6,-0.584615384615384,-0.569230769230769,
-0.553846153846154,-0.538461538461538,-0.523076923076923,-0.507692307692308,
-0.492307692307692,-0.476923076923077,-0.461538461538462,-0.446153846153846,
-0.430769230769231,-0.415384615384615,-0.4,-0.384615384615385,-0.369230769230769,
-0.353846153846154,-0.338461538461538,-0.323076923076923,-0.307692307692308,
-0.292307692307692,-0.276923076923077,-0.261538461538462,-0.246153846153846,
-0.230769230769231,-0.215384615384615,-0.2,-0.184615384615385,-0.169230769230769,
-0.153846153846154,-0.138461538461538,-0.123076923076923,-0.107692307692308,
-0.0923076923076923,-0.0769230769230769,-0.0615384615384615,-0.0461538461538462,
-0.0307692307692308,-0.0153846153846154,0.),(-1.,1.),.UNSPECIFIED.)
GEOMETRIC_REPRESENTATION_ITEM()
RATIONAL_B_SPLINE_SURFACE(((1.,1.),(1.,1.),(1.,1.),(1.,1.),(1.,1.),(1.,
1.),(1.,1.),(1.,1.),(1.,1.),(1.,1.),(1.,1.),(1.,1.),(1.,1.),(1.,1.),(1.,
1.),(1.,1.),(1.,1.),(1.,1.),(1.,1.),(1.,1.),(1.,1.),(1.,1.),(1.,1.),(1.,
1.),(1.,1.),(1.,1.),(1.,1.),(1.,1.),(1.,1.),(1.,1.),(1.,1.),(1.,1.),(1.,
1.),(1.,1.),(1.,1.),(1.,1.),(1.,1.),(1.,1.),(1.,1.),(1.,1.),(1.,1.),(1.,
1.),(1.,1.),(1.,1.),(1.,1.),(1.,1.),(1.,1.),(1.,1.),(1.,1.),(1.,1.),(1.,
1.),(1.,1.),(1.,1.),(1.,1.),(1.,1.),(1.,1.),(1.,1.),(1.,1.),(1.,1.),(1.,
1.),(1.,1.),(1.,1.),(1.,1.),(1.,1.),(1.,1.),(1.,1.),(1.,1.),(1.,1.),(1.,
1.),(1.,1.)))
REPRESENTATION_ITEM('')
SURFACE()
);
#131=(
BOUNDED_SURFACE()
B_SPLINE_SURFACE(5,1,((#64325,#64326),(#64327,#64328),(#64329,#64330),(#64331,
#64332),(#64333,#64334),(#64335,#64336),(#64337,#64338),(#64339,#64340),
(#64341,#64342),(#64343,#64344),(#64345,#64346),(#64347,#64348),(#64349,
#64350),(#64351,#64352),(#64353,#64354),(#64355,#64356),(#64357,#64358),
(#64359,#64360),(#64361,#64362),(#64363,#64364),(#64365,#64366),(#64367,
#64368),(#64369,#64370),(#64371,#64372),(#64373,#64374),(#64375,#64376),
(#64377,#64378),(#64379,#64380),(#64381,#64382),(#64383,#64384),(#64385,
#64386),(#64387,#64388),(#64389,#64390),(#64391,#64392),(#64393,#64394),
(#64395,#64396),(#64397,#64398),(#64399,#64400),(#64401,#64402),(#64403,
#64404),(#64405,#64406),(#64407,#64408),(#64409,#64410),(#64411,#64412),
(#64413,#64414),(#64415,#64416),(#64417,#64418),(#64419,#64420),(#64421,
#64422),(#64423,#64424),(#64425,#64426),(#64427,#64428),(#64429,#64430),
(#64431,#64432),(#64433,#64434),(#64435,#64436),(#64437,#64438),(#64439,
#64440),(#64441,#64442),(#64443,#64444),(#64445,#64446),(#64447,#64448),
(#64449,#64450),(#64451,#64452),(#64453,#64454),(#64455,#64456),(#64457,
#64458),(#64459,#64460),(#64461,#64462),(#64463,#64464)),.UNSPECIFIED.,
 .F.,.F.,.F.)
B_SPLINE_SURFACE_WITH_KNOTS((6,1,1,1,1,1,1,1,1,1,1,1,1,1,1,1,1,1,1,1,1,
1,1,1,1,1,1,1,1,1,1,1,1,1,1,1,1,1,1,1,1,1,1,1,1,1,1,1,1,1,1,1,1,1,1,1,1,
1,1,1,1,1,1,1,1,6),(2,2),(-1.,-0.984615384615383,-0.969230769230768,-0.953846153846152,
-0.938461538461537,-0.923076923076922,-0.907692307692306,-0.892307692307691,
-0.876923076923076,-0.86153846153846,-0.846153846153845,-0.83076923076923,
-0.815384615384614,-0.799999999999999,-0.784615384615384,-0.769230769230768,
-0.753846153846153,-0.738461538461538,-0.723076923076922,-0.707692307692307,
-0.692307692307692,-0.676923076923076,-0.661538461538461,-0.646153846153846,
-0.63076923076923,-0.615384615384615,-0.6,-0.584615384615384,-0.569230769230769,
-0.553846153846154,-0.538461538461538,-0.523076923076923,-0.507692307692308,
-0.492307692307692,-0.476923076923077,-0.461538461538462,-0.446153846153846,
-0.430769230769231,-0.415384615384615,-0.4,-0.384615384615385,-0.369230769230769,
-0.353846153846154,-0.338461538461538,-0.323076923076923,-0.307692307692308,
-0.292307692307692,-0.276923076923077,-0.261538461538462,-0.246153846153846,
-0.230769230769231,-0.215384615384615,-0.2,-0.184615384615385,-0.169230769230769,
-0.153846153846154,-0.138461538461538,-0.123076923076923,-0.107692307692308,
-0.0923076923076923,-0.0769230769230769,-0.0615384615384615,-0.0461538461538462,
-0.0307692307692308,-0.0153846153846154,0.),(-1.,1.),.UNSPECIFIED.)
GEOMETRIC_REPRESENTATION_ITEM()
RATIONAL_B_SPLINE_SURFACE(((1.,1.),(1.,1.),(1.,1.),(1.,1.),(1.,1.),(1.,
1.),(1.,1.),(1.,1.),(1.,1.),(1.,1.),(1.,1.),(1.,1.),(1.,1.),(1.,1.),(1.,
1.),(1.,1.),(1.,1.),(1.,1.),(1.,1.),(1.,1.),(1.,1.),(1.,1.),(1.,1.),(1.,
1.),(1.,1.),(1.,1.),(1.,1.),(1.,1.),(1.,1.),(1.,1.),(1.,1.),(1.,1.),(1.,
1.),(1.,1.),(1.,1.),(1.,1.),(1.,1.),(1.,1.),(1.,1.),(1.,1.),(1.,1.),(1.,
1.),(1.,1.),(1.,1.),(1.,1.),(1.,1.),(1.,1.),(1.,1.),(1.,1.),(1.,1.),(1.,
1.),(1.,1.),(1.,1.),(1.,1.),(1.,1.),(1.,1.),(1.,1.),(1.,1.),(1.,1.),(1.,
1.),(1.,1.),(1.,1.),(1.,1.),(1.,1.),(1.,1.),(1.,1.),(1.,1.),(1.,1.),(1.,
1.),(1.,1.)))
REPRESENTATION_ITEM('')
SURFACE()
);
#132=(
BOUNDED_SURFACE()
B_SPLINE_SURFACE(5,1,((#64537,#64538),(#64539,#64540),(#64541,#64542),(#64543,
#64544),(#64545,#64546),(#64547,#64548),(#64549,#64550),(#64551,#64552),
(#64553,#64554),(#64555,#64556),(#64557,#64558),(#64559,#64560),(#64561,
#64562),(#64563,#64564),(#64565,#64566),(#64567,#64568),(#64569,#64570),
(#64571,#64572),(#64573,#64574),(#64575,#64576),(#64577,#64578),(#64579,
#64580),(#64581,#64582),(#64583,#64584),(#64585,#64586),(#64587,#64588),
(#64589,#64590),(#64591,#64592),(#64593,#64594),(#64595,#64596),(#64597,
#64598),(#64599,#64600),(#64601,#64602),(#64603,#64604),(#64605,#64606),
(#64607,#64608),(#64609,#64610),(#64611,#64612),(#64613,#64614),(#64615,
#64616),(#64617,#64618),(#64619,#64620),(#64621,#64622),(#64623,#64624),
(#64625,#64626),(#64627,#64628),(#64629,#64630),(#64631,#64632),(#64633,
#64634),(#64635,#64636),(#64637,#64638),(#64639,#64640),(#64641,#64642),
(#64643,#64644),(#64645,#64646),(#64647,#64648),(#64649,#64650),(#64651,
#64652),(#64653,#64654),(#64655,#64656),(#64657,#64658),(#64659,#64660),
(#64661,#64662),(#64663,#64664),(#64665,#64666),(#64667,#64668),(#64669,
#64670),(#64671,#64672),(#64673,#64674),(#64675,#64676)),.UNSPECIFIED.,
 .F.,.F.,.F.)
B_SPLINE_SURFACE_WITH_KNOTS((6,1,1,1,1,1,1,1,1,1,1,1,1,1,1,1,1,1,1,1,1,
1,1,1,1,1,1,1,1,1,1,1,1,1,1,1,1,1,1,1,1,1,1,1,1,1,1,1,1,1,1,1,1,1,1,1,1,
1,1,1,1,1,1,1,1,6),(2,2),(-1.,-0.984615384615383,-0.969230769230768,-0.953846153846152,
-0.938461538461537,-0.923076923076922,-0.907692307692306,-0.892307692307691,
-0.876923076923076,-0.86153846153846,-0.846153846153845,-0.83076923076923,
-0.815384615384614,-0.799999999999999,-0.784615384615384,-0.769230769230768,
-0.753846153846153,-0.738461538461538,-0.723076923076922,-0.707692307692307,
-0.692307692307692,-0.676923076923076,-0.661538461538461,-0.646153846153846,
-0.63076923076923,-0.615384615384615,-0.6,-0.584615384615384,-0.569230769230769,
-0.553846153846154,-0.538461538461538,-0.523076923076923,-0.507692307692308,
-0.492307692307692,-0.476923076923077,-0.461538461538462,-0.446153846153846,
-0.430769230769231,-0.415384615384615,-0.4,-0.384615384615385,-0.369230769230769,
-0.353846153846154,-0.338461538461538,-0.323076923076923,-0.307692307692308,
-0.292307692307692,-0.276923076923077,-0.261538461538462,-0.246153846153846,
-0.230769230769231,-0.215384615384615,-0.2,-0.184615384615385,-0.169230769230769,
-0.153846153846154,-0.138461538461538,-0.123076923076923,-0.107692307692308,
-0.0923076923076923,-0.0769230769230769,-0.0615384615384615,-0.0461538461538462,
-0.0307692307692308,-0.0153846153846154,0.),(-1.,1.),.UNSPECIFIED.)
GEOMETRIC_REPRESENTATION_ITEM()
RATIONAL_B_SPLINE_SURFACE(((1.,1.),(1.,1.),(1.,1.),(1.,1.),(1.,1.),(1.,
1.),(1.,1.),(1.,1.),(1.,1.),(1.,1.),(1.,1.),(1.,1.),(1.,1.),(1.,1.),(1.,
1.),(1.,1.),(1.,1.),(1.,1.),(1.,1.),(1.,1.),(1.,1.),(1.,1.),(1.,1.),(1.,
1.),(1.,1.),(1.,1.),(1.,1.),(1.,1.),(1.,1.),(1.,1.),(1.,1.),(1.,1.),(1.,
1.),(1.,1.),(1.,1.),(1.,1.),(1.,1.),(1.,1.),(1.,1.),(1.,1.),(1.,1.),(1.,
1.),(1.,1.),(1.,1.),(1.,1.),(1.,1.),(1.,1.),(1.,1.),(1.,1.),(1.,1.),(1.,
1.),(1.,1.),(1.,1.),(1.,1.),(1.,1.),(1.,1.),(1.,1.),(1.,1.),(1.,1.),(1.,
1.),(1.,1.),(1.,1.),(1.,1.),(1.,1.),(1.,1.),(1.,1.),(1.,1.),(1.,1.),(1.,
1.),(1.,1.)))
REPRESENTATION_ITEM('')
SURFACE()
);
#133=(
BOUNDED_SURFACE()
B_SPLINE_SURFACE(5,1,((#64767,#64768),(#64769,#64770),(#64771,#64772),(#64773,
#64774),(#64775,#64776),(#64777,#64778),(#64779,#64780),(#64781,#64782),
(#64783,#64784),(#64785,#64786),(#64787,#64788),(#64789,#64790),(#64791,
#64792),(#64793,#64794),(#64795,#64796),(#64797,#64798),(#64799,#64800),
(#64801,#64802),(#64803,#64804),(#64805,#64806),(#64807,#64808),(#64809,
#64810),(#64811,#64812),(#64813,#64814),(#64815,#64816),(#64817,#64818),
(#64819,#64820),(#64821,#64822),(#64823,#64824),(#64825,#64826),(#64827,
#64828),(#64829,#64830),(#64831,#64832),(#64833,#64834),(#64835,#64836),
(#64837,#64838),(#64839,#64840),(#64841,#64842),(#64843,#64844),(#64845,
#64846),(#64847,#64848),(#64849,#64850),(#64851,#64852),(#64853,#64854),
(#64855,#64856),(#64857,#64858),(#64859,#64860),(#64861,#64862),(#64863,
#64864),(#64865,#64866),(#64867,#64868),(#64869,#64870),(#64871,#64872),
(#64873,#64874),(#64875,#64876),(#64877,#64878),(#64879,#64880),(#64881,
#64882),(#64883,#64884),(#64885,#64886),(#64887,#64888),(#64889,#64890),
(#64891,#64892),(#64893,#64894),(#64895,#64896),(#64897,#64898),(#64899,
#64900),(#64901,#64902),(#64903,#64904),(#64905,#64906)),.UNSPECIFIED.,
 .F.,.F.,.F.)
B_SPLINE_SURFACE_WITH_KNOTS((6,1,1,1,1,1,1,1,1,1,1,1,1,1,1,1,1,1,1,1,1,
1,1,1,1,1,1,1,1,1,1,1,1,1,1,1,1,1,1,1,1,1,1,1,1,1,1,1,1,1,1,1,1,1,1,1,1,
1,1,1,1,1,1,1,1,6),(2,2),(-1.,-0.984615384615383,-0.969230769230768,-0.953846153846152,
-0.938461538461537,-0.923076923076922,-0.907692307692306,-0.892307692307691,
-0.876923076923076,-0.86153846153846,-0.846153846153845,-0.83076923076923,
-0.815384615384614,-0.799999999999999,-0.784615384615384,-0.769230769230768,
-0.753846153846153,-0.738461538461538,-0.723076923076922,-0.707692307692307,
-0.692307692307692,-0.676923076923076,-0.661538461538461,-0.646153846153846,
-0.63076923076923,-0.615384615384615,-0.6,-0.584615384615384,-0.569230769230769,
-0.553846153846154,-0.538461538461538,-0.523076923076923,-0.507692307692308,
-0.492307692307692,-0.476923076923077,-0.461538461538462,-0.446153846153846,
-0.430769230769231,-0.415384615384615,-0.4,-0.384615384615385,-0.369230769230769,
-0.353846153846154,-0.338461538461538,-0.323076923076923,-0.307692307692308,
-0.292307692307692,-0.276923076923077,-0.261538461538462,-0.246153846153846,
-0.230769230769231,-0.215384615384615,-0.2,-0.184615384615385,-0.169230769230769,
-0.153846153846154,-0.138461538461538,-0.123076923076923,-0.107692307692308,
-0.0923076923076923,-0.0769230769230769,-0.0615384615384615,-0.0461538461538462,
-0.0307692307692308,-0.0153846153846154,0.),(-1.,1.),.UNSPECIFIED.)
GEOMETRIC_REPRESENTATION_ITEM()
RATIONAL_B_SPLINE_SURFACE(((1.,1.),(1.,1.),(1.,1.),(1.,1.),(1.,1.),(1.,
1.),(1.,1.),(1.,1.),(1.,1.),(1.,1.),(1.,1.),(1.,1.),(1.,1.),(1.,1.),(1.,
1.),(1.,1.),(1.,1.),(1.,1.),(1.,1.),(1.,1.),(1.,1.),(1.,1.),(1.,1.),(1.,
1.),(1.,1.),(1.,1.),(1.,1.),(1.,1.),(1.,1.),(1.,1.),(1.,1.),(1.,1.),(1.,
1.),(1.,1.),(1.,1.),(1.,1.),(1.,1.),(1.,1.),(1.,1.),(1.,1.),(1.,1.),(1.,
1.),(1.,1.),(1.,1.),(1.,1.),(1.,1.),(1.,1.),(1.,1.),(1.,1.),(1.,1.),(1.,
1.),(1.,1.),(1.,1.),(1.,1.),(1.,1.),(1.,1.),(1.,1.),(1.,1.),(1.,1.),(1.,
1.),(1.,1.),(1.,1.),(1.,1.),(1.,1.),(1.,1.),(1.,1.),(1.,1.),(1.,1.),(1.,
1.),(1.,1.)))
REPRESENTATION_ITEM('')
SURFACE()
);
#134=(
BOUNDED_SURFACE()
B_SPLINE_SURFACE(5,1,((#64979,#64980),(#64981,#64982),(#64983,#64984),(#64985,
#64986),(#64987,#64988),(#64989,#64990),(#64991,#64992),(#64993,#64994),
(#64995,#64996),(#64997,#64998),(#64999,#65000),(#65001,#65002),(#65003,
#65004),(#65005,#65006),(#65007,#65008),(#65009,#65010),(#65011,#65012),
(#65013,#65014),(#65015,#65016),(#65017,#65018),(#65019,#65020),(#65021,
#65022),(#65023,#65024),(#65025,#65026),(#65027,#65028),(#65029,#65030),
(#65031,#65032),(#65033,#65034),(#65035,#65036),(#65037,#65038),(#65039,
#65040),(#65041,#65042),(#65043,#65044),(#65045,#65046),(#65047,#65048),
(#65049,#65050),(#65051,#65052),(#65053,#65054),(#65055,#65056),(#65057,
#65058),(#65059,#65060),(#65061,#65062),(#65063,#65064),(#65065,#65066),
(#65067,#65068),(#65069,#65070),(#65071,#65072),(#65073,#65074),(#65075,
#65076),(#65077,#65078),(#65079,#65080),(#65081,#65082),(#65083,#65084),
(#65085,#65086),(#65087,#65088),(#65089,#65090),(#65091,#65092),(#65093,
#65094),(#65095,#65096),(#65097,#65098),(#65099,#65100),(#65101,#65102),
(#65103,#65104),(#65105,#65106),(#65107,#65108),(#65109,#65110),(#65111,
#65112),(#65113,#65114),(#65115,#65116),(#65117,#65118)),.UNSPECIFIED.,
 .F.,.F.,.F.)
B_SPLINE_SURFACE_WITH_KNOTS((6,1,1,1,1,1,1,1,1,1,1,1,1,1,1,1,1,1,1,1,1,
1,1,1,1,1,1,1,1,1,1,1,1,1,1,1,1,1,1,1,1,1,1,1,1,1,1,1,1,1,1,1,1,1,1,1,1,
1,1,1,1,1,1,1,1,6),(2,2),(-1.,-0.984615384615383,-0.969230769230768,-0.953846153846152,
-0.938461538461537,-0.923076923076922,-0.907692307692306,-0.892307692307691,
-0.876923076923076,-0.86153846153846,-0.846153846153845,-0.83076923076923,
-0.815384615384614,-0.799999999999999,-0.784615384615384,-0.769230769230768,
-0.753846153846153,-0.738461538461538,-0.723076923076922,-0.707692307692307,
-0.692307692307692,-0.676923076923076,-0.661538461538461,-0.646153846153846,
-0.63076923076923,-0.615384615384615,-0.6,-0.584615384615384,-0.569230769230769,
-0.553846153846154,-0.538461538461538,-0.523076923076923,-0.507692307692308,
-0.492307692307692,-0.476923076923077,-0.461538461538462,-0.446153846153846,
-0.430769230769231,-0.415384615384615,-0.4,-0.384615384615385,-0.369230769230769,
-0.353846153846154,-0.338461538461538,-0.323076923076923,-0.307692307692308,
-0.292307692307692,-0.276923076923077,-0.261538461538462,-0.246153846153846,
-0.230769230769231,-0.215384615384615,-0.2,-0.184615384615385,-0.169230769230769,
-0.153846153846154,-0.138461538461538,-0.123076923076923,-0.107692307692308,
-0.0923076923076923,-0.0769230769230769,-0.0615384615384615,-0.0461538461538462,
-0.0307692307692308,-0.0153846153846154,0.),(-1.,1.),.UNSPECIFIED.)
GEOMETRIC_REPRESENTATION_ITEM()
RATIONAL_B_SPLINE_SURFACE(((1.,1.),(1.,1.),(1.,1.),(1.,1.),(1.,1.),(1.,
1.),(1.,1.),(1.,1.),(1.,1.),(1.,1.),(1.,1.),(1.,1.),(1.,1.),(1.,1.),(1.,
1.),(1.,1.),(1.,1.),(1.,1.),(1.,1.),(1.,1.),(1.,1.),(1.,1.),(1.,1.),(1.,
1.),(1.,1.),(1.,1.),(1.,1.),(1.,1.),(1.,1.),(1.,1.),(1.,1.),(1.,1.),(1.,
1.),(1.,1.),(1.,1.),(1.,1.),(1.,1.),(1.,1.),(1.,1.),(1.,1.),(1.,1.),(1.,
1.),(1.,1.),(1.,1.),(1.,1.),(1.,1.),(1.,1.),(1.,1.),(1.,1.),(1.,1.),(1.,
1.),(1.,1.),(1.,1.),(1.,1.),(1.,1.),(1.,1.),(1.,1.),(1.,1.),(1.,1.),(1.,
1.),(1.,1.),(1.,1.),(1.,1.),(1.,1.),(1.,1.),(1.,1.),(1.,1.),(1.,1.),(1.,
1.),(1.,1.)))
REPRESENTATION_ITEM('')
SURFACE()
);
#135=(
BOUNDED_SURFACE()
B_SPLINE_SURFACE(5,1,((#65209,#65210),(#65211,#65212),(#65213,#65214),(#65215,
#65216),(#65217,#65218),(#65219,#65220),(#65221,#65222),(#65223,#65224),
(#65225,#65226),(#65227,#65228),(#65229,#65230),(#65231,#65232),(#65233,
#65234),(#65235,#65236),(#65237,#65238),(#65239,#65240),(#65241,#65242),
(#65243,#65244),(#65245,#65246),(#65247,#65248),(#65249,#65250),(#65251,
#65252),(#65253,#65254),(#65255,#65256),(#65257,#65258),(#65259,#65260),
(#65261,#65262),(#65263,#65264),(#65265,#65266),(#65267,#65268),(#65269,
#65270),(#65271,#65272),(#65273,#65274),(#65275,#65276),(#65277,#65278),
(#65279,#65280),(#65281,#65282),(#65283,#65284),(#65285,#65286),(#65287,
#65288),(#65289,#65290),(#65291,#65292),(#65293,#65294),(#65295,#65296),
(#65297,#65298),(#65299,#65300),(#65301,#65302),(#65303,#65304),(#65305,
#65306),(#65307,#65308),(#65309,#65310),(#65311,#65312),(#65313,#65314),
(#65315,#65316),(#65317,#65318),(#65319,#65320),(#65321,#65322),(#65323,
#65324),(#65325,#65326),(#65327,#65328),(#65329,#65330),(#65331,#65332),
(#65333,#65334),(#65335,#65336),(#65337,#65338),(#65339,#65340),(#65341,
#65342),(#65343,#65344),(#65345,#65346),(#65347,#65348)),.UNSPECIFIED.,
 .F.,.F.,.F.)
B_SPLINE_SURFACE_WITH_KNOTS((6,1,1,1,1,1,1,1,1,1,1,1,1,1,1,1,1,1,1,1,1,
1,1,1,1,1,1,1,1,1,1,1,1,1,1,1,1,1,1,1,1,1,1,1,1,1,1,1,1,1,1,1,1,1,1,1,1,
1,1,1,1,1,1,1,1,6),(2,2),(-1.,-0.984615384615383,-0.969230769230768,-0.953846153846152,
-0.938461538461537,-0.923076923076922,-0.907692307692306,-0.892307692307691,
-0.876923076923076,-0.86153846153846,-0.846153846153845,-0.83076923076923,
-0.815384615384614,-0.799999999999999,-0.784615384615384,-0.769230769230768,
-0.753846153846153,-0.738461538461538,-0.723076923076922,-0.707692307692307,
-0.692307692307692,-0.676923076923076,-0.661538461538461,-0.646153846153846,
-0.63076923076923,-0.615384615384615,-0.6,-0.584615384615384,-0.569230769230769,
-0.553846153846154,-0.538461538461538,-0.523076923076923,-0.507692307692308,
-0.492307692307692,-0.476923076923077,-0.461538461538462,-0.446153846153846,
-0.430769230769231,-0.415384615384615,-0.4,-0.384615384615385,-0.369230769230769,
-0.353846153846154,-0.338461538461538,-0.323076923076923,-0.307692307692308,
-0.292307692307692,-0.276923076923077,-0.261538461538462,-0.246153846153846,
-0.230769230769231,-0.215384615384615,-0.2,-0.184615384615385,-0.169230769230769,
-0.153846153846154,-0.138461538461538,-0.123076923076923,-0.107692307692308,
-0.0923076923076923,-0.0769230769230769,-0.0615384615384615,-0.0461538461538462,
-0.0307692307692308,-0.0153846153846154,0.),(-1.,1.),.UNSPECIFIED.)
GEOMETRIC_REPRESENTATION_ITEM()
RATIONAL_B_SPLINE_SURFACE(((1.,1.),(1.,1.),(1.,1.),(1.,1.),(1.,1.),(1.,
1.),(1.,1.),(1.,1.),(1.,1.),(1.,1.),(1.,1.),(1.,1.),(1.,1.),(1.,1.),(1.,
1.),(1.,1.),(1.,1.),(1.,1.),(1.,1.),(1.,1.),(1.,1.),(1.,1.),(1.,1.),(1.,
1.),(1.,1.),(1.,1.),(1.,1.),(1.,1.),(1.,1.),(1.,1.),(1.,1.),(1.,1.),(1.,
1.),(1.,1.),(1.,1.),(1.,1.),(1.,1.),(1.,1.),(1.,1.),(1.,1.),(1.,1.),(1.,
1.),(1.,1.),(1.,1.),(1.,1.),(1.,1.),(1.,1.),(1.,1.),(1.,1.),(1.,1.),(1.,
1.),(1.,1.),(1.,1.),(1.,1.),(1.,1.),(1.,1.),(1.,1.),(1.,1.),(1.,1.),(1.,
1.),(1.,1.),(1.,1.),(1.,1.),(1.,1.),(1.,1.),(1.,1.),(1.,1.),(1.,1.),(1.,
1.),(1.,1.)))
REPRESENTATION_ITEM('')
SURFACE()
);
#136=(
BOUNDED_SURFACE()
B_SPLINE_SURFACE(5,1,((#65421,#65422),(#65423,#65424),(#65425,#65426),(#65427,
#65428),(#65429,#65430),(#65431,#65432),(#65433,#65434),(#65435,#65436),
(#65437,#65438),(#65439,#65440),(#65441,#65442),(#65443,#65444),(#65445,
#65446),(#65447,#65448),(#65449,#65450),(#65451,#65452),(#65453,#65454),
(#65455,#65456),(#65457,#65458),(#65459,#65460),(#65461,#65462),(#65463,
#65464),(#65465,#65466),(#65467,#65468),(#65469,#65470),(#65471,#65472),
(#65473,#65474),(#65475,#65476),(#65477,#65478),(#65479,#65480),(#65481,
#65482),(#65483,#65484),(#65485,#65486),(#65487,#65488),(#65489,#65490),
(#65491,#65492),(#65493,#65494),(#65495,#65496),(#65497,#65498),(#65499,
#65500),(#65501,#65502),(#65503,#65504),(#65505,#65506),(#65507,#65508),
(#65509,#65510),(#65511,#65512),(#65513,#65514),(#65515,#65516),(#65517,
#65518),(#65519,#65520),(#65521,#65522),(#65523,#65524),(#65525,#65526),
(#65527,#65528),(#65529,#65530),(#65531,#65532),(#65533,#65534),(#65535,
#65536),(#65537,#65538),(#65539,#65540),(#65541,#65542),(#65543,#65544),
(#65545,#65546),(#65547,#65548),(#65549,#65550),(#65551,#65552),(#65553,
#65554),(#65555,#65556),(#65557,#65558),(#65559,#65560)),.UNSPECIFIED.,
 .F.,.F.,.F.)
B_SPLINE_SURFACE_WITH_KNOTS((6,1,1,1,1,1,1,1,1,1,1,1,1,1,1,1,1,1,1,1,1,
1,1,1,1,1,1,1,1,1,1,1,1,1,1,1,1,1,1,1,1,1,1,1,1,1,1,1,1,1,1,1,1,1,1,1,1,
1,1,1,1,1,1,1,1,6),(2,2),(-1.,-0.984615384615383,-0.969230769230768,-0.953846153846152,
-0.938461538461537,-0.923076923076922,-0.907692307692306,-0.892307692307691,
-0.876923076923076,-0.86153846153846,-0.846153846153845,-0.83076923076923,
-0.815384615384614,-0.799999999999999,-0.784615384615384,-0.769230769230768,
-0.753846153846153,-0.738461538461538,-0.723076923076922,-0.707692307692307,
-0.692307692307692,-0.676923076923076,-0.661538461538461,-0.646153846153846,
-0.63076923076923,-0.615384615384615,-0.6,-0.584615384615384,-0.569230769230769,
-0.553846153846154,-0.538461538461538,-0.523076923076923,-0.507692307692308,
-0.492307692307692,-0.476923076923077,-0.461538461538462,-0.446153846153846,
-0.430769230769231,-0.415384615384615,-0.4,-0.384615384615385,-0.369230769230769,
-0.353846153846154,-0.338461538461538,-0.323076923076923,-0.307692307692308,
-0.292307692307692,-0.276923076923077,-0.261538461538462,-0.246153846153846,
-0.230769230769231,-0.215384615384615,-0.2,-0.184615384615385,-0.169230769230769,
-0.153846153846154,-0.138461538461538,-0.123076923076923,-0.107692307692308,
-0.0923076923076923,-0.0769230769230769,-0.0615384615384615,-0.0461538461538462,
-0.0307692307692308,-0.0153846153846154,0.),(-1.,1.),.UNSPECIFIED.)
GEOMETRIC_REPRESENTATION_ITEM()
RATIONAL_B_SPLINE_SURFACE(((1.,1.),(1.,1.),(1.,1.),(1.,1.),(1.,1.),(1.,
1.),(1.,1.),(1.,1.),(1.,1.),(1.,1.),(1.,1.),(1.,1.),(1.,1.),(1.,1.),(1.,
1.),(1.,1.),(1.,1.),(1.,1.),(1.,1.),(1.,1.),(1.,1.),(1.,1.),(1.,1.),(1.,
1.),(1.,1.),(1.,1.),(1.,1.),(1.,1.),(1.,1.),(1.,1.),(1.,1.),(1.,1.),(1.,
1.),(1.,1.),(1.,1.),(1.,1.),(1.,1.),(1.,1.),(1.,1.),(1.,1.),(1.,1.),(1.,
1.),(1.,1.),(1.,1.),(1.,1.),(1.,1.),(1.,1.),(1.,1.),(1.,1.),(1.,1.),(1.,
1.),(1.,1.),(1.,1.),(1.,1.),(1.,1.),(1.,1.),(1.,1.),(1.,1.),(1.,1.),(1.,
1.),(1.,1.),(1.,1.),(1.,1.),(1.,1.),(1.,1.),(1.,1.),(1.,1.),(1.,1.),(1.,
1.),(1.,1.)))
REPRESENTATION_ITEM('')
SURFACE()
);
#137=(
BOUNDED_SURFACE()
B_SPLINE_SURFACE(5,1,((#65651,#65652),(#65653,#65654),(#65655,#65656),(#65657,
#65658),(#65659,#65660),(#65661,#65662),(#65663,#65664),(#65665,#65666),
(#65667,#65668),(#65669,#65670),(#65671,#65672),(#65673,#65674),(#65675,
#65676),(#65677,#65678),(#65679,#65680),(#65681,#65682),(#65683,#65684),
(#65685,#65686),(#65687,#65688),(#65689,#65690),(#65691,#65692),(#65693,
#65694),(#65695,#65696),(#65697,#65698),(#65699,#65700),(#65701,#65702),
(#65703,#65704),(#65705,#65706),(#65707,#65708),(#65709,#65710),(#65711,
#65712),(#65713,#65714),(#65715,#65716),(#65717,#65718),(#65719,#65720),
(#65721,#65722),(#65723,#65724),(#65725,#65726),(#65727,#65728),(#65729,
#65730),(#65731,#65732),(#65733,#65734),(#65735,#65736),(#65737,#65738),
(#65739,#65740),(#65741,#65742),(#65743,#65744),(#65745,#65746),(#65747,
#65748),(#65749,#65750),(#65751,#65752),(#65753,#65754),(#65755,#65756),
(#65757,#65758),(#65759,#65760),(#65761,#65762),(#65763,#65764),(#65765,
#65766),(#65767,#65768),(#65769,#65770),(#65771,#65772),(#65773,#65774),
(#65775,#65776),(#65777,#65778),(#65779,#65780),(#65781,#65782),(#65783,
#65784),(#65785,#65786),(#65787,#65788),(#65789,#65790)),.UNSPECIFIED.,
 .F.,.F.,.F.)
B_SPLINE_SURFACE_WITH_KNOTS((6,1,1,1,1,1,1,1,1,1,1,1,1,1,1,1,1,1,1,1,1,
1,1,1,1,1,1,1,1,1,1,1,1,1,1,1,1,1,1,1,1,1,1,1,1,1,1,1,1,1,1,1,1,1,1,1,1,
1,1,1,1,1,1,1,1,6),(2,2),(-1.,-0.984615384615383,-0.969230769230768,-0.953846153846152,
-0.938461538461537,-0.923076923076922,-0.907692307692306,-0.892307692307691,
-0.876923076923076,-0.86153846153846,-0.846153846153845,-0.83076923076923,
-0.815384615384614,-0.799999999999999,-0.784615384615384,-0.769230769230768,
-0.753846153846153,-0.738461538461538,-0.723076923076922,-0.707692307692307,
-0.692307692307692,-0.676923076923076,-0.661538461538461,-0.646153846153846,
-0.63076923076923,-0.615384615384615,-0.6,-0.584615384615384,-0.569230769230769,
-0.553846153846154,-0.538461538461538,-0.523076923076923,-0.507692307692308,
-0.492307692307692,-0.476923076923077,-0.461538461538462,-0.446153846153846,
-0.430769230769231,-0.415384615384615,-0.4,-0.384615384615385,-0.369230769230769,
-0.353846153846154,-0.338461538461538,-0.323076923076923,-0.307692307692308,
-0.292307692307692,-0.276923076923077,-0.261538461538462,-0.246153846153846,
-0.230769230769231,-0.215384615384615,-0.2,-0.184615384615385,-0.169230769230769,
-0.153846153846154,-0.138461538461538,-0.123076923076923,-0.107692307692308,
-0.0923076923076923,-0.0769230769230769,-0.0615384615384615,-0.0461538461538462,
-0.0307692307692308,-0.0153846153846154,0.),(-1.,1.),.UNSPECIFIED.)
GEOMETRIC_REPRESENTATION_ITEM()
RATIONAL_B_SPLINE_SURFACE(((1.,1.),(1.,1.),(1.,1.),(1.,1.),(1.,1.),(1.,
1.),(1.,1.),(1.,1.),(1.,1.),(1.,1.),(1.,1.),(1.,1.),(1.,1.),(1.,1.),(1.,
1.),(1.,1.),(1.,1.),(1.,1.),(1.,1.),(1.,1.),(1.,1.),(1.,1.),(1.,1.),(1.,
1.),(1.,1.),(1.,1.),(1.,1.),(1.,1.),(1.,1.),(1.,1.),(1.,1.),(1.,1.),(1.,
1.),(1.,1.),(1.,1.),(1.,1.),(1.,1.),(1.,1.),(1.,1.),(1.,1.),(1.,1.),(1.,
1.),(1.,1.),(1.,1.),(1.,1.),(1.,1.),(1.,1.),(1.,1.),(1.,1.),(1.,1.),(1.,
1.),(1.,1.),(1.,1.),(1.,1.),(1.,1.),(1.,1.),(1.,1.),(1.,1.),(1.,1.),(1.,
1.),(1.,1.),(1.,1.),(1.,1.),(1.,1.),(1.,1.),(1.,1.),(1.,1.),(1.,1.),(1.,
1.),(1.,1.)))
REPRESENTATION_ITEM('')
SURFACE()
);
#138=(
BOUNDED_SURFACE()
B_SPLINE_SURFACE(5,1,((#65863,#65864),(#65865,#65866),(#65867,#65868),(#65869,
#65870),(#65871,#65872),(#65873,#65874),(#65875,#65876),(#65877,#65878),
(#65879,#65880),(#65881,#65882),(#65883,#65884),(#65885,#65886),(#65887,
#65888),(#65889,#65890),(#65891,#65892),(#65893,#65894),(#65895,#65896),
(#65897,#65898),(#65899,#65900),(#65901,#65902),(#65903,#65904),(#65905,
#65906),(#65907,#65908),(#65909,#65910),(#65911,#65912),(#65913,#65914),
(#65915,#65916),(#65917,#65918),(#65919,#65920),(#65921,#65922),(#65923,
#65924),(#65925,#65926),(#65927,#65928),(#65929,#65930),(#65931,#65932),
(#65933,#65934),(#65935,#65936),(#65937,#65938),(#65939,#65940),(#65941,
#65942),(#65943,#65944),(#65945,#65946),(#65947,#65948),(#65949,#65950),
(#65951,#65952),(#65953,#65954),(#65955,#65956),(#65957,#65958),(#65959,
#65960),(#65961,#65962),(#65963,#65964),(#65965,#65966),(#65967,#65968),
(#65969,#65970),(#65971,#65972),(#65973,#65974),(#65975,#65976),(#65977,
#65978),(#65979,#65980),(#65981,#65982),(#65983,#65984),(#65985,#65986),
(#65987,#65988),(#65989,#65990),(#65991,#65992),(#65993,#65994),(#65995,
#65996),(#65997,#65998),(#65999,#66000),(#66001,#66002)),.UNSPECIFIED.,
 .F.,.F.,.F.)
B_SPLINE_SURFACE_WITH_KNOTS((6,1,1,1,1,1,1,1,1,1,1,1,1,1,1,1,1,1,1,1,1,
1,1,1,1,1,1,1,1,1,1,1,1,1,1,1,1,1,1,1,1,1,1,1,1,1,1,1,1,1,1,1,1,1,1,1,1,
1,1,1,1,1,1,1,1,6),(2,2),(-1.,-0.984615384615383,-0.969230769230768,-0.953846153846152,
-0.938461538461537,-0.923076923076922,-0.907692307692306,-0.892307692307691,
-0.876923076923076,-0.86153846153846,-0.846153846153845,-0.83076923076923,
-0.815384615384614,-0.799999999999999,-0.784615384615384,-0.769230769230768,
-0.753846153846153,-0.738461538461538,-0.723076923076922,-0.707692307692307,
-0.692307692307692,-0.676923076923076,-0.661538461538461,-0.646153846153846,
-0.63076923076923,-0.615384615384615,-0.6,-0.584615384615384,-0.569230769230769,
-0.553846153846154,-0.538461538461538,-0.523076923076923,-0.507692307692308,
-0.492307692307692,-0.476923076923077,-0.461538461538462,-0.446153846153846,
-0.430769230769231,-0.415384615384615,-0.4,-0.384615384615385,-0.369230769230769,
-0.353846153846154,-0.338461538461538,-0.323076923076923,-0.307692307692308,
-0.292307692307692,-0.276923076923077,-0.261538461538462,-0.246153846153846,
-0.230769230769231,-0.215384615384615,-0.2,-0.184615384615385,-0.169230769230769,
-0.153846153846154,-0.138461538461538,-0.123076923076923,-0.107692307692308,
-0.0923076923076923,-0.0769230769230769,-0.0615384615384615,-0.0461538461538462,
-0.0307692307692308,-0.0153846153846154,0.),(-1.,1.),.UNSPECIFIED.)
GEOMETRIC_REPRESENTATION_ITEM()
RATIONAL_B_SPLINE_SURFACE(((1.,1.),(1.,1.),(1.,1.),(1.,1.),(1.,1.),(1.,
1.),(1.,1.),(1.,1.),(1.,1.),(1.,1.),(1.,1.),(1.,1.),(1.,1.),(1.,1.),(1.,
1.),(1.,1.),(1.,1.),(1.,1.),(1.,1.),(1.,1.),(1.,1.),(1.,1.),(1.,1.),(1.,
1.),(1.,1.),(1.,1.),(1.,1.),(1.,1.),(1.,1.),(1.,1.),(1.,1.),(1.,1.),(1.,
1.),(1.,1.),(1.,1.),(1.,1.),(1.,1.),(1.,1.),(1.,1.),(1.,1.),(1.,1.),(1.,
1.),(1.,1.),(1.,1.),(1.,1.),(1.,1.),(1.,1.),(1.,1.),(1.,1.),(1.,1.),(1.,
1.),(1.,1.),(1.,1.),(1.,1.),(1.,1.),(1.,1.),(1.,1.),(1.,1.),(1.,1.),(1.,
1.),(1.,1.),(1.,1.),(1.,1.),(1.,1.),(1.,1.),(1.,1.),(1.,1.),(1.,1.),(1.,
1.),(1.,1.)))
REPRESENTATION_ITEM('')
SURFACE()
);
#139=(
BOUNDED_SURFACE()
B_SPLINE_SURFACE(5,1,((#66093,#66094),(#66095,#66096),(#66097,#66098),(#66099,
#66100),(#66101,#66102),(#66103,#66104),(#66105,#66106),(#66107,#66108),
(#66109,#66110),(#66111,#66112),(#66113,#66114),(#66115,#66116),(#66117,
#66118),(#66119,#66120),(#66121,#66122),(#66123,#66124),(#66125,#66126),
(#66127,#66128),(#66129,#66130),(#66131,#66132),(#66133,#66134),(#66135,
#66136),(#66137,#66138),(#66139,#66140),(#66141,#66142),(#66143,#66144),
(#66145,#66146),(#66147,#66148),(#66149,#66150),(#66151,#66152),(#66153,
#66154),(#66155,#66156),(#66157,#66158),(#66159,#66160),(#66161,#66162),
(#66163,#66164),(#66165,#66166),(#66167,#66168),(#66169,#66170),(#66171,
#66172),(#66173,#66174),(#66175,#66176),(#66177,#66178),(#66179,#66180),
(#66181,#66182),(#66183,#66184),(#66185,#66186),(#66187,#66188),(#66189,
#66190),(#66191,#66192),(#66193,#66194),(#66195,#66196),(#66197,#66198),
(#66199,#66200),(#66201,#66202),(#66203,#66204),(#66205,#66206),(#66207,
#66208),(#66209,#66210),(#66211,#66212),(#66213,#66214),(#66215,#66216),
(#66217,#66218),(#66219,#66220),(#66221,#66222),(#66223,#66224),(#66225,
#66226),(#66227,#66228),(#66229,#66230),(#66231,#66232)),.UNSPECIFIED.,
 .F.,.F.,.F.)
B_SPLINE_SURFACE_WITH_KNOTS((6,1,1,1,1,1,1,1,1,1,1,1,1,1,1,1,1,1,1,1,1,
1,1,1,1,1,1,1,1,1,1,1,1,1,1,1,1,1,1,1,1,1,1,1,1,1,1,1,1,1,1,1,1,1,1,1,1,
1,1,1,1,1,1,1,1,6),(2,2),(-1.,-0.984615384615383,-0.969230769230768,-0.953846153846152,
-0.938461538461537,-0.923076923076922,-0.907692307692306,-0.892307692307691,
-0.876923076923076,-0.86153846153846,-0.846153846153845,-0.83076923076923,
-0.815384615384614,-0.799999999999999,-0.784615384615384,-0.769230769230768,
-0.753846153846153,-0.738461538461538,-0.723076923076922,-0.707692307692307,
-0.692307692307692,-0.676923076923076,-0.661538461538461,-0.646153846153846,
-0.63076923076923,-0.615384615384615,-0.6,-0.584615384615384,-0.569230769230769,
-0.553846153846154,-0.538461538461538,-0.523076923076923,-0.507692307692308,
-0.492307692307692,-0.476923076923077,-0.461538461538462,-0.446153846153846,
-0.430769230769231,-0.415384615384615,-0.4,-0.384615384615385,-0.369230769230769,
-0.353846153846154,-0.338461538461538,-0.323076923076923,-0.307692307692308,
-0.292307692307692,-0.276923076923077,-0.261538461538462,-0.246153846153846,
-0.230769230769231,-0.215384615384615,-0.2,-0.184615384615385,-0.169230769230769,
-0.153846153846154,-0.138461538461538,-0.123076923076923,-0.107692307692308,
-0.0923076923076923,-0.0769230769230769,-0.0615384615384615,-0.0461538461538462,
-0.0307692307692308,-0.0153846153846154,0.),(-1.,1.),.UNSPECIFIED.)
GEOMETRIC_REPRESENTATION_ITEM()
RATIONAL_B_SPLINE_SURFACE(((1.,1.),(1.,1.),(1.,1.),(1.,1.),(1.,1.),(1.,
1.),(1.,1.),(1.,1.),(1.,1.),(1.,1.),(1.,1.),(1.,1.),(1.,1.),(1.,1.),(1.,
1.),(1.,1.),(1.,1.),(1.,1.),(1.,1.),(1.,1.),(1.,1.),(1.,1.),(1.,1.),(1.,
1.),(1.,1.),(1.,1.),(1.,1.),(1.,1.),(1.,1.),(1.,1.),(1.,1.),(1.,1.),(1.,
1.),(1.,1.),(1.,1.),(1.,1.),(1.,1.),(1.,1.),(1.,1.),(1.,1.),(1.,1.),(1.,
1.),(1.,1.),(1.,1.),(1.,1.),(1.,1.),(1.,1.),(1.,1.),(1.,1.),(1.,1.),(1.,
1.),(1.,1.),(1.,1.),(1.,1.),(1.,1.),(1.,1.),(1.,1.),(1.,1.),(1.,1.),(1.,
1.),(1.,1.),(1.,1.),(1.,1.),(1.,1.),(1.,1.),(1.,1.),(1.,1.),(1.,1.),(1.,
1.),(1.,1.)))
REPRESENTATION_ITEM('')
SURFACE()
);
#140=(
BOUNDED_SURFACE()
B_SPLINE_SURFACE(5,1,((#66305,#66306),(#66307,#66308),(#66309,#66310),(#66311,
#66312),(#66313,#66314),(#66315,#66316),(#66317,#66318),(#66319,#66320),
(#66321,#66322),(#66323,#66324),(#66325,#66326),(#66327,#66328),(#66329,
#66330),(#66331,#66332),(#66333,#66334),(#66335,#66336),(#66337,#66338),
(#66339,#66340),(#66341,#66342),(#66343,#66344),(#66345,#66346),(#66347,
#66348),(#66349,#66350),(#66351,#66352),(#66353,#66354),(#66355,#66356),
(#66357,#66358),(#66359,#66360),(#66361,#66362),(#66363,#66364),(#66365,
#66366),(#66367,#66368),(#66369,#66370),(#66371,#66372),(#66373,#66374),
(#66375,#66376),(#66377,#66378),(#66379,#66380),(#66381,#66382),(#66383,
#66384),(#66385,#66386),(#66387,#66388),(#66389,#66390),(#66391,#66392),
(#66393,#66394),(#66395,#66396),(#66397,#66398),(#66399,#66400),(#66401,
#66402),(#66403,#66404),(#66405,#66406),(#66407,#66408),(#66409,#66410),
(#66411,#66412),(#66413,#66414),(#66415,#66416),(#66417,#66418),(#66419,
#66420),(#66421,#66422),(#66423,#66424),(#66425,#66426),(#66427,#66428),
(#66429,#66430),(#66431,#66432),(#66433,#66434),(#66435,#66436),(#66437,
#66438),(#66439,#66440),(#66441,#66442),(#66443,#66444)),.UNSPECIFIED.,
 .F.,.F.,.F.)
B_SPLINE_SURFACE_WITH_KNOTS((6,1,1,1,1,1,1,1,1,1,1,1,1,1,1,1,1,1,1,1,1,
1,1,1,1,1,1,1,1,1,1,1,1,1,1,1,1,1,1,1,1,1,1,1,1,1,1,1,1,1,1,1,1,1,1,1,1,
1,1,1,1,1,1,1,1,6),(2,2),(-1.,-0.984615384615383,-0.969230769230768,-0.953846153846152,
-0.938461538461537,-0.923076923076922,-0.907692307692306,-0.892307692307691,
-0.876923076923076,-0.86153846153846,-0.846153846153845,-0.83076923076923,
-0.815384615384614,-0.799999999999999,-0.784615384615384,-0.769230769230768,
-0.753846153846153,-0.738461538461538,-0.723076923076922,-0.707692307692307,
-0.692307692307692,-0.676923076923076,-0.661538461538461,-0.646153846153846,
-0.63076923076923,-0.615384615384615,-0.6,-0.584615384615384,-0.569230769230769,
-0.553846153846154,-0.538461538461538,-0.523076923076923,-0.507692307692308,
-0.492307692307692,-0.476923076923077,-0.461538461538462,-0.446153846153846,
-0.430769230769231,-0.415384615384615,-0.4,-0.384615384615385,-0.369230769230769,
-0.353846153846154,-0.338461538461538,-0.323076923076923,-0.307692307692308,
-0.292307692307692,-0.276923076923077,-0.261538461538462,-0.246153846153846,
-0.230769230769231,-0.215384615384615,-0.2,-0.184615384615385,-0.169230769230769,
-0.153846153846154,-0.138461538461538,-0.123076923076923,-0.107692307692308,
-0.0923076923076923,-0.0769230769230769,-0.0615384615384615,-0.0461538461538462,
-0.0307692307692308,-0.0153846153846154,0.),(-1.,1.),.UNSPECIFIED.)
GEOMETRIC_REPRESENTATION_ITEM()
RATIONAL_B_SPLINE_SURFACE(((1.,1.),(1.,1.),(1.,1.),(1.,1.),(1.,1.),(1.,
1.),(1.,1.),(1.,1.),(1.,1.),(1.,1.),(1.,1.),(1.,1.),(1.,1.),(1.,1.),(1.,
1.),(1.,1.),(1.,1.),(1.,1.),(1.,1.),(1.,1.),(1.,1.),(1.,1.),(1.,1.),(1.,
1.),(1.,1.),(1.,1.),(1.,1.),(1.,1.),(1.,1.),(1.,1.),(1.,1.),(1.,1.),(1.,
1.),(1.,1.),(1.,1.),(1.,1.),(1.,1.),(1.,1.),(1.,1.),(1.,1.),(1.,1.),(1.,
1.),(1.,1.),(1.,1.),(1.,1.),(1.,1.),(1.,1.),(1.,1.),(1.,1.),(1.,1.),(1.,
1.),(1.,1.),(1.,1.),(1.,1.),(1.,1.),(1.,1.),(1.,1.),(1.,1.),(1.,1.),(1.,
1.),(1.,1.),(1.,1.),(1.,1.),(1.,1.),(1.,1.),(1.,1.),(1.,1.),(1.,1.),(1.,
1.),(1.,1.)))
REPRESENTATION_ITEM('')
SURFACE()
);
#141=(
BOUNDED_SURFACE()
B_SPLINE_SURFACE(5,1,((#66535,#66536),(#66537,#66538),(#66539,#66540),(#66541,
#66542),(#66543,#66544),(#66545,#66546),(#66547,#66548),(#66549,#66550),
(#66551,#66552),(#66553,#66554),(#66555,#66556),(#66557,#66558),(#66559,
#66560),(#66561,#66562),(#66563,#66564),(#66565,#66566),(#66567,#66568),
(#66569,#66570),(#66571,#66572),(#66573,#66574),(#66575,#66576),(#66577,
#66578),(#66579,#66580),(#66581,#66582),(#66583,#66584),(#66585,#66586),
(#66587,#66588),(#66589,#66590),(#66591,#66592),(#66593,#66594),(#66595,
#66596),(#66597,#66598),(#66599,#66600),(#66601,#66602),(#66603,#66604),
(#66605,#66606),(#66607,#66608),(#66609,#66610),(#66611,#66612),(#66613,
#66614),(#66615,#66616),(#66617,#66618),(#66619,#66620),(#66621,#66622),
(#66623,#66624),(#66625,#66626),(#66627,#66628),(#66629,#66630),(#66631,
#66632),(#66633,#66634),(#66635,#66636),(#66637,#66638),(#66639,#66640),
(#66641,#66642),(#66643,#66644),(#66645,#66646),(#66647,#66648),(#66649,
#66650),(#66651,#66652),(#66653,#66654),(#66655,#66656),(#66657,#66658),
(#66659,#66660),(#66661,#66662),(#66663,#66664),(#66665,#66666),(#66667,
#66668),(#66669,#66670),(#66671,#66672),(#66673,#66674)),.UNSPECIFIED.,
 .F.,.F.,.F.)
B_SPLINE_SURFACE_WITH_KNOTS((6,1,1,1,1,1,1,1,1,1,1,1,1,1,1,1,1,1,1,1,1,
1,1,1,1,1,1,1,1,1,1,1,1,1,1,1,1,1,1,1,1,1,1,1,1,1,1,1,1,1,1,1,1,1,1,1,1,
1,1,1,1,1,1,1,1,6),(2,2),(-1.,-0.984615384615383,-0.969230769230768,-0.953846153846152,
-0.938461538461537,-0.923076923076922,-0.907692307692306,-0.892307692307691,
-0.876923076923076,-0.86153846153846,-0.846153846153845,-0.83076923076923,
-0.815384615384614,-0.799999999999999,-0.784615384615384,-0.769230769230768,
-0.753846153846153,-0.738461538461538,-0.723076923076922,-0.707692307692307,
-0.692307692307692,-0.676923076923076,-0.661538461538461,-0.646153846153846,
-0.63076923076923,-0.615384615384615,-0.6,-0.584615384615384,-0.569230769230769,
-0.553846153846154,-0.538461538461538,-0.523076923076923,-0.507692307692308,
-0.492307692307692,-0.476923076923077,-0.461538461538462,-0.446153846153846,
-0.430769230769231,-0.415384615384615,-0.4,-0.384615384615385,-0.369230769230769,
-0.353846153846154,-0.338461538461538,-0.323076923076923,-0.307692307692308,
-0.292307692307692,-0.276923076923077,-0.261538461538462,-0.246153846153846,
-0.230769230769231,-0.215384615384615,-0.2,-0.184615384615385,-0.169230769230769,
-0.153846153846154,-0.138461538461538,-0.123076923076923,-0.107692307692308,
-0.0923076923076923,-0.0769230769230769,-0.0615384615384615,-0.0461538461538462,
-0.0307692307692308,-0.0153846153846154,0.),(-1.,1.),.UNSPECIFIED.)
GEOMETRIC_REPRESENTATION_ITEM()
RATIONAL_B_SPLINE_SURFACE(((1.,1.),(1.,1.),(1.,1.),(1.,1.),(1.,1.),(1.,
1.),(1.,1.),(1.,1.),(1.,1.),(1.,1.),(1.,1.),(1.,1.),(1.,1.),(1.,1.),(1.,
1.),(1.,1.),(1.,1.),(1.,1.),(1.,1.),(1.,1.),(1.,1.),(1.,1.),(1.,1.),(1.,
1.),(1.,1.),(1.,1.),(1.,1.),(1.,1.),(1.,1.),(1.,1.),(1.,1.),(1.,1.),(1.,
1.),(1.,1.),(1.,1.),(1.,1.),(1.,1.),(1.,1.),(1.,1.),(1.,1.),(1.,1.),(1.,
1.),(1.,1.),(1.,1.),(1.,1.),(1.,1.),(1.,1.),(1.,1.),(1.,1.),(1.,1.),(1.,
1.),(1.,1.),(1.,1.),(1.,1.),(1.,1.),(1.,1.),(1.,1.),(1.,1.),(1.,1.),(1.,
1.),(1.,1.),(1.,1.),(1.,1.),(1.,1.),(1.,1.),(1.,1.),(1.,1.),(1.,1.),(1.,
1.),(1.,1.)))
REPRESENTATION_ITEM('')
SURFACE()
);
#142=(
BOUNDED_SURFACE()
B_SPLINE_SURFACE(5,1,((#66747,#66748),(#66749,#66750),(#66751,#66752),(#66753,
#66754),(#66755,#66756),(#66757,#66758),(#66759,#66760),(#66761,#66762),
(#66763,#66764),(#66765,#66766),(#66767,#66768),(#66769,#66770),(#66771,
#66772),(#66773,#66774),(#66775,#66776),(#66777,#66778),(#66779,#66780),
(#66781,#66782),(#66783,#66784),(#66785,#66786),(#66787,#66788),(#66789,
#66790),(#66791,#66792),(#66793,#66794),(#66795,#66796),(#66797,#66798),
(#66799,#66800),(#66801,#66802),(#66803,#66804),(#66805,#66806),(#66807,
#66808),(#66809,#66810),(#66811,#66812),(#66813,#66814),(#66815,#66816),
(#66817,#66818),(#66819,#66820),(#66821,#66822),(#66823,#66824),(#66825,
#66826),(#66827,#66828),(#66829,#66830),(#66831,#66832),(#66833,#66834),
(#66835,#66836),(#66837,#66838),(#66839,#66840),(#66841,#66842),(#66843,
#66844),(#66845,#66846),(#66847,#66848),(#66849,#66850),(#66851,#66852),
(#66853,#66854),(#66855,#66856),(#66857,#66858),(#66859,#66860),(#66861,
#66862),(#66863,#66864),(#66865,#66866),(#66867,#66868),(#66869,#66870),
(#66871,#66872),(#66873,#66874),(#66875,#66876),(#66877,#66878),(#66879,
#66880),(#66881,#66882),(#66883,#66884),(#66885,#66886)),.UNSPECIFIED.,
 .F.,.F.,.F.)
B_SPLINE_SURFACE_WITH_KNOTS((6,1,1,1,1,1,1,1,1,1,1,1,1,1,1,1,1,1,1,1,1,
1,1,1,1,1,1,1,1,1,1,1,1,1,1,1,1,1,1,1,1,1,1,1,1,1,1,1,1,1,1,1,1,1,1,1,1,
1,1,1,1,1,1,1,1,6),(2,2),(-1.,-0.984615384615383,-0.969230769230768,-0.953846153846152,
-0.938461538461537,-0.923076923076922,-0.907692307692306,-0.892307692307691,
-0.876923076923076,-0.86153846153846,-0.846153846153845,-0.83076923076923,
-0.815384615384614,-0.799999999999999,-0.784615384615384,-0.769230769230768,
-0.753846153846153,-0.738461538461538,-0.723076923076922,-0.707692307692307,
-0.692307692307692,-0.676923076923076,-0.661538461538461,-0.646153846153846,
-0.63076923076923,-0.615384615384615,-0.6,-0.584615384615384,-0.569230769230769,
-0.553846153846154,-0.538461538461538,-0.523076923076923,-0.507692307692308,
-0.492307692307692,-0.476923076923077,-0.461538461538462,-0.446153846153846,
-0.430769230769231,-0.415384615384615,-0.4,-0.384615384615385,-0.369230769230769,
-0.353846153846154,-0.338461538461538,-0.323076923076923,-0.307692307692308,
-0.292307692307692,-0.276923076923077,-0.261538461538462,-0.246153846153846,
-0.230769230769231,-0.215384615384615,-0.2,-0.184615384615385,-0.169230769230769,
-0.153846153846154,-0.138461538461538,-0.123076923076923,-0.107692307692308,
-0.0923076923076923,-0.0769230769230769,-0.0615384615384615,-0.0461538461538462,
-0.0307692307692308,-0.0153846153846154,0.),(-1.,1.),.UNSPECIFIED.)
GEOMETRIC_REPRESENTATION_ITEM()
RATIONAL_B_SPLINE_SURFACE(((1.,1.),(1.,1.),(1.,1.),(1.,1.),(1.,1.),(1.,
1.),(1.,1.),(1.,1.),(1.,1.),(1.,1.),(1.,1.),(1.,1.),(1.,1.),(1.,1.),(1.,
1.),(1.,1.),(1.,1.),(1.,1.),(1.,1.),(1.,1.),(1.,1.),(1.,1.),(1.,1.),(1.,
1.),(1.,1.),(1.,1.),(1.,1.),(1.,1.),(1.,1.),(1.,1.),(1.,1.),(1.,1.),(1.,
1.),(1.,1.),(1.,1.),(1.,1.),(1.,1.),(1.,1.),(1.,1.),(1.,1.),(1.,1.),(1.,
1.),(1.,1.),(1.,1.),(1.,1.),(1.,1.),(1.,1.),(1.,1.),(1.,1.),(1.,1.),(1.,
1.),(1.,1.),(1.,1.),(1.,1.),(1.,1.),(1.,1.),(1.,1.),(1.,1.),(1.,1.),(1.,
1.),(1.,1.),(1.,1.),(1.,1.),(1.,1.),(1.,1.),(1.,1.),(1.,1.),(1.,1.),(1.,
1.),(1.,1.)))
REPRESENTATION_ITEM('')
SURFACE()
);
#143=(
BOUNDED_SURFACE()
B_SPLINE_SURFACE(5,1,((#66977,#66978),(#66979,#66980),(#66981,#66982),(#66983,
#66984),(#66985,#66986),(#66987,#66988),(#66989,#66990),(#66991,#66992),
(#66993,#66994),(#66995,#66996),(#66997,#66998),(#66999,#67000),(#67001,
#67002),(#67003,#67004),(#67005,#67006),(#67007,#67008),(#67009,#67010),
(#67011,#67012),(#67013,#67014),(#67015,#67016),(#67017,#67018),(#67019,
#67020),(#67021,#67022),(#67023,#67024),(#67025,#67026),(#67027,#67028),
(#67029,#67030),(#67031,#67032),(#67033,#67034),(#67035,#67036),(#67037,
#67038),(#67039,#67040),(#67041,#67042),(#67043,#67044),(#67045,#67046),
(#67047,#67048),(#67049,#67050),(#67051,#67052),(#67053,#67054),(#67055,
#67056),(#67057,#67058),(#67059,#67060),(#67061,#67062),(#67063,#67064),
(#67065,#67066),(#67067,#67068),(#67069,#67070),(#67071,#67072),(#67073,
#67074),(#67075,#67076),(#67077,#67078),(#67079,#67080),(#67081,#67082),
(#67083,#67084),(#67085,#67086),(#67087,#67088),(#67089,#67090),(#67091,
#67092),(#67093,#67094),(#67095,#67096),(#67097,#67098),(#67099,#67100),
(#67101,#67102),(#67103,#67104),(#67105,#67106),(#67107,#67108),(#67109,
#67110),(#67111,#67112),(#67113,#67114),(#67115,#67116)),.UNSPECIFIED.,
 .F.,.F.,.F.)
B_SPLINE_SURFACE_WITH_KNOTS((6,1,1,1,1,1,1,1,1,1,1,1,1,1,1,1,1,1,1,1,1,
1,1,1,1,1,1,1,1,1,1,1,1,1,1,1,1,1,1,1,1,1,1,1,1,1,1,1,1,1,1,1,1,1,1,1,1,
1,1,1,1,1,1,1,1,6),(2,2),(-1.,-0.984615384615383,-0.969230769230768,-0.953846153846152,
-0.938461538461537,-0.923076923076922,-0.907692307692306,-0.892307692307691,
-0.876923076923076,-0.86153846153846,-0.846153846153845,-0.83076923076923,
-0.815384615384614,-0.799999999999999,-0.784615384615384,-0.769230769230768,
-0.753846153846153,-0.738461538461538,-0.723076923076922,-0.707692307692307,
-0.692307692307692,-0.676923076923076,-0.661538461538461,-0.646153846153846,
-0.63076923076923,-0.615384615384615,-0.6,-0.584615384615384,-0.569230769230769,
-0.553846153846154,-0.538461538461538,-0.523076923076923,-0.507692307692308,
-0.492307692307692,-0.476923076923077,-0.461538461538462,-0.446153846153846,
-0.430769230769231,-0.415384615384615,-0.4,-0.384615384615385,-0.369230769230769,
-0.353846153846154,-0.338461538461538,-0.323076923076923,-0.307692307692308,
-0.292307692307692,-0.276923076923077,-0.261538461538462,-0.246153846153846,
-0.230769230769231,-0.215384615384615,-0.2,-0.184615384615385,-0.169230769230769,
-0.153846153846154,-0.138461538461538,-0.123076923076923,-0.107692307692308,
-0.0923076923076923,-0.0769230769230769,-0.0615384615384615,-0.0461538461538462,
-0.0307692307692308,-0.0153846153846154,0.),(-1.,1.),.UNSPECIFIED.)
GEOMETRIC_REPRESENTATION_ITEM()
RATIONAL_B_SPLINE_SURFACE(((1.,1.),(1.,1.),(1.,1.),(1.,1.),(1.,1.),(1.,
1.),(1.,1.),(1.,1.),(1.,1.),(1.,1.),(1.,1.),(1.,1.),(1.,1.),(1.,1.),(1.,
1.),(1.,1.),(1.,1.),(1.,1.),(1.,1.),(1.,1.),(1.,1.),(1.,1.),(1.,1.),(1.,
1.),(1.,1.),(1.,1.),(1.,1.),(1.,1.),(1.,1.),(1.,1.),(1.,1.),(1.,1.),(1.,
1.),(1.,1.),(1.,1.),(1.,1.),(1.,1.),(1.,1.),(1.,1.),(1.,1.),(1.,1.),(1.,
1.),(1.,1.),(1.,1.),(1.,1.),(1.,1.),(1.,1.),(1.,1.),(1.,1.),(1.,1.),(1.,
1.),(1.,1.),(1.,1.),(1.,1.),(1.,1.),(1.,1.),(1.,1.),(1.,1.),(1.,1.),(1.,
1.),(1.,1.),(1.,1.),(1.,1.),(1.,1.),(1.,1.),(1.,1.),(1.,1.),(1.,1.),(1.,
1.),(1.,1.)))
REPRESENTATION_ITEM('')
SURFACE()
);
#144=(
BOUNDED_SURFACE()
B_SPLINE_SURFACE(5,1,((#67189,#67190),(#67191,#67192),(#67193,#67194),(#67195,
#67196),(#67197,#67198),(#67199,#67200),(#67201,#67202),(#67203,#67204),
(#67205,#67206),(#67207,#67208),(#67209,#67210),(#67211,#67212),(#67213,
#67214),(#67215,#67216),(#67217,#67218),(#67219,#67220),(#67221,#67222),
(#67223,#67224),(#67225,#67226),(#67227,#67228),(#67229,#67230),(#67231,
#67232),(#67233,#67234),(#67235,#67236),(#67237,#67238),(#67239,#67240),
(#67241,#67242),(#67243,#67244),(#67245,#67246),(#67247,#67248),(#67249,
#67250),(#67251,#67252),(#67253,#67254),(#67255,#67256),(#67257,#67258),
(#67259,#67260),(#67261,#67262),(#67263,#67264),(#67265,#67266),(#67267,
#67268),(#67269,#67270),(#67271,#67272),(#67273,#67274),(#67275,#67276),
(#67277,#67278),(#67279,#67280),(#67281,#67282),(#67283,#67284),(#67285,
#67286),(#67287,#67288),(#67289,#67290),(#67291,#67292),(#67293,#67294),
(#67295,#67296),(#67297,#67298),(#67299,#67300),(#67301,#67302),(#67303,
#67304),(#67305,#67306),(#67307,#67308),(#67309,#67310),(#67311,#67312),
(#67313,#67314),(#67315,#67316),(#67317,#67318),(#67319,#67320),(#67321,
#67322),(#67323,#67324),(#67325,#67326),(#67327,#67328)),.UNSPECIFIED.,
 .F.,.F.,.F.)
B_SPLINE_SURFACE_WITH_KNOTS((6,1,1,1,1,1,1,1,1,1,1,1,1,1,1,1,1,1,1,1,1,
1,1,1,1,1,1,1,1,1,1,1,1,1,1,1,1,1,1,1,1,1,1,1,1,1,1,1,1,1,1,1,1,1,1,1,1,
1,1,1,1,1,1,1,1,6),(2,2),(-1.,-0.984615384615383,-0.969230769230768,-0.953846153846152,
-0.938461538461537,-0.923076923076922,-0.907692307692306,-0.892307692307691,
-0.876923076923076,-0.86153846153846,-0.846153846153845,-0.83076923076923,
-0.815384615384614,-0.799999999999999,-0.784615384615384,-0.769230769230768,
-0.753846153846153,-0.738461538461538,-0.723076923076922,-0.707692307692307,
-0.692307692307692,-0.676923076923076,-0.661538461538461,-0.646153846153846,
-0.63076923076923,-0.615384615384615,-0.6,-0.584615384615384,-0.569230769230769,
-0.553846153846154,-0.538461538461538,-0.523076923076923,-0.507692307692308,
-0.492307692307692,-0.476923076923077,-0.461538461538462,-0.446153846153846,
-0.430769230769231,-0.415384615384615,-0.4,-0.384615384615385,-0.369230769230769,
-0.353846153846154,-0.338461538461538,-0.323076923076923,-0.307692307692308,
-0.292307692307692,-0.276923076923077,-0.261538461538462,-0.246153846153846,
-0.230769230769231,-0.215384615384615,-0.2,-0.184615384615385,-0.169230769230769,
-0.153846153846154,-0.138461538461538,-0.123076923076923,-0.107692307692308,
-0.0923076923076923,-0.0769230769230769,-0.0615384615384615,-0.0461538461538462,
-0.0307692307692308,-0.0153846153846154,0.),(-1.,1.),.UNSPECIFIED.)
GEOMETRIC_REPRESENTATION_ITEM()
RATIONAL_B_SPLINE_SURFACE(((1.,1.),(1.,1.),(1.,1.),(1.,1.),(1.,1.),(1.,
1.),(1.,1.),(1.,1.),(1.,1.),(1.,1.),(1.,1.),(1.,1.),(1.,1.),(1.,1.),(1.,
1.),(1.,1.),(1.,1.),(1.,1.),(1.,1.),(1.,1.),(1.,1.),(1.,1.),(1.,1.),(1.,
1.),(1.,1.),(1.,1.),(1.,1.),(1.,1.),(1.,1.),(1.,1.),(1.,1.),(1.,1.),(1.,
1.),(1.,1.),(1.,1.),(1.,1.),(1.,1.),(1.,1.),(1.,1.),(1.,1.),(1.,1.),(1.,
1.),(1.,1.),(1.,1.),(1.,1.),(1.,1.),(1.,1.),(1.,1.),(1.,1.),(1.,1.),(1.,
1.),(1.,1.),(1.,1.),(1.,1.),(1.,1.),(1.,1.),(1.,1.),(1.,1.),(1.,1.),(1.,
1.),(1.,1.),(1.,1.),(1.,1.),(1.,1.),(1.,1.),(1.,1.),(1.,1.),(1.,1.),(1.,
1.),(1.,1.)))
REPRESENTATION_ITEM('')
SURFACE()
);
#145=(
BOUNDED_SURFACE()
B_SPLINE_SURFACE(5,1,((#67419,#67420),(#67421,#67422),(#67423,#67424),(#67425,
#67426),(#67427,#67428),(#67429,#67430),(#67431,#67432),(#67433,#67434),
(#67435,#67436),(#67437,#67438),(#67439,#67440),(#67441,#67442),(#67443,
#67444),(#67445,#67446),(#67447,#67448),(#67449,#67450),(#67451,#67452),
(#67453,#67454),(#67455,#67456),(#67457,#67458),(#67459,#67460),(#67461,
#67462),(#67463,#67464),(#67465,#67466),(#67467,#67468),(#67469,#67470),
(#67471,#67472),(#67473,#67474),(#67475,#67476),(#67477,#67478),(#67479,
#67480),(#67481,#67482),(#67483,#67484),(#67485,#67486),(#67487,#67488),
(#67489,#67490),(#67491,#67492),(#67493,#67494),(#67495,#67496),(#67497,
#67498),(#67499,#67500),(#67501,#67502),(#67503,#67504),(#67505,#67506),
(#67507,#67508),(#67509,#67510),(#67511,#67512),(#67513,#67514),(#67515,
#67516),(#67517,#67518),(#67519,#67520),(#67521,#67522),(#67523,#67524),
(#67525,#67526),(#67527,#67528),(#67529,#67530),(#67531,#67532),(#67533,
#67534),(#67535,#67536),(#67537,#67538),(#67539,#67540),(#67541,#67542),
(#67543,#67544),(#67545,#67546),(#67547,#67548),(#67549,#67550),(#67551,
#67552),(#67553,#67554),(#67555,#67556),(#67557,#67558)),.UNSPECIFIED.,
 .F.,.F.,.F.)
B_SPLINE_SURFACE_WITH_KNOTS((6,1,1,1,1,1,1,1,1,1,1,1,1,1,1,1,1,1,1,1,1,
1,1,1,1,1,1,1,1,1,1,1,1,1,1,1,1,1,1,1,1,1,1,1,1,1,1,1,1,1,1,1,1,1,1,1,1,
1,1,1,1,1,1,1,1,6),(2,2),(-1.,-0.984615384615383,-0.969230769230768,-0.953846153846152,
-0.938461538461537,-0.923076923076922,-0.907692307692306,-0.892307692307691,
-0.876923076923076,-0.86153846153846,-0.846153846153845,-0.83076923076923,
-0.815384615384614,-0.799999999999999,-0.784615384615384,-0.769230769230768,
-0.753846153846153,-0.738461538461538,-0.723076923076922,-0.707692307692307,
-0.692307692307692,-0.676923076923076,-0.661538461538461,-0.646153846153846,
-0.63076923076923,-0.615384615384615,-0.6,-0.584615384615384,-0.569230769230769,
-0.553846153846154,-0.538461538461538,-0.523076923076923,-0.507692307692308,
-0.492307692307692,-0.476923076923077,-0.461538461538462,-0.446153846153846,
-0.430769230769231,-0.415384615384615,-0.4,-0.384615384615385,-0.369230769230769,
-0.353846153846154,-0.338461538461538,-0.323076923076923,-0.307692307692308,
-0.292307692307692,-0.276923076923077,-0.261538461538462,-0.246153846153846,
-0.230769230769231,-0.215384615384615,-0.2,-0.184615384615385,-0.169230769230769,
-0.153846153846154,-0.138461538461538,-0.123076923076923,-0.107692307692308,
-0.0923076923076923,-0.0769230769230769,-0.0615384615384615,-0.0461538461538462,
-0.0307692307692308,-0.0153846153846154,0.),(-1.,1.),.UNSPECIFIED.)
GEOMETRIC_REPRESENTATION_ITEM()
RATIONAL_B_SPLINE_SURFACE(((1.,1.),(1.,1.),(1.,1.),(1.,1.),(1.,1.),(1.,
1.),(1.,1.),(1.,1.),(1.,1.),(1.,1.),(1.,1.),(1.,1.),(1.,1.),(1.,1.),(1.,
1.),(1.,1.),(1.,1.),(1.,1.),(1.,1.),(1.,1.),(1.,1.),(1.,1.),(1.,1.),(1.,
1.),(1.,1.),(1.,1.),(1.,1.),(1.,1.),(1.,1.),(1.,1.),(1.,1.),(1.,1.),(1.,
1.),(1.,1.),(1.,1.),(1.,1.),(1.,1.),(1.,1.),(1.,1.),(1.,1.),(1.,1.),(1.,
1.),(1.,1.),(1.,1.),(1.,1.),(1.,1.),(1.,1.),(1.,1.),(1.,1.),(1.,1.),(1.,
1.),(1.,1.),(1.,1.),(1.,1.),(1.,1.),(1.,1.),(1.,1.),(1.,1.),(1.,1.),(1.,
1.),(1.,1.),(1.,1.),(1.,1.),(1.,1.),(1.,1.),(1.,1.),(1.,1.),(1.,1.),(1.,
1.),(1.,1.)))
REPRESENTATION_ITEM('')
SURFACE()
);
#146=(
BOUNDED_SURFACE()
B_SPLINE_SURFACE(5,1,((#67631,#67632),(#67633,#67634),(#67635,#67636),(#67637,
#67638),(#67639,#67640),(#67641,#67642),(#67643,#67644),(#67645,#67646),
(#67647,#67648),(#67649,#67650),(#67651,#67652),(#67653,#67654),(#67655,
#67656),(#67657,#67658),(#67659,#67660),(#67661,#67662),(#67663,#67664),
(#67665,#67666),(#67667,#67668),(#67669,#67670),(#67671,#67672),(#67673,
#67674),(#67675,#67676),(#67677,#67678),(#67679,#67680),(#67681,#67682),
(#67683,#67684),(#67685,#67686),(#67687,#67688),(#67689,#67690),(#67691,
#67692),(#67693,#67694),(#67695,#67696),(#67697,#67698),(#67699,#67700),
(#67701,#67702),(#67703,#67704),(#67705,#67706),(#67707,#67708),(#67709,
#67710),(#67711,#67712),(#67713,#67714),(#67715,#67716),(#67717,#67718),
(#67719,#67720),(#67721,#67722),(#67723,#67724),(#67725,#67726),(#67727,
#67728),(#67729,#67730),(#67731,#67732),(#67733,#67734),(#67735,#67736),
(#67737,#67738),(#67739,#67740),(#67741,#67742),(#67743,#67744),(#67745,
#67746),(#67747,#67748),(#67749,#67750),(#67751,#67752),(#67753,#67754),
(#67755,#67756),(#67757,#67758),(#67759,#67760),(#67761,#67762),(#67763,
#67764),(#67765,#67766),(#67767,#67768),(#67769,#67770)),.UNSPECIFIED.,
 .F.,.F.,.F.)
B_SPLINE_SURFACE_WITH_KNOTS((6,1,1,1,1,1,1,1,1,1,1,1,1,1,1,1,1,1,1,1,1,
1,1,1,1,1,1,1,1,1,1,1,1,1,1,1,1,1,1,1,1,1,1,1,1,1,1,1,1,1,1,1,1,1,1,1,1,
1,1,1,1,1,1,1,1,6),(2,2),(-1.,-0.984615384615383,-0.969230769230768,-0.953846153846152,
-0.938461538461537,-0.923076923076922,-0.907692307692306,-0.892307692307691,
-0.876923076923076,-0.86153846153846,-0.846153846153845,-0.83076923076923,
-0.815384615384614,-0.799999999999999,-0.784615384615384,-0.769230769230768,
-0.753846153846153,-0.738461538461538,-0.723076923076922,-0.707692307692307,
-0.692307692307692,-0.676923076923076,-0.661538461538461,-0.646153846153846,
-0.63076923076923,-0.615384615384615,-0.6,-0.584615384615384,-0.569230769230769,
-0.553846153846154,-0.538461538461538,-0.523076923076923,-0.507692307692308,
-0.492307692307692,-0.476923076923077,-0.461538461538462,-0.446153846153846,
-0.430769230769231,-0.415384615384615,-0.4,-0.384615384615385,-0.369230769230769,
-0.353846153846154,-0.338461538461538,-0.323076923076923,-0.307692307692308,
-0.292307692307692,-0.276923076923077,-0.261538461538462,-0.246153846153846,
-0.230769230769231,-0.215384615384615,-0.2,-0.184615384615385,-0.169230769230769,
-0.153846153846154,-0.138461538461538,-0.123076923076923,-0.107692307692308,
-0.0923076923076923,-0.0769230769230769,-0.0615384615384615,-0.0461538461538462,
-0.0307692307692308,-0.0153846153846154,0.),(-1.,1.),.UNSPECIFIED.)
GEOMETRIC_REPRESENTATION_ITEM()
RATIONAL_B_SPLINE_SURFACE(((1.,1.),(1.,1.),(1.,1.),(1.,1.),(1.,1.),(1.,
1.),(1.,1.),(1.,1.),(1.,1.),(1.,1.),(1.,1.),(1.,1.),(1.,1.),(1.,1.),(1.,
1.),(1.,1.),(1.,1.),(1.,1.),(1.,1.),(1.,1.),(1.,1.),(1.,1.),(1.,1.),(1.,
1.),(1.,1.),(1.,1.),(1.,1.),(1.,1.),(1.,1.),(1.,1.),(1.,1.),(1.,1.),(1.,
1.),(1.,1.),(1.,1.),(1.,1.),(1.,1.),(1.,1.),(1.,1.),(1.,1.),(1.,1.),(1.,
1.),(1.,1.),(1.,1.),(1.,1.),(1.,1.),(1.,1.),(1.,1.),(1.,1.),(1.,1.),(1.,
1.),(1.,1.),(1.,1.),(1.,1.),(1.,1.),(1.,1.),(1.,1.),(1.,1.),(1.,1.),(1.,
1.),(1.,1.),(1.,1.),(1.,1.),(1.,1.),(1.,1.),(1.,1.),(1.,1.),(1.,1.),(1.,
1.),(1.,1.)))
REPRESENTATION_ITEM('')
SURFACE()
);
#147=(
BOUNDED_SURFACE()
B_SPLINE_SURFACE(5,1,((#67861,#67862),(#67863,#67864),(#67865,#67866),(#67867,
#67868),(#67869,#67870),(#67871,#67872),(#67873,#67874),(#67875,#67876),
(#67877,#67878),(#67879,#67880),(#67881,#67882),(#67883,#67884),(#67885,
#67886),(#67887,#67888),(#67889,#67890),(#67891,#67892),(#67893,#67894),
(#67895,#67896),(#67897,#67898),(#67899,#67900),(#67901,#67902),(#67903,
#67904),(#67905,#67906),(#67907,#67908),(#67909,#67910),(#67911,#67912),
(#67913,#67914),(#67915,#67916),(#67917,#67918),(#67919,#67920),(#67921,
#67922),(#67923,#67924),(#67925,#67926),(#67927,#67928),(#67929,#67930),
(#67931,#67932),(#67933,#67934),(#67935,#67936),(#67937,#67938),(#67939,
#67940),(#67941,#67942),(#67943,#67944),(#67945,#67946),(#67947,#67948),
(#67949,#67950),(#67951,#67952),(#67953,#67954),(#67955,#67956),(#67957,
#67958),(#67959,#67960),(#67961,#67962),(#67963,#67964),(#67965,#67966),
(#67967,#67968),(#67969,#67970),(#67971,#67972),(#67973,#67974),(#67975,
#67976),(#67977,#67978),(#67979,#67980),(#67981,#67982),(#67983,#67984),
(#67985,#67986),(#67987,#67988),(#67989,#67990),(#67991,#67992),(#67993,
#67994),(#67995,#67996),(#67997,#67998),(#67999,#68000)),.UNSPECIFIED.,
 .F.,.F.,.F.)
B_SPLINE_SURFACE_WITH_KNOTS((6,1,1,1,1,1,1,1,1,1,1,1,1,1,1,1,1,1,1,1,1,
1,1,1,1,1,1,1,1,1,1,1,1,1,1,1,1,1,1,1,1,1,1,1,1,1,1,1,1,1,1,1,1,1,1,1,1,
1,1,1,1,1,1,1,1,6),(2,2),(-1.,-0.984615384615383,-0.969230769230768,-0.953846153846152,
-0.938461538461537,-0.923076923076922,-0.907692307692306,-0.892307692307691,
-0.876923076923076,-0.86153846153846,-0.846153846153845,-0.83076923076923,
-0.815384615384614,-0.799999999999999,-0.784615384615384,-0.769230769230768,
-0.753846153846153,-0.738461538461538,-0.723076923076922,-0.707692307692307,
-0.692307692307692,-0.676923076923076,-0.661538461538461,-0.646153846153846,
-0.63076923076923,-0.615384615384615,-0.6,-0.584615384615384,-0.569230769230769,
-0.553846153846154,-0.538461538461538,-0.523076923076923,-0.507692307692308,
-0.492307692307692,-0.476923076923077,-0.461538461538462,-0.446153846153846,
-0.430769230769231,-0.415384615384615,-0.4,-0.384615384615385,-0.369230769230769,
-0.353846153846154,-0.338461538461538,-0.323076923076923,-0.307692307692308,
-0.292307692307692,-0.276923076923077,-0.261538461538462,-0.246153846153846,
-0.230769230769231,-0.215384615384615,-0.2,-0.184615384615385,-0.169230769230769,
-0.153846153846154,-0.138461538461538,-0.123076923076923,-0.107692307692308,
-0.0923076923076923,-0.0769230769230769,-0.0615384615384615,-0.0461538461538462,
-0.0307692307692308,-0.0153846153846154,0.),(-1.,1.),.UNSPECIFIED.)
GEOMETRIC_REPRESENTATION_ITEM()
RATIONAL_B_SPLINE_SURFACE(((1.,1.),(1.,1.),(1.,1.),(1.,1.),(1.,1.),(1.,
1.),(1.,1.),(1.,1.),(1.,1.),(1.,1.),(1.,1.),(1.,1.),(1.,1.),(1.,1.),(1.,
1.),(1.,1.),(1.,1.),(1.,1.),(1.,1.),(1.,1.),(1.,1.),(1.,1.),(1.,1.),(1.,
1.),(1.,1.),(1.,1.),(1.,1.),(1.,1.),(1.,1.),(1.,1.),(1.,1.),(1.,1.),(1.,
1.),(1.,1.),(1.,1.),(1.,1.),(1.,1.),(1.,1.),(1.,1.),(1.,1.),(1.,1.),(1.,
1.),(1.,1.),(1.,1.),(1.,1.),(1.,1.),(1.,1.),(1.,1.),(1.,1.),(1.,1.),(1.,
1.),(1.,1.),(1.,1.),(1.,1.),(1.,1.),(1.,1.),(1.,1.),(1.,1.),(1.,1.),(1.,
1.),(1.,1.),(1.,1.),(1.,1.),(1.,1.),(1.,1.),(1.,1.),(1.,1.),(1.,1.),(1.,
1.),(1.,1.)))
REPRESENTATION_ITEM('')
SURFACE()
);
#148=(
BOUNDED_SURFACE()
B_SPLINE_SURFACE(5,1,((#68073,#68074),(#68075,#68076),(#68077,#68078),(#68079,
#68080),(#68081,#68082),(#68083,#68084),(#68085,#68086),(#68087,#68088),
(#68089,#68090),(#68091,#68092),(#68093,#68094),(#68095,#68096),(#68097,
#68098),(#68099,#68100),(#68101,#68102),(#68103,#68104),(#68105,#68106),
(#68107,#68108),(#68109,#68110),(#68111,#68112),(#68113,#68114),(#68115,
#68116),(#68117,#68118),(#68119,#68120),(#68121,#68122),(#68123,#68124),
(#68125,#68126),(#68127,#68128),(#68129,#68130),(#68131,#68132),(#68133,
#68134),(#68135,#68136),(#68137,#68138),(#68139,#68140),(#68141,#68142),
(#68143,#68144),(#68145,#68146),(#68147,#68148),(#68149,#68150),(#68151,
#68152),(#68153,#68154),(#68155,#68156),(#68157,#68158),(#68159,#68160),
(#68161,#68162),(#68163,#68164),(#68165,#68166),(#68167,#68168),(#68169,
#68170),(#68171,#68172),(#68173,#68174),(#68175,#68176),(#68177,#68178),
(#68179,#68180),(#68181,#68182),(#68183,#68184),(#68185,#68186),(#68187,
#68188),(#68189,#68190),(#68191,#68192),(#68193,#68194),(#68195,#68196),
(#68197,#68198),(#68199,#68200),(#68201,#68202),(#68203,#68204),(#68205,
#68206),(#68207,#68208),(#68209,#68210),(#68211,#68212)),.UNSPECIFIED.,
 .F.,.F.,.F.)
B_SPLINE_SURFACE_WITH_KNOTS((6,1,1,1,1,1,1,1,1,1,1,1,1,1,1,1,1,1,1,1,1,
1,1,1,1,1,1,1,1,1,1,1,1,1,1,1,1,1,1,1,1,1,1,1,1,1,1,1,1,1,1,1,1,1,1,1,1,
1,1,1,1,1,1,1,1,6),(2,2),(-1.,-0.984615384615383,-0.969230769230768,-0.953846153846152,
-0.938461538461537,-0.923076923076922,-0.907692307692306,-0.892307692307691,
-0.876923076923076,-0.86153846153846,-0.846153846153845,-0.83076923076923,
-0.815384615384614,-0.799999999999999,-0.784615384615384,-0.769230769230768,
-0.753846153846153,-0.738461538461538,-0.723076923076922,-0.707692307692307,
-0.692307692307692,-0.676923076923076,-0.661538461538461,-0.646153846153846,
-0.63076923076923,-0.615384615384615,-0.6,-0.584615384615384,-0.569230769230769,
-0.553846153846154,-0.538461538461538,-0.523076923076923,-0.507692307692308,
-0.492307692307692,-0.476923076923077,-0.461538461538462,-0.446153846153846,
-0.430769230769231,-0.415384615384615,-0.4,-0.384615384615385,-0.369230769230769,
-0.353846153846154,-0.338461538461538,-0.323076923076923,-0.307692307692308,
-0.292307692307692,-0.276923076923077,-0.261538461538462,-0.246153846153846,
-0.230769230769231,-0.215384615384615,-0.2,-0.184615384615385,-0.169230769230769,
-0.153846153846154,-0.138461538461538,-0.123076923076923,-0.107692307692308,
-0.0923076923076923,-0.0769230769230769,-0.0615384615384615,-0.0461538461538462,
-0.0307692307692308,-0.0153846153846154,0.),(-1.,1.),.UNSPECIFIED.)
GEOMETRIC_REPRESENTATION_ITEM()
RATIONAL_B_SPLINE_SURFACE(((1.,1.),(1.,1.),(1.,1.),(1.,1.),(1.,1.),(1.,
1.),(1.,1.),(1.,1.),(1.,1.),(1.,1.),(1.,1.),(1.,1.),(1.,1.),(1.,1.),(1.,
1.),(1.,1.),(1.,1.),(1.,1.),(1.,1.),(1.,1.),(1.,1.),(1.,1.),(1.,1.),(1.,
1.),(1.,1.),(1.,1.),(1.,1.),(1.,1.),(1.,1.),(1.,1.),(1.,1.),(1.,1.),(1.,
1.),(1.,1.),(1.,1.),(1.,1.),(1.,1.),(1.,1.),(1.,1.),(1.,1.),(1.,1.),(1.,
1.),(1.,1.),(1.,1.),(1.,1.),(1.,1.),(1.,1.),(1.,1.),(1.,1.),(1.,1.),(1.,
1.),(1.,1.),(1.,1.),(1.,1.),(1.,1.),(1.,1.),(1.,1.),(1.,1.),(1.,1.),(1.,
1.),(1.,1.),(1.,1.),(1.,1.),(1.,1.),(1.,1.),(1.,1.),(1.,1.),(1.,1.),(1.,
1.),(1.,1.)))
REPRESENTATION_ITEM('')
SURFACE()
);
#149=(
BOUNDED_SURFACE()
B_SPLINE_SURFACE(5,1,((#68303,#68304),(#68305,#68306),(#68307,#68308),(#68309,
#68310),(#68311,#68312),(#68313,#68314),(#68315,#68316),(#68317,#68318),
(#68319,#68320),(#68321,#68322),(#68323,#68324),(#68325,#68326),(#68327,
#68328),(#68329,#68330),(#68331,#68332),(#68333,#68334),(#68335,#68336),
(#68337,#68338),(#68339,#68340),(#68341,#68342),(#68343,#68344),(#68345,
#68346),(#68347,#68348),(#68349,#68350),(#68351,#68352),(#68353,#68354),
(#68355,#68356),(#68357,#68358),(#68359,#68360),(#68361,#68362),(#68363,
#68364),(#68365,#68366),(#68367,#68368),(#68369,#68370),(#68371,#68372),
(#68373,#68374),(#68375,#68376),(#68377,#68378),(#68379,#68380),(#68381,
#68382),(#68383,#68384),(#68385,#68386),(#68387,#68388),(#68389,#68390),
(#68391,#68392),(#68393,#68394),(#68395,#68396),(#68397,#68398),(#68399,
#68400),(#68401,#68402),(#68403,#68404),(#68405,#68406),(#68407,#68408),
(#68409,#68410),(#68411,#68412),(#68413,#68414),(#68415,#68416),(#68417,
#68418),(#68419,#68420),(#68421,#68422),(#68423,#68424),(#68425,#68426),
(#68427,#68428),(#68429,#68430),(#68431,#68432),(#68433,#68434),(#68435,
#68436),(#68437,#68438),(#68439,#68440),(#68441,#68442)),.UNSPECIFIED.,
 .F.,.F.,.F.)
B_SPLINE_SURFACE_WITH_KNOTS((6,1,1,1,1,1,1,1,1,1,1,1,1,1,1,1,1,1,1,1,1,
1,1,1,1,1,1,1,1,1,1,1,1,1,1,1,1,1,1,1,1,1,1,1,1,1,1,1,1,1,1,1,1,1,1,1,1,
1,1,1,1,1,1,1,1,6),(2,2),(-1.,-0.984615384615383,-0.969230769230768,-0.953846153846152,
-0.938461538461537,-0.923076923076922,-0.907692307692306,-0.892307692307691,
-0.876923076923076,-0.86153846153846,-0.846153846153845,-0.83076923076923,
-0.815384615384614,-0.799999999999999,-0.784615384615384,-0.769230769230768,
-0.753846153846153,-0.738461538461538,-0.723076923076922,-0.707692307692307,
-0.692307692307692,-0.676923076923076,-0.661538461538461,-0.646153846153846,
-0.63076923076923,-0.615384615384615,-0.6,-0.584615384615384,-0.569230769230769,
-0.553846153846154,-0.538461538461538,-0.523076923076923,-0.507692307692308,
-0.492307692307692,-0.476923076923077,-0.461538461538462,-0.446153846153846,
-0.430769230769231,-0.415384615384615,-0.4,-0.384615384615385,-0.369230769230769,
-0.353846153846154,-0.338461538461538,-0.323076923076923,-0.307692307692308,
-0.292307692307692,-0.276923076923077,-0.261538461538462,-0.246153846153846,
-0.230769230769231,-0.215384615384615,-0.2,-0.184615384615385,-0.169230769230769,
-0.153846153846154,-0.138461538461538,-0.123076923076923,-0.107692307692308,
-0.0923076923076923,-0.0769230769230769,-0.0615384615384615,-0.0461538461538462,
-0.0307692307692308,-0.0153846153846154,0.),(-1.,1.),.UNSPECIFIED.)
GEOMETRIC_REPRESENTATION_ITEM()
RATIONAL_B_SPLINE_SURFACE(((1.,1.),(1.,1.),(1.,1.),(1.,1.),(1.,1.),(1.,
1.),(1.,1.),(1.,1.),(1.,1.),(1.,1.),(1.,1.),(1.,1.),(1.,1.),(1.,1.),(1.,
1.),(1.,1.),(1.,1.),(1.,1.),(1.,1.),(1.,1.),(1.,1.),(1.,1.),(1.,1.),(1.,
1.),(1.,1.),(1.,1.),(1.,1.),(1.,1.),(1.,1.),(1.,1.),(1.,1.),(1.,1.),(1.,
1.),(1.,1.),(1.,1.),(1.,1.),(1.,1.),(1.,1.),(1.,1.),(1.,1.),(1.,1.),(1.,
1.),(1.,1.),(1.,1.),(1.,1.),(1.,1.),(1.,1.),(1.,1.),(1.,1.),(1.,1.),(1.,
1.),(1.,1.),(1.,1.),(1.,1.),(1.,1.),(1.,1.),(1.,1.),(1.,1.),(1.,1.),(1.,
1.),(1.,1.),(1.,1.),(1.,1.),(1.,1.),(1.,1.),(1.,1.),(1.,1.),(1.,1.),(1.,
1.),(1.,1.)))
REPRESENTATION_ITEM('')
SURFACE()
);
#150=(
BOUNDED_SURFACE()
B_SPLINE_SURFACE(5,1,((#68515,#68516),(#68517,#68518),(#68519,#68520),(#68521,
#68522),(#68523,#68524),(#68525,#68526),(#68527,#68528),(#68529,#68530),
(#68531,#68532),(#68533,#68534),(#68535,#68536),(#68537,#68538),(#68539,
#68540),(#68541,#68542),(#68543,#68544),(#68545,#68546),(#68547,#68548),
(#68549,#68550),(#68551,#68552),(#68553,#68554),(#68555,#68556),(#68557,
#68558),(#68559,#68560),(#68561,#68562),(#68563,#68564),(#68565,#68566),
(#68567,#68568),(#68569,#68570),(#68571,#68572),(#68573,#68574),(#68575,
#68576),(#68577,#68578),(#68579,#68580),(#68581,#68582),(#68583,#68584),
(#68585,#68586),(#68587,#68588),(#68589,#68590),(#68591,#68592),(#68593,
#68594),(#68595,#68596),(#68597,#68598),(#68599,#68600),(#68601,#68602),
(#68603,#68604),(#68605,#68606),(#68607,#68608),(#68609,#68610),(#68611,
#68612),(#68613,#68614),(#68615,#68616),(#68617,#68618),(#68619,#68620),
(#68621,#68622),(#68623,#68624),(#68625,#68626),(#68627,#68628),(#68629,
#68630),(#68631,#68632),(#68633,#68634),(#68635,#68636),(#68637,#68638),
(#68639,#68640),(#68641,#68642),(#68643,#68644),(#68645,#68646),(#68647,
#68648),(#68649,#68650),(#68651,#68652),(#68653,#68654)),.UNSPECIFIED.,
 .F.,.F.,.F.)
B_SPLINE_SURFACE_WITH_KNOTS((6,1,1,1,1,1,1,1,1,1,1,1,1,1,1,1,1,1,1,1,1,
1,1,1,1,1,1,1,1,1,1,1,1,1,1,1,1,1,1,1,1,1,1,1,1,1,1,1,1,1,1,1,1,1,1,1,1,
1,1,1,1,1,1,1,1,6),(2,2),(-1.,-0.984615384615383,-0.969230769230768,-0.953846153846152,
-0.938461538461537,-0.923076923076922,-0.907692307692306,-0.892307692307691,
-0.876923076923076,-0.86153846153846,-0.846153846153845,-0.83076923076923,
-0.815384615384614,-0.799999999999999,-0.784615384615384,-0.769230769230768,
-0.753846153846153,-0.738461538461538,-0.723076923076922,-0.707692307692307,
-0.692307692307692,-0.676923076923076,-0.661538461538461,-0.646153846153846,
-0.63076923076923,-0.615384615384615,-0.6,-0.584615384615384,-0.569230769230769,
-0.553846153846154,-0.538461538461538,-0.523076923076923,-0.507692307692308,
-0.492307692307692,-0.476923076923077,-0.461538461538462,-0.446153846153846,
-0.430769230769231,-0.415384615384615,-0.4,-0.384615384615385,-0.369230769230769,
-0.353846153846154,-0.338461538461538,-0.323076923076923,-0.307692307692308,
-0.292307692307692,-0.276923076923077,-0.261538461538462,-0.246153846153846,
-0.230769230769231,-0.215384615384615,-0.2,-0.184615384615385,-0.169230769230769,
-0.153846153846154,-0.138461538461538,-0.123076923076923,-0.107692307692308,
-0.0923076923076923,-0.0769230769230769,-0.0615384615384615,-0.0461538461538462,
-0.0307692307692308,-0.0153846153846154,0.),(-1.,1.),.UNSPECIFIED.)
GEOMETRIC_REPRESENTATION_ITEM()
RATIONAL_B_SPLINE_SURFACE(((1.,1.),(1.,1.),(1.,1.),(1.,1.),(1.,1.),(1.,
1.),(1.,1.),(1.,1.),(1.,1.),(1.,1.),(1.,1.),(1.,1.),(1.,1.),(1.,1.),(1.,
1.),(1.,1.),(1.,1.),(1.,1.),(1.,1.),(1.,1.),(1.,1.),(1.,1.),(1.,1.),(1.,
1.),(1.,1.),(1.,1.),(1.,1.),(1.,1.),(1.,1.),(1.,1.),(1.,1.),(1.,1.),(1.,
1.),(1.,1.),(1.,1.),(1.,1.),(1.,1.),(1.,1.),(1.,1.),(1.,1.),(1.,1.),(1.,
1.),(1.,1.),(1.,1.),(1.,1.),(1.,1.),(1.,1.),(1.,1.),(1.,1.),(1.,1.),(1.,
1.),(1.,1.),(1.,1.),(1.,1.),(1.,1.),(1.,1.),(1.,1.),(1.,1.),(1.,1.),(1.,
1.),(1.,1.),(1.,1.),(1.,1.),(1.,1.),(1.,1.),(1.,1.),(1.,1.),(1.,1.),(1.,
1.),(1.,1.)))
REPRESENTATION_ITEM('')
SURFACE()
);
#151=(
BOUNDED_SURFACE()
B_SPLINE_SURFACE(5,1,((#68745,#68746),(#68747,#68748),(#68749,#68750),(#68751,
#68752),(#68753,#68754),(#68755,#68756),(#68757,#68758),(#68759,#68760),
(#68761,#68762),(#68763,#68764),(#68765,#68766),(#68767,#68768),(#68769,
#68770),(#68771,#68772),(#68773,#68774),(#68775,#68776),(#68777,#68778),
(#68779,#68780),(#68781,#68782),(#68783,#68784),(#68785,#68786),(#68787,
#68788),(#68789,#68790),(#68791,#68792),(#68793,#68794),(#68795,#68796),
(#68797,#68798),(#68799,#68800),(#68801,#68802),(#68803,#68804),(#68805,
#68806),(#68807,#68808),(#68809,#68810),(#68811,#68812),(#68813,#68814),
(#68815,#68816),(#68817,#68818),(#68819,#68820),(#68821,#68822),(#68823,
#68824),(#68825,#68826),(#68827,#68828),(#68829,#68830),(#68831,#68832),
(#68833,#68834),(#68835,#68836),(#68837,#68838),(#68839,#68840),(#68841,
#68842),(#68843,#68844),(#68845,#68846),(#68847,#68848),(#68849,#68850),
(#68851,#68852),(#68853,#68854),(#68855,#68856),(#68857,#68858),(#68859,
#68860),(#68861,#68862),(#68863,#68864),(#68865,#68866),(#68867,#68868),
(#68869,#68870),(#68871,#68872),(#68873,#68874),(#68875,#68876),(#68877,
#68878),(#68879,#68880),(#68881,#68882),(#68883,#68884)),.UNSPECIFIED.,
 .F.,.F.,.F.)
B_SPLINE_SURFACE_WITH_KNOTS((6,1,1,1,1,1,1,1,1,1,1,1,1,1,1,1,1,1,1,1,1,
1,1,1,1,1,1,1,1,1,1,1,1,1,1,1,1,1,1,1,1,1,1,1,1,1,1,1,1,1,1,1,1,1,1,1,1,
1,1,1,1,1,1,1,1,6),(2,2),(-1.,-0.984615384615383,-0.969230769230768,-0.953846153846152,
-0.938461538461537,-0.923076923076922,-0.907692307692306,-0.892307692307691,
-0.876923076923076,-0.86153846153846,-0.846153846153845,-0.83076923076923,
-0.815384615384614,-0.799999999999999,-0.784615384615384,-0.769230769230768,
-0.753846153846153,-0.738461538461538,-0.723076923076922,-0.707692307692307,
-0.692307692307692,-0.676923076923076,-0.661538461538461,-0.646153846153846,
-0.63076923076923,-0.615384615384615,-0.6,-0.584615384615384,-0.569230769230769,
-0.553846153846154,-0.538461538461538,-0.523076923076923,-0.507692307692308,
-0.492307692307692,-0.476923076923077,-0.461538461538462,-0.446153846153846,
-0.430769230769231,-0.415384615384615,-0.4,-0.384615384615385,-0.369230769230769,
-0.353846153846154,-0.338461538461538,-0.323076923076923,-0.307692307692308,
-0.292307692307692,-0.276923076923077,-0.261538461538462,-0.246153846153846,
-0.230769230769231,-0.215384615384615,-0.2,-0.184615384615385,-0.169230769230769,
-0.153846153846154,-0.138461538461538,-0.123076923076923,-0.107692307692308,
-0.0923076923076923,-0.0769230769230769,-0.0615384615384615,-0.0461538461538462,
-0.0307692307692308,-0.0153846153846154,0.),(-1.,1.),.UNSPECIFIED.)
GEOMETRIC_REPRESENTATION_ITEM()
RATIONAL_B_SPLINE_SURFACE(((1.,1.),(1.,1.),(1.,1.),(1.,1.),(1.,1.),(1.,
1.),(1.,1.),(1.,1.),(1.,1.),(1.,1.),(1.,1.),(1.,1.),(1.,1.),(1.,1.),(1.,
1.),(1.,1.),(1.,1.),(1.,1.),(1.,1.),(1.,1.),(1.,1.),(1.,1.),(1.,1.),(1.,
1.),(1.,1.),(1.,1.),(1.,1.),(1.,1.),(1.,1.),(1.,1.),(1.,1.),(1.,1.),(1.,
1.),(1.,1.),(1.,1.),(1.,1.),(1.,1.),(1.,1.),(1.,1.),(1.,1.),(1.,1.),(1.,
1.),(1.,1.),(1.,1.),(1.,1.),(1.,1.),(1.,1.),(1.,1.),(1.,1.),(1.,1.),(1.,
1.),(1.,1.),(1.,1.),(1.,1.),(1.,1.),(1.,1.),(1.,1.),(1.,1.),(1.,1.),(1.,
1.),(1.,1.),(1.,1.),(1.,1.),(1.,1.),(1.,1.),(1.,1.),(1.,1.),(1.,1.),(1.,
1.),(1.,1.)))
REPRESENTATION_ITEM('')
SURFACE()
);
#152=(
BOUNDED_SURFACE()
B_SPLINE_SURFACE(5,1,((#68957,#68958),(#68959,#68960),(#68961,#68962),(#68963,
#68964),(#68965,#68966),(#68967,#68968),(#68969,#68970),(#68971,#68972),
(#68973,#68974),(#68975,#68976),(#68977,#68978),(#68979,#68980),(#68981,
#68982),(#68983,#68984),(#68985,#68986),(#68987,#68988),(#68989,#68990),
(#68991,#68992),(#68993,#68994),(#68995,#68996),(#68997,#68998),(#68999,
#69000),(#69001,#69002),(#69003,#69004),(#69005,#69006),(#69007,#69008),
(#69009,#69010),(#69011,#69012),(#69013,#69014),(#69015,#69016),(#69017,
#69018),(#69019,#69020),(#69021,#69022),(#69023,#69024),(#69025,#69026),
(#69027,#69028),(#69029,#69030),(#69031,#69032),(#69033,#69034),(#69035,
#69036),(#69037,#69038),(#69039,#69040),(#69041,#69042),(#69043,#69044),
(#69045,#69046),(#69047,#69048),(#69049,#69050),(#69051,#69052),(#69053,
#69054),(#69055,#69056),(#69057,#69058),(#69059,#69060),(#69061,#69062),
(#69063,#69064),(#69065,#69066),(#69067,#69068),(#69069,#69070),(#69071,
#69072),(#69073,#69074),(#69075,#69076),(#69077,#69078),(#69079,#69080),
(#69081,#69082),(#69083,#69084),(#69085,#69086),(#69087,#69088),(#69089,
#69090),(#69091,#69092),(#69093,#69094),(#69095,#69096)),.UNSPECIFIED.,
 .F.,.F.,.F.)
B_SPLINE_SURFACE_WITH_KNOTS((6,1,1,1,1,1,1,1,1,1,1,1,1,1,1,1,1,1,1,1,1,
1,1,1,1,1,1,1,1,1,1,1,1,1,1,1,1,1,1,1,1,1,1,1,1,1,1,1,1,1,1,1,1,1,1,1,1,
1,1,1,1,1,1,1,1,6),(2,2),(-1.,-0.984615384615383,-0.969230769230768,-0.953846153846152,
-0.938461538461537,-0.923076923076922,-0.907692307692306,-0.892307692307691,
-0.876923076923076,-0.86153846153846,-0.846153846153845,-0.83076923076923,
-0.815384615384614,-0.799999999999999,-0.784615384615384,-0.769230769230768,
-0.753846153846153,-0.738461538461538,-0.723076923076922,-0.707692307692307,
-0.692307692307692,-0.676923076923076,-0.661538461538461,-0.646153846153846,
-0.63076923076923,-0.615384615384615,-0.6,-0.584615384615384,-0.569230769230769,
-0.553846153846154,-0.538461538461538,-0.523076923076923,-0.507692307692308,
-0.492307692307692,-0.476923076923077,-0.461538461538462,-0.446153846153846,
-0.430769230769231,-0.415384615384615,-0.4,-0.384615384615385,-0.369230769230769,
-0.353846153846154,-0.338461538461538,-0.323076923076923,-0.307692307692308,
-0.292307692307692,-0.276923076923077,-0.261538461538462,-0.246153846153846,
-0.230769230769231,-0.215384615384615,-0.2,-0.184615384615385,-0.169230769230769,
-0.153846153846154,-0.138461538461538,-0.123076923076923,-0.107692307692308,
-0.0923076923076923,-0.0769230769230769,-0.0615384615384615,-0.0461538461538462,
-0.0307692307692308,-0.0153846153846154,0.),(-1.,1.),.UNSPECIFIED.)
GEOMETRIC_REPRESENTATION_ITEM()
RATIONAL_B_SPLINE_SURFACE(((1.,1.),(1.,1.),(1.,1.),(1.,1.),(1.,1.),(1.,
1.),(1.,1.),(1.,1.),(1.,1.),(1.,1.),(1.,1.),(1.,1.),(1.,1.),(1.,1.),(1.,
1.),(1.,1.),(1.,1.),(1.,1.),(1.,1.),(1.,1.),(1.,1.),(1.,1.),(1.,1.),(1.,
1.),(1.,1.),(1.,1.),(1.,1.),(1.,1.),(1.,1.),(1.,1.),(1.,1.),(1.,1.),(1.,
1.),(1.,1.),(1.,1.),(1.,1.),(1.,1.),(1.,1.),(1.,1.),(1.,1.),(1.,1.),(1.,
1.),(1.,1.),(1.,1.),(1.,1.),(1.,1.),(1.,1.),(1.,1.),(1.,1.),(1.,1.),(1.,
1.),(1.,1.),(1.,1.),(1.,1.),(1.,1.),(1.,1.),(1.,1.),(1.,1.),(1.,1.),(1.,
1.),(1.,1.),(1.,1.),(1.,1.),(1.,1.),(1.,1.),(1.,1.),(1.,1.),(1.,1.),(1.,
1.),(1.,1.)))
REPRESENTATION_ITEM('')
SURFACE()
);
#153=(
BOUNDED_SURFACE()
B_SPLINE_SURFACE(5,1,((#69187,#69188),(#69189,#69190),(#69191,#69192),(#69193,
#69194),(#69195,#69196),(#69197,#69198),(#69199,#69200),(#69201,#69202),
(#69203,#69204),(#69205,#69206),(#69207,#69208),(#69209,#69210),(#69211,
#69212),(#69213,#69214),(#69215,#69216),(#69217,#69218),(#69219,#69220),
(#69221,#69222),(#69223,#69224),(#69225,#69226),(#69227,#69228),(#69229,
#69230),(#69231,#69232),(#69233,#69234),(#69235,#69236),(#69237,#69238),
(#69239,#69240),(#69241,#69242),(#69243,#69244),(#69245,#69246),(#69247,
#69248),(#69249,#69250),(#69251,#69252),(#69253,#69254),(#69255,#69256),
(#69257,#69258),(#69259,#69260),(#69261,#69262),(#69263,#69264),(#69265,
#69266),(#69267,#69268),(#69269,#69270),(#69271,#69272),(#69273,#69274),
(#69275,#69276),(#69277,#69278),(#69279,#69280),(#69281,#69282),(#69283,
#69284),(#69285,#69286),(#69287,#69288),(#69289,#69290),(#69291,#69292),
(#69293,#69294),(#69295,#69296),(#69297,#69298),(#69299,#69300),(#69301,
#69302),(#69303,#69304),(#69305,#69306),(#69307,#69308),(#69309,#69310),
(#69311,#69312),(#69313,#69314),(#69315,#69316),(#69317,#69318),(#69319,
#69320),(#69321,#69322),(#69323,#69324),(#69325,#69326)),.UNSPECIFIED.,
 .F.,.F.,.F.)
B_SPLINE_SURFACE_WITH_KNOTS((6,1,1,1,1,1,1,1,1,1,1,1,1,1,1,1,1,1,1,1,1,
1,1,1,1,1,1,1,1,1,1,1,1,1,1,1,1,1,1,1,1,1,1,1,1,1,1,1,1,1,1,1,1,1,1,1,1,
1,1,1,1,1,1,1,1,6),(2,2),(-1.,-0.984615384615383,-0.969230769230768,-0.953846153846152,
-0.938461538461537,-0.923076923076922,-0.907692307692306,-0.892307692307691,
-0.876923076923076,-0.86153846153846,-0.846153846153845,-0.83076923076923,
-0.815384615384614,-0.799999999999999,-0.784615384615384,-0.769230769230768,
-0.753846153846153,-0.738461538461538,-0.723076923076922,-0.707692307692307,
-0.692307692307692,-0.676923076923076,-0.661538461538461,-0.646153846153846,
-0.63076923076923,-0.615384615384615,-0.6,-0.584615384615384,-0.569230769230769,
-0.553846153846154,-0.538461538461538,-0.523076923076923,-0.507692307692308,
-0.492307692307692,-0.476923076923077,-0.461538461538462,-0.446153846153846,
-0.430769230769231,-0.415384615384615,-0.4,-0.384615384615385,-0.369230769230769,
-0.353846153846154,-0.338461538461538,-0.323076923076923,-0.307692307692308,
-0.292307692307692,-0.276923076923077,-0.261538461538462,-0.246153846153846,
-0.230769230769231,-0.215384615384615,-0.2,-0.184615384615385,-0.169230769230769,
-0.153846153846154,-0.138461538461538,-0.123076923076923,-0.107692307692308,
-0.0923076923076923,-0.0769230769230769,-0.0615384615384615,-0.0461538461538462,
-0.0307692307692308,-0.0153846153846154,0.),(-1.,1.),.UNSPECIFIED.)
GEOMETRIC_REPRESENTATION_ITEM()
RATIONAL_B_SPLINE_SURFACE(((1.,1.),(1.,1.),(1.,1.),(1.,1.),(1.,1.),(1.,
1.),(1.,1.),(1.,1.),(1.,1.),(1.,1.),(1.,1.),(1.,1.),(1.,1.),(1.,1.),(1.,
1.),(1.,1.),(1.,1.),(1.,1.),(1.,1.),(1.,1.),(1.,1.),(1.,1.),(1.,1.),(1.,
1.),(1.,1.),(1.,1.),(1.,1.),(1.,1.),(1.,1.),(1.,1.),(1.,1.),(1.,1.),(1.,
1.),(1.,1.),(1.,1.),(1.,1.),(1.,1.),(1.,1.),(1.,1.),(1.,1.),(1.,1.),(1.,
1.),(1.,1.),(1.,1.),(1.,1.),(1.,1.),(1.,1.),(1.,1.),(1.,1.),(1.,1.),(1.,
1.),(1.,1.),(1.,1.),(1.,1.),(1.,1.),(1.,1.),(1.,1.),(1.,1.),(1.,1.),(1.,
1.),(1.,1.),(1.,1.),(1.,1.),(1.,1.),(1.,1.),(1.,1.),(1.,1.),(1.,1.),(1.,
1.),(1.,1.)))
REPRESENTATION_ITEM('')
SURFACE()
);
#154=(
BOUNDED_SURFACE()
B_SPLINE_SURFACE(5,1,((#69399,#69400),(#69401,#69402),(#69403,#69404),(#69405,
#69406),(#69407,#69408),(#69409,#69410),(#69411,#69412),(#69413,#69414),
(#69415,#69416),(#69417,#69418),(#69419,#69420),(#69421,#69422),(#69423,
#69424),(#69425,#69426),(#69427,#69428),(#69429,#69430),(#69431,#69432),
(#69433,#69434),(#69435,#69436),(#69437,#69438),(#69439,#69440),(#69441,
#69442),(#69443,#69444),(#69445,#69446),(#69447,#69448),(#69449,#69450),
(#69451,#69452),(#69453,#69454),(#69455,#69456),(#69457,#69458),(#69459,
#69460),(#69461,#69462),(#69463,#69464),(#69465,#69466),(#69467,#69468),
(#69469,#69470),(#69471,#69472),(#69473,#69474),(#69475,#69476),(#69477,
#69478),(#69479,#69480),(#69481,#69482),(#69483,#69484),(#69485,#69486),
(#69487,#69488),(#69489,#69490),(#69491,#69492),(#69493,#69494),(#69495,
#69496),(#69497,#69498),(#69499,#69500),(#69501,#69502),(#69503,#69504),
(#69505,#69506),(#69507,#69508),(#69509,#69510),(#69511,#69512),(#69513,
#69514),(#69515,#69516),(#69517,#69518),(#69519,#69520),(#69521,#69522),
(#69523,#69524),(#69525,#69526),(#69527,#69528),(#69529,#69530),(#69531,
#69532),(#69533,#69534),(#69535,#69536),(#69537,#69538)),.UNSPECIFIED.,
 .F.,.F.,.F.)
B_SPLINE_SURFACE_WITH_KNOTS((6,1,1,1,1,1,1,1,1,1,1,1,1,1,1,1,1,1,1,1,1,
1,1,1,1,1,1,1,1,1,1,1,1,1,1,1,1,1,1,1,1,1,1,1,1,1,1,1,1,1,1,1,1,1,1,1,1,
1,1,1,1,1,1,1,1,6),(2,2),(-1.,-0.984615384615383,-0.969230769230768,-0.953846153846152,
-0.938461538461537,-0.923076923076922,-0.907692307692306,-0.892307692307691,
-0.876923076923076,-0.86153846153846,-0.846153846153845,-0.83076923076923,
-0.815384615384614,-0.799999999999999,-0.784615384615384,-0.769230769230768,
-0.753846153846153,-0.738461538461538,-0.723076923076922,-0.707692307692307,
-0.692307692307692,-0.676923076923076,-0.661538461538461,-0.646153846153846,
-0.63076923076923,-0.615384615384615,-0.6,-0.584615384615384,-0.569230769230769,
-0.553846153846154,-0.538461538461538,-0.523076923076923,-0.507692307692308,
-0.492307692307692,-0.476923076923077,-0.461538461538462,-0.446153846153846,
-0.430769230769231,-0.415384615384615,-0.4,-0.384615384615385,-0.369230769230769,
-0.353846153846154,-0.338461538461538,-0.323076923076923,-0.307692307692308,
-0.292307692307692,-0.276923076923077,-0.261538461538462,-0.246153846153846,
-0.230769230769231,-0.215384615384615,-0.2,-0.184615384615385,-0.169230769230769,
-0.153846153846154,-0.138461538461538,-0.123076923076923,-0.107692307692308,
-0.0923076923076923,-0.0769230769230769,-0.0615384615384615,-0.0461538461538462,
-0.0307692307692308,-0.0153846153846154,0.),(-1.,1.),.UNSPECIFIED.)
GEOMETRIC_REPRESENTATION_ITEM()
RATIONAL_B_SPLINE_SURFACE(((1.,1.),(1.,1.),(1.,1.),(1.,1.),(1.,1.),(1.,
1.),(1.,1.),(1.,1.),(1.,1.),(1.,1.),(1.,1.),(1.,1.),(1.,1.),(1.,1.),(1.,
1.),(1.,1.),(1.,1.),(1.,1.),(1.,1.),(1.,1.),(1.,1.),(1.,1.),(1.,1.),(1.,
1.),(1.,1.),(1.,1.),(1.,1.),(1.,1.),(1.,1.),(1.,1.),(1.,1.),(1.,1.),(1.,
1.),(1.,1.),(1.,1.),(1.,1.),(1.,1.),(1.,1.),(1.,1.),(1.,1.),(1.,1.),(1.,
1.),(1.,1.),(1.,1.),(1.,1.),(1.,1.),(1.,1.),(1.,1.),(1.,1.),(1.,1.),(1.,
1.),(1.,1.),(1.,1.),(1.,1.),(1.,1.),(1.,1.),(1.,1.),(1.,1.),(1.,1.),(1.,
1.),(1.,1.),(1.,1.),(1.,1.),(1.,1.),(1.,1.),(1.,1.),(1.,1.),(1.,1.),(1.,
1.),(1.,1.)))
REPRESENTATION_ITEM('')
SURFACE()
);
#155=(
BOUNDED_SURFACE()
B_SPLINE_SURFACE(5,1,((#69629,#69630),(#69631,#69632),(#69633,#69634),(#69635,
#69636),(#69637,#69638),(#69639,#69640),(#69641,#69642),(#69643,#69644),
(#69645,#69646),(#69647,#69648),(#69649,#69650),(#69651,#69652),(#69653,
#69654),(#69655,#69656),(#69657,#69658),(#69659,#69660),(#69661,#69662),
(#69663,#69664),(#69665,#69666),(#69667,#69668),(#69669,#69670),(#69671,
#69672),(#69673,#69674),(#69675,#69676),(#69677,#69678),(#69679,#69680),
(#69681,#69682),(#69683,#69684),(#69685,#69686),(#69687,#69688),(#69689,
#69690),(#69691,#69692),(#69693,#69694),(#69695,#69696),(#69697,#69698),
(#69699,#69700),(#69701,#69702),(#69703,#69704),(#69705,#69706),(#69707,
#69708),(#69709,#69710),(#69711,#69712),(#69713,#69714),(#69715,#69716),
(#69717,#69718),(#69719,#69720),(#69721,#69722),(#69723,#69724),(#69725,
#69726),(#69727,#69728),(#69729,#69730),(#69731,#69732),(#69733,#69734),
(#69735,#69736),(#69737,#69738),(#69739,#69740),(#69741,#69742),(#69743,
#69744),(#69745,#69746),(#69747,#69748),(#69749,#69750),(#69751,#69752),
(#69753,#69754),(#69755,#69756),(#69757,#69758),(#69759,#69760),(#69761,
#69762),(#69763,#69764),(#69765,#69766),(#69767,#69768)),.UNSPECIFIED.,
 .F.,.F.,.F.)
B_SPLINE_SURFACE_WITH_KNOTS((6,1,1,1,1,1,1,1,1,1,1,1,1,1,1,1,1,1,1,1,1,
1,1,1,1,1,1,1,1,1,1,1,1,1,1,1,1,1,1,1,1,1,1,1,1,1,1,1,1,1,1,1,1,1,1,1,1,
1,1,1,1,1,1,1,1,6),(2,2),(-1.,-0.984615384615383,-0.969230769230768,-0.953846153846152,
-0.938461538461537,-0.923076923076922,-0.907692307692306,-0.892307692307691,
-0.876923076923076,-0.86153846153846,-0.846153846153845,-0.83076923076923,
-0.815384615384614,-0.799999999999999,-0.784615384615384,-0.769230769230768,
-0.753846153846153,-0.738461538461538,-0.723076923076922,-0.707692307692307,
-0.692307692307692,-0.676923076923076,-0.661538461538461,-0.646153846153846,
-0.63076923076923,-0.615384615384615,-0.6,-0.584615384615384,-0.569230769230769,
-0.553846153846154,-0.538461538461538,-0.523076923076923,-0.507692307692308,
-0.492307692307692,-0.476923076923077,-0.461538461538462,-0.446153846153846,
-0.430769230769231,-0.415384615384615,-0.4,-0.384615384615385,-0.369230769230769,
-0.353846153846154,-0.338461538461538,-0.323076923076923,-0.307692307692308,
-0.292307692307692,-0.276923076923077,-0.261538461538462,-0.246153846153846,
-0.230769230769231,-0.215384615384615,-0.2,-0.184615384615385,-0.169230769230769,
-0.153846153846154,-0.138461538461538,-0.123076923076923,-0.107692307692308,
-0.0923076923076923,-0.0769230769230769,-0.0615384615384615,-0.0461538461538462,
-0.0307692307692308,-0.0153846153846154,0.),(-1.,1.),.UNSPECIFIED.)
GEOMETRIC_REPRESENTATION_ITEM()
RATIONAL_B_SPLINE_SURFACE(((1.,1.),(1.,1.),(1.,1.),(1.,1.),(1.,1.),(1.,
1.),(1.,1.),(1.,1.),(1.,1.),(1.,1.),(1.,1.),(1.,1.),(1.,1.),(1.,1.),(1.,
1.),(1.,1.),(1.,1.),(1.,1.),(1.,1.),(1.,1.),(1.,1.),(1.,1.),(1.,1.),(1.,
1.),(1.,1.),(1.,1.),(1.,1.),(1.,1.),(1.,1.),(1.,1.),(1.,1.),(1.,1.),(1.,
1.),(1.,1.),(1.,1.),(1.,1.),(1.,1.),(1.,1.),(1.,1.),(1.,1.),(1.,1.),(1.,
1.),(1.,1.),(1.,1.),(1.,1.),(1.,1.),(1.,1.),(1.,1.),(1.,1.),(1.,1.),(1.,
1.),(1.,1.),(1.,1.),(1.,1.),(1.,1.),(1.,1.),(1.,1.),(1.,1.),(1.,1.),(1.,
1.),(1.,1.),(1.,1.),(1.,1.),(1.,1.),(1.,1.),(1.,1.),(1.,1.),(1.,1.),(1.,
1.),(1.,1.)))
REPRESENTATION_ITEM('')
SURFACE()
);
#156=(
BOUNDED_SURFACE()
B_SPLINE_SURFACE(5,1,((#69841,#69842),(#69843,#69844),(#69845,#69846),(#69847,
#69848),(#69849,#69850),(#69851,#69852),(#69853,#69854),(#69855,#69856),
(#69857,#69858),(#69859,#69860),(#69861,#69862),(#69863,#69864),(#69865,
#69866),(#69867,#69868),(#69869,#69870),(#69871,#69872),(#69873,#69874),
(#69875,#69876),(#69877,#69878),(#69879,#69880),(#69881,#69882),(#69883,
#69884),(#69885,#69886),(#69887,#69888),(#69889,#69890),(#69891,#69892),
(#69893,#69894),(#69895,#69896),(#69897,#69898),(#69899,#69900),(#69901,
#69902),(#69903,#69904),(#69905,#69906),(#69907,#69908),(#69909,#69910),
(#69911,#69912),(#69913,#69914),(#69915,#69916),(#69917,#69918),(#69919,
#69920),(#69921,#69922),(#69923,#69924),(#69925,#69926),(#69927,#69928),
(#69929,#69930),(#69931,#69932),(#69933,#69934),(#69935,#69936),(#69937,
#69938),(#69939,#69940),(#69941,#69942),(#69943,#69944),(#69945,#69946),
(#69947,#69948),(#69949,#69950),(#69951,#69952),(#69953,#69954),(#69955,
#69956),(#69957,#69958),(#69959,#69960),(#69961,#69962),(#69963,#69964),
(#69965,#69966),(#69967,#69968),(#69969,#69970),(#69971,#69972),(#69973,
#69974),(#69975,#69976),(#69977,#69978),(#69979,#69980)),.UNSPECIFIED.,
 .F.,.F.,.F.)
B_SPLINE_SURFACE_WITH_KNOTS((6,1,1,1,1,1,1,1,1,1,1,1,1,1,1,1,1,1,1,1,1,
1,1,1,1,1,1,1,1,1,1,1,1,1,1,1,1,1,1,1,1,1,1,1,1,1,1,1,1,1,1,1,1,1,1,1,1,
1,1,1,1,1,1,1,1,6),(2,2),(-1.,-0.984615384615383,-0.969230769230768,-0.953846153846152,
-0.938461538461537,-0.923076923076922,-0.907692307692306,-0.892307692307691,
-0.876923076923076,-0.86153846153846,-0.846153846153845,-0.83076923076923,
-0.815384615384614,-0.799999999999999,-0.784615384615384,-0.769230769230768,
-0.753846153846153,-0.738461538461538,-0.723076923076922,-0.707692307692307,
-0.692307692307692,-0.676923076923076,-0.661538461538461,-0.646153846153846,
-0.63076923076923,-0.615384615384615,-0.6,-0.584615384615384,-0.569230769230769,
-0.553846153846154,-0.538461538461538,-0.523076923076923,-0.507692307692308,
-0.492307692307692,-0.476923076923077,-0.461538461538462,-0.446153846153846,
-0.430769230769231,-0.415384615384615,-0.4,-0.384615384615385,-0.369230769230769,
-0.353846153846154,-0.338461538461538,-0.323076923076923,-0.307692307692308,
-0.292307692307692,-0.276923076923077,-0.261538461538462,-0.246153846153846,
-0.230769230769231,-0.215384615384615,-0.2,-0.184615384615385,-0.169230769230769,
-0.153846153846154,-0.138461538461538,-0.123076923076923,-0.107692307692308,
-0.0923076923076923,-0.0769230769230769,-0.0615384615384615,-0.0461538461538462,
-0.0307692307692308,-0.0153846153846154,0.),(-1.,1.),.UNSPECIFIED.)
GEOMETRIC_REPRESENTATION_ITEM()
RATIONAL_B_SPLINE_SURFACE(((1.,1.),(1.,1.),(1.,1.),(1.,1.),(1.,1.),(1.,
1.),(1.,1.),(1.,1.),(1.,1.),(1.,1.),(1.,1.),(1.,1.),(1.,1.),(1.,1.),(1.,
1.),(1.,1.),(1.,1.),(1.,1.),(1.,1.),(1.,1.),(1.,1.),(1.,1.),(1.,1.),(1.,
1.),(1.,1.),(1.,1.),(1.,1.),(1.,1.),(1.,1.),(1.,1.),(1.,1.),(1.,1.),(1.,
1.),(1.,1.),(1.,1.),(1.,1.),(1.,1.),(1.,1.),(1.,1.),(1.,1.),(1.,1.),(1.,
1.),(1.,1.),(1.,1.),(1.,1.),(1.,1.),(1.,1.),(1.,1.),(1.,1.),(1.,1.),(1.,
1.),(1.,1.),(1.,1.),(1.,1.),(1.,1.),(1.,1.),(1.,1.),(1.,1.),(1.,1.),(1.,
1.),(1.,1.),(1.,1.),(1.,1.),(1.,1.),(1.,1.),(1.,1.),(1.,1.),(1.,1.),(1.,
1.),(1.,1.)))
REPRESENTATION_ITEM('')
SURFACE()
);
#157=(
BOUNDED_SURFACE()
B_SPLINE_SURFACE(5,1,((#70071,#70072),(#70073,#70074),(#70075,#70076),(#70077,
#70078),(#70079,#70080),(#70081,#70082),(#70083,#70084),(#70085,#70086),
(#70087,#70088),(#70089,#70090),(#70091,#70092),(#70093,#70094),(#70095,
#70096),(#70097,#70098),(#70099,#70100),(#70101,#70102),(#70103,#70104),
(#70105,#70106),(#70107,#70108),(#70109,#70110),(#70111,#70112),(#70113,
#70114),(#70115,#70116),(#70117,#70118),(#70119,#70120),(#70121,#70122),
(#70123,#70124),(#70125,#70126),(#70127,#70128),(#70129,#70130),(#70131,
#70132),(#70133,#70134),(#70135,#70136),(#70137,#70138),(#70139,#70140),
(#70141,#70142),(#70143,#70144),(#70145,#70146),(#70147,#70148),(#70149,
#70150),(#70151,#70152),(#70153,#70154),(#70155,#70156),(#70157,#70158),
(#70159,#70160),(#70161,#70162),(#70163,#70164),(#70165,#70166),(#70167,
#70168),(#70169,#70170),(#70171,#70172),(#70173,#70174),(#70175,#70176),
(#70177,#70178),(#70179,#70180),(#70181,#70182),(#70183,#70184),(#70185,
#70186),(#70187,#70188),(#70189,#70190),(#70191,#70192),(#70193,#70194),
(#70195,#70196),(#70197,#70198),(#70199,#70200),(#70201,#70202),(#70203,
#70204),(#70205,#70206),(#70207,#70208),(#70209,#70210)),.UNSPECIFIED.,
 .F.,.F.,.F.)
B_SPLINE_SURFACE_WITH_KNOTS((6,1,1,1,1,1,1,1,1,1,1,1,1,1,1,1,1,1,1,1,1,
1,1,1,1,1,1,1,1,1,1,1,1,1,1,1,1,1,1,1,1,1,1,1,1,1,1,1,1,1,1,1,1,1,1,1,1,
1,1,1,1,1,1,1,1,6),(2,2),(-1.,-0.984615384615383,-0.969230769230768,-0.953846153846152,
-0.938461538461537,-0.923076923076922,-0.907692307692306,-0.892307692307691,
-0.876923076923076,-0.86153846153846,-0.846153846153845,-0.83076923076923,
-0.815384615384614,-0.799999999999999,-0.784615384615384,-0.769230769230768,
-0.753846153846153,-0.738461538461538,-0.723076923076922,-0.707692307692307,
-0.692307692307692,-0.676923076923076,-0.661538461538461,-0.646153846153846,
-0.63076923076923,-0.615384615384615,-0.6,-0.584615384615384,-0.569230769230769,
-0.553846153846154,-0.538461538461538,-0.523076923076923,-0.507692307692308,
-0.492307692307692,-0.476923076923077,-0.461538461538462,-0.446153846153846,
-0.430769230769231,-0.415384615384615,-0.4,-0.384615384615385,-0.369230769230769,
-0.353846153846154,-0.338461538461538,-0.323076923076923,-0.307692307692308,
-0.292307692307692,-0.276923076923077,-0.261538461538462,-0.246153846153846,
-0.230769230769231,-0.215384615384615,-0.2,-0.184615384615385,-0.169230769230769,
-0.153846153846154,-0.138461538461538,-0.123076923076923,-0.107692307692308,
-0.0923076923076923,-0.0769230769230769,-0.0615384615384615,-0.0461538461538462,
-0.0307692307692308,-0.0153846153846154,0.),(-1.,1.),.UNSPECIFIED.)
GEOMETRIC_REPRESENTATION_ITEM()
RATIONAL_B_SPLINE_SURFACE(((1.,1.),(1.,1.),(1.,1.),(1.,1.),(1.,1.),(1.,
1.),(1.,1.),(1.,1.),(1.,1.),(1.,1.),(1.,1.),(1.,1.),(1.,1.),(1.,1.),(1.,
1.),(1.,1.),(1.,1.),(1.,1.),(1.,1.),(1.,1.),(1.,1.),(1.,1.),(1.,1.),(1.,
1.),(1.,1.),(1.,1.),(1.,1.),(1.,1.),(1.,1.),(1.,1.),(1.,1.),(1.,1.),(1.,
1.),(1.,1.),(1.,1.),(1.,1.),(1.,1.),(1.,1.),(1.,1.),(1.,1.),(1.,1.),(1.,
1.),(1.,1.),(1.,1.),(1.,1.),(1.,1.),(1.,1.),(1.,1.),(1.,1.),(1.,1.),(1.,
1.),(1.,1.),(1.,1.),(1.,1.),(1.,1.),(1.,1.),(1.,1.),(1.,1.),(1.,1.),(1.,
1.),(1.,1.),(1.,1.),(1.,1.),(1.,1.),(1.,1.),(1.,1.),(1.,1.),(1.,1.),(1.,
1.),(1.,1.)))
REPRESENTATION_ITEM('')
SURFACE()
);
#158=(
BOUNDED_SURFACE()
B_SPLINE_SURFACE(5,1,((#70283,#70284),(#70285,#70286),(#70287,#70288),(#70289,
#70290),(#70291,#70292),(#70293,#70294),(#70295,#70296),(#70297,#70298),
(#70299,#70300),(#70301,#70302),(#70303,#70304),(#70305,#70306),(#70307,
#70308),(#70309,#70310),(#70311,#70312),(#70313,#70314),(#70315,#70316),
(#70317,#70318),(#70319,#70320),(#70321,#70322),(#70323,#70324),(#70325,
#70326),(#70327,#70328),(#70329,#70330),(#70331,#70332),(#70333,#70334),
(#70335,#70336),(#70337,#70338),(#70339,#70340),(#70341,#70342),(#70343,
#70344),(#70345,#70346),(#70347,#70348),(#70349,#70350),(#70351,#70352),
(#70353,#70354),(#70355,#70356),(#70357,#70358),(#70359,#70360),(#70361,
#70362),(#70363,#70364),(#70365,#70366),(#70367,#70368),(#70369,#70370),
(#70371,#70372),(#70373,#70374),(#70375,#70376),(#70377,#70378),(#70379,
#70380),(#70381,#70382),(#70383,#70384),(#70385,#70386),(#70387,#70388),
(#70389,#70390),(#70391,#70392),(#70393,#70394),(#70395,#70396),(#70397,
#70398),(#70399,#70400),(#70401,#70402),(#70403,#70404),(#70405,#70406),
(#70407,#70408),(#70409,#70410),(#70411,#70412),(#70413,#70414),(#70415,
#70416),(#70417,#70418),(#70419,#70420),(#70421,#70422)),.UNSPECIFIED.,
 .F.,.F.,.F.)
B_SPLINE_SURFACE_WITH_KNOTS((6,1,1,1,1,1,1,1,1,1,1,1,1,1,1,1,1,1,1,1,1,
1,1,1,1,1,1,1,1,1,1,1,1,1,1,1,1,1,1,1,1,1,1,1,1,1,1,1,1,1,1,1,1,1,1,1,1,
1,1,1,1,1,1,1,1,6),(2,2),(-1.,-0.984615384615383,-0.969230769230768,-0.953846153846152,
-0.938461538461537,-0.923076923076922,-0.907692307692306,-0.892307692307691,
-0.876923076923076,-0.86153846153846,-0.846153846153845,-0.83076923076923,
-0.815384615384614,-0.799999999999999,-0.784615384615384,-0.769230769230768,
-0.753846153846153,-0.738461538461538,-0.723076923076922,-0.707692307692307,
-0.692307692307692,-0.676923076923076,-0.661538461538461,-0.646153846153846,
-0.63076923076923,-0.615384615384615,-0.6,-0.584615384615384,-0.569230769230769,
-0.553846153846154,-0.538461538461538,-0.523076923076923,-0.507692307692308,
-0.492307692307692,-0.476923076923077,-0.461538461538462,-0.446153846153846,
-0.430769230769231,-0.415384615384615,-0.4,-0.384615384615385,-0.369230769230769,
-0.353846153846154,-0.338461538461538,-0.323076923076923,-0.307692307692308,
-0.292307692307692,-0.276923076923077,-0.261538461538462,-0.246153846153846,
-0.230769230769231,-0.215384615384615,-0.2,-0.184615384615385,-0.169230769230769,
-0.153846153846154,-0.138461538461538,-0.123076923076923,-0.107692307692308,
-0.0923076923076923,-0.0769230769230769,-0.0615384615384615,-0.0461538461538462,
-0.0307692307692308,-0.0153846153846154,0.),(-1.,1.),.UNSPECIFIED.)
GEOMETRIC_REPRESENTATION_ITEM()
RATIONAL_B_SPLINE_SURFACE(((1.,1.),(1.,1.),(1.,1.),(1.,1.),(1.,1.),(1.,
1.),(1.,1.),(1.,1.),(1.,1.),(1.,1.),(1.,1.),(1.,1.),(1.,1.),(1.,1.),(1.,
1.),(1.,1.),(1.,1.),(1.,1.),(1.,1.),(1.,1.),(1.,1.),(1.,1.),(1.,1.),(1.,
1.),(1.,1.),(1.,1.),(1.,1.),(1.,1.),(1.,1.),(1.,1.),(1.,1.),(1.,1.),(1.,
1.),(1.,1.),(1.,1.),(1.,1.),(1.,1.),(1.,1.),(1.,1.),(1.,1.),(1.,1.),(1.,
1.),(1.,1.),(1.,1.),(1.,1.),(1.,1.),(1.,1.),(1.,1.),(1.,1.),(1.,1.),(1.,
1.),(1.,1.),(1.,1.),(1.,1.),(1.,1.),(1.,1.),(1.,1.),(1.,1.),(1.,1.),(1.,
1.),(1.,1.),(1.,1.),(1.,1.),(1.,1.),(1.,1.),(1.,1.),(1.,1.),(1.,1.),(1.,
1.),(1.,1.)))
REPRESENTATION_ITEM('')
SURFACE()
);
#159=(
BOUNDED_SURFACE()
B_SPLINE_SURFACE(5,1,((#70513,#70514),(#70515,#70516),(#70517,#70518),(#70519,
#70520),(#70521,#70522),(#70523,#70524),(#70525,#70526),(#70527,#70528),
(#70529,#70530),(#70531,#70532),(#70533,#70534),(#70535,#70536),(#70537,
#70538),(#70539,#70540),(#70541,#70542),(#70543,#70544),(#70545,#70546),
(#70547,#70548),(#70549,#70550),(#70551,#70552),(#70553,#70554),(#70555,
#70556),(#70557,#70558),(#70559,#70560),(#70561,#70562),(#70563,#70564),
(#70565,#70566),(#70567,#70568),(#70569,#70570),(#70571,#70572),(#70573,
#70574),(#70575,#70576),(#70577,#70578),(#70579,#70580),(#70581,#70582),
(#70583,#70584),(#70585,#70586),(#70587,#70588),(#70589,#70590),(#70591,
#70592),(#70593,#70594),(#70595,#70596),(#70597,#70598),(#70599,#70600),
(#70601,#70602),(#70603,#70604),(#70605,#70606),(#70607,#70608),(#70609,
#70610),(#70611,#70612),(#70613,#70614),(#70615,#70616),(#70617,#70618),
(#70619,#70620),(#70621,#70622),(#70623,#70624),(#70625,#70626),(#70627,
#70628),(#70629,#70630),(#70631,#70632),(#70633,#70634),(#70635,#70636),
(#70637,#70638),(#70639,#70640),(#70641,#70642),(#70643,#70644),(#70645,
#70646),(#70647,#70648),(#70649,#70650),(#70651,#70652)),.UNSPECIFIED.,
 .F.,.F.,.F.)
B_SPLINE_SURFACE_WITH_KNOTS((6,1,1,1,1,1,1,1,1,1,1,1,1,1,1,1,1,1,1,1,1,
1,1,1,1,1,1,1,1,1,1,1,1,1,1,1,1,1,1,1,1,1,1,1,1,1,1,1,1,1,1,1,1,1,1,1,1,
1,1,1,1,1,1,1,1,6),(2,2),(-1.,-0.984615384615383,-0.969230769230768,-0.953846153846152,
-0.938461538461537,-0.923076923076922,-0.907692307692306,-0.892307692307691,
-0.876923076923076,-0.86153846153846,-0.846153846153845,-0.83076923076923,
-0.815384615384614,-0.799999999999999,-0.784615384615384,-0.769230769230768,
-0.753846153846153,-0.738461538461538,-0.723076923076922,-0.707692307692307,
-0.692307692307692,-0.676923076923076,-0.661538461538461,-0.646153846153846,
-0.63076923076923,-0.615384615384615,-0.6,-0.584615384615384,-0.569230769230769,
-0.553846153846154,-0.538461538461538,-0.523076923076923,-0.507692307692308,
-0.492307692307692,-0.476923076923077,-0.461538461538462,-0.446153846153846,
-0.430769230769231,-0.415384615384615,-0.4,-0.384615384615385,-0.369230769230769,
-0.353846153846154,-0.338461538461538,-0.323076923076923,-0.307692307692308,
-0.292307692307692,-0.276923076923077,-0.261538461538462,-0.246153846153846,
-0.230769230769231,-0.215384615384615,-0.2,-0.184615384615385,-0.169230769230769,
-0.153846153846154,-0.138461538461538,-0.123076923076923,-0.107692307692308,
-0.0923076923076923,-0.0769230769230769,-0.0615384615384615,-0.0461538461538462,
-0.0307692307692308,-0.0153846153846154,0.),(-1.,1.),.UNSPECIFIED.)
GEOMETRIC_REPRESENTATION_ITEM()
RATIONAL_B_SPLINE_SURFACE(((1.,1.),(1.,1.),(1.,1.),(1.,1.),(1.,1.),(1.,
1.),(1.,1.),(1.,1.),(1.,1.),(1.,1.),(1.,1.),(1.,1.),(1.,1.),(1.,1.),(1.,
1.),(1.,1.),(1.,1.),(1.,1.),(1.,1.),(1.,1.),(1.,1.),(1.,1.),(1.,1.),(1.,
1.),(1.,1.),(1.,1.),(1.,1.),(1.,1.),(1.,1.),(1.,1.),(1.,1.),(1.,1.),(1.,
1.),(1.,1.),(1.,1.),(1.,1.),(1.,1.),(1.,1.),(1.,1.),(1.,1.),(1.,1.),(1.,
1.),(1.,1.),(1.,1.),(1.,1.),(1.,1.),(1.,1.),(1.,1.),(1.,1.),(1.,1.),(1.,
1.),(1.,1.),(1.,1.),(1.,1.),(1.,1.),(1.,1.),(1.,1.),(1.,1.),(1.,1.),(1.,
1.),(1.,1.),(1.,1.),(1.,1.),(1.,1.),(1.,1.),(1.,1.),(1.,1.),(1.,1.),(1.,
1.),(1.,1.)))
REPRESENTATION_ITEM('')
SURFACE()
);
#160=(
BOUNDED_SURFACE()
B_SPLINE_SURFACE(5,1,((#70725,#70726),(#70727,#70728),(#70729,#70730),(#70731,
#70732),(#70733,#70734),(#70735,#70736),(#70737,#70738),(#70739,#70740),
(#70741,#70742),(#70743,#70744),(#70745,#70746),(#70747,#70748),(#70749,
#70750),(#70751,#70752),(#70753,#70754),(#70755,#70756),(#70757,#70758),
(#70759,#70760),(#70761,#70762),(#70763,#70764),(#70765,#70766),(#70767,
#70768),(#70769,#70770),(#70771,#70772),(#70773,#70774),(#70775,#70776),
(#70777,#70778),(#70779,#70780),(#70781,#70782),(#70783,#70784),(#70785,
#70786),(#70787,#70788),(#70789,#70790),(#70791,#70792),(#70793,#70794),
(#70795,#70796),(#70797,#70798),(#70799,#70800),(#70801,#70802),(#70803,
#70804),(#70805,#70806),(#70807,#70808),(#70809,#70810),(#70811,#70812),
(#70813,#70814),(#70815,#70816),(#70817,#70818),(#70819,#70820),(#70821,
#70822),(#70823,#70824),(#70825,#70826),(#70827,#70828),(#70829,#70830),
(#70831,#70832),(#70833,#70834),(#70835,#70836),(#70837,#70838),(#70839,
#70840),(#70841,#70842),(#70843,#70844),(#70845,#70846),(#70847,#70848),
(#70849,#70850),(#70851,#70852),(#70853,#70854),(#70855,#70856),(#70857,
#70858),(#70859,#70860),(#70861,#70862),(#70863,#70864)),.UNSPECIFIED.,
 .F.,.F.,.F.)
B_SPLINE_SURFACE_WITH_KNOTS((6,1,1,1,1,1,1,1,1,1,1,1,1,1,1,1,1,1,1,1,1,
1,1,1,1,1,1,1,1,1,1,1,1,1,1,1,1,1,1,1,1,1,1,1,1,1,1,1,1,1,1,1,1,1,1,1,1,
1,1,1,1,1,1,1,1,6),(2,2),(-1.,-0.984615384615383,-0.969230769230768,-0.953846153846152,
-0.938461538461537,-0.923076923076922,-0.907692307692306,-0.892307692307691,
-0.876923076923076,-0.86153846153846,-0.846153846153845,-0.83076923076923,
-0.815384615384614,-0.799999999999999,-0.784615384615384,-0.769230769230768,
-0.753846153846153,-0.738461538461538,-0.723076923076922,-0.707692307692307,
-0.692307692307692,-0.676923076923076,-0.661538461538461,-0.646153846153846,
-0.63076923076923,-0.615384615384615,-0.6,-0.584615384615384,-0.569230769230769,
-0.553846153846154,-0.538461538461538,-0.523076923076923,-0.507692307692308,
-0.492307692307692,-0.476923076923077,-0.461538461538462,-0.446153846153846,
-0.430769230769231,-0.415384615384615,-0.4,-0.384615384615385,-0.369230769230769,
-0.353846153846154,-0.338461538461538,-0.323076923076923,-0.307692307692308,
-0.292307692307692,-0.276923076923077,-0.261538461538462,-0.246153846153846,
-0.230769230769231,-0.215384615384615,-0.2,-0.184615384615385,-0.169230769230769,
-0.153846153846154,-0.138461538461538,-0.123076923076923,-0.107692307692308,
-0.0923076923076923,-0.0769230769230769,-0.0615384615384615,-0.0461538461538462,
-0.0307692307692308,-0.0153846153846154,0.),(-1.,1.),.UNSPECIFIED.)
GEOMETRIC_REPRESENTATION_ITEM()
RATIONAL_B_SPLINE_SURFACE(((1.,1.),(1.,1.),(1.,1.),(1.,1.),(1.,1.),(1.,
1.),(1.,1.),(1.,1.),(1.,1.),(1.,1.),(1.,1.),(1.,1.),(1.,1.),(1.,1.),(1.,
1.),(1.,1.),(1.,1.),(1.,1.),(1.,1.),(1.,1.),(1.,1.),(1.,1.),(1.,1.),(1.,
1.),(1.,1.),(1.,1.),(1.,1.),(1.,1.),(1.,1.),(1.,1.),(1.,1.),(1.,1.),(1.,
1.),(1.,1.),(1.,1.),(1.,1.),(1.,1.),(1.,1.),(1.,1.),(1.,1.),(1.,1.),(1.,
1.),(1.,1.),(1.,1.),(1.,1.),(1.,1.),(1.,1.),(1.,1.),(1.,1.),(1.,1.),(1.,
1.),(1.,1.),(1.,1.),(1.,1.),(1.,1.),(1.,1.),(1.,1.),(1.,1.),(1.,1.),(1.,
1.),(1.,1.),(1.,1.),(1.,1.),(1.,1.),(1.,1.),(1.,1.),(1.,1.),(1.,1.),(1.,
1.),(1.,1.)))
REPRESENTATION_ITEM('')
SURFACE()
);
#161=(
BOUNDED_SURFACE()
B_SPLINE_SURFACE(5,1,((#70955,#70956),(#70957,#70958),(#70959,#70960),(#70961,
#70962),(#70963,#70964),(#70965,#70966),(#70967,#70968),(#70969,#70970),
(#70971,#70972),(#70973,#70974),(#70975,#70976),(#70977,#70978),(#70979,
#70980),(#70981,#70982),(#70983,#70984),(#70985,#70986),(#70987,#70988),
(#70989,#70990),(#70991,#70992),(#70993,#70994),(#70995,#70996),(#70997,
#70998),(#70999,#71000),(#71001,#71002),(#71003,#71004),(#71005,#71006),
(#71007,#71008),(#71009,#71010),(#71011,#71012),(#71013,#71014),(#71015,
#71016),(#71017,#71018),(#71019,#71020),(#71021,#71022),(#71023,#71024),
(#71025,#71026),(#71027,#71028),(#71029,#71030),(#71031,#71032),(#71033,
#71034),(#71035,#71036),(#71037,#71038),(#71039,#71040),(#71041,#71042),
(#71043,#71044),(#71045,#71046),(#71047,#71048),(#71049,#71050),(#71051,
#71052),(#71053,#71054),(#71055,#71056),(#71057,#71058),(#71059,#71060),
(#71061,#71062),(#71063,#71064),(#71065,#71066),(#71067,#71068),(#71069,
#71070),(#71071,#71072),(#71073,#71074),(#71075,#71076),(#71077,#71078),
(#71079,#71080),(#71081,#71082),(#71083,#71084),(#71085,#71086),(#71087,
#71088),(#71089,#71090),(#71091,#71092),(#71093,#71094)),.UNSPECIFIED.,
 .F.,.F.,.F.)
B_SPLINE_SURFACE_WITH_KNOTS((6,1,1,1,1,1,1,1,1,1,1,1,1,1,1,1,1,1,1,1,1,
1,1,1,1,1,1,1,1,1,1,1,1,1,1,1,1,1,1,1,1,1,1,1,1,1,1,1,1,1,1,1,1,1,1,1,1,
1,1,1,1,1,1,1,1,6),(2,2),(-1.,-0.984615384615383,-0.969230769230768,-0.953846153846152,
-0.938461538461537,-0.923076923076922,-0.907692307692306,-0.892307692307691,
-0.876923076923076,-0.86153846153846,-0.846153846153845,-0.83076923076923,
-0.815384615384614,-0.799999999999999,-0.784615384615384,-0.769230769230768,
-0.753846153846153,-0.738461538461538,-0.723076923076922,-0.707692307692307,
-0.692307692307692,-0.676923076923076,-0.661538461538461,-0.646153846153846,
-0.63076923076923,-0.615384615384615,-0.6,-0.584615384615384,-0.569230769230769,
-0.553846153846154,-0.538461538461538,-0.523076923076923,-0.507692307692308,
-0.492307692307692,-0.476923076923077,-0.461538461538462,-0.446153846153846,
-0.430769230769231,-0.415384615384615,-0.4,-0.384615384615385,-0.369230769230769,
-0.353846153846154,-0.338461538461538,-0.323076923076923,-0.307692307692308,
-0.292307692307692,-0.276923076923077,-0.261538461538462,-0.246153846153846,
-0.230769230769231,-0.215384615384615,-0.2,-0.184615384615385,-0.169230769230769,
-0.153846153846154,-0.138461538461538,-0.123076923076923,-0.107692307692308,
-0.0923076923076923,-0.0769230769230769,-0.0615384615384615,-0.0461538461538462,
-0.0307692307692308,-0.0153846153846154,0.),(-1.,1.),.UNSPECIFIED.)
GEOMETRIC_REPRESENTATION_ITEM()
RATIONAL_B_SPLINE_SURFACE(((1.,1.),(1.,1.),(1.,1.),(1.,1.),(1.,1.),(1.,
1.),(1.,1.),(1.,1.),(1.,1.),(1.,1.),(1.,1.),(1.,1.),(1.,1.),(1.,1.),(1.,
1.),(1.,1.),(1.,1.),(1.,1.),(1.,1.),(1.,1.),(1.,1.),(1.,1.),(1.,1.),(1.,
1.),(1.,1.),(1.,1.),(1.,1.),(1.,1.),(1.,1.),(1.,1.),(1.,1.),(1.,1.),(1.,
1.),(1.,1.),(1.,1.),(1.,1.),(1.,1.),(1.,1.),(1.,1.),(1.,1.),(1.,1.),(1.,
1.),(1.,1.),(1.,1.),(1.,1.),(1.,1.),(1.,1.),(1.,1.),(1.,1.),(1.,1.),(1.,
1.),(1.,1.),(1.,1.),(1.,1.),(1.,1.),(1.,1.),(1.,1.),(1.,1.),(1.,1.),(1.,
1.),(1.,1.),(1.,1.),(1.,1.),(1.,1.),(1.,1.),(1.,1.),(1.,1.),(1.,1.),(1.,
1.),(1.,1.)))
REPRESENTATION_ITEM('')
SURFACE()
);
#162=(
BOUNDED_SURFACE()
B_SPLINE_SURFACE(5,1,((#71167,#71168),(#71169,#71170),(#71171,#71172),(#71173,
#71174),(#71175,#71176),(#71177,#71178),(#71179,#71180),(#71181,#71182),
(#71183,#71184),(#71185,#71186),(#71187,#71188),(#71189,#71190),(#71191,
#71192),(#71193,#71194),(#71195,#71196),(#71197,#71198),(#71199,#71200),
(#71201,#71202),(#71203,#71204),(#71205,#71206),(#71207,#71208),(#71209,
#71210),(#71211,#71212),(#71213,#71214),(#71215,#71216),(#71217,#71218),
(#71219,#71220),(#71221,#71222),(#71223,#71224),(#71225,#71226),(#71227,
#71228),(#71229,#71230),(#71231,#71232),(#71233,#71234),(#71235,#71236),
(#71237,#71238),(#71239,#71240),(#71241,#71242),(#71243,#71244),(#71245,
#71246),(#71247,#71248),(#71249,#71250),(#71251,#71252),(#71253,#71254),
(#71255,#71256),(#71257,#71258),(#71259,#71260),(#71261,#71262),(#71263,
#71264),(#71265,#71266),(#71267,#71268),(#71269,#71270),(#71271,#71272),
(#71273,#71274),(#71275,#71276),(#71277,#71278),(#71279,#71280),(#71281,
#71282),(#71283,#71284),(#71285,#71286),(#71287,#71288),(#71289,#71290),
(#71291,#71292),(#71293,#71294),(#71295,#71296),(#71297,#71298),(#71299,
#71300),(#71301,#71302),(#71303,#71304),(#71305,#71306)),.UNSPECIFIED.,
 .F.,.F.,.F.)
B_SPLINE_SURFACE_WITH_KNOTS((6,1,1,1,1,1,1,1,1,1,1,1,1,1,1,1,1,1,1,1,1,
1,1,1,1,1,1,1,1,1,1,1,1,1,1,1,1,1,1,1,1,1,1,1,1,1,1,1,1,1,1,1,1,1,1,1,1,
1,1,1,1,1,1,1,1,6),(2,2),(-1.,-0.984615384615383,-0.969230769230768,-0.953846153846152,
-0.938461538461537,-0.923076923076922,-0.907692307692306,-0.892307692307691,
-0.876923076923076,-0.86153846153846,-0.846153846153845,-0.83076923076923,
-0.815384615384614,-0.799999999999999,-0.784615384615384,-0.769230769230768,
-0.753846153846153,-0.738461538461538,-0.723076923076922,-0.707692307692307,
-0.692307692307692,-0.676923076923076,-0.661538461538461,-0.646153846153846,
-0.63076923076923,-0.615384615384615,-0.6,-0.584615384615384,-0.569230769230769,
-0.553846153846154,-0.538461538461538,-0.523076923076923,-0.507692307692308,
-0.492307692307692,-0.476923076923077,-0.461538461538462,-0.446153846153846,
-0.430769230769231,-0.415384615384615,-0.4,-0.384615384615385,-0.369230769230769,
-0.353846153846154,-0.338461538461538,-0.323076923076923,-0.307692307692308,
-0.292307692307692,-0.276923076923077,-0.261538461538462,-0.246153846153846,
-0.230769230769231,-0.215384615384615,-0.2,-0.184615384615385,-0.169230769230769,
-0.153846153846154,-0.138461538461538,-0.123076923076923,-0.107692307692308,
-0.0923076923076923,-0.0769230769230769,-0.0615384615384615,-0.0461538461538462,
-0.0307692307692308,-0.0153846153846154,0.),(-1.,1.),.UNSPECIFIED.)
GEOMETRIC_REPRESENTATION_ITEM()
RATIONAL_B_SPLINE_SURFACE(((1.,1.),(1.,1.),(1.,1.),(1.,1.),(1.,1.),(1.,
1.),(1.,1.),(1.,1.),(1.,1.),(1.,1.),(1.,1.),(1.,1.),(1.,1.),(1.,1.),(1.,
1.),(1.,1.),(1.,1.),(1.,1.),(1.,1.),(1.,1.),(1.,1.),(1.,1.),(1.,1.),(1.,
1.),(1.,1.),(1.,1.),(1.,1.),(1.,1.),(1.,1.),(1.,1.),(1.,1.),(1.,1.),(1.,
1.),(1.,1.),(1.,1.),(1.,1.),(1.,1.),(1.,1.),(1.,1.),(1.,1.),(1.,1.),(1.,
1.),(1.,1.),(1.,1.),(1.,1.),(1.,1.),(1.,1.),(1.,1.),(1.,1.),(1.,1.),(1.,
1.),(1.,1.),(1.,1.),(1.,1.),(1.,1.),(1.,1.),(1.,1.),(1.,1.),(1.,1.),(1.,
1.),(1.,1.),(1.,1.),(1.,1.),(1.,1.),(1.,1.),(1.,1.),(1.,1.),(1.,1.),(1.,
1.),(1.,1.)))
REPRESENTATION_ITEM('')
SURFACE()
);
#163=(
BOUNDED_SURFACE()
B_SPLINE_SURFACE(5,1,((#71397,#71398),(#71399,#71400),(#71401,#71402),(#71403,
#71404),(#71405,#71406),(#71407,#71408),(#71409,#71410),(#71411,#71412),
(#71413,#71414),(#71415,#71416),(#71417,#71418),(#71419,#71420),(#71421,
#71422),(#71423,#71424),(#71425,#71426),(#71427,#71428),(#71429,#71430),
(#71431,#71432),(#71433,#71434),(#71435,#71436),(#71437,#71438),(#71439,
#71440),(#71441,#71442),(#71443,#71444),(#71445,#71446),(#71447,#71448),
(#71449,#71450),(#71451,#71452),(#71453,#71454),(#71455,#71456),(#71457,
#71458),(#71459,#71460),(#71461,#71462),(#71463,#71464),(#71465,#71466),
(#71467,#71468),(#71469,#71470),(#71471,#71472),(#71473,#71474),(#71475,
#71476),(#71477,#71478),(#71479,#71480),(#71481,#71482),(#71483,#71484),
(#71485,#71486),(#71487,#71488),(#71489,#71490),(#71491,#71492),(#71493,
#71494),(#71495,#71496),(#71497,#71498),(#71499,#71500),(#71501,#71502),
(#71503,#71504),(#71505,#71506),(#71507,#71508),(#71509,#71510),(#71511,
#71512),(#71513,#71514),(#71515,#71516),(#71517,#71518),(#71519,#71520),
(#71521,#71522),(#71523,#71524),(#71525,#71526),(#71527,#71528),(#71529,
#71530),(#71531,#71532),(#71533,#71534),(#71535,#71536)),.UNSPECIFIED.,
 .F.,.F.,.F.)
B_SPLINE_SURFACE_WITH_KNOTS((6,1,1,1,1,1,1,1,1,1,1,1,1,1,1,1,1,1,1,1,1,
1,1,1,1,1,1,1,1,1,1,1,1,1,1,1,1,1,1,1,1,1,1,1,1,1,1,1,1,1,1,1,1,1,1,1,1,
1,1,1,1,1,1,1,1,6),(2,2),(-1.,-0.984615384615383,-0.969230769230768,-0.953846153846152,
-0.938461538461537,-0.923076923076922,-0.907692307692306,-0.892307692307691,
-0.876923076923076,-0.86153846153846,-0.846153846153845,-0.83076923076923,
-0.815384615384614,-0.799999999999999,-0.784615384615384,-0.769230769230768,
-0.753846153846153,-0.738461538461538,-0.723076923076922,-0.707692307692307,
-0.692307692307692,-0.676923076923076,-0.661538461538461,-0.646153846153846,
-0.63076923076923,-0.615384615384615,-0.6,-0.584615384615384,-0.569230769230769,
-0.553846153846154,-0.538461538461538,-0.523076923076923,-0.507692307692308,
-0.492307692307692,-0.476923076923077,-0.461538461538462,-0.446153846153846,
-0.430769230769231,-0.415384615384615,-0.4,-0.384615384615385,-0.369230769230769,
-0.353846153846154,-0.338461538461538,-0.323076923076923,-0.307692307692308,
-0.292307692307692,-0.276923076923077,-0.261538461538462,-0.246153846153846,
-0.230769230769231,-0.215384615384615,-0.2,-0.184615384615385,-0.169230769230769,
-0.153846153846154,-0.138461538461538,-0.123076923076923,-0.107692307692308,
-0.0923076923076923,-0.0769230769230769,-0.0615384615384615,-0.0461538461538462,
-0.0307692307692308,-0.0153846153846154,0.),(-1.,1.),.UNSPECIFIED.)
GEOMETRIC_REPRESENTATION_ITEM()
RATIONAL_B_SPLINE_SURFACE(((1.,1.),(1.,1.),(1.,1.),(1.,1.),(1.,1.),(1.,
1.),(1.,1.),(1.,1.),(1.,1.),(1.,1.),(1.,1.),(1.,1.),(1.,1.),(1.,1.),(1.,
1.),(1.,1.),(1.,1.),(1.,1.),(1.,1.),(1.,1.),(1.,1.),(1.,1.),(1.,1.),(1.,
1.),(1.,1.),(1.,1.),(1.,1.),(1.,1.),(1.,1.),(1.,1.),(1.,1.),(1.,1.),(1.,
1.),(1.,1.),(1.,1.),(1.,1.),(1.,1.),(1.,1.),(1.,1.),(1.,1.),(1.,1.),(1.,
1.),(1.,1.),(1.,1.),(1.,1.),(1.,1.),(1.,1.),(1.,1.),(1.,1.),(1.,1.),(1.,
1.),(1.,1.),(1.,1.),(1.,1.),(1.,1.),(1.,1.),(1.,1.),(1.,1.),(1.,1.),(1.,
1.),(1.,1.),(1.,1.),(1.,1.),(1.,1.),(1.,1.),(1.,1.),(1.,1.),(1.,1.),(1.,
1.),(1.,1.)))
REPRESENTATION_ITEM('')
SURFACE()
);
#164=(
BOUNDED_SURFACE()
B_SPLINE_SURFACE(5,1,((#71609,#71610),(#71611,#71612),(#71613,#71614),(#71615,
#71616),(#71617,#71618),(#71619,#71620),(#71621,#71622),(#71623,#71624),
(#71625,#71626),(#71627,#71628),(#71629,#71630),(#71631,#71632),(#71633,
#71634),(#71635,#71636),(#71637,#71638),(#71639,#71640),(#71641,#71642),
(#71643,#71644),(#71645,#71646),(#71647,#71648),(#71649,#71650),(#71651,
#71652),(#71653,#71654),(#71655,#71656),(#71657,#71658),(#71659,#71660),
(#71661,#71662),(#71663,#71664),(#71665,#71666),(#71667,#71668),(#71669,
#71670),(#71671,#71672),(#71673,#71674),(#71675,#71676),(#71677,#71678),
(#71679,#71680),(#71681,#71682),(#71683,#71684),(#71685,#71686),(#71687,
#71688),(#71689,#71690),(#71691,#71692),(#71693,#71694),(#71695,#71696),
(#71697,#71698),(#71699,#71700),(#71701,#71702),(#71703,#71704),(#71705,
#71706),(#71707,#71708),(#71709,#71710),(#71711,#71712),(#71713,#71714),
(#71715,#71716),(#71717,#71718),(#71719,#71720),(#71721,#71722),(#71723,
#71724),(#71725,#71726),(#71727,#71728),(#71729,#71730),(#71731,#71732),
(#71733,#71734),(#71735,#71736),(#71737,#71738),(#71739,#71740),(#71741,
#71742),(#71743,#71744),(#71745,#71746),(#71747,#71748)),.UNSPECIFIED.,
 .F.,.F.,.F.)
B_SPLINE_SURFACE_WITH_KNOTS((6,1,1,1,1,1,1,1,1,1,1,1,1,1,1,1,1,1,1,1,1,
1,1,1,1,1,1,1,1,1,1,1,1,1,1,1,1,1,1,1,1,1,1,1,1,1,1,1,1,1,1,1,1,1,1,1,1,
1,1,1,1,1,1,1,1,6),(2,2),(-1.,-0.984615384615383,-0.969230769230768,-0.953846153846152,
-0.938461538461537,-0.923076923076922,-0.907692307692306,-0.892307692307691,
-0.876923076923076,-0.86153846153846,-0.846153846153845,-0.83076923076923,
-0.815384615384614,-0.799999999999999,-0.784615384615384,-0.769230769230768,
-0.753846153846153,-0.738461538461538,-0.723076923076922,-0.707692307692307,
-0.692307692307692,-0.676923076923076,-0.661538461538461,-0.646153846153846,
-0.63076923076923,-0.615384615384615,-0.6,-0.584615384615384,-0.569230769230769,
-0.553846153846154,-0.538461538461538,-0.523076923076923,-0.507692307692308,
-0.492307692307692,-0.476923076923077,-0.461538461538462,-0.446153846153846,
-0.430769230769231,-0.415384615384615,-0.4,-0.384615384615385,-0.369230769230769,
-0.353846153846154,-0.338461538461538,-0.323076923076923,-0.307692307692308,
-0.292307692307692,-0.276923076923077,-0.261538461538462,-0.246153846153846,
-0.230769230769231,-0.215384615384615,-0.2,-0.184615384615385,-0.169230769230769,
-0.153846153846154,-0.138461538461538,-0.123076923076923,-0.107692307692308,
-0.0923076923076923,-0.0769230769230769,-0.0615384615384615,-0.0461538461538462,
-0.0307692307692308,-0.0153846153846154,0.),(-1.,1.),.UNSPECIFIED.)
GEOMETRIC_REPRESENTATION_ITEM()
RATIONAL_B_SPLINE_SURFACE(((1.,1.),(1.,1.),(1.,1.),(1.,1.),(1.,1.),(1.,
1.),(1.,1.),(1.,1.),(1.,1.),(1.,1.),(1.,1.),(1.,1.),(1.,1.),(1.,1.),(1.,
1.),(1.,1.),(1.,1.),(1.,1.),(1.,1.),(1.,1.),(1.,1.),(1.,1.),(1.,1.),(1.,
1.),(1.,1.),(1.,1.),(1.,1.),(1.,1.),(1.,1.),(1.,1.),(1.,1.),(1.,1.),(1.,
1.),(1.,1.),(1.,1.),(1.,1.),(1.,1.),(1.,1.),(1.,1.),(1.,1.),(1.,1.),(1.,
1.),(1.,1.),(1.,1.),(1.,1.),(1.,1.),(1.,1.),(1.,1.),(1.,1.),(1.,1.),(1.,
1.),(1.,1.),(1.,1.),(1.,1.),(1.,1.),(1.,1.),(1.,1.),(1.,1.),(1.,1.),(1.,
1.),(1.,1.),(1.,1.),(1.,1.),(1.,1.),(1.,1.),(1.,1.),(1.,1.),(1.,1.),(1.,
1.),(1.,1.)))
REPRESENTATION_ITEM('')
SURFACE()
);
#165=(
BOUNDED_SURFACE()
B_SPLINE_SURFACE(5,1,((#71839,#71840),(#71841,#71842),(#71843,#71844),(#71845,
#71846),(#71847,#71848),(#71849,#71850),(#71851,#71852),(#71853,#71854),
(#71855,#71856),(#71857,#71858),(#71859,#71860),(#71861,#71862),(#71863,
#71864),(#71865,#71866),(#71867,#71868),(#71869,#71870),(#71871,#71872),
(#71873,#71874),(#71875,#71876),(#71877,#71878),(#71879,#71880),(#71881,
#71882),(#71883,#71884),(#71885,#71886),(#71887,#71888),(#71889,#71890),
(#71891,#71892),(#71893,#71894),(#71895,#71896),(#71897,#71898),(#71899,
#71900),(#71901,#71902),(#71903,#71904),(#71905,#71906),(#71907,#71908),
(#71909,#71910),(#71911,#71912),(#71913,#71914),(#71915,#71916),(#71917,
#71918),(#71919,#71920),(#71921,#71922),(#71923,#71924),(#71925,#71926),
(#71927,#71928),(#71929,#71930),(#71931,#71932),(#71933,#71934),(#71935,
#71936),(#71937,#71938),(#71939,#71940),(#71941,#71942),(#71943,#71944),
(#71945,#71946),(#71947,#71948),(#71949,#71950),(#71951,#71952),(#71953,
#71954),(#71955,#71956),(#71957,#71958),(#71959,#71960),(#71961,#71962),
(#71963,#71964),(#71965,#71966),(#71967,#71968),(#71969,#71970),(#71971,
#71972),(#71973,#71974),(#71975,#71976),(#71977,#71978)),.UNSPECIFIED.,
 .F.,.F.,.F.)
B_SPLINE_SURFACE_WITH_KNOTS((6,1,1,1,1,1,1,1,1,1,1,1,1,1,1,1,1,1,1,1,1,
1,1,1,1,1,1,1,1,1,1,1,1,1,1,1,1,1,1,1,1,1,1,1,1,1,1,1,1,1,1,1,1,1,1,1,1,
1,1,1,1,1,1,1,1,6),(2,2),(-1.,-0.984615384615383,-0.969230769230768,-0.953846153846152,
-0.938461538461537,-0.923076923076922,-0.907692307692306,-0.892307692307691,
-0.876923076923076,-0.86153846153846,-0.846153846153845,-0.83076923076923,
-0.815384615384614,-0.799999999999999,-0.784615384615384,-0.769230769230768,
-0.753846153846153,-0.738461538461538,-0.723076923076922,-0.707692307692307,
-0.692307692307692,-0.676923076923076,-0.661538461538461,-0.646153846153846,
-0.63076923076923,-0.615384615384615,-0.6,-0.584615384615384,-0.569230769230769,
-0.553846153846154,-0.538461538461538,-0.523076923076923,-0.507692307692308,
-0.492307692307692,-0.476923076923077,-0.461538461538462,-0.446153846153846,
-0.430769230769231,-0.415384615384615,-0.4,-0.384615384615385,-0.369230769230769,
-0.353846153846154,-0.338461538461538,-0.323076923076923,-0.307692307692308,
-0.292307692307692,-0.276923076923077,-0.261538461538462,-0.246153846153846,
-0.230769230769231,-0.215384615384615,-0.2,-0.184615384615385,-0.169230769230769,
-0.153846153846154,-0.138461538461538,-0.123076923076923,-0.107692307692308,
-0.0923076923076923,-0.0769230769230769,-0.0615384615384615,-0.0461538461538462,
-0.0307692307692308,-0.0153846153846154,0.),(-1.,1.),.UNSPECIFIED.)
GEOMETRIC_REPRESENTATION_ITEM()
RATIONAL_B_SPLINE_SURFACE(((1.,1.),(1.,1.),(1.,1.),(1.,1.),(1.,1.),(1.,
1.),(1.,1.),(1.,1.),(1.,1.),(1.,1.),(1.,1.),(1.,1.),(1.,1.),(1.,1.),(1.,
1.),(1.,1.),(1.,1.),(1.,1.),(1.,1.),(1.,1.),(1.,1.),(1.,1.),(1.,1.),(1.,
1.),(1.,1.),(1.,1.),(1.,1.),(1.,1.),(1.,1.),(1.,1.),(1.,1.),(1.,1.),(1.,
1.),(1.,1.),(1.,1.),(1.,1.),(1.,1.),(1.,1.),(1.,1.),(1.,1.),(1.,1.),(1.,
1.),(1.,1.),(1.,1.),(1.,1.),(1.,1.),(1.,1.),(1.,1.),(1.,1.),(1.,1.),(1.,
1.),(1.,1.),(1.,1.),(1.,1.),(1.,1.),(1.,1.),(1.,1.),(1.,1.),(1.,1.),(1.,
1.),(1.,1.),(1.,1.),(1.,1.),(1.,1.),(1.,1.),(1.,1.),(1.,1.),(1.,1.),(1.,
1.),(1.,1.)))
REPRESENTATION_ITEM('')
SURFACE()
);
#166=(
BOUNDED_SURFACE()
B_SPLINE_SURFACE(5,1,((#72051,#72052),(#72053,#72054),(#72055,#72056),(#72057,
#72058),(#72059,#72060),(#72061,#72062),(#72063,#72064),(#72065,#72066),
(#72067,#72068),(#72069,#72070),(#72071,#72072),(#72073,#72074),(#72075,
#72076),(#72077,#72078),(#72079,#72080),(#72081,#72082),(#72083,#72084),
(#72085,#72086),(#72087,#72088),(#72089,#72090),(#72091,#72092),(#72093,
#72094),(#72095,#72096),(#72097,#72098),(#72099,#72100),(#72101,#72102),
(#72103,#72104),(#72105,#72106),(#72107,#72108),(#72109,#72110),(#72111,
#72112),(#72113,#72114),(#72115,#72116),(#72117,#72118),(#72119,#72120),
(#72121,#72122),(#72123,#72124),(#72125,#72126),(#72127,#72128),(#72129,
#72130),(#72131,#72132),(#72133,#72134),(#72135,#72136),(#72137,#72138),
(#72139,#72140),(#72141,#72142),(#72143,#72144),(#72145,#72146),(#72147,
#72148),(#72149,#72150),(#72151,#72152),(#72153,#72154),(#72155,#72156),
(#72157,#72158),(#72159,#72160),(#72161,#72162),(#72163,#72164),(#72165,
#72166),(#72167,#72168),(#72169,#72170),(#72171,#72172),(#72173,#72174),
(#72175,#72176),(#72177,#72178),(#72179,#72180),(#72181,#72182),(#72183,
#72184),(#72185,#72186),(#72187,#72188),(#72189,#72190)),.UNSPECIFIED.,
 .F.,.F.,.F.)
B_SPLINE_SURFACE_WITH_KNOTS((6,1,1,1,1,1,1,1,1,1,1,1,1,1,1,1,1,1,1,1,1,
1,1,1,1,1,1,1,1,1,1,1,1,1,1,1,1,1,1,1,1,1,1,1,1,1,1,1,1,1,1,1,1,1,1,1,1,
1,1,1,1,1,1,1,1,6),(2,2),(-1.,-0.984615384615383,-0.969230769230768,-0.953846153846152,
-0.938461538461537,-0.923076923076922,-0.907692307692306,-0.892307692307691,
-0.876923076923076,-0.86153846153846,-0.846153846153845,-0.83076923076923,
-0.815384615384614,-0.799999999999999,-0.784615384615384,-0.769230769230768,
-0.753846153846153,-0.738461538461538,-0.723076923076922,-0.707692307692307,
-0.692307692307692,-0.676923076923076,-0.661538461538461,-0.646153846153846,
-0.63076923076923,-0.615384615384615,-0.6,-0.584615384615384,-0.569230769230769,
-0.553846153846154,-0.538461538461538,-0.523076923076923,-0.507692307692308,
-0.492307692307692,-0.476923076923077,-0.461538461538462,-0.446153846153846,
-0.430769230769231,-0.415384615384615,-0.4,-0.384615384615385,-0.369230769230769,
-0.353846153846154,-0.338461538461538,-0.323076923076923,-0.307692307692308,
-0.292307692307692,-0.276923076923077,-0.261538461538462,-0.246153846153846,
-0.230769230769231,-0.215384615384615,-0.2,-0.184615384615385,-0.169230769230769,
-0.153846153846154,-0.138461538461538,-0.123076923076923,-0.107692307692308,
-0.0923076923076923,-0.0769230769230769,-0.0615384615384615,-0.0461538461538462,
-0.0307692307692308,-0.0153846153846154,0.),(-1.,1.),.UNSPECIFIED.)
GEOMETRIC_REPRESENTATION_ITEM()
RATIONAL_B_SPLINE_SURFACE(((1.,1.),(1.,1.),(1.,1.),(1.,1.),(1.,1.),(1.,
1.),(1.,1.),(1.,1.),(1.,1.),(1.,1.),(1.,1.),(1.,1.),(1.,1.),(1.,1.),(1.,
1.),(1.,1.),(1.,1.),(1.,1.),(1.,1.),(1.,1.),(1.,1.),(1.,1.),(1.,1.),(1.,
1.),(1.,1.),(1.,1.),(1.,1.),(1.,1.),(1.,1.),(1.,1.),(1.,1.),(1.,1.),(1.,
1.),(1.,1.),(1.,1.),(1.,1.),(1.,1.),(1.,1.),(1.,1.),(1.,1.),(1.,1.),(1.,
1.),(1.,1.),(1.,1.),(1.,1.),(1.,1.),(1.,1.),(1.,1.),(1.,1.),(1.,1.),(1.,
1.),(1.,1.),(1.,1.),(1.,1.),(1.,1.),(1.,1.),(1.,1.),(1.,1.),(1.,1.),(1.,
1.),(1.,1.),(1.,1.),(1.,1.),(1.,1.),(1.,1.),(1.,1.),(1.,1.),(1.,1.),(1.,
1.),(1.,1.)))
REPRESENTATION_ITEM('')
SURFACE()
);
#167=(
BOUNDED_SURFACE()
B_SPLINE_SURFACE(5,1,((#72281,#72282),(#72283,#72284),(#72285,#72286),(#72287,
#72288),(#72289,#72290),(#72291,#72292),(#72293,#72294),(#72295,#72296),
(#72297,#72298),(#72299,#72300),(#72301,#72302),(#72303,#72304),(#72305,
#72306),(#72307,#72308),(#72309,#72310),(#72311,#72312),(#72313,#72314),
(#72315,#72316),(#72317,#72318),(#72319,#72320),(#72321,#72322),(#72323,
#72324),(#72325,#72326),(#72327,#72328),(#72329,#72330),(#72331,#72332),
(#72333,#72334),(#72335,#72336),(#72337,#72338),(#72339,#72340),(#72341,
#72342),(#72343,#72344),(#72345,#72346),(#72347,#72348),(#72349,#72350),
(#72351,#72352),(#72353,#72354),(#72355,#72356),(#72357,#72358),(#72359,
#72360),(#72361,#72362),(#72363,#72364),(#72365,#72366),(#72367,#72368),
(#72369,#72370),(#72371,#72372),(#72373,#72374),(#72375,#72376),(#72377,
#72378),(#72379,#72380),(#72381,#72382),(#72383,#72384),(#72385,#72386),
(#72387,#72388),(#72389,#72390),(#72391,#72392),(#72393,#72394),(#72395,
#72396),(#72397,#72398),(#72399,#72400),(#72401,#72402),(#72403,#72404),
(#72405,#72406),(#72407,#72408),(#72409,#72410),(#72411,#72412),(#72413,
#72414),(#72415,#72416),(#72417,#72418),(#72419,#72420)),.UNSPECIFIED.,
 .F.,.F.,.F.)
B_SPLINE_SURFACE_WITH_KNOTS((6,1,1,1,1,1,1,1,1,1,1,1,1,1,1,1,1,1,1,1,1,
1,1,1,1,1,1,1,1,1,1,1,1,1,1,1,1,1,1,1,1,1,1,1,1,1,1,1,1,1,1,1,1,1,1,1,1,
1,1,1,1,1,1,1,1,6),(2,2),(-1.,-0.984615384615383,-0.969230769230768,-0.953846153846152,
-0.938461538461537,-0.923076923076922,-0.907692307692306,-0.892307692307691,
-0.876923076923076,-0.86153846153846,-0.846153846153845,-0.83076923076923,
-0.815384615384614,-0.799999999999999,-0.784615384615384,-0.769230769230768,
-0.753846153846153,-0.738461538461538,-0.723076923076922,-0.707692307692307,
-0.692307692307692,-0.676923076923076,-0.661538461538461,-0.646153846153846,
-0.63076923076923,-0.615384615384615,-0.6,-0.584615384615384,-0.569230769230769,
-0.553846153846154,-0.538461538461538,-0.523076923076923,-0.507692307692308,
-0.492307692307692,-0.476923076923077,-0.461538461538462,-0.446153846153846,
-0.430769230769231,-0.415384615384615,-0.4,-0.384615384615385,-0.369230769230769,
-0.353846153846154,-0.338461538461538,-0.323076923076923,-0.307692307692308,
-0.292307692307692,-0.276923076923077,-0.261538461538462,-0.246153846153846,
-0.230769230769231,-0.215384615384615,-0.2,-0.184615384615385,-0.169230769230769,
-0.153846153846154,-0.138461538461538,-0.123076923076923,-0.107692307692308,
-0.0923076923076923,-0.0769230769230769,-0.0615384615384615,-0.0461538461538462,
-0.0307692307692308,-0.0153846153846154,0.),(-1.,1.),.UNSPECIFIED.)
GEOMETRIC_REPRESENTATION_ITEM()
RATIONAL_B_SPLINE_SURFACE(((1.,1.),(1.,1.),(1.,1.),(1.,1.),(1.,1.),(1.,
1.),(1.,1.),(1.,1.),(1.,1.),(1.,1.),(1.,1.),(1.,1.),(1.,1.),(1.,1.),(1.,
1.),(1.,1.),(1.,1.),(1.,1.),(1.,1.),(1.,1.),(1.,1.),(1.,1.),(1.,1.),(1.,
1.),(1.,1.),(1.,1.),(1.,1.),(1.,1.),(1.,1.),(1.,1.),(1.,1.),(1.,1.),(1.,
1.),(1.,1.),(1.,1.),(1.,1.),(1.,1.),(1.,1.),(1.,1.),(1.,1.),(1.,1.),(1.,
1.),(1.,1.),(1.,1.),(1.,1.),(1.,1.),(1.,1.),(1.,1.),(1.,1.),(1.,1.),(1.,
1.),(1.,1.),(1.,1.),(1.,1.),(1.,1.),(1.,1.),(1.,1.),(1.,1.),(1.,1.),(1.,
1.),(1.,1.),(1.,1.),(1.,1.),(1.,1.),(1.,1.),(1.,1.),(1.,1.),(1.,1.),(1.,
1.),(1.,1.)))
REPRESENTATION_ITEM('')
SURFACE()
);
#168=(
BOUNDED_SURFACE()
B_SPLINE_SURFACE(5,1,((#72497,#72498),(#72499,#72500),(#72501,#72502),(#72503,
#72504),(#72505,#72506),(#72507,#72508),(#72509,#72510),(#72511,#72512),
(#72513,#72514),(#72515,#72516),(#72517,#72518),(#72519,#72520),(#72521,
#72522),(#72523,#72524),(#72525,#72526),(#72527,#72528),(#72529,#72530),
(#72531,#72532),(#72533,#72534),(#72535,#72536),(#72537,#72538),(#72539,
#72540),(#72541,#72542),(#72543,#72544),(#72545,#72546),(#72547,#72548),
(#72549,#72550),(#72551,#72552),(#72553,#72554),(#72555,#72556),(#72557,
#72558),(#72559,#72560),(#72561,#72562),(#72563,#72564),(#72565,#72566),
(#72567,#72568),(#72569,#72570),(#72571,#72572),(#72573,#72574),(#72575,
#72576),(#72577,#72578),(#72579,#72580),(#72581,#72582),(#72583,#72584),
(#72585,#72586),(#72587,#72588),(#72589,#72590),(#72591,#72592),(#72593,
#72594),(#72595,#72596),(#72597,#72598),(#72599,#72600),(#72601,#72602),
(#72603,#72604),(#72605,#72606),(#72607,#72608),(#72609,#72610),(#72611,
#72612),(#72613,#72614),(#72615,#72616),(#72617,#72618),(#72619,#72620),
(#72621,#72622),(#72623,#72624),(#72625,#72626),(#72627,#72628),(#72629,
#72630),(#72631,#72632),(#72633,#72634),(#72635,#72636)),.UNSPECIFIED.,
 .F.,.F.,.F.)
B_SPLINE_SURFACE_WITH_KNOTS((6,1,1,1,1,1,1,1,1,1,1,1,1,1,1,1,1,1,1,1,1,
1,1,1,1,1,1,1,1,1,1,1,1,1,1,1,1,1,1,1,1,1,1,1,1,1,1,1,1,1,1,1,1,1,1,1,1,
1,1,1,1,1,1,1,1,6),(2,2),(-1.,-0.984615384615383,-0.969230769230768,-0.953846153846152,
-0.938461538461537,-0.923076923076922,-0.907692307692306,-0.892307692307691,
-0.876923076923076,-0.86153846153846,-0.846153846153845,-0.83076923076923,
-0.815384615384614,-0.799999999999999,-0.784615384615384,-0.769230769230768,
-0.753846153846153,-0.738461538461538,-0.723076923076922,-0.707692307692307,
-0.692307692307692,-0.676923076923076,-0.661538461538461,-0.646153846153846,
-0.63076923076923,-0.615384615384615,-0.6,-0.584615384615384,-0.569230769230769,
-0.553846153846154,-0.538461538461538,-0.523076923076923,-0.507692307692308,
-0.492307692307692,-0.476923076923077,-0.461538461538462,-0.446153846153846,
-0.430769230769231,-0.415384615384615,-0.4,-0.384615384615385,-0.369230769230769,
-0.353846153846154,-0.338461538461538,-0.323076923076923,-0.307692307692308,
-0.292307692307692,-0.276923076923077,-0.261538461538462,-0.246153846153846,
-0.230769230769231,-0.215384615384615,-0.2,-0.184615384615385,-0.169230769230769,
-0.153846153846154,-0.138461538461538,-0.123076923076923,-0.107692307692308,
-0.0923076923076923,-0.0769230769230769,-0.0615384615384615,-0.0461538461538462,
-0.0307692307692308,-0.0153846153846154,0.),(-1.,1.),.UNSPECIFIED.)
GEOMETRIC_REPRESENTATION_ITEM()
RATIONAL_B_SPLINE_SURFACE(((1.,1.),(1.,1.),(1.,1.),(1.,1.),(1.,1.),(1.,
1.),(1.,1.),(1.,1.),(1.,1.),(1.,1.),(1.,1.),(1.,1.),(1.,1.),(1.,1.),(1.,
1.),(1.,1.),(1.,1.),(1.,1.),(1.,1.),(1.,1.),(1.,1.),(1.,1.),(1.,1.),(1.,
1.),(1.,1.),(1.,1.),(1.,1.),(1.,1.),(1.,1.),(1.,1.),(1.,1.),(1.,1.),(1.,
1.),(1.,1.),(1.,1.),(1.,1.),(1.,1.),(1.,1.),(1.,1.),(1.,1.),(1.,1.),(1.,
1.),(1.,1.),(1.,1.),(1.,1.),(1.,1.),(1.,1.),(1.,1.),(1.,1.),(1.,1.),(1.,
1.),(1.,1.),(1.,1.),(1.,1.),(1.,1.),(1.,1.),(1.,1.),(1.,1.),(1.,1.),(1.,
1.),(1.,1.),(1.,1.),(1.,1.),(1.,1.),(1.,1.),(1.,1.),(1.,1.),(1.,1.),(1.,
1.),(1.,1.)))
REPRESENTATION_ITEM('')
SURFACE()
);
#169=(
BOUNDED_SURFACE()
B_SPLINE_SURFACE(5,1,((#72723,#72724),(#72725,#72726),(#72727,#72728),(#72729,
#72730),(#72731,#72732),(#72733,#72734),(#72735,#72736),(#72737,#72738),
(#72739,#72740),(#72741,#72742),(#72743,#72744),(#72745,#72746),(#72747,
#72748),(#72749,#72750),(#72751,#72752),(#72753,#72754),(#72755,#72756),
(#72757,#72758),(#72759,#72760),(#72761,#72762),(#72763,#72764),(#72765,
#72766),(#72767,#72768),(#72769,#72770),(#72771,#72772),(#72773,#72774),
(#72775,#72776),(#72777,#72778),(#72779,#72780),(#72781,#72782),(#72783,
#72784),(#72785,#72786),(#72787,#72788),(#72789,#72790),(#72791,#72792),
(#72793,#72794),(#72795,#72796),(#72797,#72798),(#72799,#72800),(#72801,
#72802),(#72803,#72804),(#72805,#72806),(#72807,#72808),(#72809,#72810),
(#72811,#72812),(#72813,#72814),(#72815,#72816),(#72817,#72818),(#72819,
#72820),(#72821,#72822),(#72823,#72824),(#72825,#72826),(#72827,#72828),
(#72829,#72830),(#72831,#72832),(#72833,#72834),(#72835,#72836),(#72837,
#72838),(#72839,#72840),(#72841,#72842),(#72843,#72844),(#72845,#72846),
(#72847,#72848),(#72849,#72850),(#72851,#72852),(#72853,#72854),(#72855,
#72856),(#72857,#72858),(#72859,#72860),(#72861,#72862)),.UNSPECIFIED.,
 .F.,.F.,.F.)
B_SPLINE_SURFACE_WITH_KNOTS((6,1,1,1,1,1,1,1,1,1,1,1,1,1,1,1,1,1,1,1,1,
1,1,1,1,1,1,1,1,1,1,1,1,1,1,1,1,1,1,1,1,1,1,1,1,1,1,1,1,1,1,1,1,1,1,1,1,
1,1,1,1,1,1,1,1,6),(2,2),(-1.,-0.984615384615383,-0.969230769230768,-0.953846153846152,
-0.938461538461537,-0.923076923076922,-0.907692307692306,-0.892307692307691,
-0.876923076923076,-0.86153846153846,-0.846153846153845,-0.83076923076923,
-0.815384615384614,-0.799999999999999,-0.784615384615384,-0.769230769230768,
-0.753846153846153,-0.738461538461538,-0.723076923076922,-0.707692307692307,
-0.692307692307692,-0.676923076923076,-0.661538461538461,-0.646153846153846,
-0.63076923076923,-0.615384615384615,-0.6,-0.584615384615384,-0.569230769230769,
-0.553846153846154,-0.538461538461538,-0.523076923076923,-0.507692307692308,
-0.492307692307692,-0.476923076923077,-0.461538461538462,-0.446153846153846,
-0.430769230769231,-0.415384615384615,-0.4,-0.384615384615385,-0.369230769230769,
-0.353846153846154,-0.338461538461538,-0.323076923076923,-0.307692307692308,
-0.292307692307692,-0.276923076923077,-0.261538461538462,-0.246153846153846,
-0.230769230769231,-0.215384615384615,-0.2,-0.184615384615385,-0.169230769230769,
-0.153846153846154,-0.138461538461538,-0.123076923076923,-0.107692307692308,
-0.0923076923076923,-0.0769230769230769,-0.0615384615384615,-0.0461538461538462,
-0.0307692307692308,-0.0153846153846154,0.),(-1.,1.),.UNSPECIFIED.)
GEOMETRIC_REPRESENTATION_ITEM()
RATIONAL_B_SPLINE_SURFACE(((1.,1.),(1.,1.),(1.,1.),(1.,1.),(1.,1.),(1.,
1.),(1.,1.),(1.,1.),(1.,1.),(1.,1.),(1.,1.),(1.,1.),(1.,1.),(1.,1.),(1.,
1.),(1.,1.),(1.,1.),(1.,1.),(1.,1.),(1.,1.),(1.,1.),(1.,1.),(1.,1.),(1.,
1.),(1.,1.),(1.,1.),(1.,1.),(1.,1.),(1.,1.),(1.,1.),(1.,1.),(1.,1.),(1.,
1.),(1.,1.),(1.,1.),(1.,1.),(1.,1.),(1.,1.),(1.,1.),(1.,1.),(1.,1.),(1.,
1.),(1.,1.),(1.,1.),(1.,1.),(1.,1.),(1.,1.),(1.,1.),(1.,1.),(1.,1.),(1.,
1.),(1.,1.),(1.,1.),(1.,1.),(1.,1.),(1.,1.),(1.,1.),(1.,1.),(1.,1.),(1.,
1.),(1.,1.),(1.,1.),(1.,1.),(1.,1.),(1.,1.),(1.,1.),(1.,1.),(1.,1.),(1.,
1.),(1.,1.)))
REPRESENTATION_ITEM('')
SURFACE()
);
#170=(
BOUNDED_SURFACE()
B_SPLINE_SURFACE(5,1,((#72942,#72943),(#72944,#72945),(#72946,#72947),(#72948,
#72949),(#72950,#72951),(#72952,#72953),(#72954,#72955),(#72956,#72957),
(#72958,#72959),(#72960,#72961),(#72962,#72963),(#72964,#72965),(#72966,
#72967),(#72968,#72969),(#72970,#72971),(#72972,#72973),(#72974,#72975),
(#72976,#72977),(#72978,#72979),(#72980,#72981),(#72982,#72983),(#72984,
#72985),(#72986,#72987),(#72988,#72989),(#72990,#72991),(#72992,#72993),
(#72994,#72995),(#72996,#72997),(#72998,#72999),(#73000,#73001),(#73002,
#73003),(#73004,#73005),(#73006,#73007),(#73008,#73009),(#73010,#73011),
(#73012,#73013),(#73014,#73015),(#73016,#73017),(#73018,#73019),(#73020,
#73021),(#73022,#73023),(#73024,#73025),(#73026,#73027),(#73028,#73029),
(#73030,#73031),(#73032,#73033),(#73034,#73035),(#73036,#73037),(#73038,
#73039),(#73040,#73041),(#73042,#73043),(#73044,#73045),(#73046,#73047),
(#73048,#73049),(#73050,#73051),(#73052,#73053),(#73054,#73055),(#73056,
#73057),(#73058,#73059),(#73060,#73061),(#73062,#73063),(#73064,#73065),
(#73066,#73067),(#73068,#73069),(#73070,#73071),(#73072,#73073),(#73074,
#73075),(#73076,#73077),(#73078,#73079),(#73080,#73081)),.UNSPECIFIED.,
 .F.,.F.,.F.)
B_SPLINE_SURFACE_WITH_KNOTS((6,1,1,1,1,1,1,1,1,1,1,1,1,1,1,1,1,1,1,1,1,
1,1,1,1,1,1,1,1,1,1,1,1,1,1,1,1,1,1,1,1,1,1,1,1,1,1,1,1,1,1,1,1,1,1,1,1,
1,1,1,1,1,1,1,1,6),(2,2),(-1.,-0.984615384615383,-0.969230769230768,-0.953846153846152,
-0.938461538461537,-0.923076923076922,-0.907692307692306,-0.892307692307691,
-0.876923076923076,-0.86153846153846,-0.846153846153845,-0.83076923076923,
-0.815384615384614,-0.799999999999999,-0.784615384615384,-0.769230769230768,
-0.753846153846153,-0.738461538461538,-0.723076923076922,-0.707692307692307,
-0.692307692307692,-0.676923076923076,-0.661538461538461,-0.646153846153846,
-0.63076923076923,-0.615384615384615,-0.6,-0.584615384615384,-0.569230769230769,
-0.553846153846154,-0.538461538461538,-0.523076923076923,-0.507692307692308,
-0.492307692307692,-0.476923076923077,-0.461538461538462,-0.446153846153846,
-0.430769230769231,-0.415384615384615,-0.4,-0.384615384615385,-0.369230769230769,
-0.353846153846154,-0.338461538461538,-0.323076923076923,-0.307692307692308,
-0.292307692307692,-0.276923076923077,-0.261538461538462,-0.246153846153846,
-0.230769230769231,-0.215384615384615,-0.2,-0.184615384615385,-0.169230769230769,
-0.153846153846154,-0.138461538461538,-0.123076923076923,-0.107692307692308,
-0.0923076923076923,-0.0769230769230769,-0.0615384615384615,-0.0461538461538462,
-0.0307692307692308,-0.0153846153846154,0.),(-1.,1.),.UNSPECIFIED.)
GEOMETRIC_REPRESENTATION_ITEM()
RATIONAL_B_SPLINE_SURFACE(((1.,1.),(1.,1.),(1.,1.),(1.,1.),(1.,1.),(1.,
1.),(1.,1.),(1.,1.),(1.,1.),(1.,1.),(1.,1.),(1.,1.),(1.,1.),(1.,1.),(1.,
1.),(1.,1.),(1.,1.),(1.,1.),(1.,1.),(1.,1.),(1.,1.),(1.,1.),(1.,1.),(1.,
1.),(1.,1.),(1.,1.),(1.,1.),(1.,1.),(1.,1.),(1.,1.),(1.,1.),(1.,1.),(1.,
1.),(1.,1.),(1.,1.),(1.,1.),(1.,1.),(1.,1.),(1.,1.),(1.,1.),(1.,1.),(1.,
1.),(1.,1.),(1.,1.),(1.,1.),(1.,1.),(1.,1.),(1.,1.),(1.,1.),(1.,1.),(1.,
1.),(1.,1.),(1.,1.),(1.,1.),(1.,1.),(1.,1.),(1.,1.),(1.,1.),(1.,1.),(1.,
1.),(1.,1.),(1.,1.),(1.,1.),(1.,1.),(1.,1.),(1.,1.),(1.,1.),(1.,1.),(1.,
1.),(1.,1.)))
REPRESENTATION_ITEM('')
SURFACE()
);
#331=(
BOUNDED_CURVE()
B_SPLINE_CURVE(5,(#49632,#49633,#49634,#49635,#49636,#49637,#49638,#49639,
#49640,#49641,#49642,#49643,#49644,#49645,#49646,#49647,#49648,#49649,#49650,
#49651,#49652,#49653,#49654,#49655,#49656,#49657,#49658,#49659,#49660,#49661,
#49662,#49663,#49664,#49665,#49666,#49667,#49668,#49669,#49670,#49671,#49672,
#49673,#49674,#49675,#49676,#49677,#49678,#49679,#49680,#49681,#49682,#49683,
#49684,#49685,#49686,#49687,#49688,#49689,#49690,#49691,#49692,#49693,#49694,
#49695,#49696,#49697,#49698,#49699,#49700,#49701),.UNSPECIFIED.,.F.,.F.)
B_SPLINE_CURVE_WITH_KNOTS((6,1,1,1,1,1,1,1,1,1,1,1,1,1,1,1,1,1,1,1,1,1,
1,1,1,1,1,1,1,1,1,1,1,1,1,1,1,1,1,1,1,1,1,1,1,1,1,1,1,1,1,1,1,1,1,1,1,1,
1,1,1,1,1,1,1,6),(0.00577184337450058,0.0153846153846154,0.0307692307692308,
0.0461538461538462,0.0615384615384615,0.0769230769230769,0.0923076923076923,
0.107692307692308,0.123076923076923,0.138461538461538,0.153846153846154,
0.169230769230769,0.184615384615385,0.2,0.215384615384615,0.230769230769231,
0.246153846153846,0.261538461538462,0.276923076923077,0.292307692307692,
0.307692307692308,0.323076923076923,0.338461538461538,0.353846153846154,
0.369230769230769,0.384615384615385,0.4,0.415384615384615,0.430769230769231,
0.446153846153846,0.461538461538462,0.476923076923077,0.492307692307692,
0.507692307692308,0.523076923076923,0.538461538461538,0.553846153846154,
0.569230769230769,0.584615384615384,0.6,0.615384615384615,0.63076923076923,
0.646153846153846,0.661538461538461,0.676923076923076,0.692307692307692,
0.707692307692307,0.723076923076922,0.738461538461538,0.753846153846153,
0.769230769230768,0.784615384615384,0.799999999999999,0.815384615384614,
0.83076923076923,0.846153846153845,0.86153846153846,0.876923076923076,0.892307692307691,
0.907692307692306,0.923076923076922,0.938461538461537,0.953846153846152,
0.969230769230768,0.984615384615383,1.),.UNSPECIFIED.)
CURVE()
GEOMETRIC_REPRESENTATION_ITEM()
RATIONAL_B_SPLINE_CURVE((1.,1.,1.,1.,1.,1.,1.,1.,1.,1.,1.,1.,1.,1.,1.,1.,
1.,1.,1.,1.,1.,1.,1.,1.,1.,1.,1.,1.,1.,1.,1.,1.,1.,1.,1.,1.,1.,1.,1.,1.,
1.,1.,1.,1.,1.,1.,1.,1.,1.,1.,1.,1.,1.,1.,1.,1.,1.,1.,1.,1.,1.,1.,1.,1.,
1.,1.,1.,1.,1.,1.))
REPRESENTATION_ITEM('')
);
#332=(
BOUNDED_CURVE()
B_SPLINE_CURVE(5,(#49705,#49706,#49707,#49708,#49709,#49710,#49711,#49712,
#49713,#49714,#49715,#49716,#49717,#49718,#49719,#49720,#49721,#49722,#49723,
#49724,#49725,#49726,#49727,#49728,#49729,#49730,#49731,#49732,#49733,#49734,
#49735,#49736,#49737,#49738,#49739,#49740,#49741,#49742,#49743,#49744,#49745,
#49746,#49747,#49748,#49749,#49750,#49751,#49752,#49753,#49754,#49755,#49756,
#49757,#49758,#49759,#49760,#49761,#49762,#49763,#49764,#49765,#49766,#49767,
#49768,#49769,#49770,#49771,#49772,#49773,#49774),.UNSPECIFIED.,.F.,.F.)
B_SPLINE_CURVE_WITH_KNOTS((6,1,1,1,1,1,1,1,1,1,1,1,1,1,1,1,1,1,1,1,1,1,
1,1,1,1,1,1,1,1,1,1,1,1,1,1,1,1,1,1,1,1,1,1,1,1,1,1,1,1,1,1,1,1,1,1,1,1,
1,1,1,1,1,1,1,6),(0.,0.0153846153846154,0.0307692307692308,0.0461538461538462,
0.0615384615384615,0.0769230769230769,0.0923076923076923,0.107692307692308,
0.123076923076923,0.138461538461538,0.153846153846154,0.169230769230769,
0.184615384615385,0.2,0.215384615384615,0.230769230769231,0.246153846153846,
0.261538461538462,0.276923076923077,0.292307692307692,0.307692307692308,
0.323076923076923,0.338461538461538,0.353846153846154,0.369230769230769,
0.384615384615385,0.4,0.415384615384615,0.430769230769231,0.446153846153846,
0.461538461538462,0.476923076923077,0.492307692307692,0.507692307692308,
0.523076923076923,0.538461538461538,0.553846153846154,0.569230769230769,
0.584615384615384,0.6,0.615384615384615,0.63076923076923,0.646153846153846,
0.661538461538461,0.676923076923076,0.692307692307692,0.707692307692307,
0.723076923076922,0.738461538461538,0.753846153846153,0.769230769230768,
0.784615384615384,0.799999999999999,0.815384615384614,0.83076923076923,
0.846153846153845,0.86153846153846,0.876923076923076,0.892307692307691,
0.907692307692306,0.923076923076922,0.938461538461537,0.953846153846152,
0.969230769230768,0.984615384615383,0.994228156739708),.UNSPECIFIED.)
CURVE()
GEOMETRIC_REPRESENTATION_ITEM()
RATIONAL_B_SPLINE_CURVE((1.,1.,1.,1.,1.,1.,1.,1.,1.,1.,1.,1.,1.,1.,1.,1.,
1.,1.,1.,1.,1.,1.,1.,1.,1.,1.,1.,1.,1.,1.,1.,1.,1.,1.,1.,1.,1.,1.,1.,1.,
1.,1.,1.,1.,1.,1.,1.,1.,1.,1.,1.,1.,1.,1.,1.,1.,1.,1.,1.,1.,1.,1.,1.,1.,
1.,1.,1.,1.,1.,1.))
REPRESENTATION_ITEM('')
);
#333=(
BOUNDED_CURVE()
B_SPLINE_CURVE(5,(#49778,#49779,#49780,#49781,#49782,#49783,#49784,#49785,
#49786,#49787,#49788,#49789,#49790,#49791,#49792,#49793,#49794,#49795,#49796,
#49797,#49798,#49799,#49800,#49801,#49802,#49803,#49804,#49805,#49806,#49807,
#49808,#49809,#49810,#49811,#49812,#49813,#49814,#49815,#49816,#49817,#49818,
#49819,#49820,#49821,#49822,#49823,#49824,#49825,#49826,#49827,#49828,#49829,
#49830,#49831,#49832,#49833,#49834,#49835,#49836,#49837,#49838,#49839,#49840,
#49841,#49842,#49843,#49844,#49845,#49846,#49847),.UNSPECIFIED.,.F.,.F.)
B_SPLINE_CURVE_WITH_KNOTS((6,1,1,1,1,1,1,1,1,1,1,1,1,1,1,1,1,1,1,1,1,1,
1,1,1,1,1,1,1,1,1,1,1,1,1,1,1,1,1,1,1,1,1,1,1,1,1,1,1,1,1,1,1,1,1,1,1,1,
1,1,1,1,1,1,1,6),(0.0057718433745091,0.0153846153846154,0.0307692307692308,
0.0461538461538462,0.0615384615384615,0.0769230769230769,0.0923076923076923,
0.107692307692308,0.123076923076923,0.138461538461538,0.153846153846154,
0.169230769230769,0.184615384615385,0.2,0.215384615384615,0.230769230769231,
0.246153846153846,0.261538461538462,0.276923076923077,0.292307692307692,
0.307692307692308,0.323076923076923,0.338461538461538,0.353846153846154,
0.369230769230769,0.384615384615385,0.4,0.415384615384615,0.430769230769231,
0.446153846153846,0.461538461538462,0.476923076923077,0.492307692307692,
0.507692307692308,0.523076923076923,0.538461538461538,0.553846153846154,
0.569230769230769,0.584615384615384,0.6,0.615384615384615,0.63076923076923,
0.646153846153846,0.661538461538461,0.676923076923076,0.692307692307692,
0.707692307692307,0.723076923076922,0.738461538461538,0.753846153846153,
0.769230769230768,0.784615384615384,0.799999999999999,0.815384615384614,
0.83076923076923,0.846153846153845,0.86153846153846,0.876923076923076,0.892307692307691,
0.907692307692306,0.923076923076922,0.938461538461537,0.953846153846152,
0.969230769230768,0.984615384615383,1.),.UNSPECIFIED.)
CURVE()
GEOMETRIC_REPRESENTATION_ITEM()
RATIONAL_B_SPLINE_CURVE((1.,1.,1.,1.,1.,1.,1.,1.,1.,1.,1.,1.,1.,1.,1.,1.,
1.,1.,1.,1.,1.,1.,1.,1.,1.,1.,1.,1.,1.,1.,1.,1.,1.,1.,1.,1.,1.,1.,1.,1.,
1.,1.,1.,1.,1.,1.,1.,1.,1.,1.,1.,1.,1.,1.,1.,1.,1.,1.,1.,1.,1.,1.,1.,1.,
1.,1.,1.,1.,1.,1.))
REPRESENTATION_ITEM('')
);
#334=(
BOUNDED_CURVE()
B_SPLINE_CURVE(5,(#49851,#49852,#49853,#49854,#49855,#49856,#49857,#49858,
#49859,#49860,#49861,#49862,#49863,#49864,#49865,#49866,#49867,#49868,#49869,
#49870,#49871,#49872,#49873,#49874,#49875,#49876,#49877,#49878,#49879,#49880,
#49881,#49882,#49883,#49884,#49885,#49886,#49887,#49888,#49889,#49890,#49891,
#49892,#49893,#49894,#49895,#49896,#49897,#49898,#49899,#49900,#49901,#49902,
#49903,#49904,#49905,#49906,#49907,#49908,#49909,#49910,#49911,#49912,#49913,
#49914,#49915,#49916,#49917,#49918,#49919,#49920),.UNSPECIFIED.,.F.,.F.)
B_SPLINE_CURVE_WITH_KNOTS((6,1,1,1,1,1,1,1,1,1,1,1,1,1,1,1,1,1,1,1,1,1,
1,1,1,1,1,1,1,1,1,1,1,1,1,1,1,1,1,1,1,1,1,1,1,1,1,1,1,1,1,1,1,1,1,1,1,1,
1,1,1,1,1,1,1,6),(0.,0.0153846153846154,0.0307692307692308,0.0461538461538462,
0.0615384615384615,0.0769230769230769,0.0923076923076923,0.107692307692308,
0.123076923076923,0.138461538461538,0.153846153846154,0.169230769230769,
0.184615384615385,0.2,0.215384615384615,0.230769230769231,0.246153846153846,
0.261538461538462,0.276923076923077,0.292307692307692,0.307692307692308,
0.323076923076923,0.338461538461538,0.353846153846154,0.369230769230769,
0.384615384615385,0.4,0.415384615384615,0.430769230769231,0.446153846153846,
0.461538461538462,0.476923076923077,0.492307692307692,0.507692307692308,
0.523076923076923,0.538461538461538,0.553846153846154,0.569230769230769,
0.584615384615384,0.6,0.615384615384615,0.63076923076923,0.646153846153846,
0.661538461538461,0.676923076923076,0.692307692307692,0.707692307692307,
0.723076923076922,0.738461538461538,0.753846153846153,0.769230769230768,
0.784615384615384,0.799999999999999,0.815384615384614,0.83076923076923,
0.846153846153845,0.86153846153846,0.876923076923076,0.892307692307691,
0.907692307692306,0.923076923076922,0.938461538461537,0.953846153846152,
0.969230769230768,0.984615384615383,0.994228156739689),.UNSPECIFIED.)
CURVE()
GEOMETRIC_REPRESENTATION_ITEM()
RATIONAL_B_SPLINE_CURVE((1.,1.,1.,1.,1.,1.,1.,1.,1.,1.,1.,1.,1.,1.,1.,1.,
1.,1.,1.,1.,1.,1.,1.,1.,1.,1.,1.,1.,1.,1.,1.,1.,1.,1.,1.,1.,1.,1.,1.,1.,
1.,1.,1.,1.,1.,1.,1.,1.,1.,1.,1.,1.,1.,1.,1.,1.,1.,1.,1.,1.,1.,1.,1.,1.,
1.,1.,1.,1.,1.,1.))
REPRESENTATION_ITEM('')
);
#335=(
BOUNDED_CURVE()
B_SPLINE_CURVE(5,(#49924,#49925,#49926,#49927,#49928,#49929,#49930,#49931,
#49932,#49933,#49934,#49935,#49936,#49937,#49938,#49939,#49940,#49941,#49942,
#49943,#49944,#49945,#49946,#49947,#49948,#49949,#49950,#49951,#49952,#49953,
#49954,#49955,#49956,#49957,#49958,#49959,#49960,#49961,#49962,#49963,#49964,
#49965,#49966,#49967,#49968,#49969,#49970,#49971,#49972,#49973,#49974,#49975,
#49976,#49977,#49978,#49979,#49980,#49981,#49982,#49983,#49984,#49985,#49986,
#49987,#49988,#49989,#49990,#49991,#49992,#49993),.UNSPECIFIED.,.F.,.F.)
B_SPLINE_CURVE_WITH_KNOTS((6,1,1,1,1,1,1,1,1,1,1,1,1,1,1,1,1,1,1,1,1,1,
1,1,1,1,1,1,1,1,1,1,1,1,1,1,1,1,1,1,1,1,1,1,1,1,1,1,1,1,1,1,1,1,1,1,1,1,
1,1,1,1,1,1,1,6),(0.00577184337448946,0.0153846153846154,0.0307692307692308,
0.0461538461538462,0.0615384615384615,0.0769230769230769,0.0923076923076923,
0.107692307692308,0.123076923076923,0.138461538461538,0.153846153846154,
0.169230769230769,0.184615384615385,0.2,0.215384615384615,0.230769230769231,
0.246153846153846,0.261538461538462,0.276923076923077,0.292307692307692,
0.307692307692308,0.323076923076923,0.338461538461538,0.353846153846154,
0.369230769230769,0.384615384615385,0.4,0.415384615384615,0.430769230769231,
0.446153846153846,0.461538461538462,0.476923076923077,0.492307692307692,
0.507692307692308,0.523076923076923,0.538461538461538,0.553846153846154,
0.569230769230769,0.584615384615384,0.6,0.615384615384615,0.63076923076923,
0.646153846153846,0.661538461538461,0.676923076923076,0.692307692307692,
0.707692307692307,0.723076923076922,0.738461538461538,0.753846153846153,
0.769230769230768,0.784615384615384,0.799999999999999,0.815384615384614,
0.83076923076923,0.846153846153845,0.86153846153846,0.876923076923076,0.892307692307691,
0.907692307692306,0.923076923076922,0.938461538461537,0.953846153846152,
0.969230769230768,0.984615384615383,1.),.UNSPECIFIED.)
CURVE()
GEOMETRIC_REPRESENTATION_ITEM()
RATIONAL_B_SPLINE_CURVE((1.,1.,1.,1.,1.,1.,1.,1.,1.,1.,1.,1.,1.,1.,1.,1.,
1.,1.,1.,1.,1.,1.,1.,1.,1.,1.,1.,1.,1.,1.,1.,1.,1.,1.,1.,1.,1.,1.,1.,1.,
1.,1.,1.,1.,1.,1.,1.,1.,1.,1.,1.,1.,1.,1.,1.,1.,1.,1.,1.,1.,1.,1.,1.,1.,
1.,1.,1.,1.,1.,1.))
REPRESENTATION_ITEM('')
);
#336=(
BOUNDED_CURVE()
B_SPLINE_CURVE(5,(#49997,#49998,#49999,#50000,#50001,#50002,#50003,#50004,
#50005,#50006,#50007,#50008,#50009,#50010,#50011,#50012,#50013,#50014,#50015,
#50016,#50017,#50018,#50019,#50020,#50021,#50022,#50023,#50024,#50025,#50026,
#50027,#50028,#50029,#50030,#50031,#50032,#50033,#50034,#50035,#50036,#50037,
#50038,#50039,#50040,#50041,#50042,#50043,#50044,#50045,#50046,#50047,#50048,
#50049,#50050,#50051,#50052,#50053,#50054,#50055,#50056,#50057,#50058,#50059,
#50060,#50061,#50062,#50063,#50064,#50065,#50066),.UNSPECIFIED.,.F.,.F.)
B_SPLINE_CURVE_WITH_KNOTS((6,1,1,1,1,1,1,1,1,1,1,1,1,1,1,1,1,1,1,1,1,1,
1,1,1,1,1,1,1,1,1,1,1,1,1,1,1,1,1,1,1,1,1,1,1,1,1,1,1,1,1,1,1,1,1,1,1,1,
1,1,1,1,1,1,1,6),(0.,0.0153846153846154,0.0307692307692308,0.0461538461538462,
0.0615384615384615,0.0769230769230769,0.0923076923076923,0.107692307692308,
0.123076923076923,0.138461538461538,0.153846153846154,0.169230769230769,
0.184615384615385,0.2,0.215384615384615,0.230769230769231,0.246153846153846,
0.261538461538462,0.276923076923077,0.292307692307692,0.307692307692308,
0.323076923076923,0.338461538461538,0.353846153846154,0.369230769230769,
0.384615384615385,0.4,0.415384615384615,0.430769230769231,0.446153846153846,
0.461538461538462,0.476923076923077,0.492307692307692,0.507692307692308,
0.523076923076923,0.538461538461538,0.553846153846154,0.569230769230769,
0.584615384615384,0.6,0.615384615384615,0.63076923076923,0.646153846153846,
0.661538461538461,0.676923076923076,0.692307692307692,0.707692307692307,
0.723076923076922,0.738461538461538,0.753846153846153,0.769230769230768,
0.784615384615384,0.799999999999999,0.815384615384614,0.83076923076923,
0.846153846153845,0.86153846153846,0.876923076923076,0.892307692307691,
0.907692307692306,0.923076923076922,0.938461538461537,0.953846153846152,
0.969230769230768,0.984615384615383,0.994228156739718),.UNSPECIFIED.)
CURVE()
GEOMETRIC_REPRESENTATION_ITEM()
RATIONAL_B_SPLINE_CURVE((1.,1.,1.,1.,1.,1.,1.,1.,1.,1.,1.,1.,1.,1.,1.,1.,
1.,1.,1.,1.,1.,1.,1.,1.,1.,1.,1.,1.,1.,1.,1.,1.,1.,1.,1.,1.,1.,1.,1.,1.,
1.,1.,1.,1.,1.,1.,1.,1.,1.,1.,1.,1.,1.,1.,1.,1.,1.,1.,1.,1.,1.,1.,1.,1.,
1.,1.,1.,1.,1.,1.))
REPRESENTATION_ITEM('')
);
#337=(
BOUNDED_CURVE()
B_SPLINE_CURVE(5,(#50070,#50071,#50072,#50073,#50074,#50075,#50076,#50077,
#50078,#50079,#50080,#50081,#50082,#50083,#50084,#50085,#50086,#50087,#50088,
#50089,#50090,#50091,#50092,#50093,#50094,#50095,#50096,#50097,#50098,#50099,
#50100,#50101,#50102,#50103,#50104,#50105,#50106,#50107,#50108,#50109,#50110,
#50111,#50112,#50113,#50114,#50115,#50116,#50117,#50118,#50119,#50120,#50121,
#50122,#50123,#50124,#50125,#50126,#50127,#50128,#50129,#50130,#50131,#50132,
#50133,#50134,#50135,#50136,#50137,#50138,#50139),.UNSPECIFIED.,.F.,.F.)
B_SPLINE_CURVE_WITH_KNOTS((6,1,1,1,1,1,1,1,1,1,1,1,1,1,1,1,1,1,1,1,1,1,
1,1,1,1,1,1,1,1,1,1,1,1,1,1,1,1,1,1,1,1,1,1,1,1,1,1,1,1,1,1,1,1,1,1,1,1,
1,1,1,1,1,1,1,6),(0.00577184337450897,0.0153846153846154,0.0307692307692308,
0.0461538461538462,0.0615384615384615,0.0769230769230769,0.0923076923076923,
0.107692307692308,0.123076923076923,0.138461538461538,0.153846153846154,
0.169230769230769,0.184615384615385,0.2,0.215384615384615,0.230769230769231,
0.246153846153846,0.261538461538462,0.276923076923077,0.292307692307692,
0.307692307692308,0.323076923076923,0.338461538461538,0.353846153846154,
0.369230769230769,0.384615384615385,0.4,0.415384615384615,0.430769230769231,
0.446153846153846,0.461538461538462,0.476923076923077,0.492307692307692,
0.507692307692308,0.523076923076923,0.538461538461538,0.553846153846154,
0.569230769230769,0.584615384615384,0.6,0.615384615384615,0.63076923076923,
0.646153846153846,0.661538461538461,0.676923076923076,0.692307692307692,
0.707692307692307,0.723076923076922,0.738461538461538,0.753846153846153,
0.769230769230768,0.784615384615384,0.799999999999999,0.815384615384614,
0.83076923076923,0.846153846153845,0.86153846153846,0.876923076923076,0.892307692307691,
0.907692307692306,0.923076923076922,0.938461538461537,0.953846153846152,
0.969230769230768,0.984615384615383,1.),.UNSPECIFIED.)
CURVE()
GEOMETRIC_REPRESENTATION_ITEM()
RATIONAL_B_SPLINE_CURVE((1.,1.,1.,1.,1.,1.,1.,1.,1.,1.,1.,1.,1.,1.,1.,1.,
1.,1.,1.,1.,1.,1.,1.,1.,1.,1.,1.,1.,1.,1.,1.,1.,1.,1.,1.,1.,1.,1.,1.,1.,
1.,1.,1.,1.,1.,1.,1.,1.,1.,1.,1.,1.,1.,1.,1.,1.,1.,1.,1.,1.,1.,1.,1.,1.,
1.,1.,1.,1.,1.,1.))
REPRESENTATION_ITEM('')
);
#338=(
BOUNDED_CURVE()
B_SPLINE_CURVE(5,(#50143,#50144,#50145,#50146,#50147,#50148,#50149,#50150,
#50151,#50152,#50153,#50154,#50155,#50156,#50157,#50158,#50159,#50160,#50161,
#50162,#50163,#50164,#50165,#50166,#50167,#50168,#50169,#50170,#50171,#50172,
#50173,#50174,#50175,#50176,#50177,#50178,#50179,#50180,#50181,#50182,#50183,
#50184,#50185,#50186,#50187,#50188,#50189,#50190,#50191,#50192,#50193,#50194,
#50195,#50196,#50197,#50198,#50199,#50200,#50201,#50202,#50203,#50204,#50205,
#50206,#50207,#50208,#50209,#50210,#50211,#50212),.UNSPECIFIED.,.F.,.F.)
B_SPLINE_CURVE_WITH_KNOTS((6,1,1,1,1,1,1,1,1,1,1,1,1,1,1,1,1,1,1,1,1,1,
1,1,1,1,1,1,1,1,1,1,1,1,1,1,1,1,1,1,1,1,1,1,1,1,1,1,1,1,1,1,1,1,1,1,1,1,
1,1,1,1,1,1,1,6),(0.,0.0153846153846154,0.0307692307692308,0.0461538461538462,
0.0615384615384615,0.0769230769230769,0.0923076923076923,0.107692307692308,
0.123076923076923,0.138461538461538,0.153846153846154,0.169230769230769,
0.184615384615385,0.2,0.215384615384615,0.230769230769231,0.246153846153846,
0.261538461538462,0.276923076923077,0.292307692307692,0.307692307692308,
0.323076923076923,0.338461538461538,0.353846153846154,0.369230769230769,
0.384615384615385,0.4,0.415384615384615,0.430769230769231,0.446153846153846,
0.461538461538462,0.476923076923077,0.492307692307692,0.507692307692308,
0.523076923076923,0.538461538461538,0.553846153846154,0.569230769230769,
0.584615384615384,0.6,0.615384615384615,0.63076923076923,0.646153846153846,
0.661538461538461,0.676923076923076,0.692307692307692,0.707692307692307,
0.723076923076922,0.738461538461538,0.753846153846153,0.769230769230768,
0.784615384615384,0.799999999999999,0.815384615384614,0.83076923076923,
0.846153846153845,0.86153846153846,0.876923076923076,0.892307692307691,
0.907692307692306,0.923076923076922,0.938461538461537,0.953846153846152,
0.969230769230768,0.984615384615383,0.994228156739701),.UNSPECIFIED.)
CURVE()
GEOMETRIC_REPRESENTATION_ITEM()
RATIONAL_B_SPLINE_CURVE((1.,1.,1.,1.,1.,1.,1.,1.,1.,1.,1.,1.,1.,1.,1.,1.,
1.,1.,1.,1.,1.,1.,1.,1.,1.,1.,1.,1.,1.,1.,1.,1.,1.,1.,1.,1.,1.,1.,1.,1.,
1.,1.,1.,1.,1.,1.,1.,1.,1.,1.,1.,1.,1.,1.,1.,1.,1.,1.,1.,1.,1.,1.,1.,1.,
1.,1.,1.,1.,1.,1.))
REPRESENTATION_ITEM('')
);
#339=(
BOUNDED_CURVE()
B_SPLINE_CURVE(5,(#50216,#50217,#50218,#50219,#50220,#50221,#50222,#50223,
#50224,#50225,#50226,#50227,#50228,#50229,#50230,#50231,#50232,#50233,#50234,
#50235,#50236,#50237,#50238,#50239,#50240,#50241,#50242,#50243,#50244,#50245,
#50246,#50247,#50248,#50249,#50250,#50251,#50252,#50253,#50254,#50255,#50256,
#50257,#50258,#50259,#50260,#50261,#50262,#50263,#50264,#50265,#50266,#50267,
#50268,#50269,#50270,#50271,#50272,#50273,#50274,#50275,#50276,#50277,#50278,
#50279,#50280,#50281,#50282,#50283,#50284,#50285),.UNSPECIFIED.,.F.,.F.)
B_SPLINE_CURVE_WITH_KNOTS((6,1,1,1,1,1,1,1,1,1,1,1,1,1,1,1,1,1,1,1,1,1,
1,1,1,1,1,1,1,1,1,1,1,1,1,1,1,1,1,1,1,1,1,1,1,1,1,1,1,1,1,1,1,1,1,1,1,1,
1,1,1,1,1,1,1,6),(0.00577184337451001,0.0153846153846154,0.0307692307692308,
0.0461538461538462,0.0615384615384615,0.0769230769230769,0.0923076923076923,
0.107692307692308,0.123076923076923,0.138461538461538,0.153846153846154,
0.169230769230769,0.184615384615385,0.2,0.215384615384615,0.230769230769231,
0.246153846153846,0.261538461538462,0.276923076923077,0.292307692307692,
0.307692307692308,0.323076923076923,0.338461538461538,0.353846153846154,
0.369230769230769,0.384615384615385,0.4,0.415384615384615,0.430769230769231,
0.446153846153846,0.461538461538462,0.476923076923077,0.492307692307692,
0.507692307692308,0.523076923076923,0.538461538461538,0.553846153846154,
0.569230769230769,0.584615384615384,0.6,0.615384615384615,0.63076923076923,
0.646153846153846,0.661538461538461,0.676923076923076,0.692307692307692,
0.707692307692307,0.723076923076922,0.738461538461538,0.753846153846153,
0.769230769230768,0.784615384615384,0.799999999999999,0.815384615384614,
0.83076923076923,0.846153846153845,0.86153846153846,0.876923076923076,0.892307692307691,
0.907692307692306,0.923076923076922,0.938461538461537,0.953846153846152,
0.969230769230768,0.984615384615383,1.),.UNSPECIFIED.)
CURVE()
GEOMETRIC_REPRESENTATION_ITEM()
RATIONAL_B_SPLINE_CURVE((1.,1.,1.,1.,1.,1.,1.,1.,1.,1.,1.,1.,1.,1.,1.,1.,
1.,1.,1.,1.,1.,1.,1.,1.,1.,1.,1.,1.,1.,1.,1.,1.,1.,1.,1.,1.,1.,1.,1.,1.,
1.,1.,1.,1.,1.,1.,1.,1.,1.,1.,1.,1.,1.,1.,1.,1.,1.,1.,1.,1.,1.,1.,1.,1.,
1.,1.,1.,1.,1.,1.))
REPRESENTATION_ITEM('')
);
#340=(
BOUNDED_CURVE()
B_SPLINE_CURVE(5,(#50289,#50290,#50291,#50292,#50293,#50294,#50295,#50296,
#50297,#50298,#50299,#50300,#50301,#50302,#50303,#50304,#50305,#50306,#50307,
#50308,#50309,#50310,#50311,#50312,#50313,#50314,#50315,#50316,#50317,#50318,
#50319,#50320,#50321,#50322,#50323,#50324,#50325,#50326,#50327,#50328,#50329,
#50330,#50331,#50332,#50333,#50334,#50335,#50336,#50337,#50338,#50339,#50340,
#50341,#50342,#50343,#50344,#50345,#50346,#50347,#50348,#50349,#50350,#50351,
#50352,#50353,#50354,#50355,#50356,#50357,#50358),.UNSPECIFIED.,.F.,.F.)
B_SPLINE_CURVE_WITH_KNOTS((6,1,1,1,1,1,1,1,1,1,1,1,1,1,1,1,1,1,1,1,1,1,
1,1,1,1,1,1,1,1,1,1,1,1,1,1,1,1,1,1,1,1,1,1,1,1,1,1,1,1,1,1,1,1,1,1,1,1,
1,1,1,1,1,1,1,6),(0.,0.0153846153846154,0.0307692307692308,0.0461538461538462,
0.0615384615384615,0.0769230769230769,0.0923076923076923,0.107692307692308,
0.123076923076923,0.138461538461538,0.153846153846154,0.169230769230769,
0.184615384615385,0.2,0.215384615384615,0.230769230769231,0.246153846153846,
0.261538461538462,0.276923076923077,0.292307692307692,0.307692307692308,
0.323076923076923,0.338461538461538,0.353846153846154,0.369230769230769,
0.384615384615385,0.4,0.415384615384615,0.430769230769231,0.446153846153846,
0.461538461538462,0.476923076923077,0.492307692307692,0.507692307692308,
0.523076923076923,0.538461538461538,0.553846153846154,0.569230769230769,
0.584615384615384,0.6,0.615384615384615,0.63076923076923,0.646153846153846,
0.661538461538461,0.676923076923076,0.692307692307692,0.707692307692307,
0.723076923076922,0.738461538461538,0.753846153846153,0.769230769230768,
0.784615384615384,0.799999999999999,0.815384615384614,0.83076923076923,
0.846153846153845,0.86153846153846,0.876923076923076,0.892307692307691,
0.907692307692306,0.923076923076922,0.938461538461537,0.953846153846152,
0.969230769230768,0.984615384615383,0.994228156739697),.UNSPECIFIED.)
CURVE()
GEOMETRIC_REPRESENTATION_ITEM()
RATIONAL_B_SPLINE_CURVE((1.,1.,1.,1.,1.,1.,1.,1.,1.,1.,1.,1.,1.,1.,1.,1.,
1.,1.,1.,1.,1.,1.,1.,1.,1.,1.,1.,1.,1.,1.,1.,1.,1.,1.,1.,1.,1.,1.,1.,1.,
1.,1.,1.,1.,1.,1.,1.,1.,1.,1.,1.,1.,1.,1.,1.,1.,1.,1.,1.,1.,1.,1.,1.,1.,
1.,1.,1.,1.,1.,1.))
REPRESENTATION_ITEM('')
);
#341=(
BOUNDED_CURVE()
B_SPLINE_CURVE(5,(#50362,#50363,#50364,#50365,#50366,#50367,#50368,#50369,
#50370,#50371,#50372,#50373,#50374,#50375,#50376,#50377,#50378,#50379,#50380,
#50381,#50382,#50383,#50384,#50385,#50386,#50387,#50388,#50389,#50390,#50391,
#50392,#50393,#50394,#50395,#50396,#50397,#50398,#50399,#50400,#50401,#50402,
#50403,#50404,#50405,#50406,#50407,#50408,#50409,#50410,#50411,#50412,#50413,
#50414,#50415,#50416,#50417,#50418,#50419,#50420,#50421,#50422,#50423,#50424,
#50425,#50426,#50427,#50428,#50429,#50430,#50431),.UNSPECIFIED.,.F.,.F.)
B_SPLINE_CURVE_WITH_KNOTS((6,1,1,1,1,1,1,1,1,1,1,1,1,1,1,1,1,1,1,1,1,1,
1,1,1,1,1,1,1,1,1,1,1,1,1,1,1,1,1,1,1,1,1,1,1,1,1,1,1,1,1,1,1,1,1,1,1,1,
1,1,1,1,1,1,1,6),(0.00577184337452306,0.0153846153846154,0.0307692307692308,
0.0461538461538462,0.0615384615384615,0.0769230769230769,0.0923076923076923,
0.107692307692308,0.123076923076923,0.138461538461538,0.153846153846154,
0.169230769230769,0.184615384615385,0.2,0.215384615384615,0.230769230769231,
0.246153846153846,0.261538461538462,0.276923076923077,0.292307692307692,
0.307692307692308,0.323076923076923,0.338461538461538,0.353846153846154,
0.369230769230769,0.384615384615385,0.4,0.415384615384615,0.430769230769231,
0.446153846153846,0.461538461538462,0.476923076923077,0.492307692307692,
0.507692307692308,0.523076923076923,0.538461538461538,0.553846153846154,
0.569230769230769,0.584615384615384,0.6,0.615384615384615,0.63076923076923,
0.646153846153846,0.661538461538461,0.676923076923076,0.692307692307692,
0.707692307692307,0.723076923076922,0.738461538461538,0.753846153846153,
0.769230769230768,0.784615384615384,0.799999999999999,0.815384615384614,
0.83076923076923,0.846153846153845,0.86153846153846,0.876923076923076,0.892307692307691,
0.907692307692306,0.923076923076922,0.938461538461537,0.953846153846152,
0.969230769230768,0.984615384615383,1.),.UNSPECIFIED.)
CURVE()
GEOMETRIC_REPRESENTATION_ITEM()
RATIONAL_B_SPLINE_CURVE((1.,1.,1.,1.,1.,1.,1.,1.,1.,1.,1.,1.,1.,1.,1.,1.,
1.,1.,1.,1.,1.,1.,1.,1.,1.,1.,1.,1.,1.,1.,1.,1.,1.,1.,1.,1.,1.,1.,1.,1.,
1.,1.,1.,1.,1.,1.,1.,1.,1.,1.,1.,1.,1.,1.,1.,1.,1.,1.,1.,1.,1.,1.,1.,1.,
1.,1.,1.,1.,1.,1.))
REPRESENTATION_ITEM('')
);
#342=(
BOUNDED_CURVE()
B_SPLINE_CURVE(5,(#50435,#50436,#50437,#50438,#50439,#50440,#50441,#50442,
#50443,#50444,#50445,#50446,#50447,#50448,#50449,#50450,#50451,#50452,#50453,
#50454,#50455,#50456,#50457,#50458,#50459,#50460,#50461,#50462,#50463,#50464,
#50465,#50466,#50467,#50468,#50469,#50470,#50471,#50472,#50473,#50474,#50475,
#50476,#50477,#50478,#50479,#50480,#50481,#50482,#50483,#50484,#50485,#50486,
#50487,#50488,#50489,#50490,#50491,#50492,#50493,#50494,#50495,#50496,#50497,
#50498,#50499,#50500,#50501,#50502,#50503,#50504),.UNSPECIFIED.,.F.,.F.)
B_SPLINE_CURVE_WITH_KNOTS((6,1,1,1,1,1,1,1,1,1,1,1,1,1,1,1,1,1,1,1,1,1,
1,1,1,1,1,1,1,1,1,1,1,1,1,1,1,1,1,1,1,1,1,1,1,1,1,1,1,1,1,1,1,1,1,1,1,1,
1,1,1,1,1,1,1,6),(0.,0.0153846153846154,0.0307692307692308,0.0461538461538462,
0.0615384615384615,0.0769230769230769,0.0923076923076923,0.107692307692308,
0.123076923076923,0.138461538461538,0.153846153846154,0.169230769230769,
0.184615384615385,0.2,0.215384615384615,0.230769230769231,0.246153846153846,
0.261538461538462,0.276923076923077,0.292307692307692,0.307692307692308,
0.323076923076923,0.338461538461538,0.353846153846154,0.369230769230769,
0.384615384615385,0.4,0.415384615384615,0.430769230769231,0.446153846153846,
0.461538461538462,0.476923076923077,0.492307692307692,0.507692307692308,
0.523076923076923,0.538461538461538,0.553846153846154,0.569230769230769,
0.584615384615384,0.6,0.615384615384615,0.63076923076923,0.646153846153846,
0.661538461538461,0.676923076923076,0.692307692307692,0.707692307692307,
0.723076923076922,0.738461538461538,0.753846153846153,0.769230769230768,
0.784615384615384,0.799999999999999,0.815384615384614,0.83076923076923,
0.846153846153845,0.86153846153846,0.876923076923076,0.892307692307691,
0.907692307692306,0.923076923076922,0.938461538461537,0.953846153846152,
0.969230769230768,0.984615384615383,0.994228156739688),.UNSPECIFIED.)
CURVE()
GEOMETRIC_REPRESENTATION_ITEM()
RATIONAL_B_SPLINE_CURVE((1.,1.,1.,1.,1.,1.,1.,1.,1.,1.,1.,1.,1.,1.,1.,1.,
1.,1.,1.,1.,1.,1.,1.,1.,1.,1.,1.,1.,1.,1.,1.,1.,1.,1.,1.,1.,1.,1.,1.,1.,
1.,1.,1.,1.,1.,1.,1.,1.,1.,1.,1.,1.,1.,1.,1.,1.,1.,1.,1.,1.,1.,1.,1.,1.,
1.,1.,1.,1.,1.,1.))
REPRESENTATION_ITEM('')
);
#343=(
BOUNDED_CURVE()
B_SPLINE_CURVE(5,(#50508,#50509,#50510,#50511,#50512,#50513,#50514,#50515,
#50516,#50517,#50518,#50519,#50520,#50521,#50522,#50523,#50524,#50525,#50526,
#50527,#50528,#50529,#50530,#50531,#50532,#50533,#50534,#50535,#50536,#50537,
#50538,#50539,#50540,#50541,#50542,#50543,#50544,#50545,#50546,#50547,#50548,
#50549,#50550,#50551,#50552,#50553,#50554,#50555,#50556,#50557,#50558,#50559,
#50560,#50561,#50562,#50563,#50564,#50565,#50566,#50567,#50568,#50569,#50570,
#50571,#50572,#50573,#50574,#50575,#50576,#50577),.UNSPECIFIED.,.F.,.F.)
B_SPLINE_CURVE_WITH_KNOTS((6,1,1,1,1,1,1,1,1,1,1,1,1,1,1,1,1,1,1,1,1,1,
1,1,1,1,1,1,1,1,1,1,1,1,1,1,1,1,1,1,1,1,1,1,1,1,1,1,1,1,1,1,1,1,1,1,1,1,
1,1,1,1,1,1,1,6),(0.00577184337449862,0.0153846153846154,0.0307692307692308,
0.0461538461538462,0.0615384615384615,0.0769230769230769,0.0923076923076923,
0.107692307692308,0.123076923076923,0.138461538461538,0.153846153846154,
0.169230769230769,0.184615384615385,0.2,0.215384615384615,0.230769230769231,
0.246153846153846,0.261538461538462,0.276923076923077,0.292307692307692,
0.307692307692308,0.323076923076923,0.338461538461538,0.353846153846154,
0.369230769230769,0.384615384615385,0.4,0.415384615384615,0.430769230769231,
0.446153846153846,0.461538461538462,0.476923076923077,0.492307692307692,
0.507692307692308,0.523076923076923,0.538461538461538,0.553846153846154,
0.569230769230769,0.584615384615384,0.6,0.615384615384615,0.63076923076923,
0.646153846153846,0.661538461538461,0.676923076923076,0.692307692307692,
0.707692307692307,0.723076923076922,0.738461538461538,0.753846153846153,
0.769230769230768,0.784615384615384,0.799999999999999,0.815384615384614,
0.83076923076923,0.846153846153845,0.86153846153846,0.876923076923076,0.892307692307691,
0.907692307692306,0.923076923076922,0.938461538461537,0.953846153846152,
0.969230769230768,0.984615384615383,1.),.UNSPECIFIED.)
CURVE()
GEOMETRIC_REPRESENTATION_ITEM()
RATIONAL_B_SPLINE_CURVE((1.,1.,1.,1.,1.,1.,1.,1.,1.,1.,1.,1.,1.,1.,1.,1.,
1.,1.,1.,1.,1.,1.,1.,1.,1.,1.,1.,1.,1.,1.,1.,1.,1.,1.,1.,1.,1.,1.,1.,1.,
1.,1.,1.,1.,1.,1.,1.,1.,1.,1.,1.,1.,1.,1.,1.,1.,1.,1.,1.,1.,1.,1.,1.,1.,
1.,1.,1.,1.,1.,1.))
REPRESENTATION_ITEM('')
);
#344=(
BOUNDED_CURVE()
B_SPLINE_CURVE(5,(#50581,#50582,#50583,#50584,#50585,#50586,#50587,#50588,
#50589,#50590,#50591,#50592,#50593,#50594,#50595,#50596,#50597,#50598,#50599,
#50600,#50601,#50602,#50603,#50604,#50605,#50606,#50607,#50608,#50609,#50610,
#50611,#50612,#50613,#50614,#50615,#50616,#50617,#50618,#50619,#50620,#50621,
#50622,#50623,#50624,#50625,#50626,#50627,#50628,#50629,#50630,#50631,#50632,
#50633,#50634,#50635,#50636,#50637,#50638,#50639,#50640,#50641,#50642,#50643,
#50644,#50645,#50646,#50647,#50648,#50649,#50650),.UNSPECIFIED.,.F.,.F.)
B_SPLINE_CURVE_WITH_KNOTS((6,1,1,1,1,1,1,1,1,1,1,1,1,1,1,1,1,1,1,1,1,1,
1,1,1,1,1,1,1,1,1,1,1,1,1,1,1,1,1,1,1,1,1,1,1,1,1,1,1,1,1,1,1,1,1,1,1,1,
1,1,1,1,1,1,1,6),(0.,0.0153846153846154,0.0307692307692308,0.0461538461538462,
0.0615384615384615,0.0769230769230769,0.0923076923076923,0.107692307692308,
0.123076923076923,0.138461538461538,0.153846153846154,0.169230769230769,
0.184615384615385,0.2,0.215384615384615,0.230769230769231,0.246153846153846,
0.261538461538462,0.276923076923077,0.292307692307692,0.307692307692308,
0.323076923076923,0.338461538461538,0.353846153846154,0.369230769230769,
0.384615384615385,0.4,0.415384615384615,0.430769230769231,0.446153846153846,
0.461538461538462,0.476923076923077,0.492307692307692,0.507692307692308,
0.523076923076923,0.538461538461538,0.553846153846154,0.569230769230769,
0.584615384615384,0.6,0.615384615384615,0.63076923076923,0.646153846153846,
0.661538461538461,0.676923076923076,0.692307692307692,0.707692307692307,
0.723076923076922,0.738461538461538,0.753846153846153,0.769230769230768,
0.784615384615384,0.799999999999999,0.815384615384614,0.83076923076923,
0.846153846153845,0.86153846153846,0.876923076923076,0.892307692307691,
0.907692307692306,0.923076923076922,0.938461538461537,0.953846153846152,
0.969230769230768,0.984615384615383,0.994228156739696),.UNSPECIFIED.)
CURVE()
GEOMETRIC_REPRESENTATION_ITEM()
RATIONAL_B_SPLINE_CURVE((1.,1.,1.,1.,1.,1.,1.,1.,1.,1.,1.,1.,1.,1.,1.,1.,
1.,1.,1.,1.,1.,1.,1.,1.,1.,1.,1.,1.,1.,1.,1.,1.,1.,1.,1.,1.,1.,1.,1.,1.,
1.,1.,1.,1.,1.,1.,1.,1.,1.,1.,1.,1.,1.,1.,1.,1.,1.,1.,1.,1.,1.,1.,1.,1.,
1.,1.,1.,1.,1.,1.))
REPRESENTATION_ITEM('')
);
#345=(
BOUNDED_CURVE()
B_SPLINE_CURVE(5,(#50654,#50655,#50656,#50657,#50658,#50659,#50660,#50661,
#50662,#50663,#50664,#50665,#50666,#50667,#50668,#50669,#50670,#50671,#50672,
#50673,#50674,#50675,#50676,#50677,#50678,#50679,#50680,#50681,#50682,#50683,
#50684,#50685,#50686,#50687,#50688,#50689,#50690,#50691,#50692,#50693,#50694,
#50695,#50696,#50697,#50698,#50699,#50700,#50701,#50702,#50703,#50704,#50705,
#50706,#50707,#50708,#50709,#50710,#50711,#50712,#50713,#50714,#50715,#50716,
#50717,#50718,#50719,#50720,#50721,#50722,#50723),.UNSPECIFIED.,.F.,.F.)
B_SPLINE_CURVE_WITH_KNOTS((6,1,1,1,1,1,1,1,1,1,1,1,1,1,1,1,1,1,1,1,1,1,
1,1,1,1,1,1,1,1,1,1,1,1,1,1,1,1,1,1,1,1,1,1,1,1,1,1,1,1,1,1,1,1,1,1,1,1,
1,1,1,1,1,1,1,6),(0.00577184337452068,0.0153846153846154,0.0307692307692308,
0.0461538461538462,0.0615384615384615,0.0769230769230769,0.0923076923076923,
0.107692307692308,0.123076923076923,0.138461538461538,0.153846153846154,
0.169230769230769,0.184615384615385,0.2,0.215384615384615,0.230769230769231,
0.246153846153846,0.261538461538462,0.276923076923077,0.292307692307692,
0.307692307692308,0.323076923076923,0.338461538461538,0.353846153846154,
0.369230769230769,0.384615384615385,0.4,0.415384615384615,0.430769230769231,
0.446153846153846,0.461538461538462,0.476923076923077,0.492307692307692,
0.507692307692308,0.523076923076923,0.538461538461538,0.553846153846154,
0.569230769230769,0.584615384615384,0.6,0.615384615384615,0.63076923076923,
0.646153846153846,0.661538461538461,0.676923076923076,0.692307692307692,
0.707692307692307,0.723076923076922,0.738461538461538,0.753846153846153,
0.769230769230768,0.784615384615384,0.799999999999999,0.815384615384614,
0.83076923076923,0.846153846153845,0.86153846153846,0.876923076923076,0.892307692307691,
0.907692307692306,0.923076923076922,0.938461538461537,0.953846153846152,
0.969230769230768,0.984615384615383,1.),.UNSPECIFIED.)
CURVE()
GEOMETRIC_REPRESENTATION_ITEM()
RATIONAL_B_SPLINE_CURVE((1.,1.,1.,1.,1.,1.,1.,1.,1.,1.,1.,1.,1.,1.,1.,1.,
1.,1.,1.,1.,1.,1.,1.,1.,1.,1.,1.,1.,1.,1.,1.,1.,1.,1.,1.,1.,1.,1.,1.,1.,
1.,1.,1.,1.,1.,1.,1.,1.,1.,1.,1.,1.,1.,1.,1.,1.,1.,1.,1.,1.,1.,1.,1.,1.,
1.,1.,1.,1.,1.,1.))
REPRESENTATION_ITEM('')
);
#346=(
BOUNDED_CURVE()
B_SPLINE_CURVE(5,(#50727,#50728,#50729,#50730,#50731,#50732,#50733,#50734,
#50735,#50736,#50737,#50738,#50739,#50740,#50741,#50742,#50743,#50744,#50745,
#50746,#50747,#50748,#50749,#50750,#50751,#50752,#50753,#50754,#50755,#50756,
#50757,#50758,#50759,#50760,#50761,#50762,#50763,#50764,#50765,#50766,#50767,
#50768,#50769,#50770,#50771,#50772,#50773,#50774,#50775,#50776,#50777,#50778,
#50779,#50780,#50781,#50782,#50783,#50784,#50785,#50786,#50787,#50788,#50789,
#50790,#50791,#50792,#50793,#50794,#50795,#50796),.UNSPECIFIED.,.F.,.F.)
B_SPLINE_CURVE_WITH_KNOTS((6,1,1,1,1,1,1,1,1,1,1,1,1,1,1,1,1,1,1,1,1,1,
1,1,1,1,1,1,1,1,1,1,1,1,1,1,1,1,1,1,1,1,1,1,1,1,1,1,1,1,1,1,1,1,1,1,1,1,
1,1,1,1,1,1,1,6),(0.,0.0153846153846154,0.0307692307692308,0.0461538461538462,
0.0615384615384615,0.0769230769230769,0.0923076923076923,0.107692307692308,
0.123076923076923,0.138461538461538,0.153846153846154,0.169230769230769,
0.184615384615385,0.2,0.215384615384615,0.230769230769231,0.246153846153846,
0.261538461538462,0.276923076923077,0.292307692307692,0.307692307692308,
0.323076923076923,0.338461538461538,0.353846153846154,0.369230769230769,
0.384615384615385,0.4,0.415384615384615,0.430769230769231,0.446153846153846,
0.461538461538462,0.476923076923077,0.492307692307692,0.507692307692308,
0.523076923076923,0.538461538461538,0.553846153846154,0.569230769230769,
0.584615384615384,0.6,0.615384615384615,0.63076923076923,0.646153846153846,
0.661538461538461,0.676923076923076,0.692307692307692,0.707692307692307,
0.723076923076922,0.738461538461538,0.753846153846153,0.769230769230768,
0.784615384615384,0.799999999999999,0.815384615384614,0.83076923076923,
0.846153846153845,0.86153846153846,0.876923076923076,0.892307692307691,
0.907692307692306,0.923076923076922,0.938461538461537,0.953846153846152,
0.969230769230768,0.984615384615383,0.994228156739698),.UNSPECIFIED.)
CURVE()
GEOMETRIC_REPRESENTATION_ITEM()
RATIONAL_B_SPLINE_CURVE((1.,1.,1.,1.,1.,1.,1.,1.,1.,1.,1.,1.,1.,1.,1.,1.,
1.,1.,1.,1.,1.,1.,1.,1.,1.,1.,1.,1.,1.,1.,1.,1.,1.,1.,1.,1.,1.,1.,1.,1.,
1.,1.,1.,1.,1.,1.,1.,1.,1.,1.,1.,1.,1.,1.,1.,1.,1.,1.,1.,1.,1.,1.,1.,1.,
1.,1.,1.,1.,1.,1.))
REPRESENTATION_ITEM('')
);
#347=(
BOUNDED_CURVE()
B_SPLINE_CURVE(5,(#50800,#50801,#50802,#50803,#50804,#50805,#50806,#50807,
#50808,#50809,#50810,#50811,#50812,#50813,#50814,#50815,#50816,#50817,#50818,
#50819,#50820,#50821,#50822,#50823,#50824,#50825,#50826,#50827,#50828,#50829,
#50830,#50831,#50832,#50833,#50834,#50835,#50836,#50837,#50838,#50839,#50840,
#50841,#50842,#50843,#50844,#50845,#50846,#50847,#50848,#50849,#50850,#50851,
#50852,#50853,#50854,#50855,#50856,#50857,#50858,#50859,#50860,#50861,#50862,
#50863,#50864,#50865,#50866,#50867,#50868,#50869),.UNSPECIFIED.,.F.,.F.)
B_SPLINE_CURVE_WITH_KNOTS((6,1,1,1,1,1,1,1,1,1,1,1,1,1,1,1,1,1,1,1,1,1,
1,1,1,1,1,1,1,1,1,1,1,1,1,1,1,1,1,1,1,1,1,1,1,1,1,1,1,1,1,1,1,1,1,1,1,1,
1,1,1,1,1,1,1,6),(0.00577184337451607,0.0153846153846154,0.0307692307692308,
0.0461538461538462,0.0615384615384615,0.0769230769230769,0.0923076923076923,
0.107692307692308,0.123076923076923,0.138461538461538,0.153846153846154,
0.169230769230769,0.184615384615385,0.2,0.215384615384615,0.230769230769231,
0.246153846153846,0.261538461538462,0.276923076923077,0.292307692307692,
0.307692307692308,0.323076923076923,0.338461538461538,0.353846153846154,
0.369230769230769,0.384615384615385,0.4,0.415384615384615,0.430769230769231,
0.446153846153846,0.461538461538462,0.476923076923077,0.492307692307692,
0.507692307692308,0.523076923076923,0.538461538461538,0.553846153846154,
0.569230769230769,0.584615384615384,0.6,0.615384615384615,0.63076923076923,
0.646153846153846,0.661538461538461,0.676923076923076,0.692307692307692,
0.707692307692307,0.723076923076922,0.738461538461538,0.753846153846153,
0.769230769230768,0.784615384615384,0.799999999999999,0.815384615384614,
0.83076923076923,0.846153846153845,0.86153846153846,0.876923076923076,0.892307692307691,
0.907692307692306,0.923076923076922,0.938461538461537,0.953846153846152,
0.969230769230768,0.984615384615383,1.),.UNSPECIFIED.)
CURVE()
GEOMETRIC_REPRESENTATION_ITEM()
RATIONAL_B_SPLINE_CURVE((1.,1.,1.,1.,1.,1.,1.,1.,1.,1.,1.,1.,1.,1.,1.,1.,
1.,1.,1.,1.,1.,1.,1.,1.,1.,1.,1.,1.,1.,1.,1.,1.,1.,1.,1.,1.,1.,1.,1.,1.,
1.,1.,1.,1.,1.,1.,1.,1.,1.,1.,1.,1.,1.,1.,1.,1.,1.,1.,1.,1.,1.,1.,1.,1.,
1.,1.,1.,1.,1.,1.))
REPRESENTATION_ITEM('')
);
#348=(
BOUNDED_CURVE()
B_SPLINE_CURVE(5,(#50873,#50874,#50875,#50876,#50877,#50878,#50879,#50880,
#50881,#50882,#50883,#50884,#50885,#50886,#50887,#50888,#50889,#50890,#50891,
#50892,#50893,#50894,#50895,#50896,#50897,#50898,#50899,#50900,#50901,#50902,
#50903,#50904,#50905,#50906,#50907,#50908,#50909,#50910,#50911,#50912,#50913,
#50914,#50915,#50916,#50917,#50918,#50919,#50920,#50921,#50922,#50923,#50924,
#50925,#50926,#50927,#50928,#50929,#50930,#50931,#50932,#50933,#50934,#50935,
#50936,#50937,#50938,#50939,#50940,#50941,#50942),.UNSPECIFIED.,.F.,.F.)
B_SPLINE_CURVE_WITH_KNOTS((6,1,1,1,1,1,1,1,1,1,1,1,1,1,1,1,1,1,1,1,1,1,
1,1,1,1,1,1,1,1,1,1,1,1,1,1,1,1,1,1,1,1,1,1,1,1,1,1,1,1,1,1,1,1,1,1,1,1,
1,1,1,1,1,1,1,6),(0.,0.0153846153846154,0.0307692307692308,0.0461538461538462,
0.0615384615384615,0.0769230769230769,0.0923076923076923,0.107692307692308,
0.123076923076923,0.138461538461538,0.153846153846154,0.169230769230769,
0.184615384615385,0.2,0.215384615384615,0.230769230769231,0.246153846153846,
0.261538461538462,0.276923076923077,0.292307692307692,0.307692307692308,
0.323076923076923,0.338461538461538,0.353846153846154,0.369230769230769,
0.384615384615385,0.4,0.415384615384615,0.430769230769231,0.446153846153846,
0.461538461538462,0.476923076923077,0.492307692307692,0.507692307692308,
0.523076923076923,0.538461538461538,0.553846153846154,0.569230769230769,
0.584615384615384,0.6,0.615384615384615,0.63076923076923,0.646153846153846,
0.661538461538461,0.676923076923076,0.692307692307692,0.707692307692307,
0.723076923076922,0.738461538461538,0.753846153846153,0.769230769230768,
0.784615384615384,0.799999999999999,0.815384615384614,0.83076923076923,
0.846153846153845,0.86153846153846,0.876923076923076,0.892307692307691,
0.907692307692306,0.923076923076922,0.938461538461537,0.953846153846152,
0.969230769230768,0.984615384615383,0.994228156739704),.UNSPECIFIED.)
CURVE()
GEOMETRIC_REPRESENTATION_ITEM()
RATIONAL_B_SPLINE_CURVE((1.,1.,1.,1.,1.,1.,1.,1.,1.,1.,1.,1.,1.,1.,1.,1.,
1.,1.,1.,1.,1.,1.,1.,1.,1.,1.,1.,1.,1.,1.,1.,1.,1.,1.,1.,1.,1.,1.,1.,1.,
1.,1.,1.,1.,1.,1.,1.,1.,1.,1.,1.,1.,1.,1.,1.,1.,1.,1.,1.,1.,1.,1.,1.,1.,
1.,1.,1.,1.,1.,1.))
REPRESENTATION_ITEM('')
);
#349=(
BOUNDED_CURVE()
B_SPLINE_CURVE(5,(#50946,#50947,#50948,#50949,#50950,#50951,#50952,#50953,
#50954,#50955,#50956,#50957,#50958,#50959,#50960,#50961,#50962,#50963,#50964,
#50965,#50966,#50967,#50968,#50969,#50970,#50971,#50972,#50973,#50974,#50975,
#50976,#50977,#50978,#50979,#50980,#50981,#50982,#50983,#50984,#50985,#50986,
#50987,#50988,#50989,#50990,#50991,#50992,#50993,#50994,#50995,#50996,#50997,
#50998,#50999,#51000,#51001,#51002,#51003,#51004,#51005,#51006,#51007,#51008,
#51009,#51010,#51011,#51012,#51013,#51014,#51015),.UNSPECIFIED.,.F.,.F.)
B_SPLINE_CURVE_WITH_KNOTS((6,1,1,1,1,1,1,1,1,1,1,1,1,1,1,1,1,1,1,1,1,1,
1,1,1,1,1,1,1,1,1,1,1,1,1,1,1,1,1,1,1,1,1,1,1,1,1,1,1,1,1,1,1,1,1,1,1,1,
1,1,1,1,1,1,1,6),(0.00577184337449692,0.0153846153846154,0.0307692307692308,
0.0461538461538462,0.0615384615384615,0.0769230769230769,0.0923076923076923,
0.107692307692308,0.123076923076923,0.138461538461538,0.153846153846154,
0.169230769230769,0.184615384615385,0.2,0.215384615384615,0.230769230769231,
0.246153846153846,0.261538461538462,0.276923076923077,0.292307692307692,
0.307692307692308,0.323076923076923,0.338461538461538,0.353846153846154,
0.369230769230769,0.384615384615385,0.4,0.415384615384615,0.430769230769231,
0.446153846153846,0.461538461538462,0.476923076923077,0.492307692307692,
0.507692307692308,0.523076923076923,0.538461538461538,0.553846153846154,
0.569230769230769,0.584615384615384,0.6,0.615384615384615,0.63076923076923,
0.646153846153846,0.661538461538461,0.676923076923076,0.692307692307692,
0.707692307692307,0.723076923076922,0.738461538461538,0.753846153846153,
0.769230769230768,0.784615384615384,0.799999999999999,0.815384615384614,
0.83076923076923,0.846153846153845,0.86153846153846,0.876923076923076,0.892307692307691,
0.907692307692306,0.923076923076922,0.938461538461537,0.953846153846152,
0.969230769230768,0.984615384615383,1.),.UNSPECIFIED.)
CURVE()
GEOMETRIC_REPRESENTATION_ITEM()
RATIONAL_B_SPLINE_CURVE((1.,1.,1.,1.,1.,1.,1.,1.,1.,1.,1.,1.,1.,1.,1.,1.,
1.,1.,1.,1.,1.,1.,1.,1.,1.,1.,1.,1.,1.,1.,1.,1.,1.,1.,1.,1.,1.,1.,1.,1.,
1.,1.,1.,1.,1.,1.,1.,1.,1.,1.,1.,1.,1.,1.,1.,1.,1.,1.,1.,1.,1.,1.,1.,1.,
1.,1.,1.,1.,1.,1.))
REPRESENTATION_ITEM('')
);
#350=(
BOUNDED_CURVE()
B_SPLINE_CURVE(5,(#51019,#51020,#51021,#51022,#51023,#51024,#51025,#51026,
#51027,#51028,#51029,#51030,#51031,#51032,#51033,#51034,#51035,#51036,#51037,
#51038,#51039,#51040,#51041,#51042,#51043,#51044,#51045,#51046,#51047,#51048,
#51049,#51050,#51051,#51052,#51053,#51054,#51055,#51056,#51057,#51058,#51059,
#51060,#51061,#51062,#51063,#51064,#51065,#51066,#51067,#51068,#51069,#51070,
#51071,#51072,#51073,#51074,#51075,#51076,#51077,#51078,#51079,#51080,#51081,
#51082,#51083,#51084,#51085,#51086,#51087,#51088),.UNSPECIFIED.,.F.,.F.)
B_SPLINE_CURVE_WITH_KNOTS((6,1,1,1,1,1,1,1,1,1,1,1,1,1,1,1,1,1,1,1,1,1,
1,1,1,1,1,1,1,1,1,1,1,1,1,1,1,1,1,1,1,1,1,1,1,1,1,1,1,1,1,1,1,1,1,1,1,1,
1,1,1,1,1,1,1,6),(0.,0.0153846153846154,0.0307692307692308,0.0461538461538462,
0.0615384615384615,0.0769230769230769,0.0923076923076923,0.107692307692308,
0.123076923076923,0.138461538461538,0.153846153846154,0.169230769230769,
0.184615384615385,0.2,0.215384615384615,0.230769230769231,0.246153846153846,
0.261538461538462,0.276923076923077,0.292307692307692,0.307692307692308,
0.323076923076923,0.338461538461538,0.353846153846154,0.369230769230769,
0.384615384615385,0.4,0.415384615384615,0.430769230769231,0.446153846153846,
0.461538461538462,0.476923076923077,0.492307692307692,0.507692307692308,
0.523076923076923,0.538461538461538,0.553846153846154,0.569230769230769,
0.584615384615384,0.6,0.615384615384615,0.63076923076923,0.646153846153846,
0.661538461538461,0.676923076923076,0.692307692307692,0.707692307692307,
0.723076923076922,0.738461538461538,0.753846153846153,0.769230769230768,
0.784615384615384,0.799999999999999,0.815384615384614,0.83076923076923,
0.846153846153845,0.86153846153846,0.876923076923076,0.892307692307691,
0.907692307692306,0.923076923076922,0.938461538461537,0.953846153846152,
0.969230769230768,0.984615384615383,0.994228156739711),.UNSPECIFIED.)
CURVE()
GEOMETRIC_REPRESENTATION_ITEM()
RATIONAL_B_SPLINE_CURVE((1.,1.,1.,1.,1.,1.,1.,1.,1.,1.,1.,1.,1.,1.,1.,1.,
1.,1.,1.,1.,1.,1.,1.,1.,1.,1.,1.,1.,1.,1.,1.,1.,1.,1.,1.,1.,1.,1.,1.,1.,
1.,1.,1.,1.,1.,1.,1.,1.,1.,1.,1.,1.,1.,1.,1.,1.,1.,1.,1.,1.,1.,1.,1.,1.,
1.,1.,1.,1.,1.,1.))
REPRESENTATION_ITEM('')
);
#351=(
BOUNDED_CURVE()
B_SPLINE_CURVE(5,(#51092,#51093,#51094,#51095,#51096,#51097,#51098,#51099,
#51100,#51101,#51102,#51103,#51104,#51105,#51106,#51107,#51108,#51109,#51110,
#51111,#51112,#51113,#51114,#51115,#51116,#51117,#51118,#51119,#51120,#51121,
#51122,#51123,#51124,#51125,#51126,#51127,#51128,#51129,#51130,#51131,#51132,
#51133,#51134,#51135,#51136,#51137,#51138,#51139,#51140,#51141,#51142,#51143,
#51144,#51145,#51146,#51147,#51148,#51149,#51150,#51151,#51152,#51153,#51154,
#51155,#51156,#51157,#51158,#51159,#51160,#51161),.UNSPECIFIED.,.F.,.F.)
B_SPLINE_CURVE_WITH_KNOTS((6,1,1,1,1,1,1,1,1,1,1,1,1,1,1,1,1,1,1,1,1,1,
1,1,1,1,1,1,1,1,1,1,1,1,1,1,1,1,1,1,1,1,1,1,1,1,1,1,1,1,1,1,1,1,1,1,1,1,
1,1,1,1,1,1,1,6),(0.00577184337450058,0.0153846153846154,0.0307692307692308,
0.0461538461538462,0.0615384615384615,0.0769230769230769,0.0923076923076923,
0.107692307692308,0.123076923076923,0.138461538461538,0.153846153846154,
0.169230769230769,0.184615384615385,0.2,0.215384615384615,0.230769230769231,
0.246153846153846,0.261538461538462,0.276923076923077,0.292307692307692,
0.307692307692308,0.323076923076923,0.338461538461538,0.353846153846154,
0.369230769230769,0.384615384615385,0.4,0.415384615384615,0.430769230769231,
0.446153846153846,0.461538461538462,0.476923076923077,0.492307692307692,
0.507692307692308,0.523076923076923,0.538461538461538,0.553846153846154,
0.569230769230769,0.584615384615384,0.6,0.615384615384615,0.63076923076923,
0.646153846153846,0.661538461538461,0.676923076923076,0.692307692307692,
0.707692307692307,0.723076923076922,0.738461538461538,0.753846153846153,
0.769230769230768,0.784615384615384,0.799999999999999,0.815384615384614,
0.83076923076923,0.846153846153845,0.86153846153846,0.876923076923076,0.892307692307691,
0.907692307692306,0.923076923076922,0.938461538461537,0.953846153846152,
0.969230769230768,0.984615384615383,1.),.UNSPECIFIED.)
CURVE()
GEOMETRIC_REPRESENTATION_ITEM()
RATIONAL_B_SPLINE_CURVE((1.,1.,1.,1.,1.,1.,1.,1.,1.,1.,1.,1.,1.,1.,1.,1.,
1.,1.,1.,1.,1.,1.,1.,1.,1.,1.,1.,1.,1.,1.,1.,1.,1.,1.,1.,1.,1.,1.,1.,1.,
1.,1.,1.,1.,1.,1.,1.,1.,1.,1.,1.,1.,1.,1.,1.,1.,1.,1.,1.,1.,1.,1.,1.,1.,
1.,1.,1.,1.,1.,1.))
REPRESENTATION_ITEM('')
);
#352=(
BOUNDED_CURVE()
B_SPLINE_CURVE(5,(#51165,#51166,#51167,#51168,#51169,#51170,#51171,#51172,
#51173,#51174,#51175,#51176,#51177,#51178,#51179,#51180,#51181,#51182,#51183,
#51184,#51185,#51186,#51187,#51188,#51189,#51190,#51191,#51192,#51193,#51194,
#51195,#51196,#51197,#51198,#51199,#51200,#51201,#51202,#51203,#51204,#51205,
#51206,#51207,#51208,#51209,#51210,#51211,#51212,#51213,#51214,#51215,#51216,
#51217,#51218,#51219,#51220,#51221,#51222,#51223,#51224,#51225,#51226,#51227,
#51228,#51229,#51230,#51231,#51232,#51233,#51234),.UNSPECIFIED.,.F.,.F.)
B_SPLINE_CURVE_WITH_KNOTS((6,1,1,1,1,1,1,1,1,1,1,1,1,1,1,1,1,1,1,1,1,1,
1,1,1,1,1,1,1,1,1,1,1,1,1,1,1,1,1,1,1,1,1,1,1,1,1,1,1,1,1,1,1,1,1,1,1,1,
1,1,1,1,1,1,1,6),(0.,0.0153846153846154,0.0307692307692308,0.0461538461538462,
0.0615384615384615,0.0769230769230769,0.0923076923076923,0.107692307692308,
0.123076923076923,0.138461538461538,0.153846153846154,0.169230769230769,
0.184615384615385,0.2,0.215384615384615,0.230769230769231,0.246153846153846,
0.261538461538462,0.276923076923077,0.292307692307692,0.307692307692308,
0.323076923076923,0.338461538461538,0.353846153846154,0.369230769230769,
0.384615384615385,0.4,0.415384615384615,0.430769230769231,0.446153846153846,
0.461538461538462,0.476923076923077,0.492307692307692,0.507692307692308,
0.523076923076923,0.538461538461538,0.553846153846154,0.569230769230769,
0.584615384615384,0.6,0.615384615384615,0.63076923076923,0.646153846153846,
0.661538461538461,0.676923076923076,0.692307692307692,0.707692307692307,
0.723076923076922,0.738461538461538,0.753846153846153,0.769230769230768,
0.784615384615384,0.799999999999999,0.815384615384614,0.83076923076923,
0.846153846153845,0.86153846153846,0.876923076923076,0.892307692307691,
0.907692307692306,0.923076923076922,0.938461538461537,0.953846153846152,
0.969230769230768,0.984615384615383,0.994228156739701),.UNSPECIFIED.)
CURVE()
GEOMETRIC_REPRESENTATION_ITEM()
RATIONAL_B_SPLINE_CURVE((1.,1.,1.,1.,1.,1.,1.,1.,1.,1.,1.,1.,1.,1.,1.,1.,
1.,1.,1.,1.,1.,1.,1.,1.,1.,1.,1.,1.,1.,1.,1.,1.,1.,1.,1.,1.,1.,1.,1.,1.,
1.,1.,1.,1.,1.,1.,1.,1.,1.,1.,1.,1.,1.,1.,1.,1.,1.,1.,1.,1.,1.,1.,1.,1.,
1.,1.,1.,1.,1.,1.))
REPRESENTATION_ITEM('')
);
#353=(
BOUNDED_CURVE()
B_SPLINE_CURVE(5,(#51238,#51239,#51240,#51241,#51242,#51243,#51244,#51245,
#51246,#51247,#51248,#51249,#51250,#51251,#51252,#51253,#51254,#51255,#51256,
#51257,#51258,#51259,#51260,#51261,#51262,#51263,#51264,#51265,#51266,#51267,
#51268,#51269,#51270,#51271,#51272,#51273,#51274,#51275,#51276,#51277,#51278,
#51279,#51280,#51281,#51282,#51283,#51284,#51285,#51286,#51287,#51288,#51289,
#51290,#51291,#51292,#51293,#51294,#51295,#51296,#51297,#51298,#51299,#51300,
#51301,#51302,#51303,#51304,#51305,#51306,#51307),.UNSPECIFIED.,.F.,.F.)
B_SPLINE_CURVE_WITH_KNOTS((6,1,1,1,1,1,1,1,1,1,1,1,1,1,1,1,1,1,1,1,1,1,
1,1,1,1,1,1,1,1,1,1,1,1,1,1,1,1,1,1,1,1,1,1,1,1,1,1,1,1,1,1,1,1,1,1,1,1,
1,1,1,1,1,1,1,6),(0.0057718433745091,0.0153846153846154,0.0307692307692308,
0.0461538461538462,0.0615384615384615,0.0769230769230769,0.0923076923076923,
0.107692307692308,0.123076923076923,0.138461538461538,0.153846153846154,
0.169230769230769,0.184615384615385,0.2,0.215384615384615,0.230769230769231,
0.246153846153846,0.261538461538462,0.276923076923077,0.292307692307692,
0.307692307692308,0.323076923076923,0.338461538461538,0.353846153846154,
0.369230769230769,0.384615384615385,0.4,0.415384615384615,0.430769230769231,
0.446153846153846,0.461538461538462,0.476923076923077,0.492307692307692,
0.507692307692308,0.523076923076923,0.538461538461538,0.553846153846154,
0.569230769230769,0.584615384615384,0.6,0.615384615384615,0.63076923076923,
0.646153846153846,0.661538461538461,0.676923076923076,0.692307692307692,
0.707692307692307,0.723076923076922,0.738461538461538,0.753846153846153,
0.769230769230768,0.784615384615384,0.799999999999999,0.815384615384614,
0.83076923076923,0.846153846153845,0.86153846153846,0.876923076923076,0.892307692307691,
0.907692307692306,0.923076923076922,0.938461538461537,0.953846153846152,
0.969230769230768,0.984615384615383,1.),.UNSPECIFIED.)
CURVE()
GEOMETRIC_REPRESENTATION_ITEM()
RATIONAL_B_SPLINE_CURVE((1.,1.,1.,1.,1.,1.,1.,1.,1.,1.,1.,1.,1.,1.,1.,1.,
1.,1.,1.,1.,1.,1.,1.,1.,1.,1.,1.,1.,1.,1.,1.,1.,1.,1.,1.,1.,1.,1.,1.,1.,
1.,1.,1.,1.,1.,1.,1.,1.,1.,1.,1.,1.,1.,1.,1.,1.,1.,1.,1.,1.,1.,1.,1.,1.,
1.,1.,1.,1.,1.,1.))
REPRESENTATION_ITEM('')
);
#354=(
BOUNDED_CURVE()
B_SPLINE_CURVE(5,(#51311,#51312,#51313,#51314,#51315,#51316,#51317,#51318,
#51319,#51320,#51321,#51322,#51323,#51324,#51325,#51326,#51327,#51328,#51329,
#51330,#51331,#51332,#51333,#51334,#51335,#51336,#51337,#51338,#51339,#51340,
#51341,#51342,#51343,#51344,#51345,#51346,#51347,#51348,#51349,#51350,#51351,
#51352,#51353,#51354,#51355,#51356,#51357,#51358,#51359,#51360,#51361,#51362,
#51363,#51364,#51365,#51366,#51367,#51368,#51369,#51370,#51371,#51372,#51373,
#51374,#51375,#51376,#51377,#51378,#51379,#51380),.UNSPECIFIED.,.F.,.F.)
B_SPLINE_CURVE_WITH_KNOTS((6,1,1,1,1,1,1,1,1,1,1,1,1,1,1,1,1,1,1,1,1,1,
1,1,1,1,1,1,1,1,1,1,1,1,1,1,1,1,1,1,1,1,1,1,1,1,1,1,1,1,1,1,1,1,1,1,1,1,
1,1,1,1,1,1,1,6),(0.,0.0153846153846154,0.0307692307692308,0.0461538461538462,
0.0615384615384615,0.0769230769230769,0.0923076923076923,0.107692307692308,
0.123076923076923,0.138461538461538,0.153846153846154,0.169230769230769,
0.184615384615385,0.2,0.215384615384615,0.230769230769231,0.246153846153846,
0.261538461538462,0.276923076923077,0.292307692307692,0.307692307692308,
0.323076923076923,0.338461538461538,0.353846153846154,0.369230769230769,
0.384615384615385,0.4,0.415384615384615,0.430769230769231,0.446153846153846,
0.461538461538462,0.476923076923077,0.492307692307692,0.507692307692308,
0.523076923076923,0.538461538461538,0.553846153846154,0.569230769230769,
0.584615384615384,0.6,0.615384615384615,0.63076923076923,0.646153846153846,
0.661538461538461,0.676923076923076,0.692307692307692,0.707692307692307,
0.723076923076922,0.738461538461538,0.753846153846153,0.769230769230768,
0.784615384615384,0.799999999999999,0.815384615384614,0.83076923076923,
0.846153846153845,0.86153846153846,0.876923076923076,0.892307692307691,
0.907692307692306,0.923076923076922,0.938461538461537,0.953846153846152,
0.969230769230768,0.984615384615383,0.994228156739689),.UNSPECIFIED.)
CURVE()
GEOMETRIC_REPRESENTATION_ITEM()
RATIONAL_B_SPLINE_CURVE((1.,1.,1.,1.,1.,1.,1.,1.,1.,1.,1.,1.,1.,1.,1.,1.,
1.,1.,1.,1.,1.,1.,1.,1.,1.,1.,1.,1.,1.,1.,1.,1.,1.,1.,1.,1.,1.,1.,1.,1.,
1.,1.,1.,1.,1.,1.,1.,1.,1.,1.,1.,1.,1.,1.,1.,1.,1.,1.,1.,1.,1.,1.,1.,1.,
1.,1.,1.,1.,1.,1.))
REPRESENTATION_ITEM('')
);
#355=(
BOUNDED_CURVE()
B_SPLINE_CURVE(5,(#51384,#51385,#51386,#51387,#51388,#51389,#51390,#51391,
#51392,#51393,#51394,#51395,#51396,#51397,#51398,#51399,#51400,#51401,#51402,
#51403,#51404,#51405,#51406,#51407,#51408,#51409,#51410,#51411,#51412,#51413,
#51414,#51415,#51416,#51417,#51418,#51419,#51420,#51421,#51422,#51423,#51424,
#51425,#51426,#51427,#51428,#51429,#51430,#51431,#51432,#51433,#51434,#51435,
#51436,#51437,#51438,#51439,#51440,#51441,#51442,#51443,#51444,#51445,#51446,
#51447,#51448,#51449,#51450,#51451,#51452,#51453),.UNSPECIFIED.,.F.,.F.)
B_SPLINE_CURVE_WITH_KNOTS((6,1,1,1,1,1,1,1,1,1,1,1,1,1,1,1,1,1,1,1,1,1,
1,1,1,1,1,1,1,1,1,1,1,1,1,1,1,1,1,1,1,1,1,1,1,1,1,1,1,1,1,1,1,1,1,1,1,1,
1,1,1,1,1,1,1,6),(0.00577184337450777,0.0153846153846154,0.0307692307692308,
0.0461538461538462,0.0615384615384615,0.0769230769230769,0.0923076923076923,
0.107692307692308,0.123076923076923,0.138461538461538,0.153846153846154,
0.169230769230769,0.184615384615385,0.2,0.215384615384615,0.230769230769231,
0.246153846153846,0.261538461538462,0.276923076923077,0.292307692307692,
0.307692307692308,0.323076923076923,0.338461538461538,0.353846153846154,
0.369230769230769,0.384615384615385,0.4,0.415384615384615,0.430769230769231,
0.446153846153846,0.461538461538462,0.476923076923077,0.492307692307692,
0.507692307692308,0.523076923076923,0.538461538461538,0.553846153846154,
0.569230769230769,0.584615384615384,0.6,0.615384615384615,0.63076923076923,
0.646153846153846,0.661538461538461,0.676923076923076,0.692307692307692,
0.707692307692307,0.723076923076922,0.738461538461538,0.753846153846153,
0.769230769230768,0.784615384615384,0.799999999999999,0.815384615384614,
0.83076923076923,0.846153846153845,0.86153846153846,0.876923076923076,0.892307692307691,
0.907692307692306,0.923076923076922,0.938461538461537,0.953846153846152,
0.969230769230768,0.984615384615383,1.),.UNSPECIFIED.)
CURVE()
GEOMETRIC_REPRESENTATION_ITEM()
RATIONAL_B_SPLINE_CURVE((1.,1.,1.,1.,1.,1.,1.,1.,1.,1.,1.,1.,1.,1.,1.,1.,
1.,1.,1.,1.,1.,1.,1.,1.,1.,1.,1.,1.,1.,1.,1.,1.,1.,1.,1.,1.,1.,1.,1.,1.,
1.,1.,1.,1.,1.,1.,1.,1.,1.,1.,1.,1.,1.,1.,1.,1.,1.,1.,1.,1.,1.,1.,1.,1.,
1.,1.,1.,1.,1.,1.))
REPRESENTATION_ITEM('')
);
#356=(
BOUNDED_CURVE()
B_SPLINE_CURVE(5,(#51457,#51458,#51459,#51460,#51461,#51462,#51463,#51464,
#51465,#51466,#51467,#51468,#51469,#51470,#51471,#51472,#51473,#51474,#51475,
#51476,#51477,#51478,#51479,#51480,#51481,#51482,#51483,#51484,#51485,#51486,
#51487,#51488,#51489,#51490,#51491,#51492,#51493,#51494,#51495,#51496,#51497,
#51498,#51499,#51500,#51501,#51502,#51503,#51504,#51505,#51506,#51507,#51508,
#51509,#51510,#51511,#51512,#51513,#51514,#51515,#51516,#51517,#51518,#51519,
#51520,#51521,#51522,#51523,#51524,#51525,#51526),.UNSPECIFIED.,.F.,.F.)
B_SPLINE_CURVE_WITH_KNOTS((6,1,1,1,1,1,1,1,1,1,1,1,1,1,1,1,1,1,1,1,1,1,
1,1,1,1,1,1,1,1,1,1,1,1,1,1,1,1,1,1,1,1,1,1,1,1,1,1,1,1,1,1,1,1,1,1,1,1,
1,1,1,1,1,1,1,6),(0.,0.0153846153846154,0.0307692307692308,0.0461538461538462,
0.0615384615384615,0.0769230769230769,0.0923076923076923,0.107692307692308,
0.123076923076923,0.138461538461538,0.153846153846154,0.169230769230769,
0.184615384615385,0.2,0.215384615384615,0.230769230769231,0.246153846153846,
0.261538461538462,0.276923076923077,0.292307692307692,0.307692307692308,
0.323076923076923,0.338461538461538,0.353846153846154,0.369230769230769,
0.384615384615385,0.4,0.415384615384615,0.430769230769231,0.446153846153846,
0.461538461538462,0.476923076923077,0.492307692307692,0.507692307692308,
0.523076923076923,0.538461538461538,0.553846153846154,0.569230769230769,
0.584615384615384,0.6,0.615384615384615,0.63076923076923,0.646153846153846,
0.661538461538461,0.676923076923076,0.692307692307692,0.707692307692307,
0.723076923076922,0.738461538461538,0.753846153846153,0.769230769230768,
0.784615384615384,0.799999999999999,0.815384615384614,0.83076923076923,
0.846153846153845,0.86153846153846,0.876923076923076,0.892307692307691,
0.907692307692306,0.923076923076922,0.938461538461537,0.953846153846152,
0.969230769230768,0.984615384615383,0.994228156739701),.UNSPECIFIED.)
CURVE()
GEOMETRIC_REPRESENTATION_ITEM()
RATIONAL_B_SPLINE_CURVE((1.,1.,1.,1.,1.,1.,1.,1.,1.,1.,1.,1.,1.,1.,1.,1.,
1.,1.,1.,1.,1.,1.,1.,1.,1.,1.,1.,1.,1.,1.,1.,1.,1.,1.,1.,1.,1.,1.,1.,1.,
1.,1.,1.,1.,1.,1.,1.,1.,1.,1.,1.,1.,1.,1.,1.,1.,1.,1.,1.,1.,1.,1.,1.,1.,
1.,1.,1.,1.,1.,1.))
REPRESENTATION_ITEM('')
);
#357=(
BOUNDED_CURVE()
B_SPLINE_CURVE(5,(#51530,#51531,#51532,#51533,#51534,#51535,#51536,#51537,
#51538,#51539,#51540,#51541,#51542,#51543,#51544,#51545,#51546,#51547,#51548,
#51549,#51550,#51551,#51552,#51553,#51554,#51555,#51556,#51557,#51558,#51559,
#51560,#51561,#51562,#51563,#51564,#51565,#51566,#51567,#51568,#51569,#51570,
#51571,#51572,#51573,#51574,#51575,#51576,#51577,#51578,#51579,#51580,#51581,
#51582,#51583,#51584,#51585,#51586,#51587,#51588,#51589,#51590,#51591,#51592,
#51593,#51594,#51595,#51596,#51597,#51598,#51599),.UNSPECIFIED.,.F.,.F.)
B_SPLINE_CURVE_WITH_KNOTS((6,1,1,1,1,1,1,1,1,1,1,1,1,1,1,1,1,1,1,1,1,1,
1,1,1,1,1,1,1,1,1,1,1,1,1,1,1,1,1,1,1,1,1,1,1,1,1,1,1,1,1,1,1,1,1,1,1,1,
1,1,1,1,1,1,1,6),(0.00577184337450172,0.0153846153846154,0.0307692307692308,
0.0461538461538462,0.0615384615384615,0.0769230769230769,0.0923076923076923,
0.107692307692308,0.123076923076923,0.138461538461538,0.153846153846154,
0.169230769230769,0.184615384615385,0.2,0.215384615384615,0.230769230769231,
0.246153846153846,0.261538461538462,0.276923076923077,0.292307692307692,
0.307692307692308,0.323076923076923,0.338461538461538,0.353846153846154,
0.369230769230769,0.384615384615385,0.4,0.415384615384615,0.430769230769231,
0.446153846153846,0.461538461538462,0.476923076923077,0.492307692307692,
0.507692307692308,0.523076923076923,0.538461538461538,0.553846153846154,
0.569230769230769,0.584615384615384,0.6,0.615384615384615,0.63076923076923,
0.646153846153846,0.661538461538461,0.676923076923076,0.692307692307692,
0.707692307692307,0.723076923076922,0.738461538461538,0.753846153846153,
0.769230769230768,0.784615384615384,0.799999999999999,0.815384615384614,
0.83076923076923,0.846153846153845,0.86153846153846,0.876923076923076,0.892307692307691,
0.907692307692306,0.923076923076922,0.938461538461537,0.953846153846152,
0.969230769230768,0.984615384615383,1.),.UNSPECIFIED.)
CURVE()
GEOMETRIC_REPRESENTATION_ITEM()
RATIONAL_B_SPLINE_CURVE((1.,1.,1.,1.,1.,1.,1.,1.,1.,1.,1.,1.,1.,1.,1.,1.,
1.,1.,1.,1.,1.,1.,1.,1.,1.,1.,1.,1.,1.,1.,1.,1.,1.,1.,1.,1.,1.,1.,1.,1.,
1.,1.,1.,1.,1.,1.,1.,1.,1.,1.,1.,1.,1.,1.,1.,1.,1.,1.,1.,1.,1.,1.,1.,1.,
1.,1.,1.,1.,1.,1.))
REPRESENTATION_ITEM('')
);
#358=(
BOUNDED_CURVE()
B_SPLINE_CURVE(5,(#51603,#51604,#51605,#51606,#51607,#51608,#51609,#51610,
#51611,#51612,#51613,#51614,#51615,#51616,#51617,#51618,#51619,#51620,#51621,
#51622,#51623,#51624,#51625,#51626,#51627,#51628,#51629,#51630,#51631,#51632,
#51633,#51634,#51635,#51636,#51637,#51638,#51639,#51640,#51641,#51642,#51643,
#51644,#51645,#51646,#51647,#51648,#51649,#51650,#51651,#51652,#51653,#51654,
#51655,#51656,#51657,#51658,#51659,#51660,#51661,#51662,#51663,#51664,#51665,
#51666,#51667,#51668,#51669,#51670,#51671,#51672),.UNSPECIFIED.,.F.,.F.)
B_SPLINE_CURVE_WITH_KNOTS((6,1,1,1,1,1,1,1,1,1,1,1,1,1,1,1,1,1,1,1,1,1,
1,1,1,1,1,1,1,1,1,1,1,1,1,1,1,1,1,1,1,1,1,1,1,1,1,1,1,1,1,1,1,1,1,1,1,1,
1,1,1,1,1,1,1,6),(0.,0.0153846153846154,0.0307692307692308,0.0461538461538462,
0.0615384615384615,0.0769230769230769,0.0923076923076923,0.107692307692308,
0.123076923076923,0.138461538461538,0.153846153846154,0.169230769230769,
0.184615384615385,0.2,0.215384615384615,0.230769230769231,0.246153846153846,
0.261538461538462,0.276923076923077,0.292307692307692,0.307692307692308,
0.323076923076923,0.338461538461538,0.353846153846154,0.369230769230769,
0.384615384615385,0.4,0.415384615384615,0.430769230769231,0.446153846153846,
0.461538461538462,0.476923076923077,0.492307692307692,0.507692307692308,
0.523076923076923,0.538461538461538,0.553846153846154,0.569230769230769,
0.584615384615384,0.6,0.615384615384615,0.63076923076923,0.646153846153846,
0.661538461538461,0.676923076923076,0.692307692307692,0.707692307692307,
0.723076923076922,0.738461538461538,0.753846153846153,0.769230769230768,
0.784615384615384,0.799999999999999,0.815384615384614,0.83076923076923,
0.846153846153845,0.86153846153846,0.876923076923076,0.892307692307691,
0.907692307692306,0.923076923076922,0.938461538461537,0.953846153846152,
0.969230769230768,0.984615384615383,0.99422815673971),.UNSPECIFIED.)
CURVE()
GEOMETRIC_REPRESENTATION_ITEM()
RATIONAL_B_SPLINE_CURVE((1.,1.,1.,1.,1.,1.,1.,1.,1.,1.,1.,1.,1.,1.,1.,1.,
1.,1.,1.,1.,1.,1.,1.,1.,1.,1.,1.,1.,1.,1.,1.,1.,1.,1.,1.,1.,1.,1.,1.,1.,
1.,1.,1.,1.,1.,1.,1.,1.,1.,1.,1.,1.,1.,1.,1.,1.,1.,1.,1.,1.,1.,1.,1.,1.,
1.,1.,1.,1.,1.,1.))
REPRESENTATION_ITEM('')
);
#359=(
BOUNDED_CURVE()
B_SPLINE_CURVE(5,(#51676,#51677,#51678,#51679,#51680,#51681,#51682,#51683,
#51684,#51685,#51686,#51687,#51688,#51689,#51690,#51691,#51692,#51693,#51694,
#51695,#51696,#51697,#51698,#51699,#51700,#51701,#51702,#51703,#51704,#51705,
#51706,#51707,#51708,#51709,#51710,#51711,#51712,#51713,#51714,#51715,#51716,
#51717,#51718,#51719,#51720,#51721,#51722,#51723,#51724,#51725,#51726,#51727,
#51728,#51729,#51730,#51731,#51732,#51733,#51734,#51735,#51736,#51737,#51738,
#51739,#51740,#51741,#51742,#51743,#51744,#51745),.UNSPECIFIED.,.F.,.F.)
B_SPLINE_CURVE_WITH_KNOTS((6,1,1,1,1,1,1,1,1,1,1,1,1,1,1,1,1,1,1,1,1,1,
1,1,1,1,1,1,1,1,1,1,1,1,1,1,1,1,1,1,1,1,1,1,1,1,1,1,1,1,1,1,1,1,1,1,1,1,
1,1,1,1,1,1,1,6),(0.00577184337448657,0.0153846153846154,0.0307692307692308,
0.0461538461538462,0.0615384615384615,0.0769230769230769,0.0923076923076923,
0.107692307692308,0.123076923076923,0.138461538461538,0.153846153846154,
0.169230769230769,0.184615384615385,0.2,0.215384615384615,0.230769230769231,
0.246153846153846,0.261538461538462,0.276923076923077,0.292307692307692,
0.307692307692308,0.323076923076923,0.338461538461538,0.353846153846154,
0.369230769230769,0.384615384615385,0.4,0.415384615384615,0.430769230769231,
0.446153846153846,0.461538461538462,0.476923076923077,0.492307692307692,
0.507692307692308,0.523076923076923,0.538461538461538,0.553846153846154,
0.569230769230769,0.584615384615384,0.6,0.615384615384615,0.63076923076923,
0.646153846153846,0.661538461538461,0.676923076923076,0.692307692307692,
0.707692307692307,0.723076923076922,0.738461538461538,0.753846153846153,
0.769230769230768,0.784615384615384,0.799999999999999,0.815384615384614,
0.83076923076923,0.846153846153845,0.86153846153846,0.876923076923076,0.892307692307691,
0.907692307692306,0.923076923076922,0.938461538461537,0.953846153846152,
0.969230769230768,0.984615384615383,1.),.UNSPECIFIED.)
CURVE()
GEOMETRIC_REPRESENTATION_ITEM()
RATIONAL_B_SPLINE_CURVE((1.,1.,1.,1.,1.,1.,1.,1.,1.,1.,1.,1.,1.,1.,1.,1.,
1.,1.,1.,1.,1.,1.,1.,1.,1.,1.,1.,1.,1.,1.,1.,1.,1.,1.,1.,1.,1.,1.,1.,1.,
1.,1.,1.,1.,1.,1.,1.,1.,1.,1.,1.,1.,1.,1.,1.,1.,1.,1.,1.,1.,1.,1.,1.,1.,
1.,1.,1.,1.,1.,1.))
REPRESENTATION_ITEM('')
);
#360=(
BOUNDED_CURVE()
B_SPLINE_CURVE(5,(#51749,#51750,#51751,#51752,#51753,#51754,#51755,#51756,
#51757,#51758,#51759,#51760,#51761,#51762,#51763,#51764,#51765,#51766,#51767,
#51768,#51769,#51770,#51771,#51772,#51773,#51774,#51775,#51776,#51777,#51778,
#51779,#51780,#51781,#51782,#51783,#51784,#51785,#51786,#51787,#51788,#51789,
#51790,#51791,#51792,#51793,#51794,#51795,#51796,#51797,#51798,#51799,#51800,
#51801,#51802,#51803,#51804,#51805,#51806,#51807,#51808,#51809,#51810,#51811,
#51812,#51813,#51814,#51815,#51816,#51817,#51818),.UNSPECIFIED.,.F.,.F.)
B_SPLINE_CURVE_WITH_KNOTS((6,1,1,1,1,1,1,1,1,1,1,1,1,1,1,1,1,1,1,1,1,1,
1,1,1,1,1,1,1,1,1,1,1,1,1,1,1,1,1,1,1,1,1,1,1,1,1,1,1,1,1,1,1,1,1,1,1,1,
1,1,1,1,1,1,1,6),(0.,0.0153846153846154,0.0307692307692308,0.0461538461538462,
0.0615384615384615,0.0769230769230769,0.0923076923076923,0.107692307692308,
0.123076923076923,0.138461538461538,0.153846153846154,0.169230769230769,
0.184615384615385,0.2,0.215384615384615,0.230769230769231,0.246153846153846,
0.261538461538462,0.276923076923077,0.292307692307692,0.307692307692308,
0.323076923076923,0.338461538461538,0.353846153846154,0.369230769230769,
0.384615384615385,0.4,0.415384615384615,0.430769230769231,0.446153846153846,
0.461538461538462,0.476923076923077,0.492307692307692,0.507692307692308,
0.523076923076923,0.538461538461538,0.553846153846154,0.569230769230769,
0.584615384615384,0.6,0.615384615384615,0.63076923076923,0.646153846153846,
0.661538461538461,0.676923076923076,0.692307692307692,0.707692307692307,
0.723076923076922,0.738461538461538,0.753846153846153,0.769230769230768,
0.784615384615384,0.799999999999999,0.815384615384614,0.83076923076923,
0.846153846153845,0.86153846153846,0.876923076923076,0.892307692307691,
0.907692307692306,0.923076923076922,0.938461538461537,0.953846153846152,
0.969230769230768,0.984615384615383,0.994228156739709),.UNSPECIFIED.)
CURVE()
GEOMETRIC_REPRESENTATION_ITEM()
RATIONAL_B_SPLINE_CURVE((1.,1.,1.,1.,1.,1.,1.,1.,1.,1.,1.,1.,1.,1.,1.,1.,
1.,1.,1.,1.,1.,1.,1.,1.,1.,1.,1.,1.,1.,1.,1.,1.,1.,1.,1.,1.,1.,1.,1.,1.,
1.,1.,1.,1.,1.,1.,1.,1.,1.,1.,1.,1.,1.,1.,1.,1.,1.,1.,1.,1.,1.,1.,1.,1.,
1.,1.,1.,1.,1.,1.))
REPRESENTATION_ITEM('')
);
#361=(
BOUNDED_CURVE()
B_SPLINE_CURVE(5,(#51822,#51823,#51824,#51825,#51826,#51827,#51828,#51829,
#51830,#51831,#51832,#51833,#51834,#51835,#51836,#51837,#51838,#51839,#51840,
#51841,#51842,#51843,#51844,#51845,#51846,#51847,#51848,#51849,#51850,#51851,
#51852,#51853,#51854,#51855,#51856,#51857,#51858,#51859,#51860,#51861,#51862,
#51863,#51864,#51865,#51866,#51867,#51868,#51869,#51870,#51871,#51872,#51873,
#51874,#51875,#51876,#51877,#51878,#51879,#51880,#51881,#51882,#51883,#51884,
#51885,#51886,#51887,#51888,#51889,#51890,#51891),.UNSPECIFIED.,.F.,.F.)
B_SPLINE_CURVE_WITH_KNOTS((6,1,1,1,1,1,1,1,1,1,1,1,1,1,1,1,1,1,1,1,1,1,
1,1,1,1,1,1,1,1,1,1,1,1,1,1,1,1,1,1,1,1,1,1,1,1,1,1,1,1,1,1,1,1,1,1,1,1,
1,1,1,1,1,1,1,6),(0.00577184337451094,0.0153846153846154,0.0307692307692308,
0.0461538461538462,0.0615384615384615,0.0769230769230769,0.0923076923076923,
0.107692307692308,0.123076923076923,0.138461538461538,0.153846153846154,
0.169230769230769,0.184615384615385,0.2,0.215384615384615,0.230769230769231,
0.246153846153846,0.261538461538462,0.276923076923077,0.292307692307692,
0.307692307692308,0.323076923076923,0.338461538461538,0.353846153846154,
0.369230769230769,0.384615384615385,0.4,0.415384615384615,0.430769230769231,
0.446153846153846,0.461538461538462,0.476923076923077,0.492307692307692,
0.507692307692308,0.523076923076923,0.538461538461538,0.553846153846154,
0.569230769230769,0.584615384615384,0.6,0.615384615384615,0.63076923076923,
0.646153846153846,0.661538461538461,0.676923076923076,0.692307692307692,
0.707692307692307,0.723076923076922,0.738461538461538,0.753846153846153,
0.769230769230768,0.784615384615384,0.799999999999999,0.815384615384614,
0.83076923076923,0.846153846153845,0.86153846153846,0.876923076923076,0.892307692307691,
0.907692307692306,0.923076923076922,0.938461538461537,0.953846153846152,
0.969230769230768,0.984615384615383,1.),.UNSPECIFIED.)
CURVE()
GEOMETRIC_REPRESENTATION_ITEM()
RATIONAL_B_SPLINE_CURVE((1.,1.,1.,1.,1.,1.,1.,1.,1.,1.,1.,1.,1.,1.,1.,1.,
1.,1.,1.,1.,1.,1.,1.,1.,1.,1.,1.,1.,1.,1.,1.,1.,1.,1.,1.,1.,1.,1.,1.,1.,
1.,1.,1.,1.,1.,1.,1.,1.,1.,1.,1.,1.,1.,1.,1.,1.,1.,1.,1.,1.,1.,1.,1.,1.,
1.,1.,1.,1.,1.,1.))
REPRESENTATION_ITEM('')
);
#362=(
BOUNDED_CURVE()
B_SPLINE_CURVE(5,(#51895,#51896,#51897,#51898,#51899,#51900,#51901,#51902,
#51903,#51904,#51905,#51906,#51907,#51908,#51909,#51910,#51911,#51912,#51913,
#51914,#51915,#51916,#51917,#51918,#51919,#51920,#51921,#51922,#51923,#51924,
#51925,#51926,#51927,#51928,#51929,#51930,#51931,#51932,#51933,#51934,#51935,
#51936,#51937,#51938,#51939,#51940,#51941,#51942,#51943,#51944,#51945,#51946,
#51947,#51948,#51949,#51950,#51951,#51952,#51953,#51954,#51955,#51956,#51957,
#51958,#51959,#51960,#51961,#51962,#51963,#51964),.UNSPECIFIED.,.F.,.F.)
B_SPLINE_CURVE_WITH_KNOTS((6,1,1,1,1,1,1,1,1,1,1,1,1,1,1,1,1,1,1,1,1,1,
1,1,1,1,1,1,1,1,1,1,1,1,1,1,1,1,1,1,1,1,1,1,1,1,1,1,1,1,1,1,1,1,1,1,1,1,
1,1,1,1,1,1,1,6),(0.,0.0153846153846154,0.0307692307692308,0.0461538461538462,
0.0615384615384615,0.0769230769230769,0.0923076923076923,0.107692307692308,
0.123076923076923,0.138461538461538,0.153846153846154,0.169230769230769,
0.184615384615385,0.2,0.215384615384615,0.230769230769231,0.246153846153846,
0.261538461538462,0.276923076923077,0.292307692307692,0.307692307692308,
0.323076923076923,0.338461538461538,0.353846153846154,0.369230769230769,
0.384615384615385,0.4,0.415384615384615,0.430769230769231,0.446153846153846,
0.461538461538462,0.476923076923077,0.492307692307692,0.507692307692308,
0.523076923076923,0.538461538461538,0.553846153846154,0.569230769230769,
0.584615384615384,0.6,0.615384615384615,0.63076923076923,0.646153846153846,
0.661538461538461,0.676923076923076,0.692307692307692,0.707692307692307,
0.723076923076922,0.738461538461538,0.753846153846153,0.769230769230768,
0.784615384615384,0.799999999999999,0.815384615384614,0.83076923076923,
0.846153846153845,0.86153846153846,0.876923076923076,0.892307692307691,
0.907692307692306,0.923076923076922,0.938461538461537,0.953846153846152,
0.969230769230768,0.984615384615383,0.994228156739701),.UNSPECIFIED.)
CURVE()
GEOMETRIC_REPRESENTATION_ITEM()
RATIONAL_B_SPLINE_CURVE((1.,1.,1.,1.,1.,1.,1.,1.,1.,1.,1.,1.,1.,1.,1.,1.,
1.,1.,1.,1.,1.,1.,1.,1.,1.,1.,1.,1.,1.,1.,1.,1.,1.,1.,1.,1.,1.,1.,1.,1.,
1.,1.,1.,1.,1.,1.,1.,1.,1.,1.,1.,1.,1.,1.,1.,1.,1.,1.,1.,1.,1.,1.,1.,1.,
1.,1.,1.,1.,1.,1.))
REPRESENTATION_ITEM('')
);
#363=(
BOUNDED_CURVE()
B_SPLINE_CURVE(5,(#51968,#51969,#51970,#51971,#51972,#51973,#51974,#51975,
#51976,#51977,#51978,#51979,#51980,#51981,#51982,#51983,#51984,#51985,#51986,
#51987,#51988,#51989,#51990,#51991,#51992,#51993,#51994,#51995,#51996,#51997,
#51998,#51999,#52000,#52001,#52002,#52003,#52004,#52005,#52006,#52007,#52008,
#52009,#52010,#52011,#52012,#52013,#52014,#52015,#52016,#52017,#52018,#52019,
#52020,#52021,#52022,#52023,#52024,#52025,#52026,#52027,#52028,#52029,#52030,
#52031,#52032,#52033,#52034,#52035,#52036,#52037),.UNSPECIFIED.,.F.,.F.)
B_SPLINE_CURVE_WITH_KNOTS((6,1,1,1,1,1,1,1,1,1,1,1,1,1,1,1,1,1,1,1,1,1,
1,1,1,1,1,1,1,1,1,1,1,1,1,1,1,1,1,1,1,1,1,1,1,1,1,1,1,1,1,1,1,1,1,1,1,1,
1,1,1,1,1,1,1,6),(0.0057718433745102,0.0153846153846154,0.0307692307692308,
0.0461538461538462,0.0615384615384615,0.0769230769230769,0.0923076923076923,
0.107692307692308,0.123076923076923,0.138461538461538,0.153846153846154,
0.169230769230769,0.184615384615385,0.2,0.215384615384615,0.230769230769231,
0.246153846153846,0.261538461538462,0.276923076923077,0.292307692307692,
0.307692307692308,0.323076923076923,0.338461538461538,0.353846153846154,
0.369230769230769,0.384615384615385,0.4,0.415384615384615,0.430769230769231,
0.446153846153846,0.461538461538462,0.476923076923077,0.492307692307692,
0.507692307692308,0.523076923076923,0.538461538461538,0.553846153846154,
0.569230769230769,0.584615384615384,0.6,0.615384615384615,0.63076923076923,
0.646153846153846,0.661538461538461,0.676923076923076,0.692307692307692,
0.707692307692307,0.723076923076922,0.738461538461538,0.753846153846153,
0.769230769230768,0.784615384615384,0.799999999999999,0.815384615384614,
0.83076923076923,0.846153846153845,0.86153846153846,0.876923076923076,0.892307692307691,
0.907692307692306,0.923076923076922,0.938461538461537,0.953846153846152,
0.969230769230768,0.984615384615383,1.),.UNSPECIFIED.)
CURVE()
GEOMETRIC_REPRESENTATION_ITEM()
RATIONAL_B_SPLINE_CURVE((1.,1.,1.,1.,1.,1.,1.,1.,1.,1.,1.,1.,1.,1.,1.,1.,
1.,1.,1.,1.,1.,1.,1.,1.,1.,1.,1.,1.,1.,1.,1.,1.,1.,1.,1.,1.,1.,1.,1.,1.,
1.,1.,1.,1.,1.,1.,1.,1.,1.,1.,1.,1.,1.,1.,1.,1.,1.,1.,1.,1.,1.,1.,1.,1.,
1.,1.,1.,1.,1.,1.))
REPRESENTATION_ITEM('')
);
#364=(
BOUNDED_CURVE()
B_SPLINE_CURVE(5,(#52041,#52042,#52043,#52044,#52045,#52046,#52047,#52048,
#52049,#52050,#52051,#52052,#52053,#52054,#52055,#52056,#52057,#52058,#52059,
#52060,#52061,#52062,#52063,#52064,#52065,#52066,#52067,#52068,#52069,#52070,
#52071,#52072,#52073,#52074,#52075,#52076,#52077,#52078,#52079,#52080,#52081,
#52082,#52083,#52084,#52085,#52086,#52087,#52088,#52089,#52090,#52091,#52092,
#52093,#52094,#52095,#52096,#52097,#52098,#52099,#52100,#52101,#52102,#52103,
#52104,#52105,#52106,#52107,#52108,#52109,#52110),.UNSPECIFIED.,.F.,.F.)
B_SPLINE_CURVE_WITH_KNOTS((6,1,1,1,1,1,1,1,1,1,1,1,1,1,1,1,1,1,1,1,1,1,
1,1,1,1,1,1,1,1,1,1,1,1,1,1,1,1,1,1,1,1,1,1,1,1,1,1,1,1,1,1,1,1,1,1,1,1,
1,1,1,1,1,1,1,6),(0.,0.0153846153846154,0.0307692307692308,0.0461538461538462,
0.0615384615384615,0.0769230769230769,0.0923076923076923,0.107692307692308,
0.123076923076923,0.138461538461538,0.153846153846154,0.169230769230769,
0.184615384615385,0.2,0.215384615384615,0.230769230769231,0.246153846153846,
0.261538461538462,0.276923076923077,0.292307692307692,0.307692307692308,
0.323076923076923,0.338461538461538,0.353846153846154,0.369230769230769,
0.384615384615385,0.4,0.415384615384615,0.430769230769231,0.446153846153846,
0.461538461538462,0.476923076923077,0.492307692307692,0.507692307692308,
0.523076923076923,0.538461538461538,0.553846153846154,0.569230769230769,
0.584615384615384,0.6,0.615384615384615,0.63076923076923,0.646153846153846,
0.661538461538461,0.676923076923076,0.692307692307692,0.707692307692307,
0.723076923076922,0.738461538461538,0.753846153846153,0.769230769230768,
0.784615384615384,0.799999999999999,0.815384615384614,0.83076923076923,
0.846153846153845,0.86153846153846,0.876923076923076,0.892307692307691,
0.907692307692306,0.923076923076922,0.938461538461537,0.953846153846152,
0.969230769230768,0.984615384615383,0.994228156739694),.UNSPECIFIED.)
CURVE()
GEOMETRIC_REPRESENTATION_ITEM()
RATIONAL_B_SPLINE_CURVE((1.,1.,1.,1.,1.,1.,1.,1.,1.,1.,1.,1.,1.,1.,1.,1.,
1.,1.,1.,1.,1.,1.,1.,1.,1.,1.,1.,1.,1.,1.,1.,1.,1.,1.,1.,1.,1.,1.,1.,1.,
1.,1.,1.,1.,1.,1.,1.,1.,1.,1.,1.,1.,1.,1.,1.,1.,1.,1.,1.,1.,1.,1.,1.,1.,
1.,1.,1.,1.,1.,1.))
REPRESENTATION_ITEM('')
);
#365=(
BOUNDED_CURVE()
B_SPLINE_CURVE(5,(#52114,#52115,#52116,#52117,#52118,#52119,#52120,#52121,
#52122,#52123,#52124,#52125,#52126,#52127,#52128,#52129,#52130,#52131,#52132,
#52133,#52134,#52135,#52136,#52137,#52138,#52139,#52140,#52141,#52142,#52143,
#52144,#52145,#52146,#52147,#52148,#52149,#52150,#52151,#52152,#52153,#52154,
#52155,#52156,#52157,#52158,#52159,#52160,#52161,#52162,#52163,#52164,#52165,
#52166,#52167,#52168,#52169,#52170,#52171,#52172,#52173,#52174,#52175,#52176,
#52177,#52178,#52179,#52180,#52181,#52182,#52183),.UNSPECIFIED.,.F.,.F.)
B_SPLINE_CURVE_WITH_KNOTS((6,1,1,1,1,1,1,1,1,1,1,1,1,1,1,1,1,1,1,1,1,1,
1,1,1,1,1,1,1,1,1,1,1,1,1,1,1,1,1,1,1,1,1,1,1,1,1,1,1,1,1,1,1,1,1,1,1,1,
1,1,1,1,1,1,1,6),(0.00577184337452044,0.0153846153846154,0.0307692307692308,
0.0461538461538462,0.0615384615384615,0.0769230769230769,0.0923076923076923,
0.107692307692308,0.123076923076923,0.138461538461538,0.153846153846154,
0.169230769230769,0.184615384615385,0.2,0.215384615384615,0.230769230769231,
0.246153846153846,0.261538461538462,0.276923076923077,0.292307692307692,
0.307692307692308,0.323076923076923,0.338461538461538,0.353846153846154,
0.369230769230769,0.384615384615385,0.4,0.415384615384615,0.430769230769231,
0.446153846153846,0.461538461538462,0.476923076923077,0.492307692307692,
0.507692307692308,0.523076923076923,0.538461538461538,0.553846153846154,
0.569230769230769,0.584615384615384,0.6,0.615384615384615,0.63076923076923,
0.646153846153846,0.661538461538461,0.676923076923076,0.692307692307692,
0.707692307692307,0.723076923076922,0.738461538461538,0.753846153846153,
0.769230769230768,0.784615384615384,0.799999999999999,0.815384615384614,
0.83076923076923,0.846153846153845,0.86153846153846,0.876923076923076,0.892307692307691,
0.907692307692306,0.923076923076922,0.938461538461537,0.953846153846152,
0.969230769230768,0.984615384615383,1.),.UNSPECIFIED.)
CURVE()
GEOMETRIC_REPRESENTATION_ITEM()
RATIONAL_B_SPLINE_CURVE((1.,1.,1.,1.,1.,1.,1.,1.,1.,1.,1.,1.,1.,1.,1.,1.,
1.,1.,1.,1.,1.,1.,1.,1.,1.,1.,1.,1.,1.,1.,1.,1.,1.,1.,1.,1.,1.,1.,1.,1.,
1.,1.,1.,1.,1.,1.,1.,1.,1.,1.,1.,1.,1.,1.,1.,1.,1.,1.,1.,1.,1.,1.,1.,1.,
1.,1.,1.,1.,1.,1.))
REPRESENTATION_ITEM('')
);
#366=(
BOUNDED_CURVE()
B_SPLINE_CURVE(5,(#52187,#52188,#52189,#52190,#52191,#52192,#52193,#52194,
#52195,#52196,#52197,#52198,#52199,#52200,#52201,#52202,#52203,#52204,#52205,
#52206,#52207,#52208,#52209,#52210,#52211,#52212,#52213,#52214,#52215,#52216,
#52217,#52218,#52219,#52220,#52221,#52222,#52223,#52224,#52225,#52226,#52227,
#52228,#52229,#52230,#52231,#52232,#52233,#52234,#52235,#52236,#52237,#52238,
#52239,#52240,#52241,#52242,#52243,#52244,#52245,#52246,#52247,#52248,#52249,
#52250,#52251,#52252,#52253,#52254,#52255,#52256),.UNSPECIFIED.,.F.,.F.)
B_SPLINE_CURVE_WITH_KNOTS((6,1,1,1,1,1,1,1,1,1,1,1,1,1,1,1,1,1,1,1,1,1,
1,1,1,1,1,1,1,1,1,1,1,1,1,1,1,1,1,1,1,1,1,1,1,1,1,1,1,1,1,1,1,1,1,1,1,1,
1,1,1,1,1,1,1,6),(0.,0.0153846153846154,0.0307692307692308,0.0461538461538462,
0.0615384615384615,0.0769230769230769,0.0923076923076923,0.107692307692308,
0.123076923076923,0.138461538461538,0.153846153846154,0.169230769230769,
0.184615384615385,0.2,0.215384615384615,0.230769230769231,0.246153846153846,
0.261538461538462,0.276923076923077,0.292307692307692,0.307692307692308,
0.323076923076923,0.338461538461538,0.353846153846154,0.369230769230769,
0.384615384615385,0.4,0.415384615384615,0.430769230769231,0.446153846153846,
0.461538461538462,0.476923076923077,0.492307692307692,0.507692307692308,
0.523076923076923,0.538461538461538,0.553846153846154,0.569230769230769,
0.584615384615384,0.6,0.615384615384615,0.63076923076923,0.646153846153846,
0.661538461538461,0.676923076923076,0.692307692307692,0.707692307692307,
0.723076923076922,0.738461538461538,0.753846153846153,0.769230769230768,
0.784615384615384,0.799999999999999,0.815384615384614,0.83076923076923,
0.846153846153845,0.86153846153846,0.876923076923076,0.892307692307691,
0.907692307692306,0.923076923076922,0.938461538461537,0.953846153846152,
0.969230769230768,0.984615384615383,0.994228156739698),.UNSPECIFIED.)
CURVE()
GEOMETRIC_REPRESENTATION_ITEM()
RATIONAL_B_SPLINE_CURVE((1.,1.,1.,1.,1.,1.,1.,1.,1.,1.,1.,1.,1.,1.,1.,1.,
1.,1.,1.,1.,1.,1.,1.,1.,1.,1.,1.,1.,1.,1.,1.,1.,1.,1.,1.,1.,1.,1.,1.,1.,
1.,1.,1.,1.,1.,1.,1.,1.,1.,1.,1.,1.,1.,1.,1.,1.,1.,1.,1.,1.,1.,1.,1.,1.,
1.,1.,1.,1.,1.,1.))
REPRESENTATION_ITEM('')
);
#367=(
BOUNDED_CURVE()
B_SPLINE_CURVE(5,(#52260,#52261,#52262,#52263,#52264,#52265,#52266,#52267,
#52268,#52269,#52270,#52271,#52272,#52273,#52274,#52275,#52276,#52277,#52278,
#52279,#52280,#52281,#52282,#52283,#52284,#52285,#52286,#52287,#52288,#52289,
#52290,#52291,#52292,#52293,#52294,#52295,#52296,#52297,#52298,#52299,#52300,
#52301,#52302,#52303,#52304,#52305,#52306,#52307,#52308,#52309,#52310,#52311,
#52312,#52313,#52314,#52315,#52316,#52317,#52318,#52319,#52320,#52321,#52322,
#52323,#52324,#52325,#52326,#52327,#52328,#52329),.UNSPECIFIED.,.F.,.F.)
B_SPLINE_CURVE_WITH_KNOTS((6,1,1,1,1,1,1,1,1,1,1,1,1,1,1,1,1,1,1,1,1,1,
1,1,1,1,1,1,1,1,1,1,1,1,1,1,1,1,1,1,1,1,1,1,1,1,1,1,1,1,1,1,1,1,1,1,1,1,
1,1,1,1,1,1,1,6),(0.00577184337451607,0.0153846153846154,0.0307692307692308,
0.0461538461538462,0.0615384615384615,0.0769230769230769,0.0923076923076923,
0.107692307692308,0.123076923076923,0.138461538461538,0.153846153846154,
0.169230769230769,0.184615384615385,0.2,0.215384615384615,0.230769230769231,
0.246153846153846,0.261538461538462,0.276923076923077,0.292307692307692,
0.307692307692308,0.323076923076923,0.338461538461538,0.353846153846154,
0.369230769230769,0.384615384615385,0.4,0.415384615384615,0.430769230769231,
0.446153846153846,0.461538461538462,0.476923076923077,0.492307692307692,
0.507692307692308,0.523076923076923,0.538461538461538,0.553846153846154,
0.569230769230769,0.584615384615384,0.6,0.615384615384615,0.63076923076923,
0.646153846153846,0.661538461538461,0.676923076923076,0.692307692307692,
0.707692307692307,0.723076923076922,0.738461538461538,0.753846153846153,
0.769230769230768,0.784615384615384,0.799999999999999,0.815384615384614,
0.83076923076923,0.846153846153845,0.86153846153846,0.876923076923076,0.892307692307691,
0.907692307692306,0.923076923076922,0.938461538461537,0.953846153846152,
0.969230769230768,0.984615384615383,1.),.UNSPECIFIED.)
CURVE()
GEOMETRIC_REPRESENTATION_ITEM()
RATIONAL_B_SPLINE_CURVE((1.,1.,1.,1.,1.,1.,1.,1.,1.,1.,1.,1.,1.,1.,1.,1.,
1.,1.,1.,1.,1.,1.,1.,1.,1.,1.,1.,1.,1.,1.,1.,1.,1.,1.,1.,1.,1.,1.,1.,1.,
1.,1.,1.,1.,1.,1.,1.,1.,1.,1.,1.,1.,1.,1.,1.,1.,1.,1.,1.,1.,1.,1.,1.,1.,
1.,1.,1.,1.,1.,1.))
REPRESENTATION_ITEM('')
);
#368=(
BOUNDED_CURVE()
B_SPLINE_CURVE(5,(#52333,#52334,#52335,#52336,#52337,#52338,#52339,#52340,
#52341,#52342,#52343,#52344,#52345,#52346,#52347,#52348,#52349,#52350,#52351,
#52352,#52353,#52354,#52355,#52356,#52357,#52358,#52359,#52360,#52361,#52362,
#52363,#52364,#52365,#52366,#52367,#52368,#52369,#52370,#52371,#52372,#52373,
#52374,#52375,#52376,#52377,#52378,#52379,#52380,#52381,#52382,#52383,#52384,
#52385,#52386,#52387,#52388,#52389,#52390,#52391,#52392,#52393,#52394,#52395,
#52396,#52397,#52398,#52399,#52400,#52401,#52402),.UNSPECIFIED.,.F.,.F.)
B_SPLINE_CURVE_WITH_KNOTS((6,1,1,1,1,1,1,1,1,1,1,1,1,1,1,1,1,1,1,1,1,1,
1,1,1,1,1,1,1,1,1,1,1,1,1,1,1,1,1,1,1,1,1,1,1,1,1,1,1,1,1,1,1,1,1,1,1,1,
1,1,1,1,1,1,1,6),(0.,0.0153846153846154,0.0307692307692308,0.0461538461538462,
0.0615384615384615,0.0769230769230769,0.0923076923076923,0.107692307692308,
0.123076923076923,0.138461538461538,0.153846153846154,0.169230769230769,
0.184615384615385,0.2,0.215384615384615,0.230769230769231,0.246153846153846,
0.261538461538462,0.276923076923077,0.292307692307692,0.307692307692308,
0.323076923076923,0.338461538461538,0.353846153846154,0.369230769230769,
0.384615384615385,0.4,0.415384615384615,0.430769230769231,0.446153846153846,
0.461538461538462,0.476923076923077,0.492307692307692,0.507692307692308,
0.523076923076923,0.538461538461538,0.553846153846154,0.569230769230769,
0.584615384615384,0.6,0.615384615384615,0.63076923076923,0.646153846153846,
0.661538461538461,0.676923076923076,0.692307692307692,0.707692307692307,
0.723076923076922,0.738461538461538,0.753846153846153,0.769230769230768,
0.784615384615384,0.799999999999999,0.815384615384614,0.83076923076923,
0.846153846153845,0.86153846153846,0.876923076923076,0.892307692307691,
0.907692307692306,0.923076923076922,0.938461538461537,0.953846153846152,
0.969230769230768,0.984615384615383,0.994228156739704),.UNSPECIFIED.)
CURVE()
GEOMETRIC_REPRESENTATION_ITEM()
RATIONAL_B_SPLINE_CURVE((1.,1.,1.,1.,1.,1.,1.,1.,1.,1.,1.,1.,1.,1.,1.,1.,
1.,1.,1.,1.,1.,1.,1.,1.,1.,1.,1.,1.,1.,1.,1.,1.,1.,1.,1.,1.,1.,1.,1.,1.,
1.,1.,1.,1.,1.,1.,1.,1.,1.,1.,1.,1.,1.,1.,1.,1.,1.,1.,1.,1.,1.,1.,1.,1.,
1.,1.,1.,1.,1.,1.))
REPRESENTATION_ITEM('')
);
#369=(
BOUNDED_CURVE()
B_SPLINE_CURVE(5,(#52406,#52407,#52408,#52409,#52410,#52411,#52412,#52413,
#52414,#52415,#52416,#52417,#52418,#52419,#52420,#52421,#52422,#52423,#52424,
#52425,#52426,#52427,#52428,#52429,#52430,#52431,#52432,#52433,#52434,#52435,
#52436,#52437,#52438,#52439,#52440,#52441,#52442,#52443,#52444,#52445,#52446,
#52447,#52448,#52449,#52450,#52451,#52452,#52453,#52454,#52455,#52456,#52457,
#52458,#52459,#52460,#52461,#52462,#52463,#52464,#52465,#52466,#52467,#52468,
#52469,#52470,#52471,#52472,#52473,#52474,#52475),.UNSPECIFIED.,.F.,.F.)
B_SPLINE_CURVE_WITH_KNOTS((6,1,1,1,1,1,1,1,1,1,1,1,1,1,1,1,1,1,1,1,1,1,
1,1,1,1,1,1,1,1,1,1,1,1,1,1,1,1,1,1,1,1,1,1,1,1,1,1,1,1,1,1,1,1,1,1,1,1,
1,1,1,1,1,1,1,6),(0.00577184337449682,0.0153846153846154,0.0307692307692308,
0.0461538461538462,0.0615384615384615,0.0769230769230769,0.0923076923076923,
0.107692307692308,0.123076923076923,0.138461538461538,0.153846153846154,
0.169230769230769,0.184615384615385,0.2,0.215384615384615,0.230769230769231,
0.246153846153846,0.261538461538462,0.276923076923077,0.292307692307692,
0.307692307692308,0.323076923076923,0.338461538461538,0.353846153846154,
0.369230769230769,0.384615384615385,0.4,0.415384615384615,0.430769230769231,
0.446153846153846,0.461538461538462,0.476923076923077,0.492307692307692,
0.507692307692308,0.523076923076923,0.538461538461538,0.553846153846154,
0.569230769230769,0.584615384615384,0.6,0.615384615384615,0.63076923076923,
0.646153846153846,0.661538461538461,0.676923076923076,0.692307692307692,
0.707692307692307,0.723076923076922,0.738461538461538,0.753846153846153,
0.769230769230768,0.784615384615384,0.799999999999999,0.815384615384614,
0.83076923076923,0.846153846153845,0.86153846153846,0.876923076923076,0.892307692307691,
0.907692307692306,0.923076923076922,0.938461538461537,0.953846153846152,
0.969230769230768,0.984615384615383,1.),.UNSPECIFIED.)
CURVE()
GEOMETRIC_REPRESENTATION_ITEM()
RATIONAL_B_SPLINE_CURVE((1.,1.,1.,1.,1.,1.,1.,1.,1.,1.,1.,1.,1.,1.,1.,1.,
1.,1.,1.,1.,1.,1.,1.,1.,1.,1.,1.,1.,1.,1.,1.,1.,1.,1.,1.,1.,1.,1.,1.,1.,
1.,1.,1.,1.,1.,1.,1.,1.,1.,1.,1.,1.,1.,1.,1.,1.,1.,1.,1.,1.,1.,1.,1.,1.,
1.,1.,1.,1.,1.,1.))
REPRESENTATION_ITEM('')
);
#370=(
BOUNDED_CURVE()
B_SPLINE_CURVE(5,(#52479,#52480,#52481,#52482,#52483,#52484,#52485,#52486,
#52487,#52488,#52489,#52490,#52491,#52492,#52493,#52494,#52495,#52496,#52497,
#52498,#52499,#52500,#52501,#52502,#52503,#52504,#52505,#52506,#52507,#52508,
#52509,#52510,#52511,#52512,#52513,#52514,#52515,#52516,#52517,#52518,#52519,
#52520,#52521,#52522,#52523,#52524,#52525,#52526,#52527,#52528,#52529,#52530,
#52531,#52532,#52533,#52534,#52535,#52536,#52537,#52538,#52539,#52540,#52541,
#52542,#52543,#52544,#52545,#52546,#52547,#52548),.UNSPECIFIED.,.F.,.F.)
B_SPLINE_CURVE_WITH_KNOTS((6,1,1,1,1,1,1,1,1,1,1,1,1,1,1,1,1,1,1,1,1,1,
1,1,1,1,1,1,1,1,1,1,1,1,1,1,1,1,1,1,1,1,1,1,1,1,1,1,1,1,1,1,1,1,1,1,1,1,
1,1,1,1,1,1,1,6),(0.,0.0153846153846154,0.0307692307692308,0.0461538461538462,
0.0615384615384615,0.0769230769230769,0.0923076923076923,0.107692307692308,
0.123076923076923,0.138461538461538,0.153846153846154,0.169230769230769,
0.184615384615385,0.2,0.215384615384615,0.230769230769231,0.246153846153846,
0.261538461538462,0.276923076923077,0.292307692307692,0.307692307692308,
0.323076923076923,0.338461538461538,0.353846153846154,0.369230769230769,
0.384615384615385,0.4,0.415384615384615,0.430769230769231,0.446153846153846,
0.461538461538462,0.476923076923077,0.492307692307692,0.507692307692308,
0.523076923076923,0.538461538461538,0.553846153846154,0.569230769230769,
0.584615384615384,0.6,0.615384615384615,0.63076923076923,0.646153846153846,
0.661538461538461,0.676923076923076,0.692307692307692,0.707692307692307,
0.723076923076922,0.738461538461538,0.753846153846153,0.769230769230768,
0.784615384615384,0.799999999999999,0.815384615384614,0.83076923076923,
0.846153846153845,0.86153846153846,0.876923076923076,0.892307692307691,
0.907692307692306,0.923076923076922,0.938461538461537,0.953846153846152,
0.969230769230768,0.984615384615383,0.994228156739711),.UNSPECIFIED.)
CURVE()
GEOMETRIC_REPRESENTATION_ITEM()
RATIONAL_B_SPLINE_CURVE((1.,1.,1.,1.,1.,1.,1.,1.,1.,1.,1.,1.,1.,1.,1.,1.,
1.,1.,1.,1.,1.,1.,1.,1.,1.,1.,1.,1.,1.,1.,1.,1.,1.,1.,1.,1.,1.,1.,1.,1.,
1.,1.,1.,1.,1.,1.,1.,1.,1.,1.,1.,1.,1.,1.,1.,1.,1.,1.,1.,1.,1.,1.,1.,1.,
1.,1.,1.,1.,1.,1.))
REPRESENTATION_ITEM('')
);
#371=(
BOUNDED_CURVE()
B_SPLINE_CURVE(5,(#52552,#52553,#52554,#52555,#52556,#52557,#52558,#52559,
#52560,#52561,#52562,#52563,#52564,#52565,#52566,#52567,#52568,#52569,#52570,
#52571,#52572,#52573,#52574,#52575,#52576,#52577,#52578,#52579,#52580,#52581,
#52582,#52583,#52584,#52585,#52586,#52587,#52588,#52589,#52590,#52591,#52592,
#52593,#52594,#52595,#52596,#52597,#52598,#52599,#52600,#52601,#52602,#52603,
#52604,#52605,#52606,#52607,#52608,#52609,#52610,#52611,#52612,#52613,#52614,
#52615,#52616,#52617,#52618,#52619,#52620,#52621),.UNSPECIFIED.,.F.,.F.)
B_SPLINE_CURVE_WITH_KNOTS((6,1,1,1,1,1,1,1,1,1,1,1,1,1,1,1,1,1,1,1,1,1,
1,1,1,1,1,1,1,1,1,1,1,1,1,1,1,1,1,1,1,1,1,1,1,1,1,1,1,1,1,1,1,1,1,1,1,1,
1,1,1,1,1,1,1,6),(0.00577184337450313,0.0153846153846154,0.0307692307692308,
0.0461538461538462,0.0615384615384615,0.0769230769230769,0.0923076923076923,
0.107692307692308,0.123076923076923,0.138461538461538,0.153846153846154,
0.169230769230769,0.184615384615385,0.2,0.215384615384615,0.230769230769231,
0.246153846153846,0.261538461538462,0.276923076923077,0.292307692307692,
0.307692307692308,0.323076923076923,0.338461538461538,0.353846153846154,
0.369230769230769,0.384615384615385,0.4,0.415384615384615,0.430769230769231,
0.446153846153846,0.461538461538462,0.476923076923077,0.492307692307692,
0.507692307692308,0.523076923076923,0.538461538461538,0.553846153846154,
0.569230769230769,0.584615384615384,0.6,0.615384615384615,0.63076923076923,
0.646153846153846,0.661538461538461,0.676923076923076,0.692307692307692,
0.707692307692307,0.723076923076922,0.738461538461538,0.753846153846153,
0.769230769230768,0.784615384615384,0.799999999999999,0.815384615384614,
0.83076923076923,0.846153846153845,0.86153846153846,0.876923076923076,0.892307692307691,
0.907692307692306,0.923076923076922,0.938461538461537,0.953846153846152,
0.969230769230768,0.984615384615383,1.),.UNSPECIFIED.)
CURVE()
GEOMETRIC_REPRESENTATION_ITEM()
RATIONAL_B_SPLINE_CURVE((1.,1.,1.,1.,1.,1.,1.,1.,1.,1.,1.,1.,1.,1.,1.,1.,
1.,1.,1.,1.,1.,1.,1.,1.,1.,1.,1.,1.,1.,1.,1.,1.,1.,1.,1.,1.,1.,1.,1.,1.,
1.,1.,1.,1.,1.,1.,1.,1.,1.,1.,1.,1.,1.,1.,1.,1.,1.,1.,1.,1.,1.,1.,1.,1.,
1.,1.,1.,1.,1.,1.))
REPRESENTATION_ITEM('')
);
#372=(
BOUNDED_CURVE()
B_SPLINE_CURVE(5,(#52625,#52626,#52627,#52628,#52629,#52630,#52631,#52632,
#52633,#52634,#52635,#52636,#52637,#52638,#52639,#52640,#52641,#52642,#52643,
#52644,#52645,#52646,#52647,#52648,#52649,#52650,#52651,#52652,#52653,#52654,
#52655,#52656,#52657,#52658,#52659,#52660,#52661,#52662,#52663,#52664,#52665,
#52666,#52667,#52668,#52669,#52670,#52671,#52672,#52673,#52674,#52675,#52676,
#52677,#52678,#52679,#52680,#52681,#52682,#52683,#52684,#52685,#52686,#52687,
#52688,#52689,#52690,#52691,#52692,#52693,#52694),.UNSPECIFIED.,.F.,.F.)
B_SPLINE_CURVE_WITH_KNOTS((6,1,1,1,1,1,1,1,1,1,1,1,1,1,1,1,1,1,1,1,1,1,
1,1,1,1,1,1,1,1,1,1,1,1,1,1,1,1,1,1,1,1,1,1,1,1,1,1,1,1,1,1,1,1,1,1,1,1,
1,1,1,1,1,1,1,6),(0.,0.0153846153846154,0.0307692307692308,0.0461538461538462,
0.0615384615384615,0.0769230769230769,0.0923076923076923,0.107692307692308,
0.123076923076923,0.138461538461538,0.153846153846154,0.169230769230769,
0.184615384615385,0.2,0.215384615384615,0.230769230769231,0.246153846153846,
0.261538461538462,0.276923076923077,0.292307692307692,0.307692307692308,
0.323076923076923,0.338461538461538,0.353846153846154,0.369230769230769,
0.384615384615385,0.4,0.415384615384615,0.430769230769231,0.446153846153846,
0.461538461538462,0.476923076923077,0.492307692307692,0.507692307692308,
0.523076923076923,0.538461538461538,0.553846153846154,0.569230769230769,
0.584615384615384,0.6,0.615384615384615,0.63076923076923,0.646153846153846,
0.661538461538461,0.676923076923076,0.692307692307692,0.707692307692307,
0.723076923076922,0.738461538461538,0.753846153846153,0.769230769230768,
0.784615384615384,0.799999999999999,0.815384615384614,0.83076923076923,
0.846153846153845,0.86153846153846,0.876923076923076,0.892307692307691,
0.907692307692306,0.923076923076922,0.938461538461537,0.953846153846152,
0.969230769230768,0.984615384615383,0.9942281567397),.UNSPECIFIED.)
CURVE()
GEOMETRIC_REPRESENTATION_ITEM()
RATIONAL_B_SPLINE_CURVE((1.,1.,1.,1.,1.,1.,1.,1.,1.,1.,1.,1.,1.,1.,1.,1.,
1.,1.,1.,1.,1.,1.,1.,1.,1.,1.,1.,1.,1.,1.,1.,1.,1.,1.,1.,1.,1.,1.,1.,1.,
1.,1.,1.,1.,1.,1.,1.,1.,1.,1.,1.,1.,1.,1.,1.,1.,1.,1.,1.,1.,1.,1.,1.,1.,
1.,1.,1.,1.,1.,1.))
REPRESENTATION_ITEM('')
);
#373=(
BOUNDED_CURVE()
B_SPLINE_CURVE(5,(#52698,#52699,#52700,#52701,#52702,#52703,#52704,#52705,
#52706,#52707,#52708,#52709,#52710,#52711,#52712,#52713,#52714,#52715,#52716,
#52717,#52718,#52719,#52720,#52721,#52722,#52723,#52724,#52725,#52726,#52727,
#52728,#52729,#52730,#52731,#52732,#52733,#52734,#52735,#52736,#52737,#52738,
#52739,#52740,#52741,#52742,#52743,#52744,#52745,#52746,#52747,#52748,#52749,
#52750,#52751,#52752,#52753,#52754,#52755,#52756,#52757,#52758,#52759,#52760,
#52761,#52762,#52763,#52764,#52765,#52766,#52767),.UNSPECIFIED.,.F.,.F.)
B_SPLINE_CURVE_WITH_KNOTS((6,1,1,1,1,1,1,1,1,1,1,1,1,1,1,1,1,1,1,1,1,1,
1,1,1,1,1,1,1,1,1,1,1,1,1,1,1,1,1,1,1,1,1,1,1,1,1,1,1,1,1,1,1,1,1,1,1,1,
1,1,1,1,1,1,1,6),(0.00577184337452087,0.0153846153846154,0.0307692307692308,
0.0461538461538462,0.0615384615384615,0.0769230769230769,0.0923076923076923,
0.107692307692308,0.123076923076923,0.138461538461538,0.153846153846154,
0.169230769230769,0.184615384615385,0.2,0.215384615384615,0.230769230769231,
0.246153846153846,0.261538461538462,0.276923076923077,0.292307692307692,
0.307692307692308,0.323076923076923,0.338461538461538,0.353846153846154,
0.369230769230769,0.384615384615385,0.4,0.415384615384615,0.430769230769231,
0.446153846153846,0.461538461538462,0.476923076923077,0.492307692307692,
0.507692307692308,0.523076923076923,0.538461538461538,0.553846153846154,
0.569230769230769,0.584615384615384,0.6,0.615384615384615,0.63076923076923,
0.646153846153846,0.661538461538461,0.676923076923076,0.692307692307692,
0.707692307692307,0.723076923076922,0.738461538461538,0.753846153846153,
0.769230769230768,0.784615384615384,0.799999999999999,0.815384615384614,
0.83076923076923,0.846153846153845,0.86153846153846,0.876923076923076,0.892307692307691,
0.907692307692306,0.923076923076922,0.938461538461537,0.953846153846152,
0.969230769230768,0.984615384615383,1.),.UNSPECIFIED.)
CURVE()
GEOMETRIC_REPRESENTATION_ITEM()
RATIONAL_B_SPLINE_CURVE((1.,1.,1.,1.,1.,1.,1.,1.,1.,1.,1.,1.,1.,1.,1.,1.,
1.,1.,1.,1.,1.,1.,1.,1.,1.,1.,1.,1.,1.,1.,1.,1.,1.,1.,1.,1.,1.,1.,1.,1.,
1.,1.,1.,1.,1.,1.,1.,1.,1.,1.,1.,1.,1.,1.,1.,1.,1.,1.,1.,1.,1.,1.,1.,1.,
1.,1.,1.,1.,1.,1.))
REPRESENTATION_ITEM('')
);
#374=(
BOUNDED_CURVE()
B_SPLINE_CURVE(5,(#52771,#52772,#52773,#52774,#52775,#52776,#52777,#52778,
#52779,#52780,#52781,#52782,#52783,#52784,#52785,#52786,#52787,#52788,#52789,
#52790,#52791,#52792,#52793,#52794,#52795,#52796,#52797,#52798,#52799,#52800,
#52801,#52802,#52803,#52804,#52805,#52806,#52807,#52808,#52809,#52810,#52811,
#52812,#52813,#52814,#52815,#52816,#52817,#52818,#52819,#52820,#52821,#52822,
#52823,#52824,#52825,#52826,#52827,#52828,#52829,#52830,#52831,#52832,#52833,
#52834,#52835,#52836,#52837,#52838,#52839,#52840),.UNSPECIFIED.,.F.,.F.)
B_SPLINE_CURVE_WITH_KNOTS((6,1,1,1,1,1,1,1,1,1,1,1,1,1,1,1,1,1,1,1,1,1,
1,1,1,1,1,1,1,1,1,1,1,1,1,1,1,1,1,1,1,1,1,1,1,1,1,1,1,1,1,1,1,1,1,1,1,1,
1,1,1,1,1,1,1,6),(0.,0.0153846153846154,0.0307692307692308,0.0461538461538462,
0.0615384615384615,0.0769230769230769,0.0923076923076923,0.107692307692308,
0.123076923076923,0.138461538461538,0.153846153846154,0.169230769230769,
0.184615384615385,0.2,0.215384615384615,0.230769230769231,0.246153846153846,
0.261538461538462,0.276923076923077,0.292307692307692,0.307692307692308,
0.323076923076923,0.338461538461538,0.353846153846154,0.369230769230769,
0.384615384615385,0.4,0.415384615384615,0.430769230769231,0.446153846153846,
0.461538461538462,0.476923076923077,0.492307692307692,0.507692307692308,
0.523076923076923,0.538461538461538,0.553846153846154,0.569230769230769,
0.584615384615384,0.6,0.615384615384615,0.63076923076923,0.646153846153846,
0.661538461538461,0.676923076923076,0.692307692307692,0.707692307692307,
0.723076923076922,0.738461538461538,0.753846153846153,0.769230769230768,
0.784615384615384,0.799999999999999,0.815384615384614,0.83076923076923,
0.846153846153845,0.86153846153846,0.876923076923076,0.892307692307691,
0.907692307692306,0.923076923076922,0.938461538461537,0.953846153846152,
0.969230769230768,0.984615384615383,0.994228156739692),.UNSPECIFIED.)
CURVE()
GEOMETRIC_REPRESENTATION_ITEM()
RATIONAL_B_SPLINE_CURVE((1.,1.,1.,1.,1.,1.,1.,1.,1.,1.,1.,1.,1.,1.,1.,1.,
1.,1.,1.,1.,1.,1.,1.,1.,1.,1.,1.,1.,1.,1.,1.,1.,1.,1.,1.,1.,1.,1.,1.,1.,
1.,1.,1.,1.,1.,1.,1.,1.,1.,1.,1.,1.,1.,1.,1.,1.,1.,1.,1.,1.,1.,1.,1.,1.,
1.,1.,1.,1.,1.,1.))
REPRESENTATION_ITEM('')
);
#375=(
BOUNDED_CURVE()
B_SPLINE_CURVE(5,(#52844,#52845,#52846,#52847,#52848,#52849,#52850,#52851,
#52852,#52853,#52854,#52855,#52856,#52857,#52858,#52859,#52860,#52861,#52862,
#52863,#52864,#52865,#52866,#52867,#52868,#52869,#52870,#52871,#52872,#52873,
#52874,#52875,#52876,#52877,#52878,#52879,#52880,#52881,#52882,#52883,#52884,
#52885,#52886,#52887,#52888,#52889,#52890,#52891,#52892,#52893,#52894,#52895,
#52896,#52897,#52898,#52899,#52900,#52901,#52902,#52903,#52904,#52905,#52906,
#52907,#52908,#52909,#52910,#52911,#52912,#52913),.UNSPECIFIED.,.F.,.F.)
B_SPLINE_CURVE_WITH_KNOTS((6,1,1,1,1,1,1,1,1,1,1,1,1,1,1,1,1,1,1,1,1,1,
1,1,1,1,1,1,1,1,1,1,1,1,1,1,1,1,1,1,1,1,1,1,1,1,1,1,1,1,1,1,1,1,1,1,1,1,
1,1,1,1,1,1,1,6),(0.00577184337450777,0.0153846153846154,0.0307692307692308,
0.0461538461538462,0.0615384615384615,0.0769230769230769,0.0923076923076923,
0.107692307692308,0.123076923076923,0.138461538461538,0.153846153846154,
0.169230769230769,0.184615384615385,0.2,0.215384615384615,0.230769230769231,
0.246153846153846,0.261538461538462,0.276923076923077,0.292307692307692,
0.307692307692308,0.323076923076923,0.338461538461538,0.353846153846154,
0.369230769230769,0.384615384615385,0.4,0.415384615384615,0.430769230769231,
0.446153846153846,0.461538461538462,0.476923076923077,0.492307692307692,
0.507692307692308,0.523076923076923,0.538461538461538,0.553846153846154,
0.569230769230769,0.584615384615384,0.6,0.615384615384615,0.63076923076923,
0.646153846153846,0.661538461538461,0.676923076923076,0.692307692307692,
0.707692307692307,0.723076923076922,0.738461538461538,0.753846153846153,
0.769230769230768,0.784615384615384,0.799999999999999,0.815384615384614,
0.83076923076923,0.846153846153845,0.86153846153846,0.876923076923076,0.892307692307691,
0.907692307692306,0.923076923076922,0.938461538461537,0.953846153846152,
0.969230769230768,0.984615384615383,1.),.UNSPECIFIED.)
CURVE()
GEOMETRIC_REPRESENTATION_ITEM()
RATIONAL_B_SPLINE_CURVE((1.,1.,1.,1.,1.,1.,1.,1.,1.,1.,1.,1.,1.,1.,1.,1.,
1.,1.,1.,1.,1.,1.,1.,1.,1.,1.,1.,1.,1.,1.,1.,1.,1.,1.,1.,1.,1.,1.,1.,1.,
1.,1.,1.,1.,1.,1.,1.,1.,1.,1.,1.,1.,1.,1.,1.,1.,1.,1.,1.,1.,1.,1.,1.,1.,
1.,1.,1.,1.,1.,1.))
REPRESENTATION_ITEM('')
);
#376=(
BOUNDED_CURVE()
B_SPLINE_CURVE(5,(#52917,#52918,#52919,#52920,#52921,#52922,#52923,#52924,
#52925,#52926,#52927,#52928,#52929,#52930,#52931,#52932,#52933,#52934,#52935,
#52936,#52937,#52938,#52939,#52940,#52941,#52942,#52943,#52944,#52945,#52946,
#52947,#52948,#52949,#52950,#52951,#52952,#52953,#52954,#52955,#52956,#52957,
#52958,#52959,#52960,#52961,#52962,#52963,#52964,#52965,#52966,#52967,#52968,
#52969,#52970,#52971,#52972,#52973,#52974,#52975,#52976,#52977,#52978,#52979,
#52980,#52981,#52982,#52983,#52984,#52985,#52986),.UNSPECIFIED.,.F.,.F.)
B_SPLINE_CURVE_WITH_KNOTS((6,1,1,1,1,1,1,1,1,1,1,1,1,1,1,1,1,1,1,1,1,1,
1,1,1,1,1,1,1,1,1,1,1,1,1,1,1,1,1,1,1,1,1,1,1,1,1,1,1,1,1,1,1,1,1,1,1,1,
1,1,1,1,1,1,1,6),(0.,0.0153846153846154,0.0307692307692308,0.0461538461538462,
0.0615384615384615,0.0769230769230769,0.0923076923076923,0.107692307692308,
0.123076923076923,0.138461538461538,0.153846153846154,0.169230769230769,
0.184615384615385,0.2,0.215384615384615,0.230769230769231,0.246153846153846,
0.261538461538462,0.276923076923077,0.292307692307692,0.307692307692308,
0.323076923076923,0.338461538461538,0.353846153846154,0.369230769230769,
0.384615384615385,0.4,0.415384615384615,0.430769230769231,0.446153846153846,
0.461538461538462,0.476923076923077,0.492307692307692,0.507692307692308,
0.523076923076923,0.538461538461538,0.553846153846154,0.569230769230769,
0.584615384615384,0.6,0.615384615384615,0.63076923076923,0.646153846153846,
0.661538461538461,0.676923076923076,0.692307692307692,0.707692307692307,
0.723076923076922,0.738461538461538,0.753846153846153,0.769230769230768,
0.784615384615384,0.799999999999999,0.815384615384614,0.83076923076923,
0.846153846153845,0.86153846153846,0.876923076923076,0.892307692307691,
0.907692307692306,0.923076923076922,0.938461538461537,0.953846153846152,
0.969230769230768,0.984615384615383,0.994228156739701),.UNSPECIFIED.)
CURVE()
GEOMETRIC_REPRESENTATION_ITEM()
RATIONAL_B_SPLINE_CURVE((1.,1.,1.,1.,1.,1.,1.,1.,1.,1.,1.,1.,1.,1.,1.,1.,
1.,1.,1.,1.,1.,1.,1.,1.,1.,1.,1.,1.,1.,1.,1.,1.,1.,1.,1.,1.,1.,1.,1.,1.,
1.,1.,1.,1.,1.,1.,1.,1.,1.,1.,1.,1.,1.,1.,1.,1.,1.,1.,1.,1.,1.,1.,1.,1.,
1.,1.,1.,1.,1.,1.))
REPRESENTATION_ITEM('')
);
#377=(
BOUNDED_CURVE()
B_SPLINE_CURVE(5,(#52990,#52991,#52992,#52993,#52994,#52995,#52996,#52997,
#52998,#52999,#53000,#53001,#53002,#53003,#53004,#53005,#53006,#53007,#53008,
#53009,#53010,#53011,#53012,#53013,#53014,#53015,#53016,#53017,#53018,#53019,
#53020,#53021,#53022,#53023,#53024,#53025,#53026,#53027,#53028,#53029,#53030,
#53031,#53032,#53033,#53034,#53035,#53036,#53037,#53038,#53039,#53040,#53041,
#53042,#53043,#53044,#53045,#53046,#53047,#53048,#53049,#53050,#53051,#53052,
#53053,#53054,#53055,#53056,#53057,#53058,#53059),.UNSPECIFIED.,.F.,.F.)
B_SPLINE_CURVE_WITH_KNOTS((6,1,1,1,1,1,1,1,1,1,1,1,1,1,1,1,1,1,1,1,1,1,
1,1,1,1,1,1,1,1,1,1,1,1,1,1,1,1,1,1,1,1,1,1,1,1,1,1,1,1,1,1,1,1,1,1,1,1,
1,1,1,1,1,1,1,6),(0.00577184337450943,0.0153846153846154,0.0307692307692308,
0.0461538461538462,0.0615384615384615,0.0769230769230769,0.0923076923076923,
0.107692307692308,0.123076923076923,0.138461538461538,0.153846153846154,
0.169230769230769,0.184615384615385,0.2,0.215384615384615,0.230769230769231,
0.246153846153846,0.261538461538462,0.276923076923077,0.292307692307692,
0.307692307692308,0.323076923076923,0.338461538461538,0.353846153846154,
0.369230769230769,0.384615384615385,0.4,0.415384615384615,0.430769230769231,
0.446153846153846,0.461538461538462,0.476923076923077,0.492307692307692,
0.507692307692308,0.523076923076923,0.538461538461538,0.553846153846154,
0.569230769230769,0.584615384615384,0.6,0.615384615384615,0.63076923076923,
0.646153846153846,0.661538461538461,0.676923076923076,0.692307692307692,
0.707692307692307,0.723076923076922,0.738461538461538,0.753846153846153,
0.769230769230768,0.784615384615384,0.799999999999999,0.815384615384614,
0.83076923076923,0.846153846153845,0.86153846153846,0.876923076923076,0.892307692307691,
0.907692307692306,0.923076923076922,0.938461538461537,0.953846153846152,
0.969230769230768,0.984615384615383,1.),.UNSPECIFIED.)
CURVE()
GEOMETRIC_REPRESENTATION_ITEM()
RATIONAL_B_SPLINE_CURVE((1.,1.,1.,1.,1.,1.,1.,1.,1.,1.,1.,1.,1.,1.,1.,1.,
1.,1.,1.,1.,1.,1.,1.,1.,1.,1.,1.,1.,1.,1.,1.,1.,1.,1.,1.,1.,1.,1.,1.,1.,
1.,1.,1.,1.,1.,1.,1.,1.,1.,1.,1.,1.,1.,1.,1.,1.,1.,1.,1.,1.,1.,1.,1.,1.,
1.,1.,1.,1.,1.,1.))
REPRESENTATION_ITEM('')
);
#378=(
BOUNDED_CURVE()
B_SPLINE_CURVE(5,(#53063,#53064,#53065,#53066,#53067,#53068,#53069,#53070,
#53071,#53072,#53073,#53074,#53075,#53076,#53077,#53078,#53079,#53080,#53081,
#53082,#53083,#53084,#53085,#53086,#53087,#53088,#53089,#53090,#53091,#53092,
#53093,#53094,#53095,#53096,#53097,#53098,#53099,#53100,#53101,#53102,#53103,
#53104,#53105,#53106,#53107,#53108,#53109,#53110,#53111,#53112,#53113,#53114,
#53115,#53116,#53117,#53118,#53119,#53120,#53121,#53122,#53123,#53124,#53125,
#53126,#53127,#53128,#53129,#53130,#53131,#53132),.UNSPECIFIED.,.F.,.F.)
B_SPLINE_CURVE_WITH_KNOTS((6,1,1,1,1,1,1,1,1,1,1,1,1,1,1,1,1,1,1,1,1,1,
1,1,1,1,1,1,1,1,1,1,1,1,1,1,1,1,1,1,1,1,1,1,1,1,1,1,1,1,1,1,1,1,1,1,1,1,
1,1,1,1,1,1,1,6),(0.,0.0153846153846154,0.0307692307692308,0.0461538461538462,
0.0615384615384615,0.0769230769230769,0.0923076923076923,0.107692307692308,
0.123076923076923,0.138461538461538,0.153846153846154,0.169230769230769,
0.184615384615385,0.2,0.215384615384615,0.230769230769231,0.246153846153846,
0.261538461538462,0.276923076923077,0.292307692307692,0.307692307692308,
0.323076923076923,0.338461538461538,0.353846153846154,0.369230769230769,
0.384615384615385,0.4,0.415384615384615,0.430769230769231,0.446153846153846,
0.461538461538462,0.476923076923077,0.492307692307692,0.507692307692308,
0.523076923076923,0.538461538461538,0.553846153846154,0.569230769230769,
0.584615384615384,0.6,0.615384615384615,0.63076923076923,0.646153846153846,
0.661538461538461,0.676923076923076,0.692307692307692,0.707692307692307,
0.723076923076922,0.738461538461538,0.753846153846153,0.769230769230768,
0.784615384615384,0.799999999999999,0.815384615384614,0.83076923076923,
0.846153846153845,0.86153846153846,0.876923076923076,0.892307692307691,
0.907692307692306,0.923076923076922,0.938461538461537,0.953846153846152,
0.969230769230768,0.984615384615383,0.994228156739699),.UNSPECIFIED.)
CURVE()
GEOMETRIC_REPRESENTATION_ITEM()
RATIONAL_B_SPLINE_CURVE((1.,1.,1.,1.,1.,1.,1.,1.,1.,1.,1.,1.,1.,1.,1.,1.,
1.,1.,1.,1.,1.,1.,1.,1.,1.,1.,1.,1.,1.,1.,1.,1.,1.,1.,1.,1.,1.,1.,1.,1.,
1.,1.,1.,1.,1.,1.,1.,1.,1.,1.,1.,1.,1.,1.,1.,1.,1.,1.,1.,1.,1.,1.,1.,1.,
1.,1.,1.,1.,1.,1.))
REPRESENTATION_ITEM('')
);
#379=(
BOUNDED_CURVE()
B_SPLINE_CURVE(5,(#53136,#53137,#53138,#53139,#53140,#53141,#53142,#53143,
#53144,#53145,#53146,#53147,#53148,#53149,#53150,#53151,#53152,#53153,#53154,
#53155,#53156,#53157,#53158,#53159,#53160,#53161,#53162,#53163,#53164,#53165,
#53166,#53167,#53168,#53169,#53170,#53171,#53172,#53173,#53174,#53175,#53176,
#53177,#53178,#53179,#53180,#53181,#53182,#53183,#53184,#53185,#53186,#53187,
#53188,#53189,#53190,#53191,#53192,#53193,#53194,#53195,#53196,#53197,#53198,
#53199,#53200,#53201,#53202,#53203,#53204,#53205),.UNSPECIFIED.,.F.,.F.)
B_SPLINE_CURVE_WITH_KNOTS((6,1,1,1,1,1,1,1,1,1,1,1,1,1,1,1,1,1,1,1,1,1,
1,1,1,1,1,1,1,1,1,1,1,1,1,1,1,1,1,1,1,1,1,1,1,1,1,1,1,1,1,1,1,1,1,1,1,1,
1,1,1,1,1,1,1,6),(0.00577184337448657,0.0153846153846154,0.0307692307692308,
0.0461538461538462,0.0615384615384615,0.0769230769230769,0.0923076923076923,
0.107692307692308,0.123076923076923,0.138461538461538,0.153846153846154,
0.169230769230769,0.184615384615385,0.2,0.215384615384615,0.230769230769231,
0.246153846153846,0.261538461538462,0.276923076923077,0.292307692307692,
0.307692307692308,0.323076923076923,0.338461538461538,0.353846153846154,
0.369230769230769,0.384615384615385,0.4,0.415384615384615,0.430769230769231,
0.446153846153846,0.461538461538462,0.476923076923077,0.492307692307692,
0.507692307692308,0.523076923076923,0.538461538461538,0.553846153846154,
0.569230769230769,0.584615384615384,0.6,0.615384615384615,0.63076923076923,
0.646153846153846,0.661538461538461,0.676923076923076,0.692307692307692,
0.707692307692307,0.723076923076922,0.738461538461538,0.753846153846153,
0.769230769230768,0.784615384615384,0.799999999999999,0.815384615384614,
0.83076923076923,0.846153846153845,0.86153846153846,0.876923076923076,0.892307692307691,
0.907692307692306,0.923076923076922,0.938461538461537,0.953846153846152,
0.969230769230768,0.984615384615383,1.),.UNSPECIFIED.)
CURVE()
GEOMETRIC_REPRESENTATION_ITEM()
RATIONAL_B_SPLINE_CURVE((1.,1.,1.,1.,1.,1.,1.,1.,1.,1.,1.,1.,1.,1.,1.,1.,
1.,1.,1.,1.,1.,1.,1.,1.,1.,1.,1.,1.,1.,1.,1.,1.,1.,1.,1.,1.,1.,1.,1.,1.,
1.,1.,1.,1.,1.,1.,1.,1.,1.,1.,1.,1.,1.,1.,1.,1.,1.,1.,1.,1.,1.,1.,1.,1.,
1.,1.,1.,1.,1.,1.))
REPRESENTATION_ITEM('')
);
#380=(
BOUNDED_CURVE()
B_SPLINE_CURVE(5,(#53209,#53210,#53211,#53212,#53213,#53214,#53215,#53216,
#53217,#53218,#53219,#53220,#53221,#53222,#53223,#53224,#53225,#53226,#53227,
#53228,#53229,#53230,#53231,#53232,#53233,#53234,#53235,#53236,#53237,#53238,
#53239,#53240,#53241,#53242,#53243,#53244,#53245,#53246,#53247,#53248,#53249,
#53250,#53251,#53252,#53253,#53254,#53255,#53256,#53257,#53258,#53259,#53260,
#53261,#53262,#53263,#53264,#53265,#53266,#53267,#53268,#53269,#53270,#53271,
#53272,#53273,#53274,#53275,#53276,#53277,#53278),.UNSPECIFIED.,.F.,.F.)
B_SPLINE_CURVE_WITH_KNOTS((6,1,1,1,1,1,1,1,1,1,1,1,1,1,1,1,1,1,1,1,1,1,
1,1,1,1,1,1,1,1,1,1,1,1,1,1,1,1,1,1,1,1,1,1,1,1,1,1,1,1,1,1,1,1,1,1,1,1,
1,1,1,1,1,1,1,6),(0.,0.0153846153846154,0.0307692307692308,0.0461538461538462,
0.0615384615384615,0.0769230769230769,0.0923076923076923,0.107692307692308,
0.123076923076923,0.138461538461538,0.153846153846154,0.169230769230769,
0.184615384615385,0.2,0.215384615384615,0.230769230769231,0.246153846153846,
0.261538461538462,0.276923076923077,0.292307692307692,0.307692307692308,
0.323076923076923,0.338461538461538,0.353846153846154,0.369230769230769,
0.384615384615385,0.4,0.415384615384615,0.430769230769231,0.446153846153846,
0.461538461538462,0.476923076923077,0.492307692307692,0.507692307692308,
0.523076923076923,0.538461538461538,0.553846153846154,0.569230769230769,
0.584615384615384,0.6,0.615384615384615,0.63076923076923,0.646153846153846,
0.661538461538461,0.676923076923076,0.692307692307692,0.707692307692307,
0.723076923076922,0.738461538461538,0.753846153846153,0.769230769230768,
0.784615384615384,0.799999999999999,0.815384615384614,0.83076923076923,
0.846153846153845,0.86153846153846,0.876923076923076,0.892307692307691,
0.907692307692306,0.923076923076922,0.938461538461537,0.953846153846152,
0.969230769230768,0.984615384615383,0.994228156739709),.UNSPECIFIED.)
CURVE()
GEOMETRIC_REPRESENTATION_ITEM()
RATIONAL_B_SPLINE_CURVE((1.,1.,1.,1.,1.,1.,1.,1.,1.,1.,1.,1.,1.,1.,1.,1.,
1.,1.,1.,1.,1.,1.,1.,1.,1.,1.,1.,1.,1.,1.,1.,1.,1.,1.,1.,1.,1.,1.,1.,1.,
1.,1.,1.,1.,1.,1.,1.,1.,1.,1.,1.,1.,1.,1.,1.,1.,1.,1.,1.,1.,1.,1.,1.,1.,
1.,1.,1.,1.,1.,1.))
REPRESENTATION_ITEM('')
);
#381=(
BOUNDED_CURVE()
B_SPLINE_CURVE(5,(#53282,#53283,#53284,#53285,#53286,#53287,#53288,#53289,
#53290,#53291,#53292,#53293,#53294,#53295,#53296,#53297,#53298,#53299,#53300,
#53301,#53302,#53303,#53304,#53305,#53306,#53307,#53308,#53309,#53310,#53311,
#53312,#53313,#53314,#53315,#53316,#53317,#53318,#53319,#53320,#53321,#53322,
#53323,#53324,#53325,#53326,#53327,#53328,#53329,#53330,#53331,#53332,#53333,
#53334,#53335,#53336,#53337,#53338,#53339,#53340,#53341,#53342,#53343,#53344,
#53345,#53346,#53347,#53348,#53349,#53350,#53351),.UNSPECIFIED.,.F.,.F.)
B_SPLINE_CURVE_WITH_KNOTS((6,1,1,1,1,1,1,1,1,1,1,1,1,1,1,1,1,1,1,1,1,1,
1,1,1,1,1,1,1,1,1,1,1,1,1,1,1,1,1,1,1,1,1,1,1,1,1,1,1,1,1,1,1,1,1,1,1,1,
1,1,1,1,1,1,1,6),(0.00577184337451132,0.0153846153846154,0.0307692307692308,
0.0461538461538462,0.0615384615384615,0.0769230769230769,0.0923076923076923,
0.107692307692308,0.123076923076923,0.138461538461538,0.153846153846154,
0.169230769230769,0.184615384615385,0.2,0.215384615384615,0.230769230769231,
0.246153846153846,0.261538461538462,0.276923076923077,0.292307692307692,
0.307692307692308,0.323076923076923,0.338461538461538,0.353846153846154,
0.369230769230769,0.384615384615385,0.4,0.415384615384615,0.430769230769231,
0.446153846153846,0.461538461538462,0.476923076923077,0.492307692307692,
0.507692307692308,0.523076923076923,0.538461538461538,0.553846153846154,
0.569230769230769,0.584615384615384,0.6,0.615384615384615,0.63076923076923,
0.646153846153846,0.661538461538461,0.676923076923076,0.692307692307692,
0.707692307692307,0.723076923076922,0.738461538461538,0.753846153846153,
0.769230769230768,0.784615384615384,0.799999999999999,0.815384615384614,
0.83076923076923,0.846153846153845,0.86153846153846,0.876923076923076,0.892307692307691,
0.907692307692306,0.923076923076922,0.938461538461537,0.953846153846152,
0.969230769230768,0.984615384615383,1.),.UNSPECIFIED.)
CURVE()
GEOMETRIC_REPRESENTATION_ITEM()
RATIONAL_B_SPLINE_CURVE((1.,1.,1.,1.,1.,1.,1.,1.,1.,1.,1.,1.,1.,1.,1.,1.,
1.,1.,1.,1.,1.,1.,1.,1.,1.,1.,1.,1.,1.,1.,1.,1.,1.,1.,1.,1.,1.,1.,1.,1.,
1.,1.,1.,1.,1.,1.,1.,1.,1.,1.,1.,1.,1.,1.,1.,1.,1.,1.,1.,1.,1.,1.,1.,1.,
1.,1.,1.,1.,1.,1.))
REPRESENTATION_ITEM('')
);
#382=(
BOUNDED_CURVE()
B_SPLINE_CURVE(5,(#53355,#53356,#53357,#53358,#53359,#53360,#53361,#53362,
#53363,#53364,#53365,#53366,#53367,#53368,#53369,#53370,#53371,#53372,#53373,
#53374,#53375,#53376,#53377,#53378,#53379,#53380,#53381,#53382,#53383,#53384,
#53385,#53386,#53387,#53388,#53389,#53390,#53391,#53392,#53393,#53394,#53395,
#53396,#53397,#53398,#53399,#53400,#53401,#53402,#53403,#53404,#53405,#53406,
#53407,#53408,#53409,#53410,#53411,#53412,#53413,#53414,#53415,#53416,#53417,
#53418,#53419,#53420,#53421,#53422,#53423,#53424),.UNSPECIFIED.,.F.,.F.)
B_SPLINE_CURVE_WITH_KNOTS((6,1,1,1,1,1,1,1,1,1,1,1,1,1,1,1,1,1,1,1,1,1,
1,1,1,1,1,1,1,1,1,1,1,1,1,1,1,1,1,1,1,1,1,1,1,1,1,1,1,1,1,1,1,1,1,1,1,1,
1,1,1,1,1,1,1,6),(0.,0.0153846153846154,0.0307692307692308,0.0461538461538462,
0.0615384615384615,0.0769230769230769,0.0923076923076923,0.107692307692308,
0.123076923076923,0.138461538461538,0.153846153846154,0.169230769230769,
0.184615384615385,0.2,0.215384615384615,0.230769230769231,0.246153846153846,
0.261538461538462,0.276923076923077,0.292307692307692,0.307692307692308,
0.323076923076923,0.338461538461538,0.353846153846154,0.369230769230769,
0.384615384615385,0.4,0.415384615384615,0.430769230769231,0.446153846153846,
0.461538461538462,0.476923076923077,0.492307692307692,0.507692307692308,
0.523076923076923,0.538461538461538,0.553846153846154,0.569230769230769,
0.584615384615384,0.6,0.615384615384615,0.63076923076923,0.646153846153846,
0.661538461538461,0.676923076923076,0.692307692307692,0.707692307692307,
0.723076923076922,0.738461538461538,0.753846153846153,0.769230769230768,
0.784615384615384,0.799999999999999,0.815384615384614,0.83076923076923,
0.846153846153845,0.86153846153846,0.876923076923076,0.892307692307691,
0.907692307692306,0.923076923076922,0.938461538461537,0.953846153846152,
0.969230769230768,0.984615384615383,0.994228156739705),.UNSPECIFIED.)
CURVE()
GEOMETRIC_REPRESENTATION_ITEM()
RATIONAL_B_SPLINE_CURVE((1.,1.,1.,1.,1.,1.,1.,1.,1.,1.,1.,1.,1.,1.,1.,1.,
1.,1.,1.,1.,1.,1.,1.,1.,1.,1.,1.,1.,1.,1.,1.,1.,1.,1.,1.,1.,1.,1.,1.,1.,
1.,1.,1.,1.,1.,1.,1.,1.,1.,1.,1.,1.,1.,1.,1.,1.,1.,1.,1.,1.,1.,1.,1.,1.,
1.,1.,1.,1.,1.,1.))
REPRESENTATION_ITEM('')
);
#383=(
BOUNDED_CURVE()
B_SPLINE_CURVE(5,(#53428,#53429,#53430,#53431,#53432,#53433,#53434,#53435,
#53436,#53437,#53438,#53439,#53440,#53441,#53442,#53443,#53444,#53445,#53446,
#53447,#53448,#53449,#53450,#53451,#53452,#53453,#53454,#53455,#53456,#53457,
#53458,#53459,#53460,#53461,#53462,#53463,#53464,#53465,#53466,#53467,#53468,
#53469,#53470,#53471,#53472,#53473,#53474,#53475,#53476,#53477,#53478,#53479,
#53480,#53481,#53482,#53483,#53484,#53485,#53486,#53487,#53488,#53489,#53490,
#53491,#53492,#53493,#53494,#53495,#53496,#53497),.UNSPECIFIED.,.F.,.F.)
B_SPLINE_CURVE_WITH_KNOTS((6,1,1,1,1,1,1,1,1,1,1,1,1,1,1,1,1,1,1,1,1,1,
1,1,1,1,1,1,1,1,1,1,1,1,1,1,1,1,1,1,1,1,1,1,1,1,1,1,1,1,1,1,1,1,1,1,1,1,
1,1,1,1,1,1,1,6),(0.00577184337450072,0.0153846153846154,0.0307692307692308,
0.0461538461538462,0.0615384615384615,0.0769230769230769,0.0923076923076923,
0.107692307692308,0.123076923076923,0.138461538461538,0.153846153846154,
0.169230769230769,0.184615384615385,0.2,0.215384615384615,0.230769230769231,
0.246153846153846,0.261538461538462,0.276923076923077,0.292307692307692,
0.307692307692308,0.323076923076923,0.338461538461538,0.353846153846154,
0.369230769230769,0.384615384615385,0.4,0.415384615384615,0.430769230769231,
0.446153846153846,0.461538461538462,0.476923076923077,0.492307692307692,
0.507692307692308,0.523076923076923,0.538461538461538,0.553846153846154,
0.569230769230769,0.584615384615384,0.6,0.615384615384615,0.63076923076923,
0.646153846153846,0.661538461538461,0.676923076923076,0.692307692307692,
0.707692307692307,0.723076923076922,0.738461538461538,0.753846153846153,
0.769230769230768,0.784615384615384,0.799999999999999,0.815384615384614,
0.83076923076923,0.846153846153845,0.86153846153846,0.876923076923076,0.892307692307691,
0.907692307692306,0.923076923076922,0.938461538461537,0.953846153846152,
0.969230769230768,0.984615384615383,1.),.UNSPECIFIED.)
CURVE()
GEOMETRIC_REPRESENTATION_ITEM()
RATIONAL_B_SPLINE_CURVE((1.,1.,1.,1.,1.,1.,1.,1.,1.,1.,1.,1.,1.,1.,1.,1.,
1.,1.,1.,1.,1.,1.,1.,1.,1.,1.,1.,1.,1.,1.,1.,1.,1.,1.,1.,1.,1.,1.,1.,1.,
1.,1.,1.,1.,1.,1.,1.,1.,1.,1.,1.,1.,1.,1.,1.,1.,1.,1.,1.,1.,1.,1.,1.,1.,
1.,1.,1.,1.,1.,1.))
REPRESENTATION_ITEM('')
);
#384=(
BOUNDED_CURVE()
B_SPLINE_CURVE(5,(#53501,#53502,#53503,#53504,#53505,#53506,#53507,#53508,
#53509,#53510,#53511,#53512,#53513,#53514,#53515,#53516,#53517,#53518,#53519,
#53520,#53521,#53522,#53523,#53524,#53525,#53526,#53527,#53528,#53529,#53530,
#53531,#53532,#53533,#53534,#53535,#53536,#53537,#53538,#53539,#53540,#53541,
#53542,#53543,#53544,#53545,#53546,#53547,#53548,#53549,#53550,#53551,#53552,
#53553,#53554,#53555,#53556,#53557,#53558,#53559,#53560,#53561,#53562,#53563,
#53564,#53565,#53566,#53567,#53568,#53569,#53570),.UNSPECIFIED.,.F.,.F.)
B_SPLINE_CURVE_WITH_KNOTS((6,1,1,1,1,1,1,1,1,1,1,1,1,1,1,1,1,1,1,1,1,1,
1,1,1,1,1,1,1,1,1,1,1,1,1,1,1,1,1,1,1,1,1,1,1,1,1,1,1,1,1,1,1,1,1,1,1,1,
1,1,1,1,1,1,1,6),(0.,0.0153846153846154,0.0307692307692308,0.0461538461538462,
0.0615384615384615,0.0769230769230769,0.0923076923076923,0.107692307692308,
0.123076923076923,0.138461538461538,0.153846153846154,0.169230769230769,
0.184615384615385,0.2,0.215384615384615,0.230769230769231,0.246153846153846,
0.261538461538462,0.276923076923077,0.292307692307692,0.307692307692308,
0.323076923076923,0.338461538461538,0.353846153846154,0.369230769230769,
0.384615384615385,0.4,0.415384615384615,0.430769230769231,0.446153846153846,
0.461538461538462,0.476923076923077,0.492307692307692,0.507692307692308,
0.523076923076923,0.538461538461538,0.553846153846154,0.569230769230769,
0.584615384615384,0.6,0.615384615384615,0.63076923076923,0.646153846153846,
0.661538461538461,0.676923076923076,0.692307692307692,0.707692307692307,
0.723076923076922,0.738461538461538,0.753846153846153,0.769230769230768,
0.784615384615384,0.799999999999999,0.815384615384614,0.83076923076923,
0.846153846153845,0.86153846153846,0.876923076923076,0.892307692307691,
0.907692307692306,0.923076923076922,0.938461538461537,0.953846153846152,
0.969230769230768,0.984615384615383,0.994228156739706),.UNSPECIFIED.)
CURVE()
GEOMETRIC_REPRESENTATION_ITEM()
RATIONAL_B_SPLINE_CURVE((1.,1.,1.,1.,1.,1.,1.,1.,1.,1.,1.,1.,1.,1.,1.,1.,
1.,1.,1.,1.,1.,1.,1.,1.,1.,1.,1.,1.,1.,1.,1.,1.,1.,1.,1.,1.,1.,1.,1.,1.,
1.,1.,1.,1.,1.,1.,1.,1.,1.,1.,1.,1.,1.,1.,1.,1.,1.,1.,1.,1.,1.,1.,1.,1.,
1.,1.,1.,1.,1.,1.))
REPRESENTATION_ITEM('')
);
#385=(
BOUNDED_CURVE()
B_SPLINE_CURVE(5,(#53574,#53575,#53576,#53577,#53578,#53579,#53580,#53581,
#53582,#53583,#53584,#53585,#53586,#53587,#53588,#53589,#53590,#53591,#53592,
#53593,#53594,#53595,#53596,#53597,#53598,#53599,#53600,#53601,#53602,#53603,
#53604,#53605,#53606,#53607,#53608,#53609,#53610,#53611,#53612,#53613,#53614,
#53615,#53616,#53617,#53618,#53619,#53620,#53621,#53622,#53623,#53624,#53625,
#53626,#53627,#53628,#53629,#53630,#53631,#53632,#53633,#53634,#53635,#53636,
#53637,#53638,#53639,#53640,#53641,#53642,#53643),.UNSPECIFIED.,.F.,.F.)
B_SPLINE_CURVE_WITH_KNOTS((6,1,1,1,1,1,1,1,1,1,1,1,1,1,1,1,1,1,1,1,1,1,
1,1,1,1,1,1,1,1,1,1,1,1,1,1,1,1,1,1,1,1,1,1,1,1,1,1,1,1,1,1,1,1,1,1,1,1,
1,1,1,1,1,1,1,6),(0.00577184337450902,0.0153846153846154,0.0307692307692308,
0.0461538461538462,0.0615384615384615,0.0769230769230769,0.0923076923076923,
0.107692307692308,0.123076923076923,0.138461538461538,0.153846153846154,
0.169230769230769,0.184615384615385,0.2,0.215384615384615,0.230769230769231,
0.246153846153846,0.261538461538462,0.276923076923077,0.292307692307692,
0.307692307692308,0.323076923076923,0.338461538461538,0.353846153846154,
0.369230769230769,0.384615384615385,0.4,0.415384615384615,0.430769230769231,
0.446153846153846,0.461538461538462,0.476923076923077,0.492307692307692,
0.507692307692308,0.523076923076923,0.538461538461538,0.553846153846154,
0.569230769230769,0.584615384615384,0.6,0.615384615384615,0.63076923076923,
0.646153846153846,0.661538461538461,0.676923076923076,0.692307692307692,
0.707692307692307,0.723076923076922,0.738461538461538,0.753846153846153,
0.769230769230768,0.784615384615384,0.799999999999999,0.815384615384614,
0.83076923076923,0.846153846153845,0.86153846153846,0.876923076923076,0.892307692307691,
0.907692307692306,0.923076923076922,0.938461538461537,0.953846153846152,
0.969230769230768,0.984615384615383,1.),.UNSPECIFIED.)
CURVE()
GEOMETRIC_REPRESENTATION_ITEM()
RATIONAL_B_SPLINE_CURVE((1.,1.,1.,1.,1.,1.,1.,1.,1.,1.,1.,1.,1.,1.,1.,1.,
1.,1.,1.,1.,1.,1.,1.,1.,1.,1.,1.,1.,1.,1.,1.,1.,1.,1.,1.,1.,1.,1.,1.,1.,
1.,1.,1.,1.,1.,1.,1.,1.,1.,1.,1.,1.,1.,1.,1.,1.,1.,1.,1.,1.,1.,1.,1.,1.,
1.,1.,1.,1.,1.,1.))
REPRESENTATION_ITEM('')
);
#386=(
BOUNDED_CURVE()
B_SPLINE_CURVE(5,(#53647,#53648,#53649,#53650,#53651,#53652,#53653,#53654,
#53655,#53656,#53657,#53658,#53659,#53660,#53661,#53662,#53663,#53664,#53665,
#53666,#53667,#53668,#53669,#53670,#53671,#53672,#53673,#53674,#53675,#53676,
#53677,#53678,#53679,#53680,#53681,#53682,#53683,#53684,#53685,#53686,#53687,
#53688,#53689,#53690,#53691,#53692,#53693,#53694,#53695,#53696,#53697,#53698,
#53699,#53700,#53701,#53702,#53703,#53704,#53705,#53706,#53707,#53708,#53709,
#53710,#53711,#53712,#53713,#53714,#53715,#53716),.UNSPECIFIED.,.F.,.F.)
B_SPLINE_CURVE_WITH_KNOTS((6,1,1,1,1,1,1,1,1,1,1,1,1,1,1,1,1,1,1,1,1,1,
1,1,1,1,1,1,1,1,1,1,1,1,1,1,1,1,1,1,1,1,1,1,1,1,1,1,1,1,1,1,1,1,1,1,1,1,
1,1,1,1,1,1,1,6),(0.,0.0153846153846154,0.0307692307692308,0.0461538461538462,
0.0615384615384615,0.0769230769230769,0.0923076923076923,0.107692307692308,
0.123076923076923,0.138461538461538,0.153846153846154,0.169230769230769,
0.184615384615385,0.2,0.215384615384615,0.230769230769231,0.246153846153846,
0.261538461538462,0.276923076923077,0.292307692307692,0.307692307692308,
0.323076923076923,0.338461538461538,0.353846153846154,0.369230769230769,
0.384615384615385,0.4,0.415384615384615,0.430769230769231,0.446153846153846,
0.461538461538462,0.476923076923077,0.492307692307692,0.507692307692308,
0.523076923076923,0.538461538461538,0.553846153846154,0.569230769230769,
0.584615384615384,0.6,0.615384615384615,0.63076923076923,0.646153846153846,
0.661538461538461,0.676923076923076,0.692307692307692,0.707692307692307,
0.723076923076922,0.738461538461538,0.753846153846153,0.769230769230768,
0.784615384615384,0.799999999999999,0.815384615384614,0.83076923076923,
0.846153846153845,0.86153846153846,0.876923076923076,0.892307692307691,
0.907692307692306,0.923076923076922,0.938461538461537,0.953846153846152,
0.969230769230768,0.984615384615383,0.994228156739698),.UNSPECIFIED.)
CURVE()
GEOMETRIC_REPRESENTATION_ITEM()
RATIONAL_B_SPLINE_CURVE((1.,1.,1.,1.,1.,1.,1.,1.,1.,1.,1.,1.,1.,1.,1.,1.,
1.,1.,1.,1.,1.,1.,1.,1.,1.,1.,1.,1.,1.,1.,1.,1.,1.,1.,1.,1.,1.,1.,1.,1.,
1.,1.,1.,1.,1.,1.,1.,1.,1.,1.,1.,1.,1.,1.,1.,1.,1.,1.,1.,1.,1.,1.,1.,1.,
1.,1.,1.,1.,1.,1.))
REPRESENTATION_ITEM('')
);
#387=(
BOUNDED_CURVE()
B_SPLINE_CURVE(5,(#53720,#53721,#53722,#53723,#53724,#53725,#53726,#53727,
#53728,#53729,#53730,#53731,#53732,#53733,#53734,#53735,#53736,#53737,#53738,
#53739,#53740,#53741,#53742,#53743,#53744,#53745,#53746,#53747,#53748,#53749,
#53750,#53751,#53752,#53753,#53754,#53755,#53756,#53757,#53758,#53759,#53760,
#53761,#53762,#53763,#53764,#53765,#53766,#53767,#53768,#53769,#53770,#53771,
#53772,#53773,#53774,#53775,#53776,#53777,#53778,#53779,#53780,#53781,#53782,
#53783,#53784,#53785,#53786,#53787,#53788,#53789),.UNSPECIFIED.,.F.,.F.)
B_SPLINE_CURVE_WITH_KNOTS((6,1,1,1,1,1,1,1,1,1,1,1,1,1,1,1,1,1,1,1,1,1,
1,1,1,1,1,1,1,1,1,1,1,1,1,1,1,1,1,1,1,1,1,1,1,1,1,1,1,1,1,1,1,1,1,1,1,1,
1,1,1,1,1,1,1,6),(0.00577184337451611,0.0153846153846154,0.0307692307692308,
0.0461538461538462,0.0615384615384615,0.0769230769230769,0.0923076923076923,
0.107692307692308,0.123076923076923,0.138461538461538,0.153846153846154,
0.169230769230769,0.184615384615385,0.2,0.215384615384615,0.230769230769231,
0.246153846153846,0.261538461538462,0.276923076923077,0.292307692307692,
0.307692307692308,0.323076923076923,0.338461538461538,0.353846153846154,
0.369230769230769,0.384615384615385,0.4,0.415384615384615,0.430769230769231,
0.446153846153846,0.461538461538462,0.476923076923077,0.492307692307692,
0.507692307692308,0.523076923076923,0.538461538461538,0.553846153846154,
0.569230769230769,0.584615384615384,0.6,0.615384615384615,0.63076923076923,
0.646153846153846,0.661538461538461,0.676923076923076,0.692307692307692,
0.707692307692307,0.723076923076922,0.738461538461538,0.753846153846153,
0.769230769230768,0.784615384615384,0.799999999999999,0.815384615384614,
0.83076923076923,0.846153846153845,0.86153846153846,0.876923076923076,0.892307692307691,
0.907692307692306,0.923076923076922,0.938461538461537,0.953846153846152,
0.969230769230768,0.984615384615383,1.),.UNSPECIFIED.)
CURVE()
GEOMETRIC_REPRESENTATION_ITEM()
RATIONAL_B_SPLINE_CURVE((1.,1.,1.,1.,1.,1.,1.,1.,1.,1.,1.,1.,1.,1.,1.,1.,
1.,1.,1.,1.,1.,1.,1.,1.,1.,1.,1.,1.,1.,1.,1.,1.,1.,1.,1.,1.,1.,1.,1.,1.,
1.,1.,1.,1.,1.,1.,1.,1.,1.,1.,1.,1.,1.,1.,1.,1.,1.,1.,1.,1.,1.,1.,1.,1.,
1.,1.,1.,1.,1.,1.))
REPRESENTATION_ITEM('')
);
#388=(
BOUNDED_CURVE()
B_SPLINE_CURVE(5,(#53793,#53794,#53795,#53796,#53797,#53798,#53799,#53800,
#53801,#53802,#53803,#53804,#53805,#53806,#53807,#53808,#53809,#53810,#53811,
#53812,#53813,#53814,#53815,#53816,#53817,#53818,#53819,#53820,#53821,#53822,
#53823,#53824,#53825,#53826,#53827,#53828,#53829,#53830,#53831,#53832,#53833,
#53834,#53835,#53836,#53837,#53838,#53839,#53840,#53841,#53842,#53843,#53844,
#53845,#53846,#53847,#53848,#53849,#53850,#53851,#53852,#53853,#53854,#53855,
#53856,#53857,#53858,#53859,#53860,#53861,#53862),.UNSPECIFIED.,.F.,.F.)
B_SPLINE_CURVE_WITH_KNOTS((6,1,1,1,1,1,1,1,1,1,1,1,1,1,1,1,1,1,1,1,1,1,
1,1,1,1,1,1,1,1,1,1,1,1,1,1,1,1,1,1,1,1,1,1,1,1,1,1,1,1,1,1,1,1,1,1,1,1,
1,1,1,1,1,1,1,6),(0.,0.0153846153846154,0.0307692307692308,0.0461538461538462,
0.0615384615384615,0.0769230769230769,0.0923076923076923,0.107692307692308,
0.123076923076923,0.138461538461538,0.153846153846154,0.169230769230769,
0.184615384615385,0.2,0.215384615384615,0.230769230769231,0.246153846153846,
0.261538461538462,0.276923076923077,0.292307692307692,0.307692307692308,
0.323076923076923,0.338461538461538,0.353846153846154,0.369230769230769,
0.384615384615385,0.4,0.415384615384615,0.430769230769231,0.446153846153846,
0.461538461538462,0.476923076923077,0.492307692307692,0.507692307692308,
0.523076923076923,0.538461538461538,0.553846153846154,0.569230769230769,
0.584615384615384,0.6,0.615384615384615,0.63076923076923,0.646153846153846,
0.661538461538461,0.676923076923076,0.692307692307692,0.707692307692307,
0.723076923076922,0.738461538461538,0.753846153846153,0.769230769230768,
0.784615384615384,0.799999999999999,0.815384615384614,0.83076923076923,
0.846153846153845,0.86153846153846,0.876923076923076,0.892307692307691,
0.907692307692306,0.923076923076922,0.938461538461537,0.953846153846152,
0.969230769230768,0.984615384615383,0.994228156739704),.UNSPECIFIED.)
CURVE()
GEOMETRIC_REPRESENTATION_ITEM()
RATIONAL_B_SPLINE_CURVE((1.,1.,1.,1.,1.,1.,1.,1.,1.,1.,1.,1.,1.,1.,1.,1.,
1.,1.,1.,1.,1.,1.,1.,1.,1.,1.,1.,1.,1.,1.,1.,1.,1.,1.,1.,1.,1.,1.,1.,1.,
1.,1.,1.,1.,1.,1.,1.,1.,1.,1.,1.,1.,1.,1.,1.,1.,1.,1.,1.,1.,1.,1.,1.,1.,
1.,1.,1.,1.,1.,1.))
REPRESENTATION_ITEM('')
);
#389=(
BOUNDED_CURVE()
B_SPLINE_CURVE(5,(#53866,#53867,#53868,#53869,#53870,#53871,#53872,#53873,
#53874,#53875,#53876,#53877,#53878,#53879,#53880,#53881,#53882,#53883,#53884,
#53885,#53886,#53887,#53888,#53889,#53890,#53891,#53892,#53893,#53894,#53895,
#53896,#53897,#53898,#53899,#53900,#53901,#53902,#53903,#53904,#53905,#53906,
#53907,#53908,#53909,#53910,#53911,#53912,#53913,#53914,#53915,#53916,#53917,
#53918,#53919,#53920,#53921,#53922,#53923,#53924,#53925,#53926,#53927,#53928,
#53929,#53930,#53931,#53932,#53933,#53934,#53935),.UNSPECIFIED.,.F.,.F.)
B_SPLINE_CURVE_WITH_KNOTS((6,1,1,1,1,1,1,1,1,1,1,1,1,1,1,1,1,1,1,1,1,1,
1,1,1,1,1,1,1,1,1,1,1,1,1,1,1,1,1,1,1,1,1,1,1,1,1,1,1,1,1,1,1,1,1,1,1,1,
1,1,1,1,1,1,1,6),(0.00577184337449682,0.0153846153846154,0.0307692307692308,
0.0461538461538462,0.0615384615384615,0.0769230769230769,0.0923076923076923,
0.107692307692308,0.123076923076923,0.138461538461538,0.153846153846154,
0.169230769230769,0.184615384615385,0.2,0.215384615384615,0.230769230769231,
0.246153846153846,0.261538461538462,0.276923076923077,0.292307692307692,
0.307692307692308,0.323076923076923,0.338461538461538,0.353846153846154,
0.369230769230769,0.384615384615385,0.4,0.415384615384615,0.430769230769231,
0.446153846153846,0.461538461538462,0.476923076923077,0.492307692307692,
0.507692307692308,0.523076923076923,0.538461538461538,0.553846153846154,
0.569230769230769,0.584615384615384,0.6,0.615384615384615,0.63076923076923,
0.646153846153846,0.661538461538461,0.676923076923076,0.692307692307692,
0.707692307692307,0.723076923076922,0.738461538461538,0.753846153846153,
0.769230769230768,0.784615384615384,0.799999999999999,0.815384615384614,
0.83076923076923,0.846153846153845,0.86153846153846,0.876923076923076,0.892307692307691,
0.907692307692306,0.923076923076922,0.938461538461537,0.953846153846152,
0.969230769230768,0.984615384615383,1.),.UNSPECIFIED.)
CURVE()
GEOMETRIC_REPRESENTATION_ITEM()
RATIONAL_B_SPLINE_CURVE((1.,1.,1.,1.,1.,1.,1.,1.,1.,1.,1.,1.,1.,1.,1.,1.,
1.,1.,1.,1.,1.,1.,1.,1.,1.,1.,1.,1.,1.,1.,1.,1.,1.,1.,1.,1.,1.,1.,1.,1.,
1.,1.,1.,1.,1.,1.,1.,1.,1.,1.,1.,1.,1.,1.,1.,1.,1.,1.,1.,1.,1.,1.,1.,1.,
1.,1.,1.,1.,1.,1.))
REPRESENTATION_ITEM('')
);
#390=(
BOUNDED_CURVE()
B_SPLINE_CURVE(5,(#53939,#53940,#53941,#53942,#53943,#53944,#53945,#53946,
#53947,#53948,#53949,#53950,#53951,#53952,#53953,#53954,#53955,#53956,#53957,
#53958,#53959,#53960,#53961,#53962,#53963,#53964,#53965,#53966,#53967,#53968,
#53969,#53970,#53971,#53972,#53973,#53974,#53975,#53976,#53977,#53978,#53979,
#53980,#53981,#53982,#53983,#53984,#53985,#53986,#53987,#53988,#53989,#53990,
#53991,#53992,#53993,#53994,#53995,#53996,#53997,#53998,#53999,#54000,#54001,
#54002,#54003,#54004,#54005,#54006,#54007,#54008),.UNSPECIFIED.,.F.,.F.)
B_SPLINE_CURVE_WITH_KNOTS((6,1,1,1,1,1,1,1,1,1,1,1,1,1,1,1,1,1,1,1,1,1,
1,1,1,1,1,1,1,1,1,1,1,1,1,1,1,1,1,1,1,1,1,1,1,1,1,1,1,1,1,1,1,1,1,1,1,1,
1,1,1,1,1,1,1,6),(0.,0.0153846153846154,0.0307692307692308,0.0461538461538462,
0.0615384615384615,0.0769230769230769,0.0923076923076923,0.107692307692308,
0.123076923076923,0.138461538461538,0.153846153846154,0.169230769230769,
0.184615384615385,0.2,0.215384615384615,0.230769230769231,0.246153846153846,
0.261538461538462,0.276923076923077,0.292307692307692,0.307692307692308,
0.323076923076923,0.338461538461538,0.353846153846154,0.369230769230769,
0.384615384615385,0.4,0.415384615384615,0.430769230769231,0.446153846153846,
0.461538461538462,0.476923076923077,0.492307692307692,0.507692307692308,
0.523076923076923,0.538461538461538,0.553846153846154,0.569230769230769,
0.584615384615384,0.6,0.615384615384615,0.63076923076923,0.646153846153846,
0.661538461538461,0.676923076923076,0.692307692307692,0.707692307692307,
0.723076923076922,0.738461538461538,0.753846153846153,0.769230769230768,
0.784615384615384,0.799999999999999,0.815384615384614,0.83076923076923,
0.846153846153845,0.86153846153846,0.876923076923076,0.892307692307691,
0.907692307692306,0.923076923076922,0.938461538461537,0.953846153846152,
0.969230769230768,0.984615384615383,0.994228156739711),.UNSPECIFIED.)
CURVE()
GEOMETRIC_REPRESENTATION_ITEM()
RATIONAL_B_SPLINE_CURVE((1.,1.,1.,1.,1.,1.,1.,1.,1.,1.,1.,1.,1.,1.,1.,1.,
1.,1.,1.,1.,1.,1.,1.,1.,1.,1.,1.,1.,1.,1.,1.,1.,1.,1.,1.,1.,1.,1.,1.,1.,
1.,1.,1.,1.,1.,1.,1.,1.,1.,1.,1.,1.,1.,1.,1.,1.,1.,1.,1.,1.,1.,1.,1.,1.,
1.,1.,1.,1.,1.,1.))
REPRESENTATION_ITEM('')
);
#391=(
BOUNDED_CURVE()
B_SPLINE_CURVE(5,(#54012,#54013,#54014,#54015,#54016,#54017,#54018,#54019,
#54020,#54021,#54022,#54023,#54024,#54025,#54026,#54027,#54028,#54029,#54030,
#54031,#54032,#54033,#54034,#54035,#54036,#54037,#54038,#54039,#54040,#54041,
#54042,#54043,#54044,#54045,#54046,#54047,#54048,#54049,#54050,#54051,#54052,
#54053,#54054,#54055,#54056,#54057,#54058,#54059,#54060,#54061,#54062,#54063,
#54064,#54065,#54066,#54067,#54068,#54069,#54070,#54071,#54072,#54073,#54074,
#54075,#54076,#54077,#54078,#54079,#54080,#54081),.UNSPECIFIED.,.F.,.F.)
B_SPLINE_CURVE_WITH_KNOTS((6,1,1,1,1,1,1,1,1,1,1,1,1,1,1,1,1,1,1,1,1,1,
1,1,1,1,1,1,1,1,1,1,1,1,1,1,1,1,1,1,1,1,1,1,1,1,1,1,1,1,1,1,1,1,1,1,1,1,
1,1,1,1,1,1,1,6),(0.00577184337449159,0.0153846153846154,0.0307692307692308,
0.0461538461538462,0.0615384615384615,0.0769230769230769,0.0923076923076923,
0.107692307692308,0.123076923076923,0.138461538461538,0.153846153846154,
0.169230769230769,0.184615384615385,0.2,0.215384615384615,0.230769230769231,
0.246153846153846,0.261538461538462,0.276923076923077,0.292307692307692,
0.307692307692308,0.323076923076923,0.338461538461538,0.353846153846154,
0.369230769230769,0.384615384615385,0.4,0.415384615384615,0.430769230769231,
0.446153846153846,0.461538461538462,0.476923076923077,0.492307692307692,
0.507692307692308,0.523076923076923,0.538461538461538,0.553846153846154,
0.569230769230769,0.584615384615384,0.6,0.615384615384615,0.63076923076923,
0.646153846153846,0.661538461538461,0.676923076923076,0.692307692307692,
0.707692307692307,0.723076923076922,0.738461538461538,0.753846153846153,
0.769230769230768,0.784615384615384,0.799999999999999,0.815384615384614,
0.83076923076923,0.846153846153845,0.86153846153846,0.876923076923076,0.892307692307691,
0.907692307692306,0.923076923076922,0.938461538461537,0.953846153846152,
0.969230769230768,0.984615384615383,1.),.UNSPECIFIED.)
CURVE()
GEOMETRIC_REPRESENTATION_ITEM()
RATIONAL_B_SPLINE_CURVE((1.,1.,1.,1.,1.,1.,1.,1.,1.,1.,1.,1.,1.,1.,1.,1.,
1.,1.,1.,1.,1.,1.,1.,1.,1.,1.,1.,1.,1.,1.,1.,1.,1.,1.,1.,1.,1.,1.,1.,1.,
1.,1.,1.,1.,1.,1.,1.,1.,1.,1.,1.,1.,1.,1.,1.,1.,1.,1.,1.,1.,1.,1.,1.,1.,
1.,1.,1.,1.,1.,1.))
REPRESENTATION_ITEM('')
);
#392=(
BOUNDED_CURVE()
B_SPLINE_CURVE(5,(#54085,#54086,#54087,#54088,#54089,#54090,#54091,#54092,
#54093,#54094,#54095,#54096,#54097,#54098,#54099,#54100,#54101,#54102,#54103,
#54104,#54105,#54106,#54107,#54108,#54109,#54110,#54111,#54112,#54113,#54114,
#54115,#54116,#54117,#54118,#54119,#54120,#54121,#54122,#54123,#54124,#54125,
#54126,#54127,#54128,#54129,#54130,#54131,#54132,#54133,#54134,#54135,#54136,
#54137,#54138,#54139,#54140,#54141,#54142,#54143,#54144,#54145,#54146,#54147,
#54148,#54149,#54150,#54151,#54152,#54153,#54154),.UNSPECIFIED.,.F.,.F.)
B_SPLINE_CURVE_WITH_KNOTS((6,1,1,1,1,1,1,1,1,1,1,1,1,1,1,1,1,1,1,1,1,1,
1,1,1,1,1,1,1,1,1,1,1,1,1,1,1,1,1,1,1,1,1,1,1,1,1,1,1,1,1,1,1,1,1,1,1,1,
1,1,1,1,1,1,1,6),(0.,0.0153846153846154,0.0307692307692308,0.0461538461538462,
0.0615384615384615,0.0769230769230769,0.0923076923076923,0.107692307692308,
0.123076923076923,0.138461538461538,0.153846153846154,0.169230769230769,
0.184615384615385,0.2,0.215384615384615,0.230769230769231,0.246153846153846,
0.261538461538462,0.276923076923077,0.292307692307692,0.307692307692308,
0.323076923076923,0.338461538461538,0.353846153846154,0.369230769230769,
0.384615384615385,0.4,0.415384615384615,0.430769230769231,0.446153846153846,
0.461538461538462,0.476923076923077,0.492307692307692,0.507692307692308,
0.523076923076923,0.538461538461538,0.553846153846154,0.569230769230769,
0.584615384615384,0.6,0.615384615384615,0.63076923076923,0.646153846153846,
0.661538461538461,0.676923076923076,0.692307692307692,0.707692307692307,
0.723076923076922,0.738461538461538,0.753846153846153,0.769230769230768,
0.784615384615384,0.799999999999999,0.815384615384614,0.83076923076923,
0.846153846153845,0.86153846153846,0.876923076923076,0.892307692307691,
0.907692307692306,0.923076923076922,0.938461538461537,0.953846153846152,
0.969230769230768,0.984615384615383,0.994228156739723),.UNSPECIFIED.)
CURVE()
GEOMETRIC_REPRESENTATION_ITEM()
RATIONAL_B_SPLINE_CURVE((1.,1.,1.,1.,1.,1.,1.,1.,1.,1.,1.,1.,1.,1.,1.,1.,
1.,1.,1.,1.,1.,1.,1.,1.,1.,1.,1.,1.,1.,1.,1.,1.,1.,1.,1.,1.,1.,1.,1.,1.,
1.,1.,1.,1.,1.,1.,1.,1.,1.,1.,1.,1.,1.,1.,1.,1.,1.,1.,1.,1.,1.,1.,1.,1.,
1.,1.,1.,1.,1.,1.))
REPRESENTATION_ITEM('')
);
#393=(
BOUNDED_CURVE()
B_SPLINE_CURVE(5,(#54158,#54159,#54160,#54161,#54162,#54163,#54164,#54165,
#54166,#54167,#54168,#54169,#54170,#54171,#54172,#54173,#54174,#54175,#54176,
#54177,#54178,#54179,#54180,#54181,#54182,#54183,#54184,#54185,#54186,#54187,
#54188,#54189,#54190,#54191,#54192,#54193,#54194,#54195,#54196,#54197,#54198,
#54199,#54200,#54201,#54202,#54203,#54204,#54205,#54206,#54207,#54208,#54209,
#54210,#54211,#54212,#54213,#54214,#54215,#54216,#54217,#54218,#54219,#54220,
#54221,#54222,#54223,#54224,#54225,#54226,#54227),.UNSPECIFIED.,.F.,.F.)
B_SPLINE_CURVE_WITH_KNOTS((6,1,1,1,1,1,1,1,1,1,1,1,1,1,1,1,1,1,1,1,1,1,
1,1,1,1,1,1,1,1,1,1,1,1,1,1,1,1,1,1,1,1,1,1,1,1,1,1,1,1,1,1,1,1,1,1,1,1,
1,1,1,1,1,1,1,6),(0.00577184337450718,0.0153846153846154,0.0307692307692308,
0.0461538461538462,0.0615384615384615,0.0769230769230769,0.0923076923076923,
0.107692307692308,0.123076923076923,0.138461538461538,0.153846153846154,
0.169230769230769,0.184615384615385,0.2,0.215384615384615,0.230769230769231,
0.246153846153846,0.261538461538462,0.276923076923077,0.292307692307692,
0.307692307692308,0.323076923076923,0.338461538461538,0.353846153846154,
0.369230769230769,0.384615384615385,0.4,0.415384615384615,0.430769230769231,
0.446153846153846,0.461538461538462,0.476923076923077,0.492307692307692,
0.507692307692308,0.523076923076923,0.538461538461538,0.553846153846154,
0.569230769230769,0.584615384615384,0.6,0.615384615384615,0.63076923076923,
0.646153846153846,0.661538461538461,0.676923076923076,0.692307692307692,
0.707692307692307,0.723076923076922,0.738461538461538,0.753846153846153,
0.769230769230768,0.784615384615384,0.799999999999999,0.815384615384614,
0.83076923076923,0.846153846153845,0.86153846153846,0.876923076923076,0.892307692307691,
0.907692307692306,0.923076923076922,0.938461538461537,0.953846153846152,
0.969230769230768,0.984615384615383,1.),.UNSPECIFIED.)
CURVE()
GEOMETRIC_REPRESENTATION_ITEM()
RATIONAL_B_SPLINE_CURVE((1.,1.,1.,1.,1.,1.,1.,1.,1.,1.,1.,1.,1.,1.,1.,1.,
1.,1.,1.,1.,1.,1.,1.,1.,1.,1.,1.,1.,1.,1.,1.,1.,1.,1.,1.,1.,1.,1.,1.,1.,
1.,1.,1.,1.,1.,1.,1.,1.,1.,1.,1.,1.,1.,1.,1.,1.,1.,1.,1.,1.,1.,1.,1.,1.,
1.,1.,1.,1.,1.,1.))
REPRESENTATION_ITEM('')
);
#394=(
BOUNDED_CURVE()
B_SPLINE_CURVE(5,(#54231,#54232,#54233,#54234,#54235,#54236,#54237,#54238,
#54239,#54240,#54241,#54242,#54243,#54244,#54245,#54246,#54247,#54248,#54249,
#54250,#54251,#54252,#54253,#54254,#54255,#54256,#54257,#54258,#54259,#54260,
#54261,#54262,#54263,#54264,#54265,#54266,#54267,#54268,#54269,#54270,#54271,
#54272,#54273,#54274,#54275,#54276,#54277,#54278,#54279,#54280,#54281,#54282,
#54283,#54284,#54285,#54286,#54287,#54288,#54289,#54290,#54291,#54292,#54293,
#54294,#54295,#54296,#54297,#54298,#54299,#54300),.UNSPECIFIED.,.F.,.F.)
B_SPLINE_CURVE_WITH_KNOTS((6,1,1,1,1,1,1,1,1,1,1,1,1,1,1,1,1,1,1,1,1,1,
1,1,1,1,1,1,1,1,1,1,1,1,1,1,1,1,1,1,1,1,1,1,1,1,1,1,1,1,1,1,1,1,1,1,1,1,
1,1,1,1,1,1,1,6),(0.,0.0153846153846154,0.0307692307692308,0.0461538461538462,
0.0615384615384615,0.0769230769230769,0.0923076923076923,0.107692307692308,
0.123076923076923,0.138461538461538,0.153846153846154,0.169230769230769,
0.184615384615385,0.2,0.215384615384615,0.230769230769231,0.246153846153846,
0.261538461538462,0.276923076923077,0.292307692307692,0.307692307692308,
0.323076923076923,0.338461538461538,0.353846153846154,0.369230769230769,
0.384615384615385,0.4,0.415384615384615,0.430769230769231,0.446153846153846,
0.461538461538462,0.476923076923077,0.492307692307692,0.507692307692308,
0.523076923076923,0.538461538461538,0.553846153846154,0.569230769230769,
0.584615384615384,0.6,0.615384615384615,0.63076923076923,0.646153846153846,
0.661538461538461,0.676923076923076,0.692307692307692,0.707692307692307,
0.723076923076922,0.738461538461538,0.753846153846153,0.769230769230768,
0.784615384615384,0.799999999999999,0.815384615384614,0.83076923076923,
0.846153846153845,0.86153846153846,0.876923076923076,0.892307692307691,
0.907692307692306,0.923076923076922,0.938461538461537,0.953846153846152,
0.969230769230768,0.984615384615383,0.994228156739716),.UNSPECIFIED.)
CURVE()
GEOMETRIC_REPRESENTATION_ITEM()
RATIONAL_B_SPLINE_CURVE((1.,1.,1.,1.,1.,1.,1.,1.,1.,1.,1.,1.,1.,1.,1.,1.,
1.,1.,1.,1.,1.,1.,1.,1.,1.,1.,1.,1.,1.,1.,1.,1.,1.,1.,1.,1.,1.,1.,1.,1.,
1.,1.,1.,1.,1.,1.,1.,1.,1.,1.,1.,1.,1.,1.,1.,1.,1.,1.,1.,1.,1.,1.,1.,1.,
1.,1.,1.,1.,1.,1.))
REPRESENTATION_ITEM('')
);
#395=(
BOUNDED_CURVE()
B_SPLINE_CURVE(5,(#54304,#54305,#54306,#54307,#54308,#54309,#54310,#54311,
#54312,#54313,#54314,#54315,#54316,#54317,#54318,#54319,#54320,#54321,#54322,
#54323,#54324,#54325,#54326,#54327,#54328,#54329,#54330,#54331,#54332,#54333,
#54334,#54335,#54336,#54337,#54338,#54339,#54340,#54341,#54342,#54343,#54344,
#54345,#54346,#54347,#54348,#54349,#54350,#54351,#54352,#54353,#54354,#54355,
#54356,#54357,#54358,#54359,#54360,#54361,#54362,#54363,#54364,#54365,#54366,
#54367,#54368,#54369,#54370,#54371,#54372,#54373),.UNSPECIFIED.,.F.,.F.)
B_SPLINE_CURVE_WITH_KNOTS((6,1,1,1,1,1,1,1,1,1,1,1,1,1,1,1,1,1,1,1,1,1,
1,1,1,1,1,1,1,1,1,1,1,1,1,1,1,1,1,1,1,1,1,1,1,1,1,1,1,1,1,1,1,1,1,1,1,1,
1,1,1,1,1,1,1,6),(0.00577184337450174,0.0153846153846154,0.0307692307692308,
0.0461538461538462,0.0615384615384615,0.0769230769230769,0.0923076923076923,
0.107692307692308,0.123076923076923,0.138461538461538,0.153846153846154,
0.169230769230769,0.184615384615385,0.2,0.215384615384615,0.230769230769231,
0.246153846153846,0.261538461538462,0.276923076923077,0.292307692307692,
0.307692307692308,0.323076923076923,0.338461538461538,0.353846153846154,
0.369230769230769,0.384615384615385,0.4,0.415384615384615,0.430769230769231,
0.446153846153846,0.461538461538462,0.476923076923077,0.492307692307692,
0.507692307692308,0.523076923076923,0.538461538461538,0.553846153846154,
0.569230769230769,0.584615384615384,0.6,0.615384615384615,0.63076923076923,
0.646153846153846,0.661538461538461,0.676923076923076,0.692307692307692,
0.707692307692307,0.723076923076922,0.738461538461538,0.753846153846153,
0.769230769230768,0.784615384615384,0.799999999999999,0.815384615384614,
0.83076923076923,0.846153846153845,0.86153846153846,0.876923076923076,0.892307692307691,
0.907692307692306,0.923076923076922,0.938461538461537,0.953846153846152,
0.969230769230768,0.984615384615383,1.),.UNSPECIFIED.)
CURVE()
GEOMETRIC_REPRESENTATION_ITEM()
RATIONAL_B_SPLINE_CURVE((1.,1.,1.,1.,1.,1.,1.,1.,1.,1.,1.,1.,1.,1.,1.,1.,
1.,1.,1.,1.,1.,1.,1.,1.,1.,1.,1.,1.,1.,1.,1.,1.,1.,1.,1.,1.,1.,1.,1.,1.,
1.,1.,1.,1.,1.,1.,1.,1.,1.,1.,1.,1.,1.,1.,1.,1.,1.,1.,1.,1.,1.,1.,1.,1.,
1.,1.,1.,1.,1.,1.))
REPRESENTATION_ITEM('')
);
#396=(
BOUNDED_CURVE()
B_SPLINE_CURVE(5,(#54377,#54378,#54379,#54380,#54381,#54382,#54383,#54384,
#54385,#54386,#54387,#54388,#54389,#54390,#54391,#54392,#54393,#54394,#54395,
#54396,#54397,#54398,#54399,#54400,#54401,#54402,#54403,#54404,#54405,#54406,
#54407,#54408,#54409,#54410,#54411,#54412,#54413,#54414,#54415,#54416,#54417,
#54418,#54419,#54420,#54421,#54422,#54423,#54424,#54425,#54426,#54427,#54428,
#54429,#54430,#54431,#54432,#54433,#54434,#54435,#54436,#54437,#54438,#54439,
#54440,#54441,#54442,#54443,#54444,#54445,#54446),.UNSPECIFIED.,.F.,.F.)
B_SPLINE_CURVE_WITH_KNOTS((6,1,1,1,1,1,1,1,1,1,1,1,1,1,1,1,1,1,1,1,1,1,
1,1,1,1,1,1,1,1,1,1,1,1,1,1,1,1,1,1,1,1,1,1,1,1,1,1,1,1,1,1,1,1,1,1,1,1,
1,1,1,1,1,1,1,6),(0.,0.0153846153846154,0.0307692307692308,0.0461538461538462,
0.0615384615384615,0.0769230769230769,0.0923076923076923,0.107692307692308,
0.123076923076923,0.138461538461538,0.153846153846154,0.169230769230769,
0.184615384615385,0.2,0.215384615384615,0.230769230769231,0.246153846153846,
0.261538461538462,0.276923076923077,0.292307692307692,0.307692307692308,
0.323076923076923,0.338461538461538,0.353846153846154,0.369230769230769,
0.384615384615385,0.4,0.415384615384615,0.430769230769231,0.446153846153846,
0.461538461538462,0.476923076923077,0.492307692307692,0.507692307692308,
0.523076923076923,0.538461538461538,0.553846153846154,0.569230769230769,
0.584615384615384,0.6,0.615384615384615,0.63076923076923,0.646153846153846,
0.661538461538461,0.676923076923076,0.692307692307692,0.707692307692307,
0.723076923076922,0.738461538461538,0.753846153846153,0.769230769230768,
0.784615384615384,0.799999999999999,0.815384615384614,0.83076923076923,
0.846153846153845,0.86153846153846,0.876923076923076,0.892307692307691,
0.907692307692306,0.923076923076922,0.938461538461537,0.953846153846152,
0.969230769230768,0.984615384615383,0.994228156739722),.UNSPECIFIED.)
CURVE()
GEOMETRIC_REPRESENTATION_ITEM()
RATIONAL_B_SPLINE_CURVE((1.,1.,1.,1.,1.,1.,1.,1.,1.,1.,1.,1.,1.,1.,1.,1.,
1.,1.,1.,1.,1.,1.,1.,1.,1.,1.,1.,1.,1.,1.,1.,1.,1.,1.,1.,1.,1.,1.,1.,1.,
1.,1.,1.,1.,1.,1.,1.,1.,1.,1.,1.,1.,1.,1.,1.,1.,1.,1.,1.,1.,1.,1.,1.,1.,
1.,1.,1.,1.,1.,1.))
REPRESENTATION_ITEM('')
);
#397=(
BOUNDED_CURVE()
B_SPLINE_CURVE(5,(#54450,#54451,#54452,#54453,#54454,#54455,#54456,#54457,
#54458,#54459,#54460,#54461,#54462,#54463,#54464,#54465,#54466,#54467,#54468,
#54469,#54470,#54471,#54472,#54473,#54474,#54475,#54476,#54477,#54478,#54479,
#54480,#54481,#54482,#54483,#54484,#54485,#54486,#54487,#54488,#54489,#54490,
#54491,#54492,#54493,#54494,#54495,#54496,#54497,#54498,#54499,#54500,#54501,
#54502,#54503,#54504,#54505,#54506,#54507,#54508,#54509,#54510,#54511,#54512,
#54513,#54514,#54515,#54516,#54517,#54518,#54519),.UNSPECIFIED.,.F.,.F.)
B_SPLINE_CURVE_WITH_KNOTS((6,1,1,1,1,1,1,1,1,1,1,1,1,1,1,1,1,1,1,1,1,1,
1,1,1,1,1,1,1,1,1,1,1,1,1,1,1,1,1,1,1,1,1,1,1,1,1,1,1,1,1,1,1,1,1,1,1,1,
1,1,1,1,1,1,1,6),(0.00577184337450943,0.0153846153846154,0.0307692307692308,
0.0461538461538462,0.0615384615384615,0.0769230769230769,0.0923076923076923,
0.107692307692308,0.123076923076923,0.138461538461538,0.153846153846154,
0.169230769230769,0.184615384615385,0.2,0.215384615384615,0.230769230769231,
0.246153846153846,0.261538461538462,0.276923076923077,0.292307692307692,
0.307692307692308,0.323076923076923,0.338461538461538,0.353846153846154,
0.369230769230769,0.384615384615385,0.4,0.415384615384615,0.430769230769231,
0.446153846153846,0.461538461538462,0.476923076923077,0.492307692307692,
0.507692307692308,0.523076923076923,0.538461538461538,0.553846153846154,
0.569230769230769,0.584615384615384,0.6,0.615384615384615,0.63076923076923,
0.646153846153846,0.661538461538461,0.676923076923076,0.692307692307692,
0.707692307692307,0.723076923076922,0.738461538461538,0.753846153846153,
0.769230769230768,0.784615384615384,0.799999999999999,0.815384615384614,
0.83076923076923,0.846153846153845,0.86153846153846,0.876923076923076,0.892307692307691,
0.907692307692306,0.923076923076922,0.938461538461537,0.953846153846152,
0.969230769230768,0.984615384615383,1.),.UNSPECIFIED.)
CURVE()
GEOMETRIC_REPRESENTATION_ITEM()
RATIONAL_B_SPLINE_CURVE((1.,1.,1.,1.,1.,1.,1.,1.,1.,1.,1.,1.,1.,1.,1.,1.,
1.,1.,1.,1.,1.,1.,1.,1.,1.,1.,1.,1.,1.,1.,1.,1.,1.,1.,1.,1.,1.,1.,1.,1.,
1.,1.,1.,1.,1.,1.,1.,1.,1.,1.,1.,1.,1.,1.,1.,1.,1.,1.,1.,1.,1.,1.,1.,1.,
1.,1.,1.,1.,1.,1.))
REPRESENTATION_ITEM('')
);
#398=(
BOUNDED_CURVE()
B_SPLINE_CURVE(5,(#54523,#54524,#54525,#54526,#54527,#54528,#54529,#54530,
#54531,#54532,#54533,#54534,#54535,#54536,#54537,#54538,#54539,#54540,#54541,
#54542,#54543,#54544,#54545,#54546,#54547,#54548,#54549,#54550,#54551,#54552,
#54553,#54554,#54555,#54556,#54557,#54558,#54559,#54560,#54561,#54562,#54563,
#54564,#54565,#54566,#54567,#54568,#54569,#54570,#54571,#54572,#54573,#54574,
#54575,#54576,#54577,#54578,#54579,#54580,#54581,#54582,#54583,#54584,#54585,
#54586,#54587,#54588,#54589,#54590,#54591,#54592),.UNSPECIFIED.,.F.,.F.)
B_SPLINE_CURVE_WITH_KNOTS((6,1,1,1,1,1,1,1,1,1,1,1,1,1,1,1,1,1,1,1,1,1,
1,1,1,1,1,1,1,1,1,1,1,1,1,1,1,1,1,1,1,1,1,1,1,1,1,1,1,1,1,1,1,1,1,1,1,1,
1,1,1,1,1,1,1,6),(0.,0.0153846153846154,0.0307692307692308,0.0461538461538462,
0.0615384615384615,0.0769230769230769,0.0923076923076923,0.107692307692308,
0.123076923076923,0.138461538461538,0.153846153846154,0.169230769230769,
0.184615384615385,0.2,0.215384615384615,0.230769230769231,0.246153846153846,
0.261538461538462,0.276923076923077,0.292307692307692,0.307692307692308,
0.323076923076923,0.338461538461538,0.353846153846154,0.369230769230769,
0.384615384615385,0.4,0.415384615384615,0.430769230769231,0.446153846153846,
0.461538461538462,0.476923076923077,0.492307692307692,0.507692307692308,
0.523076923076923,0.538461538461538,0.553846153846154,0.569230769230769,
0.584615384615384,0.6,0.615384615384615,0.63076923076923,0.646153846153846,
0.661538461538461,0.676923076923076,0.692307692307692,0.707692307692307,
0.723076923076922,0.738461538461538,0.753846153846153,0.769230769230768,
0.784615384615384,0.799999999999999,0.815384615384614,0.83076923076923,
0.846153846153845,0.86153846153846,0.876923076923076,0.892307692307691,
0.907692307692306,0.923076923076922,0.938461538461537,0.953846153846152,
0.969230769230768,0.984615384615383,0.994228156739699),.UNSPECIFIED.)
CURVE()
GEOMETRIC_REPRESENTATION_ITEM()
RATIONAL_B_SPLINE_CURVE((1.,1.,1.,1.,1.,1.,1.,1.,1.,1.,1.,1.,1.,1.,1.,1.,
1.,1.,1.,1.,1.,1.,1.,1.,1.,1.,1.,1.,1.,1.,1.,1.,1.,1.,1.,1.,1.,1.,1.,1.,
1.,1.,1.,1.,1.,1.,1.,1.,1.,1.,1.,1.,1.,1.,1.,1.,1.,1.,1.,1.,1.,1.,1.,1.,
1.,1.,1.,1.,1.,1.))
REPRESENTATION_ITEM('')
);
#399=(
BOUNDED_CURVE()
B_SPLINE_CURVE(5,(#54596,#54597,#54598,#54599,#54600,#54601,#54602,#54603,
#54604,#54605,#54606,#54607,#54608,#54609,#54610,#54611,#54612,#54613,#54614,
#54615,#54616,#54617,#54618,#54619,#54620,#54621,#54622,#54623,#54624,#54625,
#54626,#54627,#54628,#54629,#54630,#54631,#54632,#54633,#54634,#54635,#54636,
#54637,#54638,#54639,#54640,#54641,#54642,#54643,#54644,#54645,#54646,#54647,
#54648,#54649,#54650,#54651,#54652,#54653,#54654,#54655,#54656,#54657,#54658,
#54659,#54660,#54661,#54662,#54663,#54664,#54665),.UNSPECIFIED.,.F.,.F.)
B_SPLINE_CURVE_WITH_KNOTS((6,1,1,1,1,1,1,1,1,1,1,1,1,1,1,1,1,1,1,1,1,1,
1,1,1,1,1,1,1,1,1,1,1,1,1,1,1,1,1,1,1,1,1,1,1,1,1,1,1,1,1,1,1,1,1,1,1,1,
1,1,1,1,1,1,1,6),(0.00577184337450665,0.0153846153846154,0.0307692307692308,
0.0461538461538462,0.0615384615384615,0.0769230769230769,0.0923076923076923,
0.107692307692308,0.123076923076923,0.138461538461538,0.153846153846154,
0.169230769230769,0.184615384615385,0.2,0.215384615384615,0.230769230769231,
0.246153846153846,0.261538461538462,0.276923076923077,0.292307692307692,
0.307692307692308,0.323076923076923,0.338461538461538,0.353846153846154,
0.369230769230769,0.384615384615385,0.4,0.415384615384615,0.430769230769231,
0.446153846153846,0.461538461538462,0.476923076923077,0.492307692307692,
0.507692307692308,0.523076923076923,0.538461538461538,0.553846153846154,
0.569230769230769,0.584615384615384,0.6,0.615384615384615,0.63076923076923,
0.646153846153846,0.661538461538461,0.676923076923076,0.692307692307692,
0.707692307692307,0.723076923076922,0.738461538461538,0.753846153846153,
0.769230769230768,0.784615384615384,0.799999999999999,0.815384615384614,
0.83076923076923,0.846153846153845,0.86153846153846,0.876923076923076,0.892307692307691,
0.907692307692306,0.923076923076922,0.938461538461537,0.953846153846152,
0.969230769230768,0.984615384615383,1.),.UNSPECIFIED.)
CURVE()
GEOMETRIC_REPRESENTATION_ITEM()
RATIONAL_B_SPLINE_CURVE((1.,1.,1.,1.,1.,1.,1.,1.,1.,1.,1.,1.,1.,1.,1.,1.,
1.,1.,1.,1.,1.,1.,1.,1.,1.,1.,1.,1.,1.,1.,1.,1.,1.,1.,1.,1.,1.,1.,1.,1.,
1.,1.,1.,1.,1.,1.,1.,1.,1.,1.,1.,1.,1.,1.,1.,1.,1.,1.,1.,1.,1.,1.,1.,1.,
1.,1.,1.,1.,1.,1.))
REPRESENTATION_ITEM('')
);
#400=(
BOUNDED_CURVE()
B_SPLINE_CURVE(5,(#54669,#54670,#54671,#54672,#54673,#54674,#54675,#54676,
#54677,#54678,#54679,#54680,#54681,#54682,#54683,#54684,#54685,#54686,#54687,
#54688,#54689,#54690,#54691,#54692,#54693,#54694,#54695,#54696,#54697,#54698,
#54699,#54700,#54701,#54702,#54703,#54704,#54705,#54706,#54707,#54708,#54709,
#54710,#54711,#54712,#54713,#54714,#54715,#54716,#54717,#54718,#54719,#54720,
#54721,#54722,#54723,#54724,#54725,#54726,#54727,#54728,#54729,#54730,#54731,
#54732,#54733,#54734,#54735,#54736,#54737,#54738),.UNSPECIFIED.,.F.,.F.)
B_SPLINE_CURVE_WITH_KNOTS((6,1,1,1,1,1,1,1,1,1,1,1,1,1,1,1,1,1,1,1,1,1,
1,1,1,1,1,1,1,1,1,1,1,1,1,1,1,1,1,1,1,1,1,1,1,1,1,1,1,1,1,1,1,1,1,1,1,1,
1,1,1,1,1,1,1,6),(0.,0.0153846153846154,0.0307692307692308,0.0461538461538462,
0.0615384615384615,0.0769230769230769,0.0923076923076923,0.107692307692308,
0.123076923076923,0.138461538461538,0.153846153846154,0.169230769230769,
0.184615384615385,0.2,0.215384615384615,0.230769230769231,0.246153846153846,
0.261538461538462,0.276923076923077,0.292307692307692,0.307692307692308,
0.323076923076923,0.338461538461538,0.353846153846154,0.369230769230769,
0.384615384615385,0.4,0.415384615384615,0.430769230769231,0.446153846153846,
0.461538461538462,0.476923076923077,0.492307692307692,0.507692307692308,
0.523076923076923,0.538461538461538,0.553846153846154,0.569230769230769,
0.584615384615384,0.6,0.615384615384615,0.63076923076923,0.646153846153846,
0.661538461538461,0.676923076923076,0.692307692307692,0.707692307692307,
0.723076923076922,0.738461538461538,0.753846153846153,0.769230769230768,
0.784615384615384,0.799999999999999,0.815384615384614,0.83076923076923,
0.846153846153845,0.86153846153846,0.876923076923076,0.892307692307691,
0.907692307692306,0.923076923076922,0.938461538461537,0.953846153846152,
0.969230769230768,0.984615384615383,0.994228156739691),.UNSPECIFIED.)
CURVE()
GEOMETRIC_REPRESENTATION_ITEM()
RATIONAL_B_SPLINE_CURVE((1.,1.,1.,1.,1.,1.,1.,1.,1.,1.,1.,1.,1.,1.,1.,1.,
1.,1.,1.,1.,1.,1.,1.,1.,1.,1.,1.,1.,1.,1.,1.,1.,1.,1.,1.,1.,1.,1.,1.,1.,
1.,1.,1.,1.,1.,1.,1.,1.,1.,1.,1.,1.,1.,1.,1.,1.,1.,1.,1.,1.,1.,1.,1.,1.,
1.,1.,1.,1.,1.,1.))
REPRESENTATION_ITEM('')
);
#401=(
BOUNDED_CURVE()
B_SPLINE_CURVE(5,(#54742,#54743,#54744,#54745,#54746,#54747,#54748,#54749,
#54750,#54751,#54752,#54753,#54754,#54755,#54756,#54757,#54758,#54759,#54760,
#54761,#54762,#54763,#54764,#54765,#54766,#54767,#54768,#54769,#54770,#54771,
#54772,#54773,#54774,#54775,#54776,#54777,#54778,#54779,#54780,#54781,#54782,
#54783,#54784,#54785,#54786,#54787,#54788,#54789,#54790,#54791,#54792,#54793,
#54794,#54795,#54796,#54797,#54798,#54799,#54800,#54801,#54802,#54803,#54804,
#54805,#54806,#54807,#54808,#54809,#54810,#54811),.UNSPECIFIED.,.F.,.F.)
B_SPLINE_CURVE_WITH_KNOTS((6,1,1,1,1,1,1,1,1,1,1,1,1,1,1,1,1,1,1,1,1,1,
1,1,1,1,1,1,1,1,1,1,1,1,1,1,1,1,1,1,1,1,1,1,1,1,1,1,1,1,1,1,1,1,1,1,1,1,
1,1,1,1,1,1,1,6),(0.00577184337450785,0.0153846153846154,0.0307692307692308,
0.0461538461538462,0.0615384615384615,0.0769230769230769,0.0923076923076923,
0.107692307692308,0.123076923076923,0.138461538461538,0.153846153846154,
0.169230769230769,0.184615384615385,0.2,0.215384615384615,0.230769230769231,
0.246153846153846,0.261538461538462,0.276923076923077,0.292307692307692,
0.307692307692308,0.323076923076923,0.338461538461538,0.353846153846154,
0.369230769230769,0.384615384615385,0.4,0.415384615384615,0.430769230769231,
0.446153846153846,0.461538461538462,0.476923076923077,0.492307692307692,
0.507692307692308,0.523076923076923,0.538461538461538,0.553846153846154,
0.569230769230769,0.584615384615384,0.6,0.615384615384615,0.63076923076923,
0.646153846153846,0.661538461538461,0.676923076923076,0.692307692307692,
0.707692307692307,0.723076923076922,0.738461538461538,0.753846153846153,
0.769230769230768,0.784615384615384,0.799999999999999,0.815384615384614,
0.83076923076923,0.846153846153845,0.86153846153846,0.876923076923076,0.892307692307691,
0.907692307692306,0.923076923076922,0.938461538461537,0.953846153846152,
0.969230769230768,0.984615384615383,1.),.UNSPECIFIED.)
CURVE()
GEOMETRIC_REPRESENTATION_ITEM()
RATIONAL_B_SPLINE_CURVE((1.,1.,1.,1.,1.,1.,1.,1.,1.,1.,1.,1.,1.,1.,1.,1.,
1.,1.,1.,1.,1.,1.,1.,1.,1.,1.,1.,1.,1.,1.,1.,1.,1.,1.,1.,1.,1.,1.,1.,1.,
1.,1.,1.,1.,1.,1.,1.,1.,1.,1.,1.,1.,1.,1.,1.,1.,1.,1.,1.,1.,1.,1.,1.,1.,
1.,1.,1.,1.,1.,1.))
REPRESENTATION_ITEM('')
);
#402=(
BOUNDED_CURVE()
B_SPLINE_CURVE(5,(#54815,#54816,#54817,#54818,#54819,#54820,#54821,#54822,
#54823,#54824,#54825,#54826,#54827,#54828,#54829,#54830,#54831,#54832,#54833,
#54834,#54835,#54836,#54837,#54838,#54839,#54840,#54841,#54842,#54843,#54844,
#54845,#54846,#54847,#54848,#54849,#54850,#54851,#54852,#54853,#54854,#54855,
#54856,#54857,#54858,#54859,#54860,#54861,#54862,#54863,#54864,#54865,#54866,
#54867,#54868,#54869,#54870,#54871,#54872,#54873,#54874,#54875,#54876,#54877,
#54878,#54879,#54880,#54881,#54882,#54883,#54884),.UNSPECIFIED.,.F.,.F.)
B_SPLINE_CURVE_WITH_KNOTS((6,1,1,1,1,1,1,1,1,1,1,1,1,1,1,1,1,1,1,1,1,1,
1,1,1,1,1,1,1,1,1,1,1,1,1,1,1,1,1,1,1,1,1,1,1,1,1,1,1,1,1,1,1,1,1,1,1,1,
1,1,1,1,1,1,1,6),(0.,0.0153846153846154,0.0307692307692308,0.0461538461538462,
0.0615384615384615,0.0769230769230769,0.0923076923076923,0.107692307692308,
0.123076923076923,0.138461538461538,0.153846153846154,0.169230769230769,
0.184615384615385,0.2,0.215384615384615,0.230769230769231,0.246153846153846,
0.261538461538462,0.276923076923077,0.292307692307692,0.307692307692308,
0.323076923076923,0.338461538461538,0.353846153846154,0.369230769230769,
0.384615384615385,0.4,0.415384615384615,0.430769230769231,0.446153846153846,
0.461538461538462,0.476923076923077,0.492307692307692,0.507692307692308,
0.523076923076923,0.538461538461538,0.553846153846154,0.569230769230769,
0.584615384615384,0.6,0.615384615384615,0.63076923076923,0.646153846153846,
0.661538461538461,0.676923076923076,0.692307692307692,0.707692307692307,
0.723076923076922,0.738461538461538,0.753846153846153,0.769230769230768,
0.784615384615384,0.799999999999999,0.815384615384614,0.83076923076923,
0.846153846153845,0.86153846153846,0.876923076923076,0.892307692307691,
0.907692307692306,0.923076923076922,0.938461538461537,0.953846153846152,
0.969230769230768,0.984615384615383,0.994228156739708),.UNSPECIFIED.)
CURVE()
GEOMETRIC_REPRESENTATION_ITEM()
RATIONAL_B_SPLINE_CURVE((1.,1.,1.,1.,1.,1.,1.,1.,1.,1.,1.,1.,1.,1.,1.,1.,
1.,1.,1.,1.,1.,1.,1.,1.,1.,1.,1.,1.,1.,1.,1.,1.,1.,1.,1.,1.,1.,1.,1.,1.,
1.,1.,1.,1.,1.,1.,1.,1.,1.,1.,1.,1.,1.,1.,1.,1.,1.,1.,1.,1.,1.,1.,1.,1.,
1.,1.,1.,1.,1.,1.))
REPRESENTATION_ITEM('')
);
#403=(
BOUNDED_CURVE()
B_SPLINE_CURVE(5,(#54888,#54889,#54890,#54891,#54892,#54893,#54894,#54895,
#54896,#54897,#54898,#54899,#54900,#54901,#54902,#54903,#54904,#54905,#54906,
#54907,#54908,#54909,#54910,#54911,#54912,#54913,#54914,#54915,#54916,#54917,
#54918,#54919,#54920,#54921,#54922,#54923,#54924,#54925,#54926,#54927,#54928,
#54929,#54930,#54931,#54932,#54933,#54934,#54935,#54936,#54937,#54938,#54939,
#54940,#54941,#54942,#54943,#54944,#54945,#54946,#54947,#54948,#54949,#54950,
#54951,#54952,#54953,#54954,#54955,#54956,#54957),.UNSPECIFIED.,.F.,.F.)
B_SPLINE_CURVE_WITH_KNOTS((6,1,1,1,1,1,1,1,1,1,1,1,1,1,1,1,1,1,1,1,1,1,
1,1,1,1,1,1,1,1,1,1,1,1,1,1,1,1,1,1,1,1,1,1,1,1,1,1,1,1,1,1,1,1,1,1,1,1,
1,1,1,1,1,1,1,6),(0.00577184337450072,0.0153846153846154,0.0307692307692308,
0.0461538461538462,0.0615384615384615,0.0769230769230769,0.0923076923076923,
0.107692307692308,0.123076923076923,0.138461538461538,0.153846153846154,
0.169230769230769,0.184615384615385,0.2,0.215384615384615,0.230769230769231,
0.246153846153846,0.261538461538462,0.276923076923077,0.292307692307692,
0.307692307692308,0.323076923076923,0.338461538461538,0.353846153846154,
0.369230769230769,0.384615384615385,0.4,0.415384615384615,0.430769230769231,
0.446153846153846,0.461538461538462,0.476923076923077,0.492307692307692,
0.507692307692308,0.523076923076923,0.538461538461538,0.553846153846154,
0.569230769230769,0.584615384615384,0.6,0.615384615384615,0.63076923076923,
0.646153846153846,0.661538461538461,0.676923076923076,0.692307692307692,
0.707692307692307,0.723076923076922,0.738461538461538,0.753846153846153,
0.769230769230768,0.784615384615384,0.799999999999999,0.815384615384614,
0.83076923076923,0.846153846153845,0.86153846153846,0.876923076923076,0.892307692307691,
0.907692307692306,0.923076923076922,0.938461538461537,0.953846153846152,
0.969230769230768,0.984615384615383,1.),.UNSPECIFIED.)
CURVE()
GEOMETRIC_REPRESENTATION_ITEM()
RATIONAL_B_SPLINE_CURVE((1.,1.,1.,1.,1.,1.,1.,1.,1.,1.,1.,1.,1.,1.,1.,1.,
1.,1.,1.,1.,1.,1.,1.,1.,1.,1.,1.,1.,1.,1.,1.,1.,1.,1.,1.,1.,1.,1.,1.,1.,
1.,1.,1.,1.,1.,1.,1.,1.,1.,1.,1.,1.,1.,1.,1.,1.,1.,1.,1.,1.,1.,1.,1.,1.,
1.,1.,1.,1.,1.,1.))
REPRESENTATION_ITEM('')
);
#404=(
BOUNDED_CURVE()
B_SPLINE_CURVE(5,(#54961,#54962,#54963,#54964,#54965,#54966,#54967,#54968,
#54969,#54970,#54971,#54972,#54973,#54974,#54975,#54976,#54977,#54978,#54979,
#54980,#54981,#54982,#54983,#54984,#54985,#54986,#54987,#54988,#54989,#54990,
#54991,#54992,#54993,#54994,#54995,#54996,#54997,#54998,#54999,#55000,#55001,
#55002,#55003,#55004,#55005,#55006,#55007,#55008,#55009,#55010,#55011,#55012,
#55013,#55014,#55015,#55016,#55017,#55018,#55019,#55020,#55021,#55022,#55023,
#55024,#55025,#55026,#55027,#55028,#55029,#55030),.UNSPECIFIED.,.F.,.F.)
B_SPLINE_CURVE_WITH_KNOTS((6,1,1,1,1,1,1,1,1,1,1,1,1,1,1,1,1,1,1,1,1,1,
1,1,1,1,1,1,1,1,1,1,1,1,1,1,1,1,1,1,1,1,1,1,1,1,1,1,1,1,1,1,1,1,1,1,1,1,
1,1,1,1,1,1,1,6),(0.,0.0153846153846154,0.0307692307692308,0.0461538461538462,
0.0615384615384615,0.0769230769230769,0.0923076923076923,0.107692307692308,
0.123076923076923,0.138461538461538,0.153846153846154,0.169230769230769,
0.184615384615385,0.2,0.215384615384615,0.230769230769231,0.246153846153846,
0.261538461538462,0.276923076923077,0.292307692307692,0.307692307692308,
0.323076923076923,0.338461538461538,0.353846153846154,0.369230769230769,
0.384615384615385,0.4,0.415384615384615,0.430769230769231,0.446153846153846,
0.461538461538462,0.476923076923077,0.492307692307692,0.507692307692308,
0.523076923076923,0.538461538461538,0.553846153846154,0.569230769230769,
0.584615384615384,0.6,0.615384615384615,0.63076923076923,0.646153846153846,
0.661538461538461,0.676923076923076,0.692307692307692,0.707692307692307,
0.723076923076922,0.738461538461538,0.753846153846153,0.769230769230768,
0.784615384615384,0.799999999999999,0.815384615384614,0.83076923076923,
0.846153846153845,0.86153846153846,0.876923076923076,0.892307692307691,
0.907692307692306,0.923076923076922,0.938461538461537,0.953846153846152,
0.969230769230768,0.984615384615383,0.994228156739706),.UNSPECIFIED.)
CURVE()
GEOMETRIC_REPRESENTATION_ITEM()
RATIONAL_B_SPLINE_CURVE((1.,1.,1.,1.,1.,1.,1.,1.,1.,1.,1.,1.,1.,1.,1.,1.,
1.,1.,1.,1.,1.,1.,1.,1.,1.,1.,1.,1.,1.,1.,1.,1.,1.,1.,1.,1.,1.,1.,1.,1.,
1.,1.,1.,1.,1.,1.,1.,1.,1.,1.,1.,1.,1.,1.,1.,1.,1.,1.,1.,1.,1.,1.,1.,1.,
1.,1.,1.,1.,1.,1.))
REPRESENTATION_ITEM('')
);
#405=(
BOUNDED_CURVE()
B_SPLINE_CURVE(5,(#55034,#55035,#55036,#55037,#55038,#55039,#55040,#55041,
#55042,#55043,#55044,#55045,#55046,#55047,#55048,#55049,#55050,#55051,#55052,
#55053,#55054,#55055,#55056,#55057,#55058,#55059,#55060,#55061,#55062,#55063,
#55064,#55065,#55066,#55067,#55068,#55069,#55070,#55071,#55072,#55073,#55074,
#55075,#55076,#55077,#55078,#55079,#55080,#55081,#55082,#55083,#55084,#55085,
#55086,#55087,#55088,#55089,#55090,#55091,#55092,#55093,#55094,#55095,#55096,
#55097,#55098,#55099,#55100,#55101,#55102,#55103),.UNSPECIFIED.,.F.,.F.)
B_SPLINE_CURVE_WITH_KNOTS((6,1,1,1,1,1,1,1,1,1,1,1,1,1,1,1,1,1,1,1,1,1,
1,1,1,1,1,1,1,1,1,1,1,1,1,1,1,1,1,1,1,1,1,1,1,1,1,1,1,1,1,1,1,1,1,1,1,1,
1,1,1,1,1,1,1,6),(0.00577184337450902,0.0153846153846154,0.0307692307692308,
0.0461538461538462,0.0615384615384615,0.0769230769230769,0.0923076923076923,
0.107692307692308,0.123076923076923,0.138461538461538,0.153846153846154,
0.169230769230769,0.184615384615385,0.2,0.215384615384615,0.230769230769231,
0.246153846153846,0.261538461538462,0.276923076923077,0.292307692307692,
0.307692307692308,0.323076923076923,0.338461538461538,0.353846153846154,
0.369230769230769,0.384615384615385,0.4,0.415384615384615,0.430769230769231,
0.446153846153846,0.461538461538462,0.476923076923077,0.492307692307692,
0.507692307692308,0.523076923076923,0.538461538461538,0.553846153846154,
0.569230769230769,0.584615384615384,0.6,0.615384615384615,0.63076923076923,
0.646153846153846,0.661538461538461,0.676923076923076,0.692307692307692,
0.707692307692307,0.723076923076922,0.738461538461538,0.753846153846153,
0.769230769230768,0.784615384615384,0.799999999999999,0.815384615384614,
0.83076923076923,0.846153846153845,0.86153846153846,0.876923076923076,0.892307692307691,
0.907692307692306,0.923076923076922,0.938461538461537,0.953846153846152,
0.969230769230768,0.984615384615383,1.),.UNSPECIFIED.)
CURVE()
GEOMETRIC_REPRESENTATION_ITEM()
RATIONAL_B_SPLINE_CURVE((1.,1.,1.,1.,1.,1.,1.,1.,1.,1.,1.,1.,1.,1.,1.,1.,
1.,1.,1.,1.,1.,1.,1.,1.,1.,1.,1.,1.,1.,1.,1.,1.,1.,1.,1.,1.,1.,1.,1.,1.,
1.,1.,1.,1.,1.,1.,1.,1.,1.,1.,1.,1.,1.,1.,1.,1.,1.,1.,1.,1.,1.,1.,1.,1.,
1.,1.,1.,1.,1.,1.))
REPRESENTATION_ITEM('')
);
#406=(
BOUNDED_CURVE()
B_SPLINE_CURVE(5,(#55107,#55108,#55109,#55110,#55111,#55112,#55113,#55114,
#55115,#55116,#55117,#55118,#55119,#55120,#55121,#55122,#55123,#55124,#55125,
#55126,#55127,#55128,#55129,#55130,#55131,#55132,#55133,#55134,#55135,#55136,
#55137,#55138,#55139,#55140,#55141,#55142,#55143,#55144,#55145,#55146,#55147,
#55148,#55149,#55150,#55151,#55152,#55153,#55154,#55155,#55156,#55157,#55158,
#55159,#55160,#55161,#55162,#55163,#55164,#55165,#55166,#55167,#55168,#55169,
#55170,#55171,#55172,#55173,#55174,#55175,#55176),.UNSPECIFIED.,.F.,.F.)
B_SPLINE_CURVE_WITH_KNOTS((6,1,1,1,1,1,1,1,1,1,1,1,1,1,1,1,1,1,1,1,1,1,
1,1,1,1,1,1,1,1,1,1,1,1,1,1,1,1,1,1,1,1,1,1,1,1,1,1,1,1,1,1,1,1,1,1,1,1,
1,1,1,1,1,1,1,6),(0.,0.0153846153846154,0.0307692307692308,0.0461538461538462,
0.0615384615384615,0.0769230769230769,0.0923076923076923,0.107692307692308,
0.123076923076923,0.138461538461538,0.153846153846154,0.169230769230769,
0.184615384615385,0.2,0.215384615384615,0.230769230769231,0.246153846153846,
0.261538461538462,0.276923076923077,0.292307692307692,0.307692307692308,
0.323076923076923,0.338461538461538,0.353846153846154,0.369230769230769,
0.384615384615385,0.4,0.415384615384615,0.430769230769231,0.446153846153846,
0.461538461538462,0.476923076923077,0.492307692307692,0.507692307692308,
0.523076923076923,0.538461538461538,0.553846153846154,0.569230769230769,
0.584615384615384,0.6,0.615384615384615,0.63076923076923,0.646153846153846,
0.661538461538461,0.676923076923076,0.692307692307692,0.707692307692307,
0.723076923076922,0.738461538461538,0.753846153846153,0.769230769230768,
0.784615384615384,0.799999999999999,0.815384615384614,0.83076923076923,
0.846153846153845,0.86153846153846,0.876923076923076,0.892307692307691,
0.907692307692306,0.923076923076922,0.938461538461537,0.953846153846152,
0.969230769230768,0.984615384615383,0.994228156739698),.UNSPECIFIED.)
CURVE()
GEOMETRIC_REPRESENTATION_ITEM()
RATIONAL_B_SPLINE_CURVE((1.,1.,1.,1.,1.,1.,1.,1.,1.,1.,1.,1.,1.,1.,1.,1.,
1.,1.,1.,1.,1.,1.,1.,1.,1.,1.,1.,1.,1.,1.,1.,1.,1.,1.,1.,1.,1.,1.,1.,1.,
1.,1.,1.,1.,1.,1.,1.,1.,1.,1.,1.,1.,1.,1.,1.,1.,1.,1.,1.,1.,1.,1.,1.,1.,
1.,1.,1.,1.,1.,1.))
REPRESENTATION_ITEM('')
);
#407=(
BOUNDED_CURVE()
B_SPLINE_CURVE(5,(#55180,#55181,#55182,#55183,#55184,#55185,#55186,#55187,
#55188,#55189,#55190,#55191,#55192,#55193,#55194,#55195,#55196,#55197,#55198,
#55199,#55200,#55201,#55202,#55203,#55204,#55205,#55206,#55207,#55208,#55209,
#55210,#55211,#55212,#55213,#55214,#55215,#55216,#55217,#55218,#55219,#55220,
#55221,#55222,#55223,#55224,#55225,#55226,#55227,#55228,#55229,#55230,#55231,
#55232,#55233,#55234,#55235,#55236,#55237,#55238,#55239,#55240,#55241,#55242,
#55243,#55244,#55245,#55246,#55247,#55248,#55249),.UNSPECIFIED.,.F.,.F.)
B_SPLINE_CURVE_WITH_KNOTS((6,1,1,1,1,1,1,1,1,1,1,1,1,1,1,1,1,1,1,1,1,1,
1,1,1,1,1,1,1,1,1,1,1,1,1,1,1,1,1,1,1,1,1,1,1,1,1,1,1,1,1,1,1,1,1,1,1,1,
1,1,1,1,1,1,1,6),(0.00577184337451611,0.0153846153846154,0.0307692307692308,
0.0461538461538462,0.0615384615384615,0.0769230769230769,0.0923076923076923,
0.107692307692308,0.123076923076923,0.138461538461538,0.153846153846154,
0.169230769230769,0.184615384615385,0.2,0.215384615384615,0.230769230769231,
0.246153846153846,0.261538461538462,0.276923076923077,0.292307692307692,
0.307692307692308,0.323076923076923,0.338461538461538,0.353846153846154,
0.369230769230769,0.384615384615385,0.4,0.415384615384615,0.430769230769231,
0.446153846153846,0.461538461538462,0.476923076923077,0.492307692307692,
0.507692307692308,0.523076923076923,0.538461538461538,0.553846153846154,
0.569230769230769,0.584615384615384,0.6,0.615384615384615,0.63076923076923,
0.646153846153846,0.661538461538461,0.676923076923076,0.692307692307692,
0.707692307692307,0.723076923076922,0.738461538461538,0.753846153846153,
0.769230769230768,0.784615384615384,0.799999999999999,0.815384615384614,
0.83076923076923,0.846153846153845,0.86153846153846,0.876923076923076,0.892307692307691,
0.907692307692306,0.923076923076922,0.938461538461537,0.953846153846152,
0.969230769230768,0.984615384615383,1.),.UNSPECIFIED.)
CURVE()
GEOMETRIC_REPRESENTATION_ITEM()
RATIONAL_B_SPLINE_CURVE((1.,1.,1.,1.,1.,1.,1.,1.,1.,1.,1.,1.,1.,1.,1.,1.,
1.,1.,1.,1.,1.,1.,1.,1.,1.,1.,1.,1.,1.,1.,1.,1.,1.,1.,1.,1.,1.,1.,1.,1.,
1.,1.,1.,1.,1.,1.,1.,1.,1.,1.,1.,1.,1.,1.,1.,1.,1.,1.,1.,1.,1.,1.,1.,1.,
1.,1.,1.,1.,1.,1.))
REPRESENTATION_ITEM('')
);
#408=(
BOUNDED_CURVE()
B_SPLINE_CURVE(5,(#55253,#55254,#55255,#55256,#55257,#55258,#55259,#55260,
#55261,#55262,#55263,#55264,#55265,#55266,#55267,#55268,#55269,#55270,#55271,
#55272,#55273,#55274,#55275,#55276,#55277,#55278,#55279,#55280,#55281,#55282,
#55283,#55284,#55285,#55286,#55287,#55288,#55289,#55290,#55291,#55292,#55293,
#55294,#55295,#55296,#55297,#55298,#55299,#55300,#55301,#55302,#55303,#55304,
#55305,#55306,#55307,#55308,#55309,#55310,#55311,#55312,#55313,#55314,#55315,
#55316,#55317,#55318,#55319,#55320,#55321,#55322),.UNSPECIFIED.,.F.,.F.)
B_SPLINE_CURVE_WITH_KNOTS((6,1,1,1,1,1,1,1,1,1,1,1,1,1,1,1,1,1,1,1,1,1,
1,1,1,1,1,1,1,1,1,1,1,1,1,1,1,1,1,1,1,1,1,1,1,1,1,1,1,1,1,1,1,1,1,1,1,1,
1,1,1,1,1,1,1,6),(0.,0.0153846153846154,0.0307692307692308,0.0461538461538462,
0.0615384615384615,0.0769230769230769,0.0923076923076923,0.107692307692308,
0.123076923076923,0.138461538461538,0.153846153846154,0.169230769230769,
0.184615384615385,0.2,0.215384615384615,0.230769230769231,0.246153846153846,
0.261538461538462,0.276923076923077,0.292307692307692,0.307692307692308,
0.323076923076923,0.338461538461538,0.353846153846154,0.369230769230769,
0.384615384615385,0.4,0.415384615384615,0.430769230769231,0.446153846153846,
0.461538461538462,0.476923076923077,0.492307692307692,0.507692307692308,
0.523076923076923,0.538461538461538,0.553846153846154,0.569230769230769,
0.584615384615384,0.6,0.615384615384615,0.63076923076923,0.646153846153846,
0.661538461538461,0.676923076923076,0.692307692307692,0.707692307692307,
0.723076923076922,0.738461538461538,0.753846153846153,0.769230769230768,
0.784615384615384,0.799999999999999,0.815384615384614,0.83076923076923,
0.846153846153845,0.86153846153846,0.876923076923076,0.892307692307691,
0.907692307692306,0.923076923076922,0.938461538461537,0.953846153846152,
0.969230769230768,0.984615384615383,0.994228156739704),.UNSPECIFIED.)
CURVE()
GEOMETRIC_REPRESENTATION_ITEM()
RATIONAL_B_SPLINE_CURVE((1.,1.,1.,1.,1.,1.,1.,1.,1.,1.,1.,1.,1.,1.,1.,1.,
1.,1.,1.,1.,1.,1.,1.,1.,1.,1.,1.,1.,1.,1.,1.,1.,1.,1.,1.,1.,1.,1.,1.,1.,
1.,1.,1.,1.,1.,1.,1.,1.,1.,1.,1.,1.,1.,1.,1.,1.,1.,1.,1.,1.,1.,1.,1.,1.,
1.,1.,1.,1.,1.,1.))
REPRESENTATION_ITEM('')
);
#409=(
BOUNDED_CURVE()
B_SPLINE_CURVE(5,(#55326,#55327,#55328,#55329,#55330,#55331,#55332,#55333,
#55334,#55335,#55336,#55337,#55338,#55339,#55340,#55341,#55342,#55343,#55344,
#55345,#55346,#55347,#55348,#55349,#55350,#55351,#55352,#55353,#55354,#55355,
#55356,#55357,#55358,#55359,#55360,#55361,#55362,#55363,#55364,#55365,#55366,
#55367,#55368,#55369,#55370,#55371,#55372,#55373,#55374,#55375,#55376,#55377,
#55378,#55379,#55380,#55381,#55382,#55383,#55384,#55385,#55386,#55387,#55388,
#55389,#55390,#55391,#55392,#55393,#55394,#55395),.UNSPECIFIED.,.F.,.F.)
B_SPLINE_CURVE_WITH_KNOTS((6,1,1,1,1,1,1,1,1,1,1,1,1,1,1,1,1,1,1,1,1,1,
1,1,1,1,1,1,1,1,1,1,1,1,1,1,1,1,1,1,1,1,1,1,1,1,1,1,1,1,1,1,1,1,1,1,1,1,
1,1,1,1,1,1,1,6),(0.00577184337449692,0.0153846153846154,0.0307692307692308,
0.0461538461538462,0.0615384615384615,0.0769230769230769,0.0923076923076923,
0.107692307692308,0.123076923076923,0.138461538461538,0.153846153846154,
0.169230769230769,0.184615384615385,0.2,0.215384615384615,0.230769230769231,
0.246153846153846,0.261538461538462,0.276923076923077,0.292307692307692,
0.307692307692308,0.323076923076923,0.338461538461538,0.353846153846154,
0.369230769230769,0.384615384615385,0.4,0.415384615384615,0.430769230769231,
0.446153846153846,0.461538461538462,0.476923076923077,0.492307692307692,
0.507692307692308,0.523076923076923,0.538461538461538,0.553846153846154,
0.569230769230769,0.584615384615384,0.6,0.615384615384615,0.63076923076923,
0.646153846153846,0.661538461538461,0.676923076923076,0.692307692307692,
0.707692307692307,0.723076923076922,0.738461538461538,0.753846153846153,
0.769230769230768,0.784615384615384,0.799999999999999,0.815384615384614,
0.83076923076923,0.846153846153845,0.86153846153846,0.876923076923076,0.892307692307691,
0.907692307692306,0.923076923076922,0.938461538461537,0.953846153846152,
0.969230769230768,0.984615384615383,1.),.UNSPECIFIED.)
CURVE()
GEOMETRIC_REPRESENTATION_ITEM()
RATIONAL_B_SPLINE_CURVE((1.,1.,1.,1.,1.,1.,1.,1.,1.,1.,1.,1.,1.,1.,1.,1.,
1.,1.,1.,1.,1.,1.,1.,1.,1.,1.,1.,1.,1.,1.,1.,1.,1.,1.,1.,1.,1.,1.,1.,1.,
1.,1.,1.,1.,1.,1.,1.,1.,1.,1.,1.,1.,1.,1.,1.,1.,1.,1.,1.,1.,1.,1.,1.,1.,
1.,1.,1.,1.,1.,1.))
REPRESENTATION_ITEM('')
);
#410=(
BOUNDED_CURVE()
B_SPLINE_CURVE(5,(#55398,#55399,#55400,#55401,#55402,#55403,#55404,#55405,
#55406,#55407,#55408,#55409,#55410,#55411,#55412,#55413,#55414,#55415,#55416,
#55417,#55418,#55419,#55420,#55421,#55422,#55423,#55424,#55425,#55426,#55427,
#55428,#55429,#55430,#55431,#55432,#55433,#55434,#55435,#55436,#55437,#55438,
#55439,#55440,#55441,#55442,#55443,#55444,#55445,#55446,#55447,#55448,#55449,
#55450,#55451,#55452,#55453,#55454,#55455,#55456,#55457,#55458,#55459,#55460,
#55461,#55462,#55463,#55464,#55465,#55466,#55467),.UNSPECIFIED.,.F.,.F.)
B_SPLINE_CURVE_WITH_KNOTS((6,1,1,1,1,1,1,1,1,1,1,1,1,1,1,1,1,1,1,1,1,1,
1,1,1,1,1,1,1,1,1,1,1,1,1,1,1,1,1,1,1,1,1,1,1,1,1,1,1,1,1,1,1,1,1,1,1,1,
1,1,1,1,1,1,1,6),(0.,0.0153846153846154,0.0307692307692308,0.0461538461538462,
0.0615384615384615,0.0769230769230769,0.0923076923076923,0.107692307692308,
0.123076923076923,0.138461538461538,0.153846153846154,0.169230769230769,
0.184615384615385,0.2,0.215384615384615,0.230769230769231,0.246153846153846,
0.261538461538462,0.276923076923077,0.292307692307692,0.307692307692308,
0.323076923076923,0.338461538461538,0.353846153846154,0.369230769230769,
0.384615384615385,0.4,0.415384615384615,0.430769230769231,0.446153846153846,
0.461538461538462,0.476923076923077,0.492307692307692,0.507692307692308,
0.523076923076923,0.538461538461538,0.553846153846154,0.569230769230769,
0.584615384615384,0.6,0.615384615384615,0.63076923076923,0.646153846153846,
0.661538461538461,0.676923076923076,0.692307692307692,0.707692307692307,
0.723076923076922,0.738461538461538,0.753846153846153,0.769230769230768,
0.784615384615384,0.799999999999999,0.815384615384614,0.83076923076923,
0.846153846153845,0.86153846153846,0.876923076923076,0.892307692307691,
0.907692307692306,0.923076923076922,0.938461538461537,0.953846153846152,
0.969230769230768,0.984615384615383,0.994228156739723),.UNSPECIFIED.)
CURVE()
GEOMETRIC_REPRESENTATION_ITEM()
RATIONAL_B_SPLINE_CURVE((1.,1.,1.,1.,1.,1.,1.,1.,1.,1.,1.,1.,1.,1.,1.,1.,
1.,1.,1.,1.,1.,1.,1.,1.,1.,1.,1.,1.,1.,1.,1.,1.,1.,1.,1.,1.,1.,1.,1.,1.,
1.,1.,1.,1.,1.,1.,1.,1.,1.,1.,1.,1.,1.,1.,1.,1.,1.,1.,1.,1.,1.,1.,1.,1.,
1.,1.,1.,1.,1.,1.))
REPRESENTATION_ITEM('')
);
#411=(
BOUNDED_CURVE()
B_SPLINE_CURVE(5,(#55626,#55627,#55628,#55629,#55630,#55631,#55632,#55633,
#55634,#55635,#55636,#55637,#55638,#55639,#55640,#55641,#55642,#55643,#55644,
#55645,#55646,#55647,#55648,#55649,#55650,#55651,#55652,#55653,#55654,#55655,
#55656,#55657,#55658,#55659,#55660,#55661,#55662,#55663,#55664,#55665,#55666,
#55667,#55668,#55669,#55670,#55671,#55672,#55673,#55674,#55675,#55676,#55677,
#55678,#55679,#55680,#55681,#55682,#55683,#55684,#55685,#55686,#55687,#55688,
#55689,#55690,#55691,#55692,#55693,#55694,#55695),.UNSPECIFIED.,.F.,.F.)
B_SPLINE_CURVE_WITH_KNOTS((6,1,1,1,1,1,1,1,1,1,1,1,1,1,1,1,1,1,1,1,1,1,
1,1,1,1,1,1,1,1,1,1,1,1,1,1,1,1,1,1,1,1,1,1,1,1,1,1,1,1,1,1,1,1,1,1,1,1,
1,1,1,1,1,1,1,6),(-1.,-0.984615384615383,-0.969230769230768,-0.953846153846152,
-0.938461538461537,-0.923076923076922,-0.907692307692306,-0.892307692307691,
-0.876923076923076,-0.86153846153846,-0.846153846153845,-0.83076923076923,
-0.815384615384614,-0.799999999999999,-0.784615384615384,-0.769230769230768,
-0.753846153846153,-0.738461538461538,-0.723076923076922,-0.707692307692307,
-0.692307692307692,-0.676923076923076,-0.661538461538461,-0.646153846153846,
-0.63076923076923,-0.615384615384615,-0.6,-0.584615384615384,-0.569230769230769,
-0.553846153846154,-0.538461538461538,-0.523076923076923,-0.507692307692308,
-0.492307692307692,-0.476923076923077,-0.461538461538462,-0.446153846153846,
-0.430769230769231,-0.415384615384615,-0.4,-0.384615384615385,-0.369230769230769,
-0.353846153846154,-0.338461538461538,-0.323076923076923,-0.307692307692308,
-0.292307692307692,-0.276923076923077,-0.261538461538462,-0.246153846153846,
-0.230769230769231,-0.215384615384615,-0.2,-0.184615384615385,-0.169230769230769,
-0.153846153846154,-0.138461538461538,-0.123076923076923,-0.107692307692308,
-0.0923076923076923,-0.0769230769230769,-0.0615384615384615,-0.0461538461538462,
-0.0307692307692308,-0.0153846153846154,-0.00577184337448906),
 .UNSPECIFIED.)
CURVE()
GEOMETRIC_REPRESENTATION_ITEM()
RATIONAL_B_SPLINE_CURVE((1.,1.,1.,1.,1.,1.,1.,1.,1.,1.,1.,1.,1.,1.,1.,1.,
1.,1.,1.,1.,1.,1.,1.,1.,1.,1.,1.,1.,1.,1.,1.,1.,1.,1.,1.,1.,1.,1.,1.,1.,
1.,1.,1.,1.,1.,1.,1.,1.,1.,1.,1.,1.,1.,1.,1.,1.,1.,1.,1.,1.,1.,1.,1.,1.,
1.,1.,1.,1.,1.,1.))
REPRESENTATION_ITEM('')
);
#412=(
BOUNDED_CURVE()
B_SPLINE_CURVE(5,(#55846,#55847,#55848,#55849,#55850,#55851,#55852,#55853,
#55854,#55855,#55856,#55857,#55858,#55859,#55860,#55861,#55862,#55863,#55864,
#55865,#55866,#55867,#55868,#55869,#55870,#55871,#55872,#55873,#55874,#55875,
#55876,#55877,#55878,#55879,#55880,#55881,#55882,#55883,#55884,#55885,#55886,
#55887,#55888,#55889,#55890,#55891,#55892,#55893,#55894,#55895,#55896,#55897,
#55898,#55899,#55900,#55901,#55902,#55903,#55904,#55905,#55906,#55907,#55908,
#55909,#55910,#55911,#55912,#55913,#55914,#55915),.UNSPECIFIED.,.F.,.F.)
B_SPLINE_CURVE_WITH_KNOTS((6,1,1,1,1,1,1,1,1,1,1,1,1,1,1,1,1,1,1,1,1,1,
1,1,1,1,1,1,1,1,1,1,1,1,1,1,1,1,1,1,1,1,1,1,1,1,1,1,1,1,1,1,1,1,1,1,1,1,
1,1,1,1,1,1,1,6),(-0.994228156739728,-0.984615384615383,-0.969230769230768,
-0.953846153846152,-0.938461538461537,-0.923076923076922,-0.907692307692306,
-0.892307692307691,-0.876923076923076,-0.86153846153846,-0.846153846153845,
-0.83076923076923,-0.815384615384614,-0.799999999999999,-0.784615384615384,
-0.769230769230768,-0.753846153846153,-0.738461538461538,-0.723076923076922,
-0.707692307692307,-0.692307692307692,-0.676923076923076,-0.661538461538461,
-0.646153846153846,-0.63076923076923,-0.615384615384615,-0.6,-0.584615384615384,
-0.569230769230769,-0.553846153846154,-0.538461538461538,-0.523076923076923,
-0.507692307692308,-0.492307692307692,-0.476923076923077,-0.461538461538462,
-0.446153846153846,-0.430769230769231,-0.415384615384615,-0.4,-0.384615384615385,
-0.369230769230769,-0.353846153846154,-0.338461538461538,-0.323076923076923,
-0.307692307692308,-0.292307692307692,-0.276923076923077,-0.261538461538462,
-0.246153846153846,-0.230769230769231,-0.215384615384615,-0.2,-0.184615384615385,
-0.169230769230769,-0.153846153846154,-0.138461538461538,-0.123076923076923,
-0.107692307692308,-0.0923076923076923,-0.0769230769230769,-0.0615384615384615,
-0.0461538461538462,-0.0307692307692308,-0.0153846153846154,0.),
 .UNSPECIFIED.)
CURVE()
GEOMETRIC_REPRESENTATION_ITEM()
RATIONAL_B_SPLINE_CURVE((1.,1.,1.,1.,1.,1.,1.,1.,1.,1.,1.,1.,1.,1.,1.,1.,
1.,1.,1.,1.,1.,1.,1.,1.,1.,1.,1.,1.,1.,1.,1.,1.,1.,1.,1.,1.,1.,1.,1.,1.,
1.,1.,1.,1.,1.,1.,1.,1.,1.,1.,1.,1.,1.,1.,1.,1.,1.,1.,1.,1.,1.,1.,1.,1.,
1.,1.,1.,1.,1.,1.))
REPRESENTATION_ITEM('')
);
#413=(
BOUNDED_CURVE()
B_SPLINE_CURVE(5,(#56068,#56069,#56070,#56071,#56072,#56073,#56074,#56075,
#56076,#56077,#56078,#56079,#56080,#56081,#56082,#56083,#56084,#56085,#56086,
#56087,#56088,#56089,#56090,#56091,#56092,#56093,#56094,#56095,#56096,#56097,
#56098,#56099,#56100,#56101,#56102,#56103,#56104,#56105,#56106,#56107,#56108,
#56109,#56110,#56111,#56112,#56113,#56114,#56115,#56116,#56117,#56118,#56119,
#56120,#56121,#56122,#56123,#56124,#56125,#56126,#56127,#56128,#56129,#56130,
#56131,#56132,#56133,#56134,#56135,#56136,#56137),.UNSPECIFIED.,.F.,.F.)
B_SPLINE_CURVE_WITH_KNOTS((6,1,1,1,1,1,1,1,1,1,1,1,1,1,1,1,1,1,1,1,1,1,
1,1,1,1,1,1,1,1,1,1,1,1,1,1,1,1,1,1,1,1,1,1,1,1,1,1,1,1,1,1,1,1,1,1,1,1,
1,1,1,1,1,1,1,6),(-1.,-0.984615384615383,-0.969230769230768,-0.953846153846152,
-0.938461538461537,-0.923076923076922,-0.907692307692306,-0.892307692307691,
-0.876923076923076,-0.86153846153846,-0.846153846153845,-0.83076923076923,
-0.815384615384614,-0.799999999999999,-0.784615384615384,-0.769230769230768,
-0.753846153846153,-0.738461538461538,-0.723076923076922,-0.707692307692307,
-0.692307692307692,-0.676923076923076,-0.661538461538461,-0.646153846153846,
-0.63076923076923,-0.615384615384615,-0.6,-0.584615384615384,-0.569230769230769,
-0.553846153846154,-0.538461538461538,-0.523076923076923,-0.507692307692308,
-0.492307692307692,-0.476923076923077,-0.461538461538462,-0.446153846153846,
-0.430769230769231,-0.415384615384615,-0.4,-0.384615384615385,-0.369230769230769,
-0.353846153846154,-0.338461538461538,-0.323076923076923,-0.307692307692308,
-0.292307692307692,-0.276923076923077,-0.261538461538462,-0.246153846153846,
-0.230769230769231,-0.215384615384615,-0.2,-0.184615384615385,-0.169230769230769,
-0.153846153846154,-0.138461538461538,-0.123076923076923,-0.107692307692308,
-0.0923076923076923,-0.0769230769230769,-0.0615384615384615,-0.0461538461538462,
-0.0307692307692308,-0.0153846153846154,-0.0057718433744926),
 .UNSPECIFIED.)
CURVE()
GEOMETRIC_REPRESENTATION_ITEM()
RATIONAL_B_SPLINE_CURVE((1.,1.,1.,1.,1.,1.,1.,1.,1.,1.,1.,1.,1.,1.,1.,1.,
1.,1.,1.,1.,1.,1.,1.,1.,1.,1.,1.,1.,1.,1.,1.,1.,1.,1.,1.,1.,1.,1.,1.,1.,
1.,1.,1.,1.,1.,1.,1.,1.,1.,1.,1.,1.,1.,1.,1.,1.,1.,1.,1.,1.,1.,1.,1.,1.,
1.,1.,1.,1.,1.,1.))
REPRESENTATION_ITEM('')
);
#414=(
BOUNDED_CURVE()
B_SPLINE_CURVE(5,(#56288,#56289,#56290,#56291,#56292,#56293,#56294,#56295,
#56296,#56297,#56298,#56299,#56300,#56301,#56302,#56303,#56304,#56305,#56306,
#56307,#56308,#56309,#56310,#56311,#56312,#56313,#56314,#56315,#56316,#56317,
#56318,#56319,#56320,#56321,#56322,#56323,#56324,#56325,#56326,#56327,#56328,
#56329,#56330,#56331,#56332,#56333,#56334,#56335,#56336,#56337,#56338,#56339,
#56340,#56341,#56342,#56343,#56344,#56345,#56346,#56347,#56348,#56349,#56350,
#56351,#56352,#56353,#56354,#56355,#56356,#56357),.UNSPECIFIED.,.F.,.F.)
B_SPLINE_CURVE_WITH_KNOTS((6,1,1,1,1,1,1,1,1,1,1,1,1,1,1,1,1,1,1,1,1,1,
1,1,1,1,1,1,1,1,1,1,1,1,1,1,1,1,1,1,1,1,1,1,1,1,1,1,1,1,1,1,1,1,1,1,1,1,
1,1,1,1,1,1,1,6),(-0.994228156739718,-0.984615384615383,-0.969230769230768,
-0.953846153846152,-0.938461538461537,-0.923076923076922,-0.907692307692306,
-0.892307692307691,-0.876923076923076,-0.86153846153846,-0.846153846153845,
-0.83076923076923,-0.815384615384614,-0.799999999999999,-0.784615384615384,
-0.769230769230768,-0.753846153846153,-0.738461538461538,-0.723076923076922,
-0.707692307692307,-0.692307692307692,-0.676923076923076,-0.661538461538461,
-0.646153846153846,-0.63076923076923,-0.615384615384615,-0.6,-0.584615384615384,
-0.569230769230769,-0.553846153846154,-0.538461538461538,-0.523076923076923,
-0.507692307692308,-0.492307692307692,-0.476923076923077,-0.461538461538462,
-0.446153846153846,-0.430769230769231,-0.415384615384615,-0.4,-0.384615384615385,
-0.369230769230769,-0.353846153846154,-0.338461538461538,-0.323076923076923,
-0.307692307692308,-0.292307692307692,-0.276923076923077,-0.261538461538462,
-0.246153846153846,-0.230769230769231,-0.215384615384615,-0.2,-0.184615384615385,
-0.169230769230769,-0.153846153846154,-0.138461538461538,-0.123076923076923,
-0.107692307692308,-0.0923076923076923,-0.0769230769230769,-0.0615384615384615,
-0.0461538461538462,-0.0307692307692308,-0.0153846153846154,0.),
 .UNSPECIFIED.)
CURVE()
GEOMETRIC_REPRESENTATION_ITEM()
RATIONAL_B_SPLINE_CURVE((1.,1.,1.,1.,1.,1.,1.,1.,1.,1.,1.,1.,1.,1.,1.,1.,
1.,1.,1.,1.,1.,1.,1.,1.,1.,1.,1.,1.,1.,1.,1.,1.,1.,1.,1.,1.,1.,1.,1.,1.,
1.,1.,1.,1.,1.,1.,1.,1.,1.,1.,1.,1.,1.,1.,1.,1.,1.,1.,1.,1.,1.,1.,1.,1.,
1.,1.,1.,1.,1.,1.))
REPRESENTATION_ITEM('')
);
#415=(
BOUNDED_CURVE()
B_SPLINE_CURVE(5,(#56510,#56511,#56512,#56513,#56514,#56515,#56516,#56517,
#56518,#56519,#56520,#56521,#56522,#56523,#56524,#56525,#56526,#56527,#56528,
#56529,#56530,#56531,#56532,#56533,#56534,#56535,#56536,#56537,#56538,#56539,
#56540,#56541,#56542,#56543,#56544,#56545,#56546,#56547,#56548,#56549,#56550,
#56551,#56552,#56553,#56554,#56555,#56556,#56557,#56558,#56559,#56560,#56561,
#56562,#56563,#56564,#56565,#56566,#56567,#56568,#56569,#56570,#56571,#56572,
#56573,#56574,#56575,#56576,#56577,#56578,#56579),.UNSPECIFIED.,.F.,.F.)
B_SPLINE_CURVE_WITH_KNOTS((6,1,1,1,1,1,1,1,1,1,1,1,1,1,1,1,1,1,1,1,1,1,
1,1,1,1,1,1,1,1,1,1,1,1,1,1,1,1,1,1,1,1,1,1,1,1,1,1,1,1,1,1,1,1,1,1,1,1,
1,1,1,1,1,1,1,6),(-1.,-0.984615384615383,-0.969230769230768,-0.953846153846152,
-0.938461538461537,-0.923076923076922,-0.907692307692306,-0.892307692307691,
-0.876923076923076,-0.86153846153846,-0.846153846153845,-0.83076923076923,
-0.815384615384614,-0.799999999999999,-0.784615384615384,-0.769230769230768,
-0.753846153846153,-0.738461538461538,-0.723076923076922,-0.707692307692307,
-0.692307692307692,-0.676923076923076,-0.661538461538461,-0.646153846153846,
-0.63076923076923,-0.615384615384615,-0.6,-0.584615384615384,-0.569230769230769,
-0.553846153846154,-0.538461538461538,-0.523076923076923,-0.507692307692308,
-0.492307692307692,-0.476923076923077,-0.461538461538462,-0.446153846153846,
-0.430769230769231,-0.415384615384615,-0.4,-0.384615384615385,-0.369230769230769,
-0.353846153846154,-0.338461538461538,-0.323076923076923,-0.307692307692308,
-0.292307692307692,-0.276923076923077,-0.261538461538462,-0.246153846153846,
-0.230769230769231,-0.215384615384615,-0.2,-0.184615384615385,-0.169230769230769,
-0.153846153846154,-0.138461538461538,-0.123076923076923,-0.107692307692308,
-0.0923076923076923,-0.0769230769230769,-0.0615384615384615,-0.0461538461538462,
-0.0307692307692308,-0.0153846153846154,-0.00577184337449396),
 .UNSPECIFIED.)
CURVE()
GEOMETRIC_REPRESENTATION_ITEM()
RATIONAL_B_SPLINE_CURVE((1.,1.,1.,1.,1.,1.,1.,1.,1.,1.,1.,1.,1.,1.,1.,1.,
1.,1.,1.,1.,1.,1.,1.,1.,1.,1.,1.,1.,1.,1.,1.,1.,1.,1.,1.,1.,1.,1.,1.,1.,
1.,1.,1.,1.,1.,1.,1.,1.,1.,1.,1.,1.,1.,1.,1.,1.,1.,1.,1.,1.,1.,1.,1.,1.,
1.,1.,1.,1.,1.,1.))
REPRESENTATION_ITEM('')
);
#416=(
BOUNDED_CURVE()
B_SPLINE_CURVE(5,(#56730,#56731,#56732,#56733,#56734,#56735,#56736,#56737,
#56738,#56739,#56740,#56741,#56742,#56743,#56744,#56745,#56746,#56747,#56748,
#56749,#56750,#56751,#56752,#56753,#56754,#56755,#56756,#56757,#56758,#56759,
#56760,#56761,#56762,#56763,#56764,#56765,#56766,#56767,#56768,#56769,#56770,
#56771,#56772,#56773,#56774,#56775,#56776,#56777,#56778,#56779,#56780,#56781,
#56782,#56783,#56784,#56785,#56786,#56787,#56788,#56789,#56790,#56791,#56792,
#56793,#56794,#56795,#56796,#56797,#56798,#56799),.UNSPECIFIED.,.F.,.F.)
B_SPLINE_CURVE_WITH_KNOTS((6,1,1,1,1,1,1,1,1,1,1,1,1,1,1,1,1,1,1,1,1,1,
1,1,1,1,1,1,1,1,1,1,1,1,1,1,1,1,1,1,1,1,1,1,1,1,1,1,1,1,1,1,1,1,1,1,1,1,
1,1,1,1,1,1,1,6),(-0.994228156739702,-0.984615384615383,-0.969230769230768,
-0.953846153846152,-0.938461538461537,-0.923076923076922,-0.907692307692306,
-0.892307692307691,-0.876923076923076,-0.86153846153846,-0.846153846153845,
-0.83076923076923,-0.815384615384614,-0.799999999999999,-0.784615384615384,
-0.769230769230768,-0.753846153846153,-0.738461538461538,-0.723076923076922,
-0.707692307692307,-0.692307692307692,-0.676923076923076,-0.661538461538461,
-0.646153846153846,-0.63076923076923,-0.615384615384615,-0.6,-0.584615384615384,
-0.569230769230769,-0.553846153846154,-0.538461538461538,-0.523076923076923,
-0.507692307692308,-0.492307692307692,-0.476923076923077,-0.461538461538462,
-0.446153846153846,-0.430769230769231,-0.415384615384615,-0.4,-0.384615384615385,
-0.369230769230769,-0.353846153846154,-0.338461538461538,-0.323076923076923,
-0.307692307692308,-0.292307692307692,-0.276923076923077,-0.261538461538462,
-0.246153846153846,-0.230769230769231,-0.215384615384615,-0.2,-0.184615384615385,
-0.169230769230769,-0.153846153846154,-0.138461538461538,-0.123076923076923,
-0.107692307692308,-0.0923076923076923,-0.0769230769230769,-0.0615384615384615,
-0.0461538461538462,-0.0307692307692308,-0.0153846153846154,0.),
 .UNSPECIFIED.)
CURVE()
GEOMETRIC_REPRESENTATION_ITEM()
RATIONAL_B_SPLINE_CURVE((1.,1.,1.,1.,1.,1.,1.,1.,1.,1.,1.,1.,1.,1.,1.,1.,
1.,1.,1.,1.,1.,1.,1.,1.,1.,1.,1.,1.,1.,1.,1.,1.,1.,1.,1.,1.,1.,1.,1.,1.,
1.,1.,1.,1.,1.,1.,1.,1.,1.,1.,1.,1.,1.,1.,1.,1.,1.,1.,1.,1.,1.,1.,1.,1.,
1.,1.,1.,1.,1.,1.))
REPRESENTATION_ITEM('')
);
#417=(
BOUNDED_CURVE()
B_SPLINE_CURVE(5,(#56952,#56953,#56954,#56955,#56956,#56957,#56958,#56959,
#56960,#56961,#56962,#56963,#56964,#56965,#56966,#56967,#56968,#56969,#56970,
#56971,#56972,#56973,#56974,#56975,#56976,#56977,#56978,#56979,#56980,#56981,
#56982,#56983,#56984,#56985,#56986,#56987,#56988,#56989,#56990,#56991,#56992,
#56993,#56994,#56995,#56996,#56997,#56998,#56999,#57000,#57001,#57002,#57003,
#57004,#57005,#57006,#57007,#57008,#57009,#57010,#57011,#57012,#57013,#57014,
#57015,#57016,#57017,#57018,#57019,#57020,#57021),.UNSPECIFIED.,.F.,.F.)
B_SPLINE_CURVE_WITH_KNOTS((6,1,1,1,1,1,1,1,1,1,1,1,1,1,1,1,1,1,1,1,1,1,
1,1,1,1,1,1,1,1,1,1,1,1,1,1,1,1,1,1,1,1,1,1,1,1,1,1,1,1,1,1,1,1,1,1,1,1,
1,1,1,1,1,1,1,6),(-1.,-0.984615384615383,-0.969230769230768,-0.953846153846152,
-0.938461538461537,-0.923076923076922,-0.907692307692306,-0.892307692307691,
-0.876923076923076,-0.86153846153846,-0.846153846153845,-0.83076923076923,
-0.815384615384614,-0.799999999999999,-0.784615384615384,-0.769230769230768,
-0.753846153846153,-0.738461538461538,-0.723076923076922,-0.707692307692307,
-0.692307692307692,-0.676923076923076,-0.661538461538461,-0.646153846153846,
-0.63076923076923,-0.615384615384615,-0.6,-0.584615384615384,-0.569230769230769,
-0.553846153846154,-0.538461538461538,-0.523076923076923,-0.507692307692308,
-0.492307692307692,-0.476923076923077,-0.461538461538462,-0.446153846153846,
-0.430769230769231,-0.415384615384615,-0.4,-0.384615384615385,-0.369230769230769,
-0.353846153846154,-0.338461538461538,-0.323076923076923,-0.307692307692308,
-0.292307692307692,-0.276923076923077,-0.261538461538462,-0.246153846153846,
-0.230769230769231,-0.215384615384615,-0.2,-0.184615384615385,-0.169230769230769,
-0.153846153846154,-0.138461538461538,-0.123076923076923,-0.107692307692308,
-0.0923076923076923,-0.0769230769230769,-0.0615384615384615,-0.0461538461538462,
-0.0307692307692308,-0.0153846153846154,-0.00577184337450989),
 .UNSPECIFIED.)
CURVE()
GEOMETRIC_REPRESENTATION_ITEM()
RATIONAL_B_SPLINE_CURVE((1.,1.,1.,1.,1.,1.,1.,1.,1.,1.,1.,1.,1.,1.,1.,1.,
1.,1.,1.,1.,1.,1.,1.,1.,1.,1.,1.,1.,1.,1.,1.,1.,1.,1.,1.,1.,1.,1.,1.,1.,
1.,1.,1.,1.,1.,1.,1.,1.,1.,1.,1.,1.,1.,1.,1.,1.,1.,1.,1.,1.,1.,1.,1.,1.,
1.,1.,1.,1.,1.,1.))
REPRESENTATION_ITEM('')
);
#418=(
BOUNDED_CURVE()
B_SPLINE_CURVE(5,(#57172,#57173,#57174,#57175,#57176,#57177,#57178,#57179,
#57180,#57181,#57182,#57183,#57184,#57185,#57186,#57187,#57188,#57189,#57190,
#57191,#57192,#57193,#57194,#57195,#57196,#57197,#57198,#57199,#57200,#57201,
#57202,#57203,#57204,#57205,#57206,#57207,#57208,#57209,#57210,#57211,#57212,
#57213,#57214,#57215,#57216,#57217,#57218,#57219,#57220,#57221,#57222,#57223,
#57224,#57225,#57226,#57227,#57228,#57229,#57230,#57231,#57232,#57233,#57234,
#57235,#57236,#57237,#57238,#57239,#57240,#57241),.UNSPECIFIED.,.F.,.F.)
B_SPLINE_CURVE_WITH_KNOTS((6,1,1,1,1,1,1,1,1,1,1,1,1,1,1,1,1,1,1,1,1,1,
1,1,1,1,1,1,1,1,1,1,1,1,1,1,1,1,1,1,1,1,1,1,1,1,1,1,1,1,1,1,1,1,1,1,1,1,
1,1,1,1,1,1,1,6),(-0.994228156739736,-0.984615384615383,-0.969230769230768,
-0.953846153846152,-0.938461538461537,-0.923076923076922,-0.907692307692306,
-0.892307692307691,-0.876923076923076,-0.86153846153846,-0.846153846153845,
-0.83076923076923,-0.815384615384614,-0.799999999999999,-0.784615384615384,
-0.769230769230768,-0.753846153846153,-0.738461538461538,-0.723076923076922,
-0.707692307692307,-0.692307692307692,-0.676923076923076,-0.661538461538461,
-0.646153846153846,-0.63076923076923,-0.615384615384615,-0.6,-0.584615384615384,
-0.569230769230769,-0.553846153846154,-0.538461538461538,-0.523076923076923,
-0.507692307692308,-0.492307692307692,-0.476923076923077,-0.461538461538462,
-0.446153846153846,-0.430769230769231,-0.415384615384615,-0.4,-0.384615384615385,
-0.369230769230769,-0.353846153846154,-0.338461538461538,-0.323076923076923,
-0.307692307692308,-0.292307692307692,-0.276923076923077,-0.261538461538462,
-0.246153846153846,-0.230769230769231,-0.215384615384615,-0.2,-0.184615384615385,
-0.169230769230769,-0.153846153846154,-0.138461538461538,-0.123076923076923,
-0.107692307692308,-0.0923076923076923,-0.0769230769230769,-0.0615384615384615,
-0.0461538461538462,-0.0307692307692308,-0.0153846153846154,0.),
 .UNSPECIFIED.)
CURVE()
GEOMETRIC_REPRESENTATION_ITEM()
RATIONAL_B_SPLINE_CURVE((1.,1.,1.,1.,1.,1.,1.,1.,1.,1.,1.,1.,1.,1.,1.,1.,
1.,1.,1.,1.,1.,1.,1.,1.,1.,1.,1.,1.,1.,1.,1.,1.,1.,1.,1.,1.,1.,1.,1.,1.,
1.,1.,1.,1.,1.,1.,1.,1.,1.,1.,1.,1.,1.,1.,1.,1.,1.,1.,1.,1.,1.,1.,1.,1.,
1.,1.,1.,1.,1.,1.))
REPRESENTATION_ITEM('')
);
#419=(
BOUNDED_CURVE()
B_SPLINE_CURVE(5,(#57394,#57395,#57396,#57397,#57398,#57399,#57400,#57401,
#57402,#57403,#57404,#57405,#57406,#57407,#57408,#57409,#57410,#57411,#57412,
#57413,#57414,#57415,#57416,#57417,#57418,#57419,#57420,#57421,#57422,#57423,
#57424,#57425,#57426,#57427,#57428,#57429,#57430,#57431,#57432,#57433,#57434,
#57435,#57436,#57437,#57438,#57439,#57440,#57441,#57442,#57443,#57444,#57445,
#57446,#57447,#57448,#57449,#57450,#57451,#57452,#57453,#57454,#57455,#57456,
#57457,#57458,#57459,#57460,#57461,#57462,#57463),.UNSPECIFIED.,.F.,.F.)
B_SPLINE_CURVE_WITH_KNOTS((6,1,1,1,1,1,1,1,1,1,1,1,1,1,1,1,1,1,1,1,1,1,
1,1,1,1,1,1,1,1,1,1,1,1,1,1,1,1,1,1,1,1,1,1,1,1,1,1,1,1,1,1,1,1,1,1,1,1,
1,1,1,1,1,1,1,6),(-1.,-0.984615384615383,-0.969230769230768,-0.953846153846152,
-0.938461538461537,-0.923076923076922,-0.907692307692306,-0.892307692307691,
-0.876923076923076,-0.86153846153846,-0.846153846153845,-0.83076923076923,
-0.815384615384614,-0.799999999999999,-0.784615384615384,-0.769230769230768,
-0.753846153846153,-0.738461538461538,-0.723076923076922,-0.707692307692307,
-0.692307692307692,-0.676923076923076,-0.661538461538461,-0.646153846153846,
-0.63076923076923,-0.615384615384615,-0.6,-0.584615384615384,-0.569230769230769,
-0.553846153846154,-0.538461538461538,-0.523076923076923,-0.507692307692308,
-0.492307692307692,-0.476923076923077,-0.461538461538462,-0.446153846153846,
-0.430769230769231,-0.415384615384615,-0.4,-0.384615384615385,-0.369230769230769,
-0.353846153846154,-0.338461538461538,-0.323076923076923,-0.307692307692308,
-0.292307692307692,-0.276923076923077,-0.261538461538462,-0.246153846153846,
-0.230769230769231,-0.215384615384615,-0.2,-0.184615384615385,-0.169230769230769,
-0.153846153846154,-0.138461538461538,-0.123076923076923,-0.107692307692308,
-0.0923076923076923,-0.0769230769230769,-0.0615384615384615,-0.0461538461538462,
-0.0307692307692308,-0.0153846153846154,-0.00577184337452469),
 .UNSPECIFIED.)
CURVE()
GEOMETRIC_REPRESENTATION_ITEM()
RATIONAL_B_SPLINE_CURVE((1.,1.,1.,1.,1.,1.,1.,1.,1.,1.,1.,1.,1.,1.,1.,1.,
1.,1.,1.,1.,1.,1.,1.,1.,1.,1.,1.,1.,1.,1.,1.,1.,1.,1.,1.,1.,1.,1.,1.,1.,
1.,1.,1.,1.,1.,1.,1.,1.,1.,1.,1.,1.,1.,1.,1.,1.,1.,1.,1.,1.,1.,1.,1.,1.,
1.,1.,1.,1.,1.,1.))
REPRESENTATION_ITEM('')
);
#420=(
BOUNDED_CURVE()
B_SPLINE_CURVE(5,(#57614,#57615,#57616,#57617,#57618,#57619,#57620,#57621,
#57622,#57623,#57624,#57625,#57626,#57627,#57628,#57629,#57630,#57631,#57632,
#57633,#57634,#57635,#57636,#57637,#57638,#57639,#57640,#57641,#57642,#57643,
#57644,#57645,#57646,#57647,#57648,#57649,#57650,#57651,#57652,#57653,#57654,
#57655,#57656,#57657,#57658,#57659,#57660,#57661,#57662,#57663,#57664,#57665,
#57666,#57667,#57668,#57669,#57670,#57671,#57672,#57673,#57674,#57675,#57676,
#57677,#57678,#57679,#57680,#57681,#57682,#57683),.UNSPECIFIED.,.F.,.F.)
B_SPLINE_CURVE_WITH_KNOTS((6,1,1,1,1,1,1,1,1,1,1,1,1,1,1,1,1,1,1,1,1,1,
1,1,1,1,1,1,1,1,1,1,1,1,1,1,1,1,1,1,1,1,1,1,1,1,1,1,1,1,1,1,1,1,1,1,1,1,
1,1,1,1,1,1,1,6),(-0.994228156739717,-0.984615384615383,-0.969230769230768,
-0.953846153846152,-0.938461538461537,-0.923076923076922,-0.907692307692306,
-0.892307692307691,-0.876923076923076,-0.86153846153846,-0.846153846153845,
-0.83076923076923,-0.815384615384614,-0.799999999999999,-0.784615384615384,
-0.769230769230768,-0.753846153846153,-0.738461538461538,-0.723076923076922,
-0.707692307692307,-0.692307692307692,-0.676923076923076,-0.661538461538461,
-0.646153846153846,-0.63076923076923,-0.615384615384615,-0.6,-0.584615384615384,
-0.569230769230769,-0.553846153846154,-0.538461538461538,-0.523076923076923,
-0.507692307692308,-0.492307692307692,-0.476923076923077,-0.461538461538462,
-0.446153846153846,-0.430769230769231,-0.415384615384615,-0.4,-0.384615384615385,
-0.369230769230769,-0.353846153846154,-0.338461538461538,-0.323076923076923,
-0.307692307692308,-0.292307692307692,-0.276923076923077,-0.261538461538462,
-0.246153846153846,-0.230769230769231,-0.215384615384615,-0.2,-0.184615384615385,
-0.169230769230769,-0.153846153846154,-0.138461538461538,-0.123076923076923,
-0.107692307692308,-0.0923076923076923,-0.0769230769230769,-0.0615384615384615,
-0.0461538461538462,-0.0307692307692308,-0.0153846153846154,0.),
 .UNSPECIFIED.)
CURVE()
GEOMETRIC_REPRESENTATION_ITEM()
RATIONAL_B_SPLINE_CURVE((1.,1.,1.,1.,1.,1.,1.,1.,1.,1.,1.,1.,1.,1.,1.,1.,
1.,1.,1.,1.,1.,1.,1.,1.,1.,1.,1.,1.,1.,1.,1.,1.,1.,1.,1.,1.,1.,1.,1.,1.,
1.,1.,1.,1.,1.,1.,1.,1.,1.,1.,1.,1.,1.,1.,1.,1.,1.,1.,1.,1.,1.,1.,1.,1.,
1.,1.,1.,1.,1.,1.))
REPRESENTATION_ITEM('')
);
#421=(
BOUNDED_CURVE()
B_SPLINE_CURVE(5,(#57836,#57837,#57838,#57839,#57840,#57841,#57842,#57843,
#57844,#57845,#57846,#57847,#57848,#57849,#57850,#57851,#57852,#57853,#57854,
#57855,#57856,#57857,#57858,#57859,#57860,#57861,#57862,#57863,#57864,#57865,
#57866,#57867,#57868,#57869,#57870,#57871,#57872,#57873,#57874,#57875,#57876,
#57877,#57878,#57879,#57880,#57881,#57882,#57883,#57884,#57885,#57886,#57887,
#57888,#57889,#57890,#57891,#57892,#57893,#57894,#57895,#57896,#57897,#57898,
#57899,#57900,#57901,#57902,#57903,#57904,#57905),.UNSPECIFIED.,.F.,.F.)
B_SPLINE_CURVE_WITH_KNOTS((6,1,1,1,1,1,1,1,1,1,1,1,1,1,1,1,1,1,1,1,1,1,
1,1,1,1,1,1,1,1,1,1,1,1,1,1,1,1,1,1,1,1,1,1,1,1,1,1,1,1,1,1,1,1,1,1,1,1,
1,1,1,1,1,1,1,6),(-1.,-0.984615384615383,-0.969230769230768,-0.953846153846152,
-0.938461538461537,-0.923076923076922,-0.907692307692306,-0.892307692307691,
-0.876923076923076,-0.86153846153846,-0.846153846153845,-0.83076923076923,
-0.815384615384614,-0.799999999999999,-0.784615384615384,-0.769230769230768,
-0.753846153846153,-0.738461538461538,-0.723076923076922,-0.707692307692307,
-0.692307692307692,-0.676923076923076,-0.661538461538461,-0.646153846153846,
-0.63076923076923,-0.615384615384615,-0.6,-0.584615384615384,-0.569230769230769,
-0.553846153846154,-0.538461538461538,-0.523076923076923,-0.507692307692308,
-0.492307692307692,-0.476923076923077,-0.461538461538462,-0.446153846153846,
-0.430769230769231,-0.415384615384615,-0.4,-0.384615384615385,-0.369230769230769,
-0.353846153846154,-0.338461538461538,-0.323076923076923,-0.307692307692308,
-0.292307692307692,-0.276923076923077,-0.261538461538462,-0.246153846153846,
-0.230769230769231,-0.215384615384615,-0.2,-0.184615384615385,-0.169230769230769,
-0.153846153846154,-0.138461538461538,-0.123076923076923,-0.107692307692308,
-0.0923076923076923,-0.0769230769230769,-0.0615384615384615,-0.0461538461538462,
-0.0307692307692308,-0.0153846153846154,-0.00577184337453472),
 .UNSPECIFIED.)
CURVE()
GEOMETRIC_REPRESENTATION_ITEM()
RATIONAL_B_SPLINE_CURVE((1.,1.,1.,1.,1.,1.,1.,1.,1.,1.,1.,1.,1.,1.,1.,1.,
1.,1.,1.,1.,1.,1.,1.,1.,1.,1.,1.,1.,1.,1.,1.,1.,1.,1.,1.,1.,1.,1.,1.,1.,
1.,1.,1.,1.,1.,1.,1.,1.,1.,1.,1.,1.,1.,1.,1.,1.,1.,1.,1.,1.,1.,1.,1.,1.,
1.,1.,1.,1.,1.,1.))
REPRESENTATION_ITEM('')
);
#422=(
BOUNDED_CURVE()
B_SPLINE_CURVE(5,(#58056,#58057,#58058,#58059,#58060,#58061,#58062,#58063,
#58064,#58065,#58066,#58067,#58068,#58069,#58070,#58071,#58072,#58073,#58074,
#58075,#58076,#58077,#58078,#58079,#58080,#58081,#58082,#58083,#58084,#58085,
#58086,#58087,#58088,#58089,#58090,#58091,#58092,#58093,#58094,#58095,#58096,
#58097,#58098,#58099,#58100,#58101,#58102,#58103,#58104,#58105,#58106,#58107,
#58108,#58109,#58110,#58111,#58112,#58113,#58114,#58115,#58116,#58117,#58118,
#58119,#58120,#58121,#58122,#58123,#58124,#58125),.UNSPECIFIED.,.F.,.F.)
B_SPLINE_CURVE_WITH_KNOTS((6,1,1,1,1,1,1,1,1,1,1,1,1,1,1,1,1,1,1,1,1,1,
1,1,1,1,1,1,1,1,1,1,1,1,1,1,1,1,1,1,1,1,1,1,1,1,1,1,1,1,1,1,1,1,1,1,1,1,
1,1,1,1,1,1,1,6),(-0.994228156739652,-0.984615384615383,-0.969230769230768,
-0.953846153846152,-0.938461538461537,-0.923076923076922,-0.907692307692306,
-0.892307692307691,-0.876923076923076,-0.86153846153846,-0.846153846153845,
-0.83076923076923,-0.815384615384614,-0.799999999999999,-0.784615384615384,
-0.769230769230768,-0.753846153846153,-0.738461538461538,-0.723076923076922,
-0.707692307692307,-0.692307692307692,-0.676923076923076,-0.661538461538461,
-0.646153846153846,-0.63076923076923,-0.615384615384615,-0.6,-0.584615384615384,
-0.569230769230769,-0.553846153846154,-0.538461538461538,-0.523076923076923,
-0.507692307692308,-0.492307692307692,-0.476923076923077,-0.461538461538462,
-0.446153846153846,-0.430769230769231,-0.415384615384615,-0.4,-0.384615384615385,
-0.369230769230769,-0.353846153846154,-0.338461538461538,-0.323076923076923,
-0.307692307692308,-0.292307692307692,-0.276923076923077,-0.261538461538462,
-0.246153846153846,-0.230769230769231,-0.215384615384615,-0.2,-0.184615384615385,
-0.169230769230769,-0.153846153846154,-0.138461538461538,-0.123076923076923,
-0.107692307692308,-0.0923076923076923,-0.0769230769230769,-0.0615384615384615,
-0.0461538461538462,-0.0307692307692308,-0.0153846153846154,0.),
 .UNSPECIFIED.)
CURVE()
GEOMETRIC_REPRESENTATION_ITEM()
RATIONAL_B_SPLINE_CURVE((1.,1.,1.,1.,1.,1.,1.,1.,1.,1.,1.,1.,1.,1.,1.,1.,
1.,1.,1.,1.,1.,1.,1.,1.,1.,1.,1.,1.,1.,1.,1.,1.,1.,1.,1.,1.,1.,1.,1.,1.,
1.,1.,1.,1.,1.,1.,1.,1.,1.,1.,1.,1.,1.,1.,1.,1.,1.,1.,1.,1.,1.,1.,1.,1.,
1.,1.,1.,1.,1.,1.))
REPRESENTATION_ITEM('')
);
#423=(
BOUNDED_CURVE()
B_SPLINE_CURVE(5,(#58278,#58279,#58280,#58281,#58282,#58283,#58284,#58285,
#58286,#58287,#58288,#58289,#58290,#58291,#58292,#58293,#58294,#58295,#58296,
#58297,#58298,#58299,#58300,#58301,#58302,#58303,#58304,#58305,#58306,#58307,
#58308,#58309,#58310,#58311,#58312,#58313,#58314,#58315,#58316,#58317,#58318,
#58319,#58320,#58321,#58322,#58323,#58324,#58325,#58326,#58327,#58328,#58329,
#58330,#58331,#58332,#58333,#58334,#58335,#58336,#58337,#58338,#58339,#58340,
#58341,#58342,#58343,#58344,#58345,#58346,#58347),.UNSPECIFIED.,.F.,.F.)
B_SPLINE_CURVE_WITH_KNOTS((6,1,1,1,1,1,1,1,1,1,1,1,1,1,1,1,1,1,1,1,1,1,
1,1,1,1,1,1,1,1,1,1,1,1,1,1,1,1,1,1,1,1,1,1,1,1,1,1,1,1,1,1,1,1,1,1,1,1,
1,1,1,1,1,1,1,6),(-1.,-0.984615384615383,-0.969230769230768,-0.953846153846152,
-0.938461538461537,-0.923076923076922,-0.907692307692306,-0.892307692307691,
-0.876923076923076,-0.86153846153846,-0.846153846153845,-0.83076923076923,
-0.815384615384614,-0.799999999999999,-0.784615384615384,-0.769230769230768,
-0.753846153846153,-0.738461538461538,-0.723076923076922,-0.707692307692307,
-0.692307692307692,-0.676923076923076,-0.661538461538461,-0.646153846153846,
-0.63076923076923,-0.615384615384615,-0.6,-0.584615384615384,-0.569230769230769,
-0.553846153846154,-0.538461538461538,-0.523076923076923,-0.507692307692308,
-0.492307692307692,-0.476923076923077,-0.461538461538462,-0.446153846153846,
-0.430769230769231,-0.415384615384615,-0.4,-0.384615384615385,-0.369230769230769,
-0.353846153846154,-0.338461538461538,-0.323076923076923,-0.307692307692308,
-0.292307692307692,-0.276923076923077,-0.261538461538462,-0.246153846153846,
-0.230769230769231,-0.215384615384615,-0.2,-0.184615384615385,-0.169230769230769,
-0.153846153846154,-0.138461538461538,-0.123076923076923,-0.107692307692308,
-0.0923076923076923,-0.0769230769230769,-0.0615384615384615,-0.0461538461538462,
-0.0307692307692308,-0.0153846153846154,-0.00577184337450876),
 .UNSPECIFIED.)
CURVE()
GEOMETRIC_REPRESENTATION_ITEM()
RATIONAL_B_SPLINE_CURVE((1.,1.,1.,1.,1.,1.,1.,1.,1.,1.,1.,1.,1.,1.,1.,1.,
1.,1.,1.,1.,1.,1.,1.,1.,1.,1.,1.,1.,1.,1.,1.,1.,1.,1.,1.,1.,1.,1.,1.,1.,
1.,1.,1.,1.,1.,1.,1.,1.,1.,1.,1.,1.,1.,1.,1.,1.,1.,1.,1.,1.,1.,1.,1.,1.,
1.,1.,1.,1.,1.,1.))
REPRESENTATION_ITEM('')
);
#424=(
BOUNDED_CURVE()
B_SPLINE_CURVE(5,(#58498,#58499,#58500,#58501,#58502,#58503,#58504,#58505,
#58506,#58507,#58508,#58509,#58510,#58511,#58512,#58513,#58514,#58515,#58516,
#58517,#58518,#58519,#58520,#58521,#58522,#58523,#58524,#58525,#58526,#58527,
#58528,#58529,#58530,#58531,#58532,#58533,#58534,#58535,#58536,#58537,#58538,
#58539,#58540,#58541,#58542,#58543,#58544,#58545,#58546,#58547,#58548,#58549,
#58550,#58551,#58552,#58553,#58554,#58555,#58556,#58557,#58558,#58559,#58560,
#58561,#58562,#58563,#58564,#58565,#58566,#58567),.UNSPECIFIED.,.F.,.F.)
B_SPLINE_CURVE_WITH_KNOTS((6,1,1,1,1,1,1,1,1,1,1,1,1,1,1,1,1,1,1,1,1,1,
1,1,1,1,1,1,1,1,1,1,1,1,1,1,1,1,1,1,1,1,1,1,1,1,1,1,1,1,1,1,1,1,1,1,1,1,
1,1,1,1,1,1,1,6),(-0.994228156739683,-0.984615384615383,-0.969230769230768,
-0.953846153846152,-0.938461538461537,-0.923076923076922,-0.907692307692306,
-0.892307692307691,-0.876923076923076,-0.86153846153846,-0.846153846153845,
-0.83076923076923,-0.815384615384614,-0.799999999999999,-0.784615384615384,
-0.769230769230768,-0.753846153846153,-0.738461538461538,-0.723076923076922,
-0.707692307692307,-0.692307692307692,-0.676923076923076,-0.661538461538461,
-0.646153846153846,-0.63076923076923,-0.615384615384615,-0.6,-0.584615384615384,
-0.569230769230769,-0.553846153846154,-0.538461538461538,-0.523076923076923,
-0.507692307692308,-0.492307692307692,-0.476923076923077,-0.461538461538462,
-0.446153846153846,-0.430769230769231,-0.415384615384615,-0.4,-0.384615384615385,
-0.369230769230769,-0.353846153846154,-0.338461538461538,-0.323076923076923,
-0.307692307692308,-0.292307692307692,-0.276923076923077,-0.261538461538462,
-0.246153846153846,-0.230769230769231,-0.215384615384615,-0.2,-0.184615384615385,
-0.169230769230769,-0.153846153846154,-0.138461538461538,-0.123076923076923,
-0.107692307692308,-0.0923076923076923,-0.0769230769230769,-0.0615384615384615,
-0.0461538461538462,-0.0307692307692308,-0.0153846153846154,0.),
 .UNSPECIFIED.)
CURVE()
GEOMETRIC_REPRESENTATION_ITEM()
RATIONAL_B_SPLINE_CURVE((1.,1.,1.,1.,1.,1.,1.,1.,1.,1.,1.,1.,1.,1.,1.,1.,
1.,1.,1.,1.,1.,1.,1.,1.,1.,1.,1.,1.,1.,1.,1.,1.,1.,1.,1.,1.,1.,1.,1.,1.,
1.,1.,1.,1.,1.,1.,1.,1.,1.,1.,1.,1.,1.,1.,1.,1.,1.,1.,1.,1.,1.,1.,1.,1.,
1.,1.,1.,1.,1.,1.))
REPRESENTATION_ITEM('')
);
#425=(
BOUNDED_CURVE()
B_SPLINE_CURVE(5,(#58720,#58721,#58722,#58723,#58724,#58725,#58726,#58727,
#58728,#58729,#58730,#58731,#58732,#58733,#58734,#58735,#58736,#58737,#58738,
#58739,#58740,#58741,#58742,#58743,#58744,#58745,#58746,#58747,#58748,#58749,
#58750,#58751,#58752,#58753,#58754,#58755,#58756,#58757,#58758,#58759,#58760,
#58761,#58762,#58763,#58764,#58765,#58766,#58767,#58768,#58769,#58770,#58771,
#58772,#58773,#58774,#58775,#58776,#58777,#58778,#58779,#58780,#58781,#58782,
#58783,#58784,#58785,#58786,#58787,#58788,#58789),.UNSPECIFIED.,.F.,.F.)
B_SPLINE_CURVE_WITH_KNOTS((6,1,1,1,1,1,1,1,1,1,1,1,1,1,1,1,1,1,1,1,1,1,
1,1,1,1,1,1,1,1,1,1,1,1,1,1,1,1,1,1,1,1,1,1,1,1,1,1,1,1,1,1,1,1,1,1,1,1,
1,1,1,1,1,1,1,6),(-1.,-0.984615384615383,-0.969230769230768,-0.953846153846152,
-0.938461538461537,-0.923076923076922,-0.907692307692306,-0.892307692307691,
-0.876923076923076,-0.86153846153846,-0.846153846153845,-0.83076923076923,
-0.815384615384614,-0.799999999999999,-0.784615384615384,-0.769230769230768,
-0.753846153846153,-0.738461538461538,-0.723076923076922,-0.707692307692307,
-0.692307692307692,-0.676923076923076,-0.661538461538461,-0.646153846153846,
-0.63076923076923,-0.615384615384615,-0.6,-0.584615384615384,-0.569230769230769,
-0.553846153846154,-0.538461538461538,-0.523076923076923,-0.507692307692308,
-0.492307692307692,-0.476923076923077,-0.461538461538462,-0.446153846153846,
-0.430769230769231,-0.415384615384615,-0.4,-0.384615384615385,-0.369230769230769,
-0.353846153846154,-0.338461538461538,-0.323076923076923,-0.307692307692308,
-0.292307692307692,-0.276923076923077,-0.261538461538462,-0.246153846153846,
-0.230769230769231,-0.215384615384615,-0.2,-0.184615384615385,-0.169230769230769,
-0.153846153846154,-0.138461538461538,-0.123076923076923,-0.107692307692308,
-0.0923076923076923,-0.0769230769230769,-0.0615384615384615,-0.0461538461538462,
-0.0307692307692308,-0.0153846153846154,-0.00577184337450277),
 .UNSPECIFIED.)
CURVE()
GEOMETRIC_REPRESENTATION_ITEM()
RATIONAL_B_SPLINE_CURVE((1.,1.,1.,1.,1.,1.,1.,1.,1.,1.,1.,1.,1.,1.,1.,1.,
1.,1.,1.,1.,1.,1.,1.,1.,1.,1.,1.,1.,1.,1.,1.,1.,1.,1.,1.,1.,1.,1.,1.,1.,
1.,1.,1.,1.,1.,1.,1.,1.,1.,1.,1.,1.,1.,1.,1.,1.,1.,1.,1.,1.,1.,1.,1.,1.,
1.,1.,1.,1.,1.,1.))
REPRESENTATION_ITEM('')
);
#426=(
BOUNDED_CURVE()
B_SPLINE_CURVE(5,(#58940,#58941,#58942,#58943,#58944,#58945,#58946,#58947,
#58948,#58949,#58950,#58951,#58952,#58953,#58954,#58955,#58956,#58957,#58958,
#58959,#58960,#58961,#58962,#58963,#58964,#58965,#58966,#58967,#58968,#58969,
#58970,#58971,#58972,#58973,#58974,#58975,#58976,#58977,#58978,#58979,#58980,
#58981,#58982,#58983,#58984,#58985,#58986,#58987,#58988,#58989,#58990,#58991,
#58992,#58993,#58994,#58995,#58996,#58997,#58998,#58999,#59000,#59001,#59002,
#59003,#59004,#59005,#59006,#59007,#59008,#59009),.UNSPECIFIED.,.F.,.F.)
B_SPLINE_CURVE_WITH_KNOTS((6,1,1,1,1,1,1,1,1,1,1,1,1,1,1,1,1,1,1,1,1,1,
1,1,1,1,1,1,1,1,1,1,1,1,1,1,1,1,1,1,1,1,1,1,1,1,1,1,1,1,1,1,1,1,1,1,1,1,
1,1,1,1,1,1,1,6),(-0.994228156739689,-0.984615384615383,-0.969230769230768,
-0.953846153846152,-0.938461538461537,-0.923076923076922,-0.907692307692306,
-0.892307692307691,-0.876923076923076,-0.86153846153846,-0.846153846153845,
-0.83076923076923,-0.815384615384614,-0.799999999999999,-0.784615384615384,
-0.769230769230768,-0.753846153846153,-0.738461538461538,-0.723076923076922,
-0.707692307692307,-0.692307692307692,-0.676923076923076,-0.661538461538461,
-0.646153846153846,-0.63076923076923,-0.615384615384615,-0.6,-0.584615384615384,
-0.569230769230769,-0.553846153846154,-0.538461538461538,-0.523076923076923,
-0.507692307692308,-0.492307692307692,-0.476923076923077,-0.461538461538462,
-0.446153846153846,-0.430769230769231,-0.415384615384615,-0.4,-0.384615384615385,
-0.369230769230769,-0.353846153846154,-0.338461538461538,-0.323076923076923,
-0.307692307692308,-0.292307692307692,-0.276923076923077,-0.261538461538462,
-0.246153846153846,-0.230769230769231,-0.215384615384615,-0.2,-0.184615384615385,
-0.169230769230769,-0.153846153846154,-0.138461538461538,-0.123076923076923,
-0.107692307692308,-0.0923076923076923,-0.0769230769230769,-0.0615384615384615,
-0.0461538461538462,-0.0307692307692308,-0.0153846153846154,0.),
 .UNSPECIFIED.)
CURVE()
GEOMETRIC_REPRESENTATION_ITEM()
RATIONAL_B_SPLINE_CURVE((1.,1.,1.,1.,1.,1.,1.,1.,1.,1.,1.,1.,1.,1.,1.,1.,
1.,1.,1.,1.,1.,1.,1.,1.,1.,1.,1.,1.,1.,1.,1.,1.,1.,1.,1.,1.,1.,1.,1.,1.,
1.,1.,1.,1.,1.,1.,1.,1.,1.,1.,1.,1.,1.,1.,1.,1.,1.,1.,1.,1.,1.,1.,1.,1.,
1.,1.,1.,1.,1.,1.))
REPRESENTATION_ITEM('')
);
#427=(
BOUNDED_CURVE()
B_SPLINE_CURVE(5,(#59162,#59163,#59164,#59165,#59166,#59167,#59168,#59169,
#59170,#59171,#59172,#59173,#59174,#59175,#59176,#59177,#59178,#59179,#59180,
#59181,#59182,#59183,#59184,#59185,#59186,#59187,#59188,#59189,#59190,#59191,
#59192,#59193,#59194,#59195,#59196,#59197,#59198,#59199,#59200,#59201,#59202,
#59203,#59204,#59205,#59206,#59207,#59208,#59209,#59210,#59211,#59212,#59213,
#59214,#59215,#59216,#59217,#59218,#59219,#59220,#59221,#59222,#59223,#59224,
#59225,#59226,#59227,#59228,#59229,#59230,#59231),.UNSPECIFIED.,.F.,.F.)
B_SPLINE_CURVE_WITH_KNOTS((6,1,1,1,1,1,1,1,1,1,1,1,1,1,1,1,1,1,1,1,1,1,
1,1,1,1,1,1,1,1,1,1,1,1,1,1,1,1,1,1,1,1,1,1,1,1,1,1,1,1,1,1,1,1,1,1,1,1,
1,1,1,1,1,1,1,6),(-1.,-0.984615384615383,-0.969230769230768,-0.953846153846152,
-0.938461538461537,-0.923076923076922,-0.907692307692306,-0.892307692307691,
-0.876923076923076,-0.86153846153846,-0.846153846153845,-0.83076923076923,
-0.815384615384614,-0.799999999999999,-0.784615384615384,-0.769230769230768,
-0.753846153846153,-0.738461538461538,-0.723076923076922,-0.707692307692307,
-0.692307692307692,-0.676923076923076,-0.661538461538461,-0.646153846153846,
-0.63076923076923,-0.615384615384615,-0.6,-0.584615384615384,-0.569230769230769,
-0.553846153846154,-0.538461538461538,-0.523076923076923,-0.507692307692308,
-0.492307692307692,-0.476923076923077,-0.461538461538462,-0.446153846153846,
-0.430769230769231,-0.415384615384615,-0.4,-0.384615384615385,-0.369230769230769,
-0.353846153846154,-0.338461538461538,-0.323076923076923,-0.307692307692308,
-0.292307692307692,-0.276923076923077,-0.261538461538462,-0.246153846153846,
-0.230769230769231,-0.215384615384615,-0.2,-0.184615384615385,-0.169230769230769,
-0.153846153846154,-0.138461538461538,-0.123076923076923,-0.107692307692308,
-0.0923076923076923,-0.0769230769230769,-0.0615384615384615,-0.0461538461538462,
-0.0307692307692308,-0.0153846153846154,-0.00577184337451766),
 .UNSPECIFIED.)
CURVE()
GEOMETRIC_REPRESENTATION_ITEM()
RATIONAL_B_SPLINE_CURVE((1.,1.,1.,1.,1.,1.,1.,1.,1.,1.,1.,1.,1.,1.,1.,1.,
1.,1.,1.,1.,1.,1.,1.,1.,1.,1.,1.,1.,1.,1.,1.,1.,1.,1.,1.,1.,1.,1.,1.,1.,
1.,1.,1.,1.,1.,1.,1.,1.,1.,1.,1.,1.,1.,1.,1.,1.,1.,1.,1.,1.,1.,1.,1.,1.,
1.,1.,1.,1.,1.,1.))
REPRESENTATION_ITEM('')
);
#428=(
BOUNDED_CURVE()
B_SPLINE_CURVE(5,(#59382,#59383,#59384,#59385,#59386,#59387,#59388,#59389,
#59390,#59391,#59392,#59393,#59394,#59395,#59396,#59397,#59398,#59399,#59400,
#59401,#59402,#59403,#59404,#59405,#59406,#59407,#59408,#59409,#59410,#59411,
#59412,#59413,#59414,#59415,#59416,#59417,#59418,#59419,#59420,#59421,#59422,
#59423,#59424,#59425,#59426,#59427,#59428,#59429,#59430,#59431,#59432,#59433,
#59434,#59435,#59436,#59437,#59438,#59439,#59440,#59441,#59442,#59443,#59444,
#59445,#59446,#59447,#59448,#59449,#59450,#59451),.UNSPECIFIED.,.F.,.F.)
B_SPLINE_CURVE_WITH_KNOTS((6,1,1,1,1,1,1,1,1,1,1,1,1,1,1,1,1,1,1,1,1,1,
1,1,1,1,1,1,1,1,1,1,1,1,1,1,1,1,1,1,1,1,1,1,1,1,1,1,1,1,1,1,1,1,1,1,1,1,
1,1,1,1,1,1,1,6),(-0.994228156739687,-0.984615384615383,-0.969230769230768,
-0.953846153846152,-0.938461538461537,-0.923076923076922,-0.907692307692306,
-0.892307692307691,-0.876923076923076,-0.86153846153846,-0.846153846153845,
-0.83076923076923,-0.815384615384614,-0.799999999999999,-0.784615384615384,
-0.769230769230768,-0.753846153846153,-0.738461538461538,-0.723076923076922,
-0.707692307692307,-0.692307692307692,-0.676923076923076,-0.661538461538461,
-0.646153846153846,-0.63076923076923,-0.615384615384615,-0.6,-0.584615384615384,
-0.569230769230769,-0.553846153846154,-0.538461538461538,-0.523076923076923,
-0.507692307692308,-0.492307692307692,-0.476923076923077,-0.461538461538462,
-0.446153846153846,-0.430769230769231,-0.415384615384615,-0.4,-0.384615384615385,
-0.369230769230769,-0.353846153846154,-0.338461538461538,-0.323076923076923,
-0.307692307692308,-0.292307692307692,-0.276923076923077,-0.261538461538462,
-0.246153846153846,-0.230769230769231,-0.215384615384615,-0.2,-0.184615384615385,
-0.169230769230769,-0.153846153846154,-0.138461538461538,-0.123076923076923,
-0.107692307692308,-0.0923076923076923,-0.0769230769230769,-0.0615384615384615,
-0.0461538461538462,-0.0307692307692308,-0.0153846153846154,0.),
 .UNSPECIFIED.)
CURVE()
GEOMETRIC_REPRESENTATION_ITEM()
RATIONAL_B_SPLINE_CURVE((1.,1.,1.,1.,1.,1.,1.,1.,1.,1.,1.,1.,1.,1.,1.,1.,
1.,1.,1.,1.,1.,1.,1.,1.,1.,1.,1.,1.,1.,1.,1.,1.,1.,1.,1.,1.,1.,1.,1.,1.,
1.,1.,1.,1.,1.,1.,1.,1.,1.,1.,1.,1.,1.,1.,1.,1.,1.,1.,1.,1.,1.,1.,1.,1.,
1.,1.,1.,1.,1.,1.))
REPRESENTATION_ITEM('')
);
#429=(
BOUNDED_CURVE()
B_SPLINE_CURVE(5,(#59604,#59605,#59606,#59607,#59608,#59609,#59610,#59611,
#59612,#59613,#59614,#59615,#59616,#59617,#59618,#59619,#59620,#59621,#59622,
#59623,#59624,#59625,#59626,#59627,#59628,#59629,#59630,#59631,#59632,#59633,
#59634,#59635,#59636,#59637,#59638,#59639,#59640,#59641,#59642,#59643,#59644,
#59645,#59646,#59647,#59648,#59649,#59650,#59651,#59652,#59653,#59654,#59655,
#59656,#59657,#59658,#59659,#59660,#59661,#59662,#59663,#59664,#59665,#59666,
#59667,#59668,#59669,#59670,#59671,#59672,#59673),.UNSPECIFIED.,.F.,.F.)
B_SPLINE_CURVE_WITH_KNOTS((6,1,1,1,1,1,1,1,1,1,1,1,1,1,1,1,1,1,1,1,1,1,
1,1,1,1,1,1,1,1,1,1,1,1,1,1,1,1,1,1,1,1,1,1,1,1,1,1,1,1,1,1,1,1,1,1,1,1,
1,1,1,1,1,1,1,6),(-1.,-0.984615384615383,-0.969230769230768,-0.953846153846152,
-0.938461538461537,-0.923076923076922,-0.907692307692306,-0.892307692307691,
-0.876923076923076,-0.86153846153846,-0.846153846153845,-0.83076923076923,
-0.815384615384614,-0.799999999999999,-0.784615384615384,-0.769230769230768,
-0.753846153846153,-0.738461538461538,-0.723076923076922,-0.707692307692307,
-0.692307692307692,-0.676923076923076,-0.661538461538461,-0.646153846153846,
-0.63076923076923,-0.615384615384615,-0.6,-0.584615384615384,-0.569230769230769,
-0.553846153846154,-0.538461538461538,-0.523076923076923,-0.507692307692308,
-0.492307692307692,-0.476923076923077,-0.461538461538462,-0.446153846153846,
-0.430769230769231,-0.415384615384615,-0.4,-0.384615384615385,-0.369230769230769,
-0.353846153846154,-0.338461538461538,-0.323076923076923,-0.307692307692308,
-0.292307692307692,-0.276923076923077,-0.261538461538462,-0.246153846153846,
-0.230769230769231,-0.215384615384615,-0.2,-0.184615384615385,-0.169230769230769,
-0.153846153846154,-0.138461538461538,-0.123076923076923,-0.107692307692308,
-0.0923076923076923,-0.0769230769230769,-0.0615384615384615,-0.0461538461538462,
-0.0307692307692308,-0.0153846153846154,-0.00577184337452512),
 .UNSPECIFIED.)
CURVE()
GEOMETRIC_REPRESENTATION_ITEM()
RATIONAL_B_SPLINE_CURVE((1.,1.,1.,1.,1.,1.,1.,1.,1.,1.,1.,1.,1.,1.,1.,1.,
1.,1.,1.,1.,1.,1.,1.,1.,1.,1.,1.,1.,1.,1.,1.,1.,1.,1.,1.,1.,1.,1.,1.,1.,
1.,1.,1.,1.,1.,1.,1.,1.,1.,1.,1.,1.,1.,1.,1.,1.,1.,1.,1.,1.,1.,1.,1.,1.,
1.,1.,1.,1.,1.,1.))
REPRESENTATION_ITEM('')
);
#430=(
BOUNDED_CURVE()
B_SPLINE_CURVE(5,(#59824,#59825,#59826,#59827,#59828,#59829,#59830,#59831,
#59832,#59833,#59834,#59835,#59836,#59837,#59838,#59839,#59840,#59841,#59842,
#59843,#59844,#59845,#59846,#59847,#59848,#59849,#59850,#59851,#59852,#59853,
#59854,#59855,#59856,#59857,#59858,#59859,#59860,#59861,#59862,#59863,#59864,
#59865,#59866,#59867,#59868,#59869,#59870,#59871,#59872,#59873,#59874,#59875,
#59876,#59877,#59878,#59879,#59880,#59881,#59882,#59883,#59884,#59885,#59886,
#59887,#59888,#59889,#59890,#59891,#59892,#59893),.UNSPECIFIED.,.F.,.F.)
B_SPLINE_CURVE_WITH_KNOTS((6,1,1,1,1,1,1,1,1,1,1,1,1,1,1,1,1,1,1,1,1,1,
1,1,1,1,1,1,1,1,1,1,1,1,1,1,1,1,1,1,1,1,1,1,1,1,1,1,1,1,1,1,1,1,1,1,1,1,
1,1,1,1,1,1,1,6),(-0.994228156739691,-0.984615384615383,-0.969230769230768,
-0.953846153846152,-0.938461538461537,-0.923076923076922,-0.907692307692306,
-0.892307692307691,-0.876923076923076,-0.86153846153846,-0.846153846153845,
-0.83076923076923,-0.815384615384614,-0.799999999999999,-0.784615384615384,
-0.769230769230768,-0.753846153846153,-0.738461538461538,-0.723076923076922,
-0.707692307692307,-0.692307692307692,-0.676923076923076,-0.661538461538461,
-0.646153846153846,-0.63076923076923,-0.615384615384615,-0.6,-0.584615384615384,
-0.569230769230769,-0.553846153846154,-0.538461538461538,-0.523076923076923,
-0.507692307692308,-0.492307692307692,-0.476923076923077,-0.461538461538462,
-0.446153846153846,-0.430769230769231,-0.415384615384615,-0.4,-0.384615384615385,
-0.369230769230769,-0.353846153846154,-0.338461538461538,-0.323076923076923,
-0.307692307692308,-0.292307692307692,-0.276923076923077,-0.261538461538462,
-0.246153846153846,-0.230769230769231,-0.215384615384615,-0.2,-0.184615384615385,
-0.169230769230769,-0.153846153846154,-0.138461538461538,-0.123076923076923,
-0.107692307692308,-0.0923076923076923,-0.0769230769230769,-0.0615384615384615,
-0.0461538461538462,-0.0307692307692308,-0.0153846153846154,0.),
 .UNSPECIFIED.)
CURVE()
GEOMETRIC_REPRESENTATION_ITEM()
RATIONAL_B_SPLINE_CURVE((1.,1.,1.,1.,1.,1.,1.,1.,1.,1.,1.,1.,1.,1.,1.,1.,
1.,1.,1.,1.,1.,1.,1.,1.,1.,1.,1.,1.,1.,1.,1.,1.,1.,1.,1.,1.,1.,1.,1.,1.,
1.,1.,1.,1.,1.,1.,1.,1.,1.,1.,1.,1.,1.,1.,1.,1.,1.,1.,1.,1.,1.,1.,1.,1.,
1.,1.,1.,1.,1.,1.))
REPRESENTATION_ITEM('')
);
#431=(
BOUNDED_CURVE()
B_SPLINE_CURVE(5,(#60046,#60047,#60048,#60049,#60050,#60051,#60052,#60053,
#60054,#60055,#60056,#60057,#60058,#60059,#60060,#60061,#60062,#60063,#60064,
#60065,#60066,#60067,#60068,#60069,#60070,#60071,#60072,#60073,#60074,#60075,
#60076,#60077,#60078,#60079,#60080,#60081,#60082,#60083,#60084,#60085,#60086,
#60087,#60088,#60089,#60090,#60091,#60092,#60093,#60094,#60095,#60096,#60097,
#60098,#60099,#60100,#60101,#60102,#60103,#60104,#60105,#60106,#60107,#60108,
#60109,#60110,#60111,#60112,#60113,#60114,#60115),.UNSPECIFIED.,.F.,.F.)
B_SPLINE_CURVE_WITH_KNOTS((6,1,1,1,1,1,1,1,1,1,1,1,1,1,1,1,1,1,1,1,1,1,
1,1,1,1,1,1,1,1,1,1,1,1,1,1,1,1,1,1,1,1,1,1,1,1,1,1,1,1,1,1,1,1,1,1,1,1,
1,1,1,1,1,1,1,6),(-1.,-0.984615384615383,-0.969230769230768,-0.953846153846152,
-0.938461538461537,-0.923076923076922,-0.907692307692306,-0.892307692307691,
-0.876923076923076,-0.86153846153846,-0.846153846153845,-0.83076923076923,
-0.815384615384614,-0.799999999999999,-0.784615384615384,-0.769230769230768,
-0.753846153846153,-0.738461538461538,-0.723076923076922,-0.707692307692307,
-0.692307692307692,-0.676923076923076,-0.661538461538461,-0.646153846153846,
-0.63076923076923,-0.615384615384615,-0.6,-0.584615384615384,-0.569230769230769,
-0.553846153846154,-0.538461538461538,-0.523076923076923,-0.507692307692308,
-0.492307692307692,-0.476923076923077,-0.461538461538462,-0.446153846153846,
-0.430769230769231,-0.415384615384615,-0.4,-0.384615384615385,-0.369230769230769,
-0.353846153846154,-0.338461538461538,-0.323076923076923,-0.307692307692308,
-0.292307692307692,-0.276923076923077,-0.261538461538462,-0.246153846153846,
-0.230769230769231,-0.215384615384615,-0.2,-0.184615384615385,-0.169230769230769,
-0.153846153846154,-0.138461538461538,-0.123076923076923,-0.107692307692308,
-0.0923076923076923,-0.0769230769230769,-0.0615384615384615,-0.0461538461538462,
-0.0307692307692308,-0.0153846153846154,-0.00577184337448448),
 .UNSPECIFIED.)
CURVE()
GEOMETRIC_REPRESENTATION_ITEM()
RATIONAL_B_SPLINE_CURVE((1.,1.,1.,1.,1.,1.,1.,1.,1.,1.,1.,1.,1.,1.,1.,1.,
1.,1.,1.,1.,1.,1.,1.,1.,1.,1.,1.,1.,1.,1.,1.,1.,1.,1.,1.,1.,1.,1.,1.,1.,
1.,1.,1.,1.,1.,1.,1.,1.,1.,1.,1.,1.,1.,1.,1.,1.,1.,1.,1.,1.,1.,1.,1.,1.,
1.,1.,1.,1.,1.,1.))
REPRESENTATION_ITEM('')
);
#432=(
BOUNDED_CURVE()
B_SPLINE_CURVE(5,(#60266,#60267,#60268,#60269,#60270,#60271,#60272,#60273,
#60274,#60275,#60276,#60277,#60278,#60279,#60280,#60281,#60282,#60283,#60284,
#60285,#60286,#60287,#60288,#60289,#60290,#60291,#60292,#60293,#60294,#60295,
#60296,#60297,#60298,#60299,#60300,#60301,#60302,#60303,#60304,#60305,#60306,
#60307,#60308,#60309,#60310,#60311,#60312,#60313,#60314,#60315,#60316,#60317,
#60318,#60319,#60320,#60321,#60322,#60323,#60324,#60325,#60326,#60327,#60328,
#60329,#60330,#60331,#60332,#60333,#60334,#60335),.UNSPECIFIED.,.F.,.F.)
B_SPLINE_CURVE_WITH_KNOTS((6,1,1,1,1,1,1,1,1,1,1,1,1,1,1,1,1,1,1,1,1,1,
1,1,1,1,1,1,1,1,1,1,1,1,1,1,1,1,1,1,1,1,1,1,1,1,1,1,1,1,1,1,1,1,1,1,1,1,
1,1,1,1,1,1,1,6),(-0.99422815673972,-0.984615384615383,-0.969230769230768,
-0.953846153846152,-0.938461538461537,-0.923076923076922,-0.907692307692306,
-0.892307692307691,-0.876923076923076,-0.86153846153846,-0.846153846153845,
-0.83076923076923,-0.815384615384614,-0.799999999999999,-0.784615384615384,
-0.769230769230768,-0.753846153846153,-0.738461538461538,-0.723076923076922,
-0.707692307692307,-0.692307692307692,-0.676923076923076,-0.661538461538461,
-0.646153846153846,-0.63076923076923,-0.615384615384615,-0.6,-0.584615384615384,
-0.569230769230769,-0.553846153846154,-0.538461538461538,-0.523076923076923,
-0.507692307692308,-0.492307692307692,-0.476923076923077,-0.461538461538462,
-0.446153846153846,-0.430769230769231,-0.415384615384615,-0.4,-0.384615384615385,
-0.369230769230769,-0.353846153846154,-0.338461538461538,-0.323076923076923,
-0.307692307692308,-0.292307692307692,-0.276923076923077,-0.261538461538462,
-0.246153846153846,-0.230769230769231,-0.215384615384615,-0.2,-0.184615384615385,
-0.169230769230769,-0.153846153846154,-0.138461538461538,-0.123076923076923,
-0.107692307692308,-0.0923076923076923,-0.0769230769230769,-0.0615384615384615,
-0.0461538461538462,-0.0307692307692308,-0.0153846153846154,0.),
 .UNSPECIFIED.)
CURVE()
GEOMETRIC_REPRESENTATION_ITEM()
RATIONAL_B_SPLINE_CURVE((1.,1.,1.,1.,1.,1.,1.,1.,1.,1.,1.,1.,1.,1.,1.,1.,
1.,1.,1.,1.,1.,1.,1.,1.,1.,1.,1.,1.,1.,1.,1.,1.,1.,1.,1.,1.,1.,1.,1.,1.,
1.,1.,1.,1.,1.,1.,1.,1.,1.,1.,1.,1.,1.,1.,1.,1.,1.,1.,1.,1.,1.,1.,1.,1.,
1.,1.,1.,1.,1.,1.))
REPRESENTATION_ITEM('')
);
#433=(
BOUNDED_CURVE()
B_SPLINE_CURVE(5,(#60488,#60489,#60490,#60491,#60492,#60493,#60494,#60495,
#60496,#60497,#60498,#60499,#60500,#60501,#60502,#60503,#60504,#60505,#60506,
#60507,#60508,#60509,#60510,#60511,#60512,#60513,#60514,#60515,#60516,#60517,
#60518,#60519,#60520,#60521,#60522,#60523,#60524,#60525,#60526,#60527,#60528,
#60529,#60530,#60531,#60532,#60533,#60534,#60535,#60536,#60537,#60538,#60539,
#60540,#60541,#60542,#60543,#60544,#60545,#60546,#60547,#60548,#60549,#60550,
#60551,#60552,#60553,#60554,#60555,#60556,#60557),.UNSPECIFIED.,.F.,.F.)
B_SPLINE_CURVE_WITH_KNOTS((6,1,1,1,1,1,1,1,1,1,1,1,1,1,1,1,1,1,1,1,1,1,
1,1,1,1,1,1,1,1,1,1,1,1,1,1,1,1,1,1,1,1,1,1,1,1,1,1,1,1,1,1,1,1,1,1,1,1,
1,1,1,1,1,1,1,6),(-1.,-0.984615384615383,-0.969230769230768,-0.953846153846152,
-0.938461538461537,-0.923076923076922,-0.907692307692306,-0.892307692307691,
-0.876923076923076,-0.86153846153846,-0.846153846153845,-0.83076923076923,
-0.815384615384614,-0.799999999999999,-0.784615384615384,-0.769230769230768,
-0.753846153846153,-0.738461538461538,-0.723076923076922,-0.707692307692307,
-0.692307692307692,-0.676923076923076,-0.661538461538461,-0.646153846153846,
-0.63076923076923,-0.615384615384615,-0.6,-0.584615384615384,-0.569230769230769,
-0.553846153846154,-0.538461538461538,-0.523076923076923,-0.507692307692308,
-0.492307692307692,-0.476923076923077,-0.461538461538462,-0.446153846153846,
-0.430769230769231,-0.415384615384615,-0.4,-0.384615384615385,-0.369230769230769,
-0.353846153846154,-0.338461538461538,-0.323076923076923,-0.307692307692308,
-0.292307692307692,-0.276923076923077,-0.261538461538462,-0.246153846153846,
-0.230769230769231,-0.215384615384615,-0.2,-0.184615384615385,-0.169230769230769,
-0.153846153846154,-0.138461538461538,-0.123076923076923,-0.107692307692308,
-0.0923076923076923,-0.0769230769230769,-0.0615384615384615,-0.0461538461538462,
-0.0307692307692308,-0.0153846153846154,-0.00577184337448251),
 .UNSPECIFIED.)
CURVE()
GEOMETRIC_REPRESENTATION_ITEM()
RATIONAL_B_SPLINE_CURVE((1.,1.,1.,1.,1.,1.,1.,1.,1.,1.,1.,1.,1.,1.,1.,1.,
1.,1.,1.,1.,1.,1.,1.,1.,1.,1.,1.,1.,1.,1.,1.,1.,1.,1.,1.,1.,1.,1.,1.,1.,
1.,1.,1.,1.,1.,1.,1.,1.,1.,1.,1.,1.,1.,1.,1.,1.,1.,1.,1.,1.,1.,1.,1.,1.,
1.,1.,1.,1.,1.,1.))
REPRESENTATION_ITEM('')
);
#434=(
BOUNDED_CURVE()
B_SPLINE_CURVE(5,(#60708,#60709,#60710,#60711,#60712,#60713,#60714,#60715,
#60716,#60717,#60718,#60719,#60720,#60721,#60722,#60723,#60724,#60725,#60726,
#60727,#60728,#60729,#60730,#60731,#60732,#60733,#60734,#60735,#60736,#60737,
#60738,#60739,#60740,#60741,#60742,#60743,#60744,#60745,#60746,#60747,#60748,
#60749,#60750,#60751,#60752,#60753,#60754,#60755,#60756,#60757,#60758,#60759,
#60760,#60761,#60762,#60763,#60764,#60765,#60766,#60767,#60768,#60769,#60770,
#60771,#60772,#60773,#60774,#60775,#60776,#60777),.UNSPECIFIED.,.F.,.F.)
B_SPLINE_CURVE_WITH_KNOTS((6,1,1,1,1,1,1,1,1,1,1,1,1,1,1,1,1,1,1,1,1,1,
1,1,1,1,1,1,1,1,1,1,1,1,1,1,1,1,1,1,1,1,1,1,1,1,1,1,1,1,1,1,1,1,1,1,1,1,
1,1,1,1,1,1,1,6),(-0.994228156739703,-0.984615384615383,-0.969230769230768,
-0.953846153846152,-0.938461538461537,-0.923076923076922,-0.907692307692306,
-0.892307692307691,-0.876923076923076,-0.86153846153846,-0.846153846153845,
-0.83076923076923,-0.815384615384614,-0.799999999999999,-0.784615384615384,
-0.769230769230768,-0.753846153846153,-0.738461538461538,-0.723076923076922,
-0.707692307692307,-0.692307692307692,-0.676923076923076,-0.661538461538461,
-0.646153846153846,-0.63076923076923,-0.615384615384615,-0.6,-0.584615384615384,
-0.569230769230769,-0.553846153846154,-0.538461538461538,-0.523076923076923,
-0.507692307692308,-0.492307692307692,-0.476923076923077,-0.461538461538462,
-0.446153846153846,-0.430769230769231,-0.415384615384615,-0.4,-0.384615384615385,
-0.369230769230769,-0.353846153846154,-0.338461538461538,-0.323076923076923,
-0.307692307692308,-0.292307692307692,-0.276923076923077,-0.261538461538462,
-0.246153846153846,-0.230769230769231,-0.215384615384615,-0.2,-0.184615384615385,
-0.169230769230769,-0.153846153846154,-0.138461538461538,-0.123076923076923,
-0.107692307692308,-0.0923076923076923,-0.0769230769230769,-0.0615384615384615,
-0.0461538461538462,-0.0307692307692308,-0.0153846153846154,0.),
 .UNSPECIFIED.)
CURVE()
GEOMETRIC_REPRESENTATION_ITEM()
RATIONAL_B_SPLINE_CURVE((1.,1.,1.,1.,1.,1.,1.,1.,1.,1.,1.,1.,1.,1.,1.,1.,
1.,1.,1.,1.,1.,1.,1.,1.,1.,1.,1.,1.,1.,1.,1.,1.,1.,1.,1.,1.,1.,1.,1.,1.,
1.,1.,1.,1.,1.,1.,1.,1.,1.,1.,1.,1.,1.,1.,1.,1.,1.,1.,1.,1.,1.,1.,1.,1.,
1.,1.,1.,1.,1.,1.))
REPRESENTATION_ITEM('')
);
#435=(
BOUNDED_CURVE()
B_SPLINE_CURVE(5,(#60930,#60931,#60932,#60933,#60934,#60935,#60936,#60937,
#60938,#60939,#60940,#60941,#60942,#60943,#60944,#60945,#60946,#60947,#60948,
#60949,#60950,#60951,#60952,#60953,#60954,#60955,#60956,#60957,#60958,#60959,
#60960,#60961,#60962,#60963,#60964,#60965,#60966,#60967,#60968,#60969,#60970,
#60971,#60972,#60973,#60974,#60975,#60976,#60977,#60978,#60979,#60980,#60981,
#60982,#60983,#60984,#60985,#60986,#60987,#60988,#60989,#60990,#60991,#60992,
#60993,#60994,#60995,#60996,#60997,#60998,#60999),.UNSPECIFIED.,.F.,.F.)
B_SPLINE_CURVE_WITH_KNOTS((6,1,1,1,1,1,1,1,1,1,1,1,1,1,1,1,1,1,1,1,1,1,
1,1,1,1,1,1,1,1,1,1,1,1,1,1,1,1,1,1,1,1,1,1,1,1,1,1,1,1,1,1,1,1,1,1,1,1,
1,1,1,1,1,1,1,6),(-1.,-0.984615384615383,-0.969230769230768,-0.953846153846152,
-0.938461538461537,-0.923076923076922,-0.907692307692306,-0.892307692307691,
-0.876923076923076,-0.86153846153846,-0.846153846153845,-0.83076923076923,
-0.815384615384614,-0.799999999999999,-0.784615384615384,-0.769230769230768,
-0.753846153846153,-0.738461538461538,-0.723076923076922,-0.707692307692307,
-0.692307692307692,-0.676923076923076,-0.661538461538461,-0.646153846153846,
-0.63076923076923,-0.615384615384615,-0.6,-0.584615384615384,-0.569230769230769,
-0.553846153846154,-0.538461538461538,-0.523076923076923,-0.507692307692308,
-0.492307692307692,-0.476923076923077,-0.461538461538462,-0.446153846153846,
-0.430769230769231,-0.415384615384615,-0.4,-0.384615384615385,-0.369230769230769,
-0.353846153846154,-0.338461538461538,-0.323076923076923,-0.307692307692308,
-0.292307692307692,-0.276923076923077,-0.261538461538462,-0.246153846153846,
-0.230769230769231,-0.215384615384615,-0.2,-0.184615384615385,-0.169230769230769,
-0.153846153846154,-0.138461538461538,-0.123076923076923,-0.107692307692308,
-0.0923076923076923,-0.0769230769230769,-0.0615384615384615,-0.0461538461538462,
-0.0307692307692308,-0.0153846153846154,-0.00577184337449602),
 .UNSPECIFIED.)
CURVE()
GEOMETRIC_REPRESENTATION_ITEM()
RATIONAL_B_SPLINE_CURVE((1.,1.,1.,1.,1.,1.,1.,1.,1.,1.,1.,1.,1.,1.,1.,1.,
1.,1.,1.,1.,1.,1.,1.,1.,1.,1.,1.,1.,1.,1.,1.,1.,1.,1.,1.,1.,1.,1.,1.,1.,
1.,1.,1.,1.,1.,1.,1.,1.,1.,1.,1.,1.,1.,1.,1.,1.,1.,1.,1.,1.,1.,1.,1.,1.,
1.,1.,1.,1.,1.,1.))
REPRESENTATION_ITEM('')
);
#436=(
BOUNDED_CURVE()
B_SPLINE_CURVE(5,(#61150,#61151,#61152,#61153,#61154,#61155,#61156,#61157,
#61158,#61159,#61160,#61161,#61162,#61163,#61164,#61165,#61166,#61167,#61168,
#61169,#61170,#61171,#61172,#61173,#61174,#61175,#61176,#61177,#61178,#61179,
#61180,#61181,#61182,#61183,#61184,#61185,#61186,#61187,#61188,#61189,#61190,
#61191,#61192,#61193,#61194,#61195,#61196,#61197,#61198,#61199,#61200,#61201,
#61202,#61203,#61204,#61205,#61206,#61207,#61208,#61209,#61210,#61211,#61212,
#61213,#61214,#61215,#61216,#61217,#61218,#61219),.UNSPECIFIED.,.F.,.F.)
B_SPLINE_CURVE_WITH_KNOTS((6,1,1,1,1,1,1,1,1,1,1,1,1,1,1,1,1,1,1,1,1,1,
1,1,1,1,1,1,1,1,1,1,1,1,1,1,1,1,1,1,1,1,1,1,1,1,1,1,1,1,1,1,1,1,1,1,1,1,
1,1,1,1,1,1,1,6),(-0.994228156739695,-0.984615384615383,-0.969230769230768,
-0.953846153846152,-0.938461538461537,-0.923076923076922,-0.907692307692306,
-0.892307692307691,-0.876923076923076,-0.86153846153846,-0.846153846153845,
-0.83076923076923,-0.815384615384614,-0.799999999999999,-0.784615384615384,
-0.769230769230768,-0.753846153846153,-0.738461538461538,-0.723076923076922,
-0.707692307692307,-0.692307692307692,-0.676923076923076,-0.661538461538461,
-0.646153846153846,-0.63076923076923,-0.615384615384615,-0.6,-0.584615384615384,
-0.569230769230769,-0.553846153846154,-0.538461538461538,-0.523076923076923,
-0.507692307692308,-0.492307692307692,-0.476923076923077,-0.461538461538462,
-0.446153846153846,-0.430769230769231,-0.415384615384615,-0.4,-0.384615384615385,
-0.369230769230769,-0.353846153846154,-0.338461538461538,-0.323076923076923,
-0.307692307692308,-0.292307692307692,-0.276923076923077,-0.261538461538462,
-0.246153846153846,-0.230769230769231,-0.215384615384615,-0.2,-0.184615384615385,
-0.169230769230769,-0.153846153846154,-0.138461538461538,-0.123076923076923,
-0.107692307692308,-0.0923076923076923,-0.0769230769230769,-0.0615384615384615,
-0.0461538461538462,-0.0307692307692308,-0.0153846153846154,0.),
 .UNSPECIFIED.)
CURVE()
GEOMETRIC_REPRESENTATION_ITEM()
RATIONAL_B_SPLINE_CURVE((1.,1.,1.,1.,1.,1.,1.,1.,1.,1.,1.,1.,1.,1.,1.,1.,
1.,1.,1.,1.,1.,1.,1.,1.,1.,1.,1.,1.,1.,1.,1.,1.,1.,1.,1.,1.,1.,1.,1.,1.,
1.,1.,1.,1.,1.,1.,1.,1.,1.,1.,1.,1.,1.,1.,1.,1.,1.,1.,1.,1.,1.,1.,1.,1.,
1.,1.,1.,1.,1.,1.))
REPRESENTATION_ITEM('')
);
#437=(
BOUNDED_CURVE()
B_SPLINE_CURVE(5,(#61372,#61373,#61374,#61375,#61376,#61377,#61378,#61379,
#61380,#61381,#61382,#61383,#61384,#61385,#61386,#61387,#61388,#61389,#61390,
#61391,#61392,#61393,#61394,#61395,#61396,#61397,#61398,#61399,#61400,#61401,
#61402,#61403,#61404,#61405,#61406,#61407,#61408,#61409,#61410,#61411,#61412,
#61413,#61414,#61415,#61416,#61417,#61418,#61419,#61420,#61421,#61422,#61423,
#61424,#61425,#61426,#61427,#61428,#61429,#61430,#61431,#61432,#61433,#61434,
#61435,#61436,#61437,#61438,#61439,#61440,#61441),.UNSPECIFIED.,.F.,.F.)
B_SPLINE_CURVE_WITH_KNOTS((6,1,1,1,1,1,1,1,1,1,1,1,1,1,1,1,1,1,1,1,1,1,
1,1,1,1,1,1,1,1,1,1,1,1,1,1,1,1,1,1,1,1,1,1,1,1,1,1,1,1,1,1,1,1,1,1,1,1,
1,1,1,1,1,1,1,6),(-1.,-0.984615384615383,-0.969230769230768,-0.953846153846152,
-0.938461538461537,-0.923076923076922,-0.907692307692306,-0.892307692307691,
-0.876923076923076,-0.86153846153846,-0.846153846153845,-0.83076923076923,
-0.815384615384614,-0.799999999999999,-0.784615384615384,-0.769230769230768,
-0.753846153846153,-0.738461538461538,-0.723076923076922,-0.707692307692307,
-0.692307692307692,-0.676923076923076,-0.661538461538461,-0.646153846153846,
-0.63076923076923,-0.615384615384615,-0.6,-0.584615384615384,-0.569230769230769,
-0.553846153846154,-0.538461538461538,-0.523076923076923,-0.507692307692308,
-0.492307692307692,-0.476923076923077,-0.461538461538462,-0.446153846153846,
-0.430769230769231,-0.415384615384615,-0.4,-0.384615384615385,-0.369230769230769,
-0.353846153846154,-0.338461538461538,-0.323076923076923,-0.307692307692308,
-0.292307692307692,-0.276923076923077,-0.261538461538462,-0.246153846153846,
-0.230769230769231,-0.215384615384615,-0.2,-0.184615384615385,-0.169230769230769,
-0.153846153846154,-0.138461538461538,-0.123076923076923,-0.107692307692308,
-0.0923076923076923,-0.0769230769230769,-0.0615384615384615,-0.0461538461538462,
-0.0307692307692308,-0.0153846153846154,-0.00577184337450911),
 .UNSPECIFIED.)
CURVE()
GEOMETRIC_REPRESENTATION_ITEM()
RATIONAL_B_SPLINE_CURVE((1.,1.,1.,1.,1.,1.,1.,1.,1.,1.,1.,1.,1.,1.,1.,1.,
1.,1.,1.,1.,1.,1.,1.,1.,1.,1.,1.,1.,1.,1.,1.,1.,1.,1.,1.,1.,1.,1.,1.,1.,
1.,1.,1.,1.,1.,1.,1.,1.,1.,1.,1.,1.,1.,1.,1.,1.,1.,1.,1.,1.,1.,1.,1.,1.,
1.,1.,1.,1.,1.,1.))
REPRESENTATION_ITEM('')
);
#438=(
BOUNDED_CURVE()
B_SPLINE_CURVE(5,(#61592,#61593,#61594,#61595,#61596,#61597,#61598,#61599,
#61600,#61601,#61602,#61603,#61604,#61605,#61606,#61607,#61608,#61609,#61610,
#61611,#61612,#61613,#61614,#61615,#61616,#61617,#61618,#61619,#61620,#61621,
#61622,#61623,#61624,#61625,#61626,#61627,#61628,#61629,#61630,#61631,#61632,
#61633,#61634,#61635,#61636,#61637,#61638,#61639,#61640,#61641,#61642,#61643,
#61644,#61645,#61646,#61647,#61648,#61649,#61650,#61651,#61652,#61653,#61654,
#61655,#61656,#61657,#61658,#61659,#61660,#61661),.UNSPECIFIED.,.F.,.F.)
B_SPLINE_CURVE_WITH_KNOTS((6,1,1,1,1,1,1,1,1,1,1,1,1,1,1,1,1,1,1,1,1,1,
1,1,1,1,1,1,1,1,1,1,1,1,1,1,1,1,1,1,1,1,1,1,1,1,1,1,1,1,1,1,1,1,1,1,1,1,
1,1,1,1,1,1,1,6),(-0.994228156739712,-0.984615384615383,-0.969230769230768,
-0.953846153846152,-0.938461538461537,-0.923076923076922,-0.907692307692306,
-0.892307692307691,-0.876923076923076,-0.86153846153846,-0.846153846153845,
-0.83076923076923,-0.815384615384614,-0.799999999999999,-0.784615384615384,
-0.769230769230768,-0.753846153846153,-0.738461538461538,-0.723076923076922,
-0.707692307692307,-0.692307692307692,-0.676923076923076,-0.661538461538461,
-0.646153846153846,-0.63076923076923,-0.615384615384615,-0.6,-0.584615384615384,
-0.569230769230769,-0.553846153846154,-0.538461538461538,-0.523076923076923,
-0.507692307692308,-0.492307692307692,-0.476923076923077,-0.461538461538462,
-0.446153846153846,-0.430769230769231,-0.415384615384615,-0.4,-0.384615384615385,
-0.369230769230769,-0.353846153846154,-0.338461538461538,-0.323076923076923,
-0.307692307692308,-0.292307692307692,-0.276923076923077,-0.261538461538462,
-0.246153846153846,-0.230769230769231,-0.215384615384615,-0.2,-0.184615384615385,
-0.169230769230769,-0.153846153846154,-0.138461538461538,-0.123076923076923,
-0.107692307692308,-0.0923076923076923,-0.0769230769230769,-0.0615384615384615,
-0.0461538461538462,-0.0307692307692308,-0.0153846153846154,0.),
 .UNSPECIFIED.)
CURVE()
GEOMETRIC_REPRESENTATION_ITEM()
RATIONAL_B_SPLINE_CURVE((1.,1.,1.,1.,1.,1.,1.,1.,1.,1.,1.,1.,1.,1.,1.,1.,
1.,1.,1.,1.,1.,1.,1.,1.,1.,1.,1.,1.,1.,1.,1.,1.,1.,1.,1.,1.,1.,1.,1.,1.,
1.,1.,1.,1.,1.,1.,1.,1.,1.,1.,1.,1.,1.,1.,1.,1.,1.,1.,1.,1.,1.,1.,1.,1.,
1.,1.,1.,1.,1.,1.))
REPRESENTATION_ITEM('')
);
#439=(
BOUNDED_CURVE()
B_SPLINE_CURVE(5,(#61814,#61815,#61816,#61817,#61818,#61819,#61820,#61821,
#61822,#61823,#61824,#61825,#61826,#61827,#61828,#61829,#61830,#61831,#61832,
#61833,#61834,#61835,#61836,#61837,#61838,#61839,#61840,#61841,#61842,#61843,
#61844,#61845,#61846,#61847,#61848,#61849,#61850,#61851,#61852,#61853,#61854,
#61855,#61856,#61857,#61858,#61859,#61860,#61861,#61862,#61863,#61864,#61865,
#61866,#61867,#61868,#61869,#61870,#61871,#61872,#61873,#61874,#61875,#61876,
#61877,#61878,#61879,#61880,#61881,#61882,#61883),.UNSPECIFIED.,.F.,.F.)
B_SPLINE_CURVE_WITH_KNOTS((6,1,1,1,1,1,1,1,1,1,1,1,1,1,1,1,1,1,1,1,1,1,
1,1,1,1,1,1,1,1,1,1,1,1,1,1,1,1,1,1,1,1,1,1,1,1,1,1,1,1,1,1,1,1,1,1,1,1,
1,1,1,1,1,1,1,6),(-1.,-0.984615384615383,-0.969230769230768,-0.953846153846152,
-0.938461538461537,-0.923076923076922,-0.907692307692306,-0.892307692307691,
-0.876923076923076,-0.86153846153846,-0.846153846153845,-0.83076923076923,
-0.815384615384614,-0.799999999999999,-0.784615384615384,-0.769230769230768,
-0.753846153846153,-0.738461538461538,-0.723076923076922,-0.707692307692307,
-0.692307692307692,-0.676923076923076,-0.661538461538461,-0.646153846153846,
-0.63076923076923,-0.615384615384615,-0.6,-0.584615384615384,-0.569230769230769,
-0.553846153846154,-0.538461538461538,-0.523076923076923,-0.507692307692308,
-0.492307692307692,-0.476923076923077,-0.461538461538462,-0.446153846153846,
-0.430769230769231,-0.415384615384615,-0.4,-0.384615384615385,-0.369230769230769,
-0.353846153846154,-0.338461538461538,-0.323076923076923,-0.307692307692308,
-0.292307692307692,-0.276923076923077,-0.261538461538462,-0.246153846153846,
-0.230769230769231,-0.215384615384615,-0.2,-0.184615384615385,-0.169230769230769,
-0.153846153846154,-0.138461538461538,-0.123076923076923,-0.107692307692308,
-0.0923076923076923,-0.0769230769230769,-0.0615384615384615,-0.0461538461538462,
-0.0307692307692308,-0.0153846153846154,-0.00577184337451206),
 .UNSPECIFIED.)
CURVE()
GEOMETRIC_REPRESENTATION_ITEM()
RATIONAL_B_SPLINE_CURVE((1.,1.,1.,1.,1.,1.,1.,1.,1.,1.,1.,1.,1.,1.,1.,1.,
1.,1.,1.,1.,1.,1.,1.,1.,1.,1.,1.,1.,1.,1.,1.,1.,1.,1.,1.,1.,1.,1.,1.,1.,
1.,1.,1.,1.,1.,1.,1.,1.,1.,1.,1.,1.,1.,1.,1.,1.,1.,1.,1.,1.,1.,1.,1.,1.,
1.,1.,1.,1.,1.,1.))
REPRESENTATION_ITEM('')
);
#440=(
BOUNDED_CURVE()
B_SPLINE_CURVE(5,(#62034,#62035,#62036,#62037,#62038,#62039,#62040,#62041,
#62042,#62043,#62044,#62045,#62046,#62047,#62048,#62049,#62050,#62051,#62052,
#62053,#62054,#62055,#62056,#62057,#62058,#62059,#62060,#62061,#62062,#62063,
#62064,#62065,#62066,#62067,#62068,#62069,#62070,#62071,#62072,#62073,#62074,
#62075,#62076,#62077,#62078,#62079,#62080,#62081,#62082,#62083,#62084,#62085,
#62086,#62087,#62088,#62089,#62090,#62091,#62092,#62093,#62094,#62095,#62096,
#62097,#62098,#62099,#62100,#62101,#62102,#62103),.UNSPECIFIED.,.F.,.F.)
B_SPLINE_CURVE_WITH_KNOTS((6,1,1,1,1,1,1,1,1,1,1,1,1,1,1,1,1,1,1,1,1,1,
1,1,1,1,1,1,1,1,1,1,1,1,1,1,1,1,1,1,1,1,1,1,1,1,1,1,1,1,1,1,1,1,1,1,1,1,
1,1,1,1,1,1,1,6),(-0.994228156739717,-0.984615384615383,-0.969230769230768,
-0.953846153846152,-0.938461538461537,-0.923076923076922,-0.907692307692306,
-0.892307692307691,-0.876923076923076,-0.86153846153846,-0.846153846153845,
-0.83076923076923,-0.815384615384614,-0.799999999999999,-0.784615384615384,
-0.769230769230768,-0.753846153846153,-0.738461538461538,-0.723076923076922,
-0.707692307692307,-0.692307692307692,-0.676923076923076,-0.661538461538461,
-0.646153846153846,-0.63076923076923,-0.615384615384615,-0.6,-0.584615384615384,
-0.569230769230769,-0.553846153846154,-0.538461538461538,-0.523076923076923,
-0.507692307692308,-0.492307692307692,-0.476923076923077,-0.461538461538462,
-0.446153846153846,-0.430769230769231,-0.415384615384615,-0.4,-0.384615384615385,
-0.369230769230769,-0.353846153846154,-0.338461538461538,-0.323076923076923,
-0.307692307692308,-0.292307692307692,-0.276923076923077,-0.261538461538462,
-0.246153846153846,-0.230769230769231,-0.215384615384615,-0.2,-0.184615384615385,
-0.169230769230769,-0.153846153846154,-0.138461538461538,-0.123076923076923,
-0.107692307692308,-0.0923076923076923,-0.0769230769230769,-0.0615384615384615,
-0.0461538461538462,-0.0307692307692308,-0.0153846153846154,0.),
 .UNSPECIFIED.)
CURVE()
GEOMETRIC_REPRESENTATION_ITEM()
RATIONAL_B_SPLINE_CURVE((1.,1.,1.,1.,1.,1.,1.,1.,1.,1.,1.,1.,1.,1.,1.,1.,
1.,1.,1.,1.,1.,1.,1.,1.,1.,1.,1.,1.,1.,1.,1.,1.,1.,1.,1.,1.,1.,1.,1.,1.,
1.,1.,1.,1.,1.,1.,1.,1.,1.,1.,1.,1.,1.,1.,1.,1.,1.,1.,1.,1.,1.,1.,1.,1.,
1.,1.,1.,1.,1.,1.))
REPRESENTATION_ITEM('')
);
#441=(
BOUNDED_CURVE()
B_SPLINE_CURVE(5,(#62256,#62257,#62258,#62259,#62260,#62261,#62262,#62263,
#62264,#62265,#62266,#62267,#62268,#62269,#62270,#62271,#62272,#62273,#62274,
#62275,#62276,#62277,#62278,#62279,#62280,#62281,#62282,#62283,#62284,#62285,
#62286,#62287,#62288,#62289,#62290,#62291,#62292,#62293,#62294,#62295,#62296,
#62297,#62298,#62299,#62300,#62301,#62302,#62303,#62304,#62305,#62306,#62307,
#62308,#62309,#62310,#62311,#62312,#62313,#62314,#62315,#62316,#62317,#62318,
#62319,#62320,#62321,#62322,#62323,#62324,#62325),.UNSPECIFIED.,.F.,.F.)
B_SPLINE_CURVE_WITH_KNOTS((6,1,1,1,1,1,1,1,1,1,1,1,1,1,1,1,1,1,1,1,1,1,
1,1,1,1,1,1,1,1,1,1,1,1,1,1,1,1,1,1,1,1,1,1,1,1,1,1,1,1,1,1,1,1,1,1,1,1,
1,1,1,1,1,1,1,6),(-1.,-0.984615384615383,-0.969230769230768,-0.953846153846152,
-0.938461538461537,-0.923076923076922,-0.907692307692306,-0.892307692307691,
-0.876923076923076,-0.86153846153846,-0.846153846153845,-0.83076923076923,
-0.815384615384614,-0.799999999999999,-0.784615384615384,-0.769230769230768,
-0.753846153846153,-0.738461538461538,-0.723076923076922,-0.707692307692307,
-0.692307692307692,-0.676923076923076,-0.661538461538461,-0.646153846153846,
-0.63076923076923,-0.615384615384615,-0.6,-0.584615384615384,-0.569230769230769,
-0.553846153846154,-0.538461538461538,-0.523076923076923,-0.507692307692308,
-0.492307692307692,-0.476923076923077,-0.461538461538462,-0.446153846153846,
-0.430769230769231,-0.415384615384615,-0.4,-0.384615384615385,-0.369230769230769,
-0.353846153846154,-0.338461538461538,-0.323076923076923,-0.307692307692308,
-0.292307692307692,-0.276923076923077,-0.261538461538462,-0.246153846153846,
-0.230769230769231,-0.215384615384615,-0.2,-0.184615384615385,-0.169230769230769,
-0.153846153846154,-0.138461538461538,-0.123076923076923,-0.107692307692308,
-0.0923076923076923,-0.0769230769230769,-0.0615384615384615,-0.0461538461538462,
-0.0307692307692308,-0.0153846153846154,-0.00577184337448646),
 .UNSPECIFIED.)
CURVE()
GEOMETRIC_REPRESENTATION_ITEM()
RATIONAL_B_SPLINE_CURVE((1.,1.,1.,1.,1.,1.,1.,1.,1.,1.,1.,1.,1.,1.,1.,1.,
1.,1.,1.,1.,1.,1.,1.,1.,1.,1.,1.,1.,1.,1.,1.,1.,1.,1.,1.,1.,1.,1.,1.,1.,
1.,1.,1.,1.,1.,1.,1.,1.,1.,1.,1.,1.,1.,1.,1.,1.,1.,1.,1.,1.,1.,1.,1.,1.,
1.,1.,1.,1.,1.,1.))
REPRESENTATION_ITEM('')
);
#442=(
BOUNDED_CURVE()
B_SPLINE_CURVE(5,(#62476,#62477,#62478,#62479,#62480,#62481,#62482,#62483,
#62484,#62485,#62486,#62487,#62488,#62489,#62490,#62491,#62492,#62493,#62494,
#62495,#62496,#62497,#62498,#62499,#62500,#62501,#62502,#62503,#62504,#62505,
#62506,#62507,#62508,#62509,#62510,#62511,#62512,#62513,#62514,#62515,#62516,
#62517,#62518,#62519,#62520,#62521,#62522,#62523,#62524,#62525,#62526,#62527,
#62528,#62529,#62530,#62531,#62532,#62533,#62534,#62535,#62536,#62537,#62538,
#62539,#62540,#62541,#62542,#62543,#62544,#62545),.UNSPECIFIED.,.F.,.F.)
B_SPLINE_CURVE_WITH_KNOTS((6,1,1,1,1,1,1,1,1,1,1,1,1,1,1,1,1,1,1,1,1,1,
1,1,1,1,1,1,1,1,1,1,1,1,1,1,1,1,1,1,1,1,1,1,1,1,1,1,1,1,1,1,1,1,1,1,1,1,
1,1,1,1,1,1,1,6),(-0.994228156739708,-0.984615384615383,-0.969230769230768,
-0.953846153846152,-0.938461538461537,-0.923076923076922,-0.907692307692306,
-0.892307692307691,-0.876923076923076,-0.86153846153846,-0.846153846153845,
-0.83076923076923,-0.815384615384614,-0.799999999999999,-0.784615384615384,
-0.769230769230768,-0.753846153846153,-0.738461538461538,-0.723076923076922,
-0.707692307692307,-0.692307692307692,-0.676923076923076,-0.661538461538461,
-0.646153846153846,-0.63076923076923,-0.615384615384615,-0.6,-0.584615384615384,
-0.569230769230769,-0.553846153846154,-0.538461538461538,-0.523076923076923,
-0.507692307692308,-0.492307692307692,-0.476923076923077,-0.461538461538462,
-0.446153846153846,-0.430769230769231,-0.415384615384615,-0.4,-0.384615384615385,
-0.369230769230769,-0.353846153846154,-0.338461538461538,-0.323076923076923,
-0.307692307692308,-0.292307692307692,-0.276923076923077,-0.261538461538462,
-0.246153846153846,-0.230769230769231,-0.215384615384615,-0.2,-0.184615384615385,
-0.169230769230769,-0.153846153846154,-0.138461538461538,-0.123076923076923,
-0.107692307692308,-0.0923076923076923,-0.0769230769230769,-0.0615384615384615,
-0.0461538461538462,-0.0307692307692308,-0.0153846153846154,0.),
 .UNSPECIFIED.)
CURVE()
GEOMETRIC_REPRESENTATION_ITEM()
RATIONAL_B_SPLINE_CURVE((1.,1.,1.,1.,1.,1.,1.,1.,1.,1.,1.,1.,1.,1.,1.,1.,
1.,1.,1.,1.,1.,1.,1.,1.,1.,1.,1.,1.,1.,1.,1.,1.,1.,1.,1.,1.,1.,1.,1.,1.,
1.,1.,1.,1.,1.,1.,1.,1.,1.,1.,1.,1.,1.,1.,1.,1.,1.,1.,1.,1.,1.,1.,1.,1.,
1.,1.,1.,1.,1.,1.))
REPRESENTATION_ITEM('')
);
#443=(
BOUNDED_CURVE()
B_SPLINE_CURVE(5,(#62698,#62699,#62700,#62701,#62702,#62703,#62704,#62705,
#62706,#62707,#62708,#62709,#62710,#62711,#62712,#62713,#62714,#62715,#62716,
#62717,#62718,#62719,#62720,#62721,#62722,#62723,#62724,#62725,#62726,#62727,
#62728,#62729,#62730,#62731,#62732,#62733,#62734,#62735,#62736,#62737,#62738,
#62739,#62740,#62741,#62742,#62743,#62744,#62745,#62746,#62747,#62748,#62749,
#62750,#62751,#62752,#62753,#62754,#62755,#62756,#62757,#62758,#62759,#62760,
#62761,#62762,#62763,#62764,#62765,#62766,#62767),.UNSPECIFIED.,.F.,.F.)
B_SPLINE_CURVE_WITH_KNOTS((6,1,1,1,1,1,1,1,1,1,1,1,1,1,1,1,1,1,1,1,1,1,
1,1,1,1,1,1,1,1,1,1,1,1,1,1,1,1,1,1,1,1,1,1,1,1,1,1,1,1,1,1,1,1,1,1,1,1,
1,1,1,1,1,1,1,6),(-1.,-0.984615384615383,-0.969230769230768,-0.953846153846152,
-0.938461538461537,-0.923076923076922,-0.907692307692306,-0.892307692307691,
-0.876923076923076,-0.86153846153846,-0.846153846153845,-0.83076923076923,
-0.815384615384614,-0.799999999999999,-0.784615384615384,-0.769230769230768,
-0.753846153846153,-0.738461538461538,-0.723076923076922,-0.707692307692307,
-0.692307692307692,-0.676923076923076,-0.661538461538461,-0.646153846153846,
-0.63076923076923,-0.615384615384615,-0.6,-0.584615384615384,-0.569230769230769,
-0.553846153846154,-0.538461538461538,-0.523076923076923,-0.507692307692308,
-0.492307692307692,-0.476923076923077,-0.461538461538462,-0.446153846153846,
-0.430769230769231,-0.415384615384615,-0.4,-0.384615384615385,-0.369230769230769,
-0.353846153846154,-0.338461538461538,-0.323076923076923,-0.307692307692308,
-0.292307692307692,-0.276923076923077,-0.261538461538462,-0.246153846153846,
-0.230769230769231,-0.215384615384615,-0.2,-0.184615384615385,-0.169230769230769,
-0.153846153846154,-0.138461538461538,-0.123076923076923,-0.107692307692308,
-0.0923076923076923,-0.0769230769230769,-0.0615384615384615,-0.0461538461538462,
-0.0307692307692308,-0.0153846153846154,-0.00577184337451626),
 .UNSPECIFIED.)
CURVE()
GEOMETRIC_REPRESENTATION_ITEM()
RATIONAL_B_SPLINE_CURVE((1.,1.,1.,1.,1.,1.,1.,1.,1.,1.,1.,1.,1.,1.,1.,1.,
1.,1.,1.,1.,1.,1.,1.,1.,1.,1.,1.,1.,1.,1.,1.,1.,1.,1.,1.,1.,1.,1.,1.,1.,
1.,1.,1.,1.,1.,1.,1.,1.,1.,1.,1.,1.,1.,1.,1.,1.,1.,1.,1.,1.,1.,1.,1.,1.,
1.,1.,1.,1.,1.,1.))
REPRESENTATION_ITEM('')
);
#444=(
BOUNDED_CURVE()
B_SPLINE_CURVE(5,(#62918,#62919,#62920,#62921,#62922,#62923,#62924,#62925,
#62926,#62927,#62928,#62929,#62930,#62931,#62932,#62933,#62934,#62935,#62936,
#62937,#62938,#62939,#62940,#62941,#62942,#62943,#62944,#62945,#62946,#62947,
#62948,#62949,#62950,#62951,#62952,#62953,#62954,#62955,#62956,#62957,#62958,
#62959,#62960,#62961,#62962,#62963,#62964,#62965,#62966,#62967,#62968,#62969,
#62970,#62971,#62972,#62973,#62974,#62975,#62976,#62977,#62978,#62979,#62980,
#62981,#62982,#62983,#62984,#62985,#62986,#62987),.UNSPECIFIED.,.F.,.F.)
B_SPLINE_CURVE_WITH_KNOTS((6,1,1,1,1,1,1,1,1,1,1,1,1,1,1,1,1,1,1,1,1,1,
1,1,1,1,1,1,1,1,1,1,1,1,1,1,1,1,1,1,1,1,1,1,1,1,1,1,1,1,1,1,1,1,1,1,1,1,
1,1,1,1,1,1,1,6),(-0.994228156739708,-0.984615384615383,-0.969230769230768,
-0.953846153846152,-0.938461538461537,-0.923076923076922,-0.907692307692306,
-0.892307692307691,-0.876923076923076,-0.86153846153846,-0.846153846153845,
-0.83076923076923,-0.815384615384614,-0.799999999999999,-0.784615384615384,
-0.769230769230768,-0.753846153846153,-0.738461538461538,-0.723076923076922,
-0.707692307692307,-0.692307692307692,-0.676923076923076,-0.661538461538461,
-0.646153846153846,-0.63076923076923,-0.615384615384615,-0.6,-0.584615384615384,
-0.569230769230769,-0.553846153846154,-0.538461538461538,-0.523076923076923,
-0.507692307692308,-0.492307692307692,-0.476923076923077,-0.461538461538462,
-0.446153846153846,-0.430769230769231,-0.415384615384615,-0.4,-0.384615384615385,
-0.369230769230769,-0.353846153846154,-0.338461538461538,-0.323076923076923,
-0.307692307692308,-0.292307692307692,-0.276923076923077,-0.261538461538462,
-0.246153846153846,-0.230769230769231,-0.215384615384615,-0.2,-0.184615384615385,
-0.169230769230769,-0.153846153846154,-0.138461538461538,-0.123076923076923,
-0.107692307692308,-0.0923076923076923,-0.0769230769230769,-0.0615384615384615,
-0.0461538461538462,-0.0307692307692308,-0.0153846153846154,0.),
 .UNSPECIFIED.)
CURVE()
GEOMETRIC_REPRESENTATION_ITEM()
RATIONAL_B_SPLINE_CURVE((1.,1.,1.,1.,1.,1.,1.,1.,1.,1.,1.,1.,1.,1.,1.,1.,
1.,1.,1.,1.,1.,1.,1.,1.,1.,1.,1.,1.,1.,1.,1.,1.,1.,1.,1.,1.,1.,1.,1.,1.,
1.,1.,1.,1.,1.,1.,1.,1.,1.,1.,1.,1.,1.,1.,1.,1.,1.,1.,1.,1.,1.,1.,1.,1.,
1.,1.,1.,1.,1.,1.))
REPRESENTATION_ITEM('')
);
#445=(
BOUNDED_CURVE()
B_SPLINE_CURVE(5,(#63140,#63141,#63142,#63143,#63144,#63145,#63146,#63147,
#63148,#63149,#63150,#63151,#63152,#63153,#63154,#63155,#63156,#63157,#63158,
#63159,#63160,#63161,#63162,#63163,#63164,#63165,#63166,#63167,#63168,#63169,
#63170,#63171,#63172,#63173,#63174,#63175,#63176,#63177,#63178,#63179,#63180,
#63181,#63182,#63183,#63184,#63185,#63186,#63187,#63188,#63189,#63190,#63191,
#63192,#63193,#63194,#63195,#63196,#63197,#63198,#63199,#63200,#63201,#63202,
#63203,#63204,#63205,#63206,#63207,#63208,#63209),.UNSPECIFIED.,.F.,.F.)
B_SPLINE_CURVE_WITH_KNOTS((6,1,1,1,1,1,1,1,1,1,1,1,1,1,1,1,1,1,1,1,1,1,
1,1,1,1,1,1,1,1,1,1,1,1,1,1,1,1,1,1,1,1,1,1,1,1,1,1,1,1,1,1,1,1,1,1,1,1,
1,1,1,1,1,1,1,6),(-1.,-0.984615384615383,-0.969230769230768,-0.953846153846152,
-0.938461538461537,-0.923076923076922,-0.907692307692306,-0.892307692307691,
-0.876923076923076,-0.86153846153846,-0.846153846153845,-0.83076923076923,
-0.815384615384614,-0.799999999999999,-0.784615384615384,-0.769230769230768,
-0.753846153846153,-0.738461538461538,-0.723076923076922,-0.707692307692307,
-0.692307692307692,-0.676923076923076,-0.661538461538461,-0.646153846153846,
-0.63076923076923,-0.615384615384615,-0.6,-0.584615384615384,-0.569230769230769,
-0.553846153846154,-0.538461538461538,-0.523076923076923,-0.507692307692308,
-0.492307692307692,-0.476923076923077,-0.461538461538462,-0.446153846153846,
-0.430769230769231,-0.415384615384615,-0.4,-0.384615384615385,-0.369230769230769,
-0.353846153846154,-0.338461538461538,-0.323076923076923,-0.307692307692308,
-0.292307692307692,-0.276923076923077,-0.261538461538462,-0.246153846153846,
-0.230769230769231,-0.215384615384615,-0.2,-0.184615384615385,-0.169230769230769,
-0.153846153846154,-0.138461538461538,-0.123076923076923,-0.107692307692308,
-0.0923076923076923,-0.0769230769230769,-0.0615384615384615,-0.0461538461538462,
-0.0307692307692308,-0.0153846153846154,-0.00577184337451372),
 .UNSPECIFIED.)
CURVE()
GEOMETRIC_REPRESENTATION_ITEM()
RATIONAL_B_SPLINE_CURVE((1.,1.,1.,1.,1.,1.,1.,1.,1.,1.,1.,1.,1.,1.,1.,1.,
1.,1.,1.,1.,1.,1.,1.,1.,1.,1.,1.,1.,1.,1.,1.,1.,1.,1.,1.,1.,1.,1.,1.,1.,
1.,1.,1.,1.,1.,1.,1.,1.,1.,1.,1.,1.,1.,1.,1.,1.,1.,1.,1.,1.,1.,1.,1.,1.,
1.,1.,1.,1.,1.,1.))
REPRESENTATION_ITEM('')
);
#446=(
BOUNDED_CURVE()
B_SPLINE_CURVE(5,(#63360,#63361,#63362,#63363,#63364,#63365,#63366,#63367,
#63368,#63369,#63370,#63371,#63372,#63373,#63374,#63375,#63376,#63377,#63378,
#63379,#63380,#63381,#63382,#63383,#63384,#63385,#63386,#63387,#63388,#63389,
#63390,#63391,#63392,#63393,#63394,#63395,#63396,#63397,#63398,#63399,#63400,
#63401,#63402,#63403,#63404,#63405,#63406,#63407,#63408,#63409,#63410,#63411,
#63412,#63413,#63414,#63415,#63416,#63417,#63418,#63419,#63420,#63421,#63422,
#63423,#63424,#63425,#63426,#63427,#63428,#63429),.UNSPECIFIED.,.F.,.F.)
B_SPLINE_CURVE_WITH_KNOTS((6,1,1,1,1,1,1,1,1,1,1,1,1,1,1,1,1,1,1,1,1,1,
1,1,1,1,1,1,1,1,1,1,1,1,1,1,1,1,1,1,1,1,1,1,1,1,1,1,1,1,1,1,1,1,1,1,1,1,
1,1,1,1,1,1,1,6),(-0.994228156739703,-0.984615384615383,-0.969230769230768,
-0.953846153846152,-0.938461538461537,-0.923076923076922,-0.907692307692306,
-0.892307692307691,-0.876923076923076,-0.86153846153846,-0.846153846153845,
-0.83076923076923,-0.815384615384614,-0.799999999999999,-0.784615384615384,
-0.769230769230768,-0.753846153846153,-0.738461538461538,-0.723076923076922,
-0.707692307692307,-0.692307692307692,-0.676923076923076,-0.661538461538461,
-0.646153846153846,-0.63076923076923,-0.615384615384615,-0.6,-0.584615384615384,
-0.569230769230769,-0.553846153846154,-0.538461538461538,-0.523076923076923,
-0.507692307692308,-0.492307692307692,-0.476923076923077,-0.461538461538462,
-0.446153846153846,-0.430769230769231,-0.415384615384615,-0.4,-0.384615384615385,
-0.369230769230769,-0.353846153846154,-0.338461538461538,-0.323076923076923,
-0.307692307692308,-0.292307692307692,-0.276923076923077,-0.261538461538462,
-0.246153846153846,-0.230769230769231,-0.215384615384615,-0.2,-0.184615384615385,
-0.169230769230769,-0.153846153846154,-0.138461538461538,-0.123076923076923,
-0.107692307692308,-0.0923076923076923,-0.0769230769230769,-0.0615384615384615,
-0.0461538461538462,-0.0307692307692308,-0.0153846153846154,0.),
 .UNSPECIFIED.)
CURVE()
GEOMETRIC_REPRESENTATION_ITEM()
RATIONAL_B_SPLINE_CURVE((1.,1.,1.,1.,1.,1.,1.,1.,1.,1.,1.,1.,1.,1.,1.,1.,
1.,1.,1.,1.,1.,1.,1.,1.,1.,1.,1.,1.,1.,1.,1.,1.,1.,1.,1.,1.,1.,1.,1.,1.,
1.,1.,1.,1.,1.,1.,1.,1.,1.,1.,1.,1.,1.,1.,1.,1.,1.,1.,1.,1.,1.,1.,1.,1.,
1.,1.,1.,1.,1.,1.))
REPRESENTATION_ITEM('')
);
#447=(
BOUNDED_CURVE()
B_SPLINE_CURVE(5,(#63582,#63583,#63584,#63585,#63586,#63587,#63588,#63589,
#63590,#63591,#63592,#63593,#63594,#63595,#63596,#63597,#63598,#63599,#63600,
#63601,#63602,#63603,#63604,#63605,#63606,#63607,#63608,#63609,#63610,#63611,
#63612,#63613,#63614,#63615,#63616,#63617,#63618,#63619,#63620,#63621,#63622,
#63623,#63624,#63625,#63626,#63627,#63628,#63629,#63630,#63631,#63632,#63633,
#63634,#63635,#63636,#63637,#63638,#63639,#63640,#63641,#63642,#63643,#63644,
#63645,#63646,#63647,#63648,#63649,#63650,#63651),.UNSPECIFIED.,.F.,.F.)
B_SPLINE_CURVE_WITH_KNOTS((6,1,1,1,1,1,1,1,1,1,1,1,1,1,1,1,1,1,1,1,1,1,
1,1,1,1,1,1,1,1,1,1,1,1,1,1,1,1,1,1,1,1,1,1,1,1,1,1,1,1,1,1,1,1,1,1,1,1,
1,1,1,1,1,1,1,6),(-1.,-0.984615384615383,-0.969230769230768,-0.953846153846152,
-0.938461538461537,-0.923076923076922,-0.907692307692306,-0.892307692307691,
-0.876923076923076,-0.86153846153846,-0.846153846153845,-0.83076923076923,
-0.815384615384614,-0.799999999999999,-0.784615384615384,-0.769230769230768,
-0.753846153846153,-0.738461538461538,-0.723076923076922,-0.707692307692307,
-0.692307692307692,-0.676923076923076,-0.661538461538461,-0.646153846153846,
-0.63076923076923,-0.615384615384615,-0.6,-0.584615384615384,-0.569230769230769,
-0.553846153846154,-0.538461538461538,-0.523076923076923,-0.507692307692308,
-0.492307692307692,-0.476923076923077,-0.461538461538462,-0.446153846153846,
-0.430769230769231,-0.415384615384615,-0.4,-0.384615384615385,-0.369230769230769,
-0.353846153846154,-0.338461538461538,-0.323076923076923,-0.307692307692308,
-0.292307692307692,-0.276923076923077,-0.261538461538462,-0.246153846153846,
-0.230769230769231,-0.215384615384615,-0.2,-0.184615384615385,-0.169230769230769,
-0.153846153846154,-0.138461538461538,-0.123076923076923,-0.107692307692308,
-0.0923076923076923,-0.0769230769230769,-0.0615384615384615,-0.0461538461538462,
-0.0307692307692308,-0.0153846153846154,-0.00577184337451698),
 .UNSPECIFIED.)
CURVE()
GEOMETRIC_REPRESENTATION_ITEM()
RATIONAL_B_SPLINE_CURVE((1.,1.,1.,1.,1.,1.,1.,1.,1.,1.,1.,1.,1.,1.,1.,1.,
1.,1.,1.,1.,1.,1.,1.,1.,1.,1.,1.,1.,1.,1.,1.,1.,1.,1.,1.,1.,1.,1.,1.,1.,
1.,1.,1.,1.,1.,1.,1.,1.,1.,1.,1.,1.,1.,1.,1.,1.,1.,1.,1.,1.,1.,1.,1.,1.,
1.,1.,1.,1.,1.,1.))
REPRESENTATION_ITEM('')
);
#448=(
BOUNDED_CURVE()
B_SPLINE_CURVE(5,(#63802,#63803,#63804,#63805,#63806,#63807,#63808,#63809,
#63810,#63811,#63812,#63813,#63814,#63815,#63816,#63817,#63818,#63819,#63820,
#63821,#63822,#63823,#63824,#63825,#63826,#63827,#63828,#63829,#63830,#63831,
#63832,#63833,#63834,#63835,#63836,#63837,#63838,#63839,#63840,#63841,#63842,
#63843,#63844,#63845,#63846,#63847,#63848,#63849,#63850,#63851,#63852,#63853,
#63854,#63855,#63856,#63857,#63858,#63859,#63860,#63861,#63862,#63863,#63864,
#63865,#63866,#63867,#63868,#63869,#63870,#63871),.UNSPECIFIED.,.F.,.F.)
B_SPLINE_CURVE_WITH_KNOTS((6,1,1,1,1,1,1,1,1,1,1,1,1,1,1,1,1,1,1,1,1,1,
1,1,1,1,1,1,1,1,1,1,1,1,1,1,1,1,1,1,1,1,1,1,1,1,1,1,1,1,1,1,1,1,1,1,1,1,
1,1,1,1,1,1,1,6),(-0.994228156739706,-0.984615384615383,-0.969230769230768,
-0.953846153846152,-0.938461538461537,-0.923076923076922,-0.907692307692306,
-0.892307692307691,-0.876923076923076,-0.86153846153846,-0.846153846153845,
-0.83076923076923,-0.815384615384614,-0.799999999999999,-0.784615384615384,
-0.769230769230768,-0.753846153846153,-0.738461538461538,-0.723076923076922,
-0.707692307692307,-0.692307692307692,-0.676923076923076,-0.661538461538461,
-0.646153846153846,-0.63076923076923,-0.615384615384615,-0.6,-0.584615384615384,
-0.569230769230769,-0.553846153846154,-0.538461538461538,-0.523076923076923,
-0.507692307692308,-0.492307692307692,-0.476923076923077,-0.461538461538462,
-0.446153846153846,-0.430769230769231,-0.415384615384615,-0.4,-0.384615384615385,
-0.369230769230769,-0.353846153846154,-0.338461538461538,-0.323076923076923,
-0.307692307692308,-0.292307692307692,-0.276923076923077,-0.261538461538462,
-0.246153846153846,-0.230769230769231,-0.215384615384615,-0.2,-0.184615384615385,
-0.169230769230769,-0.153846153846154,-0.138461538461538,-0.123076923076923,
-0.107692307692308,-0.0923076923076923,-0.0769230769230769,-0.0615384615384615,
-0.0461538461538462,-0.0307692307692308,-0.0153846153846154,0.),
 .UNSPECIFIED.)
CURVE()
GEOMETRIC_REPRESENTATION_ITEM()
RATIONAL_B_SPLINE_CURVE((1.,1.,1.,1.,1.,1.,1.,1.,1.,1.,1.,1.,1.,1.,1.,1.,
1.,1.,1.,1.,1.,1.,1.,1.,1.,1.,1.,1.,1.,1.,1.,1.,1.,1.,1.,1.,1.,1.,1.,1.,
1.,1.,1.,1.,1.,1.,1.,1.,1.,1.,1.,1.,1.,1.,1.,1.,1.,1.,1.,1.,1.,1.,1.,1.,
1.,1.,1.,1.,1.,1.))
REPRESENTATION_ITEM('')
);
#449=(
BOUNDED_CURVE()
B_SPLINE_CURVE(5,(#64024,#64025,#64026,#64027,#64028,#64029,#64030,#64031,
#64032,#64033,#64034,#64035,#64036,#64037,#64038,#64039,#64040,#64041,#64042,
#64043,#64044,#64045,#64046,#64047,#64048,#64049,#64050,#64051,#64052,#64053,
#64054,#64055,#64056,#64057,#64058,#64059,#64060,#64061,#64062,#64063,#64064,
#64065,#64066,#64067,#64068,#64069,#64070,#64071,#64072,#64073,#64074,#64075,
#64076,#64077,#64078,#64079,#64080,#64081,#64082,#64083,#64084,#64085,#64086,
#64087,#64088,#64089,#64090,#64091,#64092,#64093),.UNSPECIFIED.,.F.,.F.)
B_SPLINE_CURVE_WITH_KNOTS((6,1,1,1,1,1,1,1,1,1,1,1,1,1,1,1,1,1,1,1,1,1,
1,1,1,1,1,1,1,1,1,1,1,1,1,1,1,1,1,1,1,1,1,1,1,1,1,1,1,1,1,1,1,1,1,1,1,1,
1,1,1,1,1,1,1,6),(-1.,-0.984615384615383,-0.969230769230768,-0.953846153846152,
-0.938461538461537,-0.923076923076922,-0.907692307692306,-0.892307692307691,
-0.876923076923076,-0.86153846153846,-0.846153846153845,-0.83076923076923,
-0.815384615384614,-0.799999999999999,-0.784615384615384,-0.769230769230768,
-0.753846153846153,-0.738461538461538,-0.723076923076922,-0.707692307692307,
-0.692307692307692,-0.676923076923076,-0.661538461538461,-0.646153846153846,
-0.63076923076923,-0.615384615384615,-0.6,-0.584615384615384,-0.569230769230769,
-0.553846153846154,-0.538461538461538,-0.523076923076923,-0.507692307692308,
-0.492307692307692,-0.476923076923077,-0.461538461538462,-0.446153846153846,
-0.430769230769231,-0.415384615384615,-0.4,-0.384615384615385,-0.369230769230769,
-0.353846153846154,-0.338461538461538,-0.323076923076923,-0.307692307692308,
-0.292307692307692,-0.276923076923077,-0.261538461538462,-0.246153846153846,
-0.230769230769231,-0.215384615384615,-0.2,-0.184615384615385,-0.169230769230769,
-0.153846153846154,-0.138461538461538,-0.123076923076923,-0.107692307692308,
-0.0923076923076923,-0.0769230769230769,-0.0615384615384615,-0.0461538461538462,
-0.0307692307692308,-0.0153846153846154,-0.00577184337452512),
 .UNSPECIFIED.)
CURVE()
GEOMETRIC_REPRESENTATION_ITEM()
RATIONAL_B_SPLINE_CURVE((1.,1.,1.,1.,1.,1.,1.,1.,1.,1.,1.,1.,1.,1.,1.,1.,
1.,1.,1.,1.,1.,1.,1.,1.,1.,1.,1.,1.,1.,1.,1.,1.,1.,1.,1.,1.,1.,1.,1.,1.,
1.,1.,1.,1.,1.,1.,1.,1.,1.,1.,1.,1.,1.,1.,1.,1.,1.,1.,1.,1.,1.,1.,1.,1.,
1.,1.,1.,1.,1.,1.))
REPRESENTATION_ITEM('')
);
#450=(
BOUNDED_CURVE()
B_SPLINE_CURVE(5,(#64244,#64245,#64246,#64247,#64248,#64249,#64250,#64251,
#64252,#64253,#64254,#64255,#64256,#64257,#64258,#64259,#64260,#64261,#64262,
#64263,#64264,#64265,#64266,#64267,#64268,#64269,#64270,#64271,#64272,#64273,
#64274,#64275,#64276,#64277,#64278,#64279,#64280,#64281,#64282,#64283,#64284,
#64285,#64286,#64287,#64288,#64289,#64290,#64291,#64292,#64293,#64294,#64295,
#64296,#64297,#64298,#64299,#64300,#64301,#64302,#64303,#64304,#64305,#64306,
#64307,#64308,#64309,#64310,#64311,#64312,#64313),.UNSPECIFIED.,.F.,.F.)
B_SPLINE_CURVE_WITH_KNOTS((6,1,1,1,1,1,1,1,1,1,1,1,1,1,1,1,1,1,1,1,1,1,
1,1,1,1,1,1,1,1,1,1,1,1,1,1,1,1,1,1,1,1,1,1,1,1,1,1,1,1,1,1,1,1,1,1,1,1,
1,1,1,1,1,1,1,6),(-0.994228156739713,-0.984615384615383,-0.969230769230768,
-0.953846153846152,-0.938461538461537,-0.923076923076922,-0.907692307692306,
-0.892307692307691,-0.876923076923076,-0.86153846153846,-0.846153846153845,
-0.83076923076923,-0.815384615384614,-0.799999999999999,-0.784615384615384,
-0.769230769230768,-0.753846153846153,-0.738461538461538,-0.723076923076922,
-0.707692307692307,-0.692307692307692,-0.676923076923076,-0.661538461538461,
-0.646153846153846,-0.63076923076923,-0.615384615384615,-0.6,-0.584615384615384,
-0.569230769230769,-0.553846153846154,-0.538461538461538,-0.523076923076923,
-0.507692307692308,-0.492307692307692,-0.476923076923077,-0.461538461538462,
-0.446153846153846,-0.430769230769231,-0.415384615384615,-0.4,-0.384615384615385,
-0.369230769230769,-0.353846153846154,-0.338461538461538,-0.323076923076923,
-0.307692307692308,-0.292307692307692,-0.276923076923077,-0.261538461538462,
-0.246153846153846,-0.230769230769231,-0.215384615384615,-0.2,-0.184615384615385,
-0.169230769230769,-0.153846153846154,-0.138461538461538,-0.123076923076923,
-0.107692307692308,-0.0923076923076923,-0.0769230769230769,-0.0615384615384615,
-0.0461538461538462,-0.0307692307692308,-0.0153846153846154,0.),
 .UNSPECIFIED.)
CURVE()
GEOMETRIC_REPRESENTATION_ITEM()
RATIONAL_B_SPLINE_CURVE((1.,1.,1.,1.,1.,1.,1.,1.,1.,1.,1.,1.,1.,1.,1.,1.,
1.,1.,1.,1.,1.,1.,1.,1.,1.,1.,1.,1.,1.,1.,1.,1.,1.,1.,1.,1.,1.,1.,1.,1.,
1.,1.,1.,1.,1.,1.,1.,1.,1.,1.,1.,1.,1.,1.,1.,1.,1.,1.,1.,1.,1.,1.,1.,1.,
1.,1.,1.,1.,1.,1.))
REPRESENTATION_ITEM('')
);
#451=(
BOUNDED_CURVE()
B_SPLINE_CURVE(5,(#64466,#64467,#64468,#64469,#64470,#64471,#64472,#64473,
#64474,#64475,#64476,#64477,#64478,#64479,#64480,#64481,#64482,#64483,#64484,
#64485,#64486,#64487,#64488,#64489,#64490,#64491,#64492,#64493,#64494,#64495,
#64496,#64497,#64498,#64499,#64500,#64501,#64502,#64503,#64504,#64505,#64506,
#64507,#64508,#64509,#64510,#64511,#64512,#64513,#64514,#64515,#64516,#64517,
#64518,#64519,#64520,#64521,#64522,#64523,#64524,#64525,#64526,#64527,#64528,
#64529,#64530,#64531,#64532,#64533,#64534,#64535),.UNSPECIFIED.,.F.,.F.)
B_SPLINE_CURVE_WITH_KNOTS((6,1,1,1,1,1,1,1,1,1,1,1,1,1,1,1,1,1,1,1,1,1,
1,1,1,1,1,1,1,1,1,1,1,1,1,1,1,1,1,1,1,1,1,1,1,1,1,1,1,1,1,1,1,1,1,1,1,1,
1,1,1,1,1,1,1,6),(-1.,-0.984615384615383,-0.969230769230768,-0.953846153846152,
-0.938461538461537,-0.923076923076922,-0.907692307692306,-0.892307692307691,
-0.876923076923076,-0.86153846153846,-0.846153846153845,-0.83076923076923,
-0.815384615384614,-0.799999999999999,-0.784615384615384,-0.769230769230768,
-0.753846153846153,-0.738461538461538,-0.723076923076922,-0.707692307692307,
-0.692307692307692,-0.676923076923076,-0.661538461538461,-0.646153846153846,
-0.63076923076923,-0.615384615384615,-0.6,-0.584615384615384,-0.569230769230769,
-0.553846153846154,-0.538461538461538,-0.523076923076923,-0.507692307692308,
-0.492307692307692,-0.476923076923077,-0.461538461538462,-0.446153846153846,
-0.430769230769231,-0.415384615384615,-0.4,-0.384615384615385,-0.369230769230769,
-0.353846153846154,-0.338461538461538,-0.323076923076923,-0.307692307692308,
-0.292307692307692,-0.276923076923077,-0.261538461538462,-0.246153846153846,
-0.230769230769231,-0.215384615384615,-0.2,-0.184615384615385,-0.169230769230769,
-0.153846153846154,-0.138461538461538,-0.123076923076923,-0.107692307692308,
-0.0923076923076923,-0.0769230769230769,-0.0615384615384615,-0.0461538461538462,
-0.0307692307692308,-0.0153846153846154,-0.00577184337450204),
 .UNSPECIFIED.)
CURVE()
GEOMETRIC_REPRESENTATION_ITEM()
RATIONAL_B_SPLINE_CURVE((1.,1.,1.,1.,1.,1.,1.,1.,1.,1.,1.,1.,1.,1.,1.,1.,
1.,1.,1.,1.,1.,1.,1.,1.,1.,1.,1.,1.,1.,1.,1.,1.,1.,1.,1.,1.,1.,1.,1.,1.,
1.,1.,1.,1.,1.,1.,1.,1.,1.,1.,1.,1.,1.,1.,1.,1.,1.,1.,1.,1.,1.,1.,1.,1.,
1.,1.,1.,1.,1.,1.))
REPRESENTATION_ITEM('')
);
#452=(
BOUNDED_CURVE()
B_SPLINE_CURVE(5,(#64686,#64687,#64688,#64689,#64690,#64691,#64692,#64693,
#64694,#64695,#64696,#64697,#64698,#64699,#64700,#64701,#64702,#64703,#64704,
#64705,#64706,#64707,#64708,#64709,#64710,#64711,#64712,#64713,#64714,#64715,
#64716,#64717,#64718,#64719,#64720,#64721,#64722,#64723,#64724,#64725,#64726,
#64727,#64728,#64729,#64730,#64731,#64732,#64733,#64734,#64735,#64736,#64737,
#64738,#64739,#64740,#64741,#64742,#64743,#64744,#64745,#64746,#64747,#64748,
#64749,#64750,#64751,#64752,#64753,#64754,#64755),.UNSPECIFIED.,.F.,.F.)
B_SPLINE_CURVE_WITH_KNOTS((6,1,1,1,1,1,1,1,1,1,1,1,1,1,1,1,1,1,1,1,1,1,
1,1,1,1,1,1,1,1,1,1,1,1,1,1,1,1,1,1,1,1,1,1,1,1,1,1,1,1,1,1,1,1,1,1,1,1,
1,1,1,1,1,1,1,6),(-0.99422815673972,-0.984615384615383,-0.969230769230768,
-0.953846153846152,-0.938461538461537,-0.923076923076922,-0.907692307692306,
-0.892307692307691,-0.876923076923076,-0.86153846153846,-0.846153846153845,
-0.83076923076923,-0.815384615384614,-0.799999999999999,-0.784615384615384,
-0.769230769230768,-0.753846153846153,-0.738461538461538,-0.723076923076922,
-0.707692307692307,-0.692307692307692,-0.676923076923076,-0.661538461538461,
-0.646153846153846,-0.63076923076923,-0.615384615384615,-0.6,-0.584615384615384,
-0.569230769230769,-0.553846153846154,-0.538461538461538,-0.523076923076923,
-0.507692307692308,-0.492307692307692,-0.476923076923077,-0.461538461538462,
-0.446153846153846,-0.430769230769231,-0.415384615384615,-0.4,-0.384615384615385,
-0.369230769230769,-0.353846153846154,-0.338461538461538,-0.323076923076923,
-0.307692307692308,-0.292307692307692,-0.276923076923077,-0.261538461538462,
-0.246153846153846,-0.230769230769231,-0.215384615384615,-0.2,-0.184615384615385,
-0.169230769230769,-0.153846153846154,-0.138461538461538,-0.123076923076923,
-0.107692307692308,-0.0923076923076923,-0.0769230769230769,-0.0615384615384615,
-0.0461538461538462,-0.0307692307692308,-0.0153846153846154,0.),
 .UNSPECIFIED.)
CURVE()
GEOMETRIC_REPRESENTATION_ITEM()
RATIONAL_B_SPLINE_CURVE((1.,1.,1.,1.,1.,1.,1.,1.,1.,1.,1.,1.,1.,1.,1.,1.,
1.,1.,1.,1.,1.,1.,1.,1.,1.,1.,1.,1.,1.,1.,1.,1.,1.,1.,1.,1.,1.,1.,1.,1.,
1.,1.,1.,1.,1.,1.,1.,1.,1.,1.,1.,1.,1.,1.,1.,1.,1.,1.,1.,1.,1.,1.,1.,1.,
1.,1.,1.,1.,1.,1.))
REPRESENTATION_ITEM('')
);
#453=(
BOUNDED_CURVE()
B_SPLINE_CURVE(5,(#64908,#64909,#64910,#64911,#64912,#64913,#64914,#64915,
#64916,#64917,#64918,#64919,#64920,#64921,#64922,#64923,#64924,#64925,#64926,
#64927,#64928,#64929,#64930,#64931,#64932,#64933,#64934,#64935,#64936,#64937,
#64938,#64939,#64940,#64941,#64942,#64943,#64944,#64945,#64946,#64947,#64948,
#64949,#64950,#64951,#64952,#64953,#64954,#64955,#64956,#64957,#64958,#64959,
#64960,#64961,#64962,#64963,#64964,#64965,#64966,#64967,#64968,#64969,#64970,
#64971,#64972,#64973,#64974,#64975,#64976,#64977),.UNSPECIFIED.,.F.,.F.)
B_SPLINE_CURVE_WITH_KNOTS((6,1,1,1,1,1,1,1,1,1,1,1,1,1,1,1,1,1,1,1,1,1,
1,1,1,1,1,1,1,1,1,1,1,1,1,1,1,1,1,1,1,1,1,1,1,1,1,1,1,1,1,1,1,1,1,1,1,1,
1,1,1,1,1,1,1,6),(-1.,-0.984615384615383,-0.969230769230768,-0.953846153846152,
-0.938461538461537,-0.923076923076922,-0.907692307692306,-0.892307692307691,
-0.876923076923076,-0.86153846153846,-0.846153846153845,-0.83076923076923,
-0.815384615384614,-0.799999999999999,-0.784615384615384,-0.769230769230768,
-0.753846153846153,-0.738461538461538,-0.723076923076922,-0.707692307692307,
-0.692307692307692,-0.676923076923076,-0.661538461538461,-0.646153846153846,
-0.63076923076923,-0.615384615384615,-0.6,-0.584615384615384,-0.569230769230769,
-0.553846153846154,-0.538461538461538,-0.523076923076923,-0.507692307692308,
-0.492307692307692,-0.476923076923077,-0.461538461538462,-0.446153846153846,
-0.430769230769231,-0.415384615384615,-0.4,-0.384615384615385,-0.369230769230769,
-0.353846153846154,-0.338461538461538,-0.323076923076923,-0.307692307692308,
-0.292307692307692,-0.276923076923077,-0.261538461538462,-0.246153846153846,
-0.230769230769231,-0.215384615384615,-0.2,-0.184615384615385,-0.169230769230769,
-0.153846153846154,-0.138461538461538,-0.123076923076923,-0.107692307692308,
-0.0923076923076923,-0.0769230769230769,-0.0615384615384615,-0.0461538461538462,
-0.0307692307692308,-0.0153846153846154,-0.0057718433745107),
 .UNSPECIFIED.)
CURVE()
GEOMETRIC_REPRESENTATION_ITEM()
RATIONAL_B_SPLINE_CURVE((1.,1.,1.,1.,1.,1.,1.,1.,1.,1.,1.,1.,1.,1.,1.,1.,
1.,1.,1.,1.,1.,1.,1.,1.,1.,1.,1.,1.,1.,1.,1.,1.,1.,1.,1.,1.,1.,1.,1.,1.,
1.,1.,1.,1.,1.,1.,1.,1.,1.,1.,1.,1.,1.,1.,1.,1.,1.,1.,1.,1.,1.,1.,1.,1.,
1.,1.,1.,1.,1.,1.))
REPRESENTATION_ITEM('')
);
#454=(
BOUNDED_CURVE()
B_SPLINE_CURVE(5,(#65128,#65129,#65130,#65131,#65132,#65133,#65134,#65135,
#65136,#65137,#65138,#65139,#65140,#65141,#65142,#65143,#65144,#65145,#65146,
#65147,#65148,#65149,#65150,#65151,#65152,#65153,#65154,#65155,#65156,#65157,
#65158,#65159,#65160,#65161,#65162,#65163,#65164,#65165,#65166,#65167,#65168,
#65169,#65170,#65171,#65172,#65173,#65174,#65175,#65176,#65177,#65178,#65179,
#65180,#65181,#65182,#65183,#65184,#65185,#65186,#65187,#65188,#65189,#65190,
#65191,#65192,#65193,#65194,#65195,#65196,#65197),.UNSPECIFIED.,.F.,.F.)
B_SPLINE_CURVE_WITH_KNOTS((6,1,1,1,1,1,1,1,1,1,1,1,1,1,1,1,1,1,1,1,1,1,
1,1,1,1,1,1,1,1,1,1,1,1,1,1,1,1,1,1,1,1,1,1,1,1,1,1,1,1,1,1,1,1,1,1,1,1,
1,1,1,1,1,1,1,6),(-0.994228156739708,-0.984615384615383,-0.969230769230768,
-0.953846153846152,-0.938461538461537,-0.923076923076922,-0.907692307692306,
-0.892307692307691,-0.876923076923076,-0.86153846153846,-0.846153846153845,
-0.83076923076923,-0.815384615384614,-0.799999999999999,-0.784615384615384,
-0.769230769230768,-0.753846153846153,-0.738461538461538,-0.723076923076922,
-0.707692307692307,-0.692307692307692,-0.676923076923076,-0.661538461538461,
-0.646153846153846,-0.63076923076923,-0.615384615384615,-0.6,-0.584615384615384,
-0.569230769230769,-0.553846153846154,-0.538461538461538,-0.523076923076923,
-0.507692307692308,-0.492307692307692,-0.476923076923077,-0.461538461538462,
-0.446153846153846,-0.430769230769231,-0.415384615384615,-0.4,-0.384615384615385,
-0.369230769230769,-0.353846153846154,-0.338461538461538,-0.323076923076923,
-0.307692307692308,-0.292307692307692,-0.276923076923077,-0.261538461538462,
-0.246153846153846,-0.230769230769231,-0.215384615384615,-0.2,-0.184615384615385,
-0.169230769230769,-0.153846153846154,-0.138461538461538,-0.123076923076923,
-0.107692307692308,-0.0923076923076923,-0.0769230769230769,-0.0615384615384615,
-0.0461538461538462,-0.0307692307692308,-0.0153846153846154,0.),
 .UNSPECIFIED.)
CURVE()
GEOMETRIC_REPRESENTATION_ITEM()
RATIONAL_B_SPLINE_CURVE((1.,1.,1.,1.,1.,1.,1.,1.,1.,1.,1.,1.,1.,1.,1.,1.,
1.,1.,1.,1.,1.,1.,1.,1.,1.,1.,1.,1.,1.,1.,1.,1.,1.,1.,1.,1.,1.,1.,1.,1.,
1.,1.,1.,1.,1.,1.,1.,1.,1.,1.,1.,1.,1.,1.,1.,1.,1.,1.,1.,1.,1.,1.,1.,1.,
1.,1.,1.,1.,1.,1.))
REPRESENTATION_ITEM('')
);
#455=(
BOUNDED_CURVE()
B_SPLINE_CURVE(5,(#65350,#65351,#65352,#65353,#65354,#65355,#65356,#65357,
#65358,#65359,#65360,#65361,#65362,#65363,#65364,#65365,#65366,#65367,#65368,
#65369,#65370,#65371,#65372,#65373,#65374,#65375,#65376,#65377,#65378,#65379,
#65380,#65381,#65382,#65383,#65384,#65385,#65386,#65387,#65388,#65389,#65390,
#65391,#65392,#65393,#65394,#65395,#65396,#65397,#65398,#65399,#65400,#65401,
#65402,#65403,#65404,#65405,#65406,#65407,#65408,#65409,#65410,#65411,#65412,
#65413,#65414,#65415,#65416,#65417,#65418,#65419),.UNSPECIFIED.,.F.,.F.)
B_SPLINE_CURVE_WITH_KNOTS((6,1,1,1,1,1,1,1,1,1,1,1,1,1,1,1,1,1,1,1,1,1,
1,1,1,1,1,1,1,1,1,1,1,1,1,1,1,1,1,1,1,1,1,1,1,1,1,1,1,1,1,1,1,1,1,1,1,1,
1,1,1,1,1,1,1,6),(-1.,-0.984615384615383,-0.969230769230768,-0.953846153846152,
-0.938461538461537,-0.923076923076922,-0.907692307692306,-0.892307692307691,
-0.876923076923076,-0.86153846153846,-0.846153846153845,-0.83076923076923,
-0.815384615384614,-0.799999999999999,-0.784615384615384,-0.769230769230768,
-0.753846153846153,-0.738461538461538,-0.723076923076922,-0.707692307692307,
-0.692307692307692,-0.676923076923076,-0.661538461538461,-0.646153846153846,
-0.63076923076923,-0.615384615384615,-0.6,-0.584615384615384,-0.569230769230769,
-0.553846153846154,-0.538461538461538,-0.523076923076923,-0.507692307692308,
-0.492307692307692,-0.476923076923077,-0.461538461538462,-0.446153846153846,
-0.430769230769231,-0.415384615384615,-0.4,-0.384615384615385,-0.369230769230769,
-0.353846153846154,-0.338461538461538,-0.323076923076923,-0.307692307692308,
-0.292307692307692,-0.276923076923077,-0.261538461538462,-0.246153846153846,
-0.230769230769231,-0.215384615384615,-0.2,-0.184615384615385,-0.169230769230769,
-0.153846153846154,-0.138461538461538,-0.123076923076923,-0.107692307692308,
-0.0923076923076923,-0.0769230769230769,-0.0615384615384615,-0.0461538461538462,
-0.0307692307692308,-0.0153846153846154,-0.00577184337451708),
 .UNSPECIFIED.)
CURVE()
GEOMETRIC_REPRESENTATION_ITEM()
RATIONAL_B_SPLINE_CURVE((1.,1.,1.,1.,1.,1.,1.,1.,1.,1.,1.,1.,1.,1.,1.,1.,
1.,1.,1.,1.,1.,1.,1.,1.,1.,1.,1.,1.,1.,1.,1.,1.,1.,1.,1.,1.,1.,1.,1.,1.,
1.,1.,1.,1.,1.,1.,1.,1.,1.,1.,1.,1.,1.,1.,1.,1.,1.,1.,1.,1.,1.,1.,1.,1.,
1.,1.,1.,1.,1.,1.))
REPRESENTATION_ITEM('')
);
#456=(
BOUNDED_CURVE()
B_SPLINE_CURVE(5,(#65570,#65571,#65572,#65573,#65574,#65575,#65576,#65577,
#65578,#65579,#65580,#65581,#65582,#65583,#65584,#65585,#65586,#65587,#65588,
#65589,#65590,#65591,#65592,#65593,#65594,#65595,#65596,#65597,#65598,#65599,
#65600,#65601,#65602,#65603,#65604,#65605,#65606,#65607,#65608,#65609,#65610,
#65611,#65612,#65613,#65614,#65615,#65616,#65617,#65618,#65619,#65620,#65621,
#65622,#65623,#65624,#65625,#65626,#65627,#65628,#65629,#65630,#65631,#65632,
#65633,#65634,#65635,#65636,#65637,#65638,#65639),.UNSPECIFIED.,.F.,.F.)
B_SPLINE_CURVE_WITH_KNOTS((6,1,1,1,1,1,1,1,1,1,1,1,1,1,1,1,1,1,1,1,1,1,
1,1,1,1,1,1,1,1,1,1,1,1,1,1,1,1,1,1,1,1,1,1,1,1,1,1,1,1,1,1,1,1,1,1,1,1,
1,1,1,1,1,1,1,6),(-0.994228156739669,-0.984615384615383,-0.969230769230768,
-0.953846153846152,-0.938461538461537,-0.923076923076922,-0.907692307692306,
-0.892307692307691,-0.876923076923076,-0.86153846153846,-0.846153846153845,
-0.83076923076923,-0.815384615384614,-0.799999999999999,-0.784615384615384,
-0.769230769230768,-0.753846153846153,-0.738461538461538,-0.723076923076922,
-0.707692307692307,-0.692307692307692,-0.676923076923076,-0.661538461538461,
-0.646153846153846,-0.63076923076923,-0.615384615384615,-0.6,-0.584615384615384,
-0.569230769230769,-0.553846153846154,-0.538461538461538,-0.523076923076923,
-0.507692307692308,-0.492307692307692,-0.476923076923077,-0.461538461538462,
-0.446153846153846,-0.430769230769231,-0.415384615384615,-0.4,-0.384615384615385,
-0.369230769230769,-0.353846153846154,-0.338461538461538,-0.323076923076923,
-0.307692307692308,-0.292307692307692,-0.276923076923077,-0.261538461538462,
-0.246153846153846,-0.230769230769231,-0.215384615384615,-0.2,-0.184615384615385,
-0.169230769230769,-0.153846153846154,-0.138461538461538,-0.123076923076923,
-0.107692307692308,-0.0923076923076923,-0.0769230769230769,-0.0615384615384615,
-0.0461538461538462,-0.0307692307692308,-0.0153846153846154,0.),
 .UNSPECIFIED.)
CURVE()
GEOMETRIC_REPRESENTATION_ITEM()
RATIONAL_B_SPLINE_CURVE((1.,1.,1.,1.,1.,1.,1.,1.,1.,1.,1.,1.,1.,1.,1.,1.,
1.,1.,1.,1.,1.,1.,1.,1.,1.,1.,1.,1.,1.,1.,1.,1.,1.,1.,1.,1.,1.,1.,1.,1.,
1.,1.,1.,1.,1.,1.,1.,1.,1.,1.,1.,1.,1.,1.,1.,1.,1.,1.,1.,1.,1.,1.,1.,1.,
1.,1.,1.,1.,1.,1.))
REPRESENTATION_ITEM('')
);
#457=(
BOUNDED_CURVE()
B_SPLINE_CURVE(5,(#65792,#65793,#65794,#65795,#65796,#65797,#65798,#65799,
#65800,#65801,#65802,#65803,#65804,#65805,#65806,#65807,#65808,#65809,#65810,
#65811,#65812,#65813,#65814,#65815,#65816,#65817,#65818,#65819,#65820,#65821,
#65822,#65823,#65824,#65825,#65826,#65827,#65828,#65829,#65830,#65831,#65832,
#65833,#65834,#65835,#65836,#65837,#65838,#65839,#65840,#65841,#65842,#65843,
#65844,#65845,#65846,#65847,#65848,#65849,#65850,#65851,#65852,#65853,#65854,
#65855,#65856,#65857,#65858,#65859,#65860,#65861),.UNSPECIFIED.,.F.,.F.)
B_SPLINE_CURVE_WITH_KNOTS((6,1,1,1,1,1,1,1,1,1,1,1,1,1,1,1,1,1,1,1,1,1,
1,1,1,1,1,1,1,1,1,1,1,1,1,1,1,1,1,1,1,1,1,1,1,1,1,1,1,1,1,1,1,1,1,1,1,1,
1,1,1,1,1,1,1,6),(-1.,-0.984615384615383,-0.969230769230768,-0.953846153846152,
-0.938461538461537,-0.923076923076922,-0.907692307692306,-0.892307692307691,
-0.876923076923076,-0.86153846153846,-0.846153846153845,-0.83076923076923,
-0.815384615384614,-0.799999999999999,-0.784615384615384,-0.769230769230768,
-0.753846153846153,-0.738461538461538,-0.723076923076922,-0.707692307692307,
-0.692307692307692,-0.676923076923076,-0.661538461538461,-0.646153846153846,
-0.63076923076923,-0.615384615384615,-0.6,-0.584615384615384,-0.569230769230769,
-0.553846153846154,-0.538461538461538,-0.523076923076923,-0.507692307692308,
-0.492307692307692,-0.476923076923077,-0.461538461538462,-0.446153846153846,
-0.430769230769231,-0.415384615384615,-0.4,-0.384615384615385,-0.369230769230769,
-0.353846153846154,-0.338461538461538,-0.323076923076923,-0.307692307692308,
-0.292307692307692,-0.276923076923077,-0.261538461538462,-0.246153846153846,
-0.230769230769231,-0.215384615384615,-0.2,-0.184615384615385,-0.169230769230769,
-0.153846153846154,-0.138461538461538,-0.123076923076923,-0.107692307692308,
-0.0923076923076923,-0.0769230769230769,-0.0615384615384615,-0.0461538461538462,
-0.0307692307692308,-0.0153846153846154,-0.0057718433744903),
 .UNSPECIFIED.)
CURVE()
GEOMETRIC_REPRESENTATION_ITEM()
RATIONAL_B_SPLINE_CURVE((1.,1.,1.,1.,1.,1.,1.,1.,1.,1.,1.,1.,1.,1.,1.,1.,
1.,1.,1.,1.,1.,1.,1.,1.,1.,1.,1.,1.,1.,1.,1.,1.,1.,1.,1.,1.,1.,1.,1.,1.,
1.,1.,1.,1.,1.,1.,1.,1.,1.,1.,1.,1.,1.,1.,1.,1.,1.,1.,1.,1.,1.,1.,1.,1.,
1.,1.,1.,1.,1.,1.))
REPRESENTATION_ITEM('')
);
#458=(
BOUNDED_CURVE()
B_SPLINE_CURVE(5,(#66012,#66013,#66014,#66015,#66016,#66017,#66018,#66019,
#66020,#66021,#66022,#66023,#66024,#66025,#66026,#66027,#66028,#66029,#66030,
#66031,#66032,#66033,#66034,#66035,#66036,#66037,#66038,#66039,#66040,#66041,
#66042,#66043,#66044,#66045,#66046,#66047,#66048,#66049,#66050,#66051,#66052,
#66053,#66054,#66055,#66056,#66057,#66058,#66059,#66060,#66061,#66062,#66063,
#66064,#66065,#66066,#66067,#66068,#66069,#66070,#66071,#66072,#66073,#66074,
#66075,#66076,#66077,#66078,#66079,#66080,#66081),.UNSPECIFIED.,.F.,.F.)
B_SPLINE_CURVE_WITH_KNOTS((6,1,1,1,1,1,1,1,1,1,1,1,1,1,1,1,1,1,1,1,1,1,
1,1,1,1,1,1,1,1,1,1,1,1,1,1,1,1,1,1,1,1,1,1,1,1,1,1,1,1,1,1,1,1,1,1,1,1,
1,1,1,1,1,1,1,6),(-0.994228156739712,-0.984615384615383,-0.969230769230768,
-0.953846153846152,-0.938461538461537,-0.923076923076922,-0.907692307692306,
-0.892307692307691,-0.876923076923076,-0.86153846153846,-0.846153846153845,
-0.83076923076923,-0.815384615384614,-0.799999999999999,-0.784615384615384,
-0.769230769230768,-0.753846153846153,-0.738461538461538,-0.723076923076922,
-0.707692307692307,-0.692307692307692,-0.676923076923076,-0.661538461538461,
-0.646153846153846,-0.63076923076923,-0.615384615384615,-0.6,-0.584615384615384,
-0.569230769230769,-0.553846153846154,-0.538461538461538,-0.523076923076923,
-0.507692307692308,-0.492307692307692,-0.476923076923077,-0.461538461538462,
-0.446153846153846,-0.430769230769231,-0.415384615384615,-0.4,-0.384615384615385,
-0.369230769230769,-0.353846153846154,-0.338461538461538,-0.323076923076923,
-0.307692307692308,-0.292307692307692,-0.276923076923077,-0.261538461538462,
-0.246153846153846,-0.230769230769231,-0.215384615384615,-0.2,-0.184615384615385,
-0.169230769230769,-0.153846153846154,-0.138461538461538,-0.123076923076923,
-0.107692307692308,-0.0923076923076923,-0.0769230769230769,-0.0615384615384615,
-0.0461538461538462,-0.0307692307692308,-0.0153846153846154,0.),
 .UNSPECIFIED.)
CURVE()
GEOMETRIC_REPRESENTATION_ITEM()
RATIONAL_B_SPLINE_CURVE((1.,1.,1.,1.,1.,1.,1.,1.,1.,1.,1.,1.,1.,1.,1.,1.,
1.,1.,1.,1.,1.,1.,1.,1.,1.,1.,1.,1.,1.,1.,1.,1.,1.,1.,1.,1.,1.,1.,1.,1.,
1.,1.,1.,1.,1.,1.,1.,1.,1.,1.,1.,1.,1.,1.,1.,1.,1.,1.,1.,1.,1.,1.,1.,1.,
1.,1.,1.,1.,1.,1.))
REPRESENTATION_ITEM('')
);
#459=(
BOUNDED_CURVE()
B_SPLINE_CURVE(5,(#66234,#66235,#66236,#66237,#66238,#66239,#66240,#66241,
#66242,#66243,#66244,#66245,#66246,#66247,#66248,#66249,#66250,#66251,#66252,
#66253,#66254,#66255,#66256,#66257,#66258,#66259,#66260,#66261,#66262,#66263,
#66264,#66265,#66266,#66267,#66268,#66269,#66270,#66271,#66272,#66273,#66274,
#66275,#66276,#66277,#66278,#66279,#66280,#66281,#66282,#66283,#66284,#66285,
#66286,#66287,#66288,#66289,#66290,#66291,#66292,#66293,#66294,#66295,#66296,
#66297,#66298,#66299,#66300,#66301,#66302,#66303),.UNSPECIFIED.,.F.,.F.)
B_SPLINE_CURVE_WITH_KNOTS((6,1,1,1,1,1,1,1,1,1,1,1,1,1,1,1,1,1,1,1,1,1,
1,1,1,1,1,1,1,1,1,1,1,1,1,1,1,1,1,1,1,1,1,1,1,1,1,1,1,1,1,1,1,1,1,1,1,1,
1,1,1,1,1,1,1,6),(-1.,-0.984615384615383,-0.969230769230768,-0.953846153846152,
-0.938461538461537,-0.923076923076922,-0.907692307692306,-0.892307692307691,
-0.876923076923076,-0.86153846153846,-0.846153846153845,-0.83076923076923,
-0.815384615384614,-0.799999999999999,-0.784615384615384,-0.769230769230768,
-0.753846153846153,-0.738461538461538,-0.723076923076922,-0.707692307692307,
-0.692307692307692,-0.676923076923076,-0.661538461538461,-0.646153846153846,
-0.63076923076923,-0.615384615384615,-0.6,-0.584615384615384,-0.569230769230769,
-0.553846153846154,-0.538461538461538,-0.523076923076923,-0.507692307692308,
-0.492307692307692,-0.476923076923077,-0.461538461538462,-0.446153846153846,
-0.430769230769231,-0.415384615384615,-0.4,-0.384615384615385,-0.369230769230769,
-0.353846153846154,-0.338461538461538,-0.323076923076923,-0.307692307692308,
-0.292307692307692,-0.276923076923077,-0.261538461538462,-0.246153846153846,
-0.230769230769231,-0.215384615384615,-0.2,-0.184615384615385,-0.169230769230769,
-0.153846153846154,-0.138461538461538,-0.123076923076923,-0.107692307692308,
-0.0923076923076923,-0.0769230769230769,-0.0615384615384615,-0.0461538461538462,
-0.0307692307692308,-0.0153846153846154,-0.0057718433745291),
 .UNSPECIFIED.)
CURVE()
GEOMETRIC_REPRESENTATION_ITEM()
RATIONAL_B_SPLINE_CURVE((1.,1.,1.,1.,1.,1.,1.,1.,1.,1.,1.,1.,1.,1.,1.,1.,
1.,1.,1.,1.,1.,1.,1.,1.,1.,1.,1.,1.,1.,1.,1.,1.,1.,1.,1.,1.,1.,1.,1.,1.,
1.,1.,1.,1.,1.,1.,1.,1.,1.,1.,1.,1.,1.,1.,1.,1.,1.,1.,1.,1.,1.,1.,1.,1.,
1.,1.,1.,1.,1.,1.))
REPRESENTATION_ITEM('')
);
#460=(
BOUNDED_CURVE()
B_SPLINE_CURVE(5,(#66454,#66455,#66456,#66457,#66458,#66459,#66460,#66461,
#66462,#66463,#66464,#66465,#66466,#66467,#66468,#66469,#66470,#66471,#66472,
#66473,#66474,#66475,#66476,#66477,#66478,#66479,#66480,#66481,#66482,#66483,
#66484,#66485,#66486,#66487,#66488,#66489,#66490,#66491,#66492,#66493,#66494,
#66495,#66496,#66497,#66498,#66499,#66500,#66501,#66502,#66503,#66504,#66505,
#66506,#66507,#66508,#66509,#66510,#66511,#66512,#66513,#66514,#66515,#66516,
#66517,#66518,#66519,#66520,#66521,#66522,#66523),.UNSPECIFIED.,.F.,.F.)
B_SPLINE_CURVE_WITH_KNOTS((6,1,1,1,1,1,1,1,1,1,1,1,1,1,1,1,1,1,1,1,1,1,
1,1,1,1,1,1,1,1,1,1,1,1,1,1,1,1,1,1,1,1,1,1,1,1,1,1,1,1,1,1,1,1,1,1,1,1,
1,1,1,1,1,1,1,6),(-0.994228156739695,-0.984615384615383,-0.969230769230768,
-0.953846153846152,-0.938461538461537,-0.923076923076922,-0.907692307692306,
-0.892307692307691,-0.876923076923076,-0.86153846153846,-0.846153846153845,
-0.83076923076923,-0.815384615384614,-0.799999999999999,-0.784615384615384,
-0.769230769230768,-0.753846153846153,-0.738461538461538,-0.723076923076922,
-0.707692307692307,-0.692307692307692,-0.676923076923076,-0.661538461538461,
-0.646153846153846,-0.63076923076923,-0.615384615384615,-0.6,-0.584615384615384,
-0.569230769230769,-0.553846153846154,-0.538461538461538,-0.523076923076923,
-0.507692307692308,-0.492307692307692,-0.476923076923077,-0.461538461538462,
-0.446153846153846,-0.430769230769231,-0.415384615384615,-0.4,-0.384615384615385,
-0.369230769230769,-0.353846153846154,-0.338461538461538,-0.323076923076923,
-0.307692307692308,-0.292307692307692,-0.276923076923077,-0.261538461538462,
-0.246153846153846,-0.230769230769231,-0.215384615384615,-0.2,-0.184615384615385,
-0.169230769230769,-0.153846153846154,-0.138461538461538,-0.123076923076923,
-0.107692307692308,-0.0923076923076923,-0.0769230769230769,-0.0615384615384615,
-0.0461538461538462,-0.0307692307692308,-0.0153846153846154,0.),
 .UNSPECIFIED.)
CURVE()
GEOMETRIC_REPRESENTATION_ITEM()
RATIONAL_B_SPLINE_CURVE((1.,1.,1.,1.,1.,1.,1.,1.,1.,1.,1.,1.,1.,1.,1.,1.,
1.,1.,1.,1.,1.,1.,1.,1.,1.,1.,1.,1.,1.,1.,1.,1.,1.,1.,1.,1.,1.,1.,1.,1.,
1.,1.,1.,1.,1.,1.,1.,1.,1.,1.,1.,1.,1.,1.,1.,1.,1.,1.,1.,1.,1.,1.,1.,1.,
1.,1.,1.,1.,1.,1.))
REPRESENTATION_ITEM('')
);
#461=(
BOUNDED_CURVE()
B_SPLINE_CURVE(5,(#66676,#66677,#66678,#66679,#66680,#66681,#66682,#66683,
#66684,#66685,#66686,#66687,#66688,#66689,#66690,#66691,#66692,#66693,#66694,
#66695,#66696,#66697,#66698,#66699,#66700,#66701,#66702,#66703,#66704,#66705,
#66706,#66707,#66708,#66709,#66710,#66711,#66712,#66713,#66714,#66715,#66716,
#66717,#66718,#66719,#66720,#66721,#66722,#66723,#66724,#66725,#66726,#66727,
#66728,#66729,#66730,#66731,#66732,#66733,#66734,#66735,#66736,#66737,#66738,
#66739,#66740,#66741,#66742,#66743,#66744,#66745),.UNSPECIFIED.,.F.,.F.)
B_SPLINE_CURVE_WITH_KNOTS((6,1,1,1,1,1,1,1,1,1,1,1,1,1,1,1,1,1,1,1,1,1,
1,1,1,1,1,1,1,1,1,1,1,1,1,1,1,1,1,1,1,1,1,1,1,1,1,1,1,1,1,1,1,1,1,1,1,1,
1,1,1,1,1,1,1,6),(-1.,-0.984615384615383,-0.969230769230768,-0.953846153846152,
-0.938461538461537,-0.923076923076922,-0.907692307692306,-0.892307692307691,
-0.876923076923076,-0.86153846153846,-0.846153846153845,-0.83076923076923,
-0.815384615384614,-0.799999999999999,-0.784615384615384,-0.769230769230768,
-0.753846153846153,-0.738461538461538,-0.723076923076922,-0.707692307692307,
-0.692307692307692,-0.676923076923076,-0.661538461538461,-0.646153846153846,
-0.63076923076923,-0.615384615384615,-0.6,-0.584615384615384,-0.569230769230769,
-0.553846153846154,-0.538461538461538,-0.523076923076923,-0.507692307692308,
-0.492307692307692,-0.476923076923077,-0.461538461538462,-0.446153846153846,
-0.430769230769231,-0.415384615384615,-0.4,-0.384615384615385,-0.369230769230769,
-0.353846153846154,-0.338461538461538,-0.323076923076923,-0.307692307692308,
-0.292307692307692,-0.276923076923077,-0.261538461538462,-0.246153846153846,
-0.230769230769231,-0.215384615384615,-0.2,-0.184615384615385,-0.169230769230769,
-0.153846153846154,-0.138461538461538,-0.123076923076923,-0.107692307692308,
-0.0923076923076923,-0.0769230769230769,-0.0615384615384615,-0.0461538461538462,
-0.0307692307692308,-0.0153846153846154,-0.00577184337450344),
 .UNSPECIFIED.)
CURVE()
GEOMETRIC_REPRESENTATION_ITEM()
RATIONAL_B_SPLINE_CURVE((1.,1.,1.,1.,1.,1.,1.,1.,1.,1.,1.,1.,1.,1.,1.,1.,
1.,1.,1.,1.,1.,1.,1.,1.,1.,1.,1.,1.,1.,1.,1.,1.,1.,1.,1.,1.,1.,1.,1.,1.,
1.,1.,1.,1.,1.,1.,1.,1.,1.,1.,1.,1.,1.,1.,1.,1.,1.,1.,1.,1.,1.,1.,1.,1.,
1.,1.,1.,1.,1.,1.))
REPRESENTATION_ITEM('')
);
#462=(
BOUNDED_CURVE()
B_SPLINE_CURVE(5,(#66896,#66897,#66898,#66899,#66900,#66901,#66902,#66903,
#66904,#66905,#66906,#66907,#66908,#66909,#66910,#66911,#66912,#66913,#66914,
#66915,#66916,#66917,#66918,#66919,#66920,#66921,#66922,#66923,#66924,#66925,
#66926,#66927,#66928,#66929,#66930,#66931,#66932,#66933,#66934,#66935,#66936,
#66937,#66938,#66939,#66940,#66941,#66942,#66943,#66944,#66945,#66946,#66947,
#66948,#66949,#66950,#66951,#66952,#66953,#66954,#66955,#66956,#66957,#66958,
#66959,#66960,#66961,#66962,#66963,#66964,#66965),.UNSPECIFIED.,.F.,.F.)
B_SPLINE_CURVE_WITH_KNOTS((6,1,1,1,1,1,1,1,1,1,1,1,1,1,1,1,1,1,1,1,1,1,
1,1,1,1,1,1,1,1,1,1,1,1,1,1,1,1,1,1,1,1,1,1,1,1,1,1,1,1,1,1,1,1,1,1,1,1,
1,1,1,1,1,1,1,6),(-0.994228156739669,-0.984615384615383,-0.969230769230768,
-0.953846153846152,-0.938461538461537,-0.923076923076922,-0.907692307692306,
-0.892307692307691,-0.876923076923076,-0.86153846153846,-0.846153846153845,
-0.83076923076923,-0.815384615384614,-0.799999999999999,-0.784615384615384,
-0.769230769230768,-0.753846153846153,-0.738461538461538,-0.723076923076922,
-0.707692307692307,-0.692307692307692,-0.676923076923076,-0.661538461538461,
-0.646153846153846,-0.63076923076923,-0.615384615384615,-0.6,-0.584615384615384,
-0.569230769230769,-0.553846153846154,-0.538461538461538,-0.523076923076923,
-0.507692307692308,-0.492307692307692,-0.476923076923077,-0.461538461538462,
-0.446153846153846,-0.430769230769231,-0.415384615384615,-0.4,-0.384615384615385,
-0.369230769230769,-0.353846153846154,-0.338461538461538,-0.323076923076923,
-0.307692307692308,-0.292307692307692,-0.276923076923077,-0.261538461538462,
-0.246153846153846,-0.230769230769231,-0.215384615384615,-0.2,-0.184615384615385,
-0.169230769230769,-0.153846153846154,-0.138461538461538,-0.123076923076923,
-0.107692307692308,-0.0923076923076923,-0.0769230769230769,-0.0615384615384615,
-0.0461538461538462,-0.0307692307692308,-0.0153846153846154,0.),
 .UNSPECIFIED.)
CURVE()
GEOMETRIC_REPRESENTATION_ITEM()
RATIONAL_B_SPLINE_CURVE((1.,1.,1.,1.,1.,1.,1.,1.,1.,1.,1.,1.,1.,1.,1.,1.,
1.,1.,1.,1.,1.,1.,1.,1.,1.,1.,1.,1.,1.,1.,1.,1.,1.,1.,1.,1.,1.,1.,1.,1.,
1.,1.,1.,1.,1.,1.,1.,1.,1.,1.,1.,1.,1.,1.,1.,1.,1.,1.,1.,1.,1.,1.,1.,1.,
1.,1.,1.,1.,1.,1.))
REPRESENTATION_ITEM('')
);
#463=(
BOUNDED_CURVE()
B_SPLINE_CURVE(5,(#67118,#67119,#67120,#67121,#67122,#67123,#67124,#67125,
#67126,#67127,#67128,#67129,#67130,#67131,#67132,#67133,#67134,#67135,#67136,
#67137,#67138,#67139,#67140,#67141,#67142,#67143,#67144,#67145,#67146,#67147,
#67148,#67149,#67150,#67151,#67152,#67153,#67154,#67155,#67156,#67157,#67158,
#67159,#67160,#67161,#67162,#67163,#67164,#67165,#67166,#67167,#67168,#67169,
#67170,#67171,#67172,#67173,#67174,#67175,#67176,#67177,#67178,#67179,#67180,
#67181,#67182,#67183,#67184,#67185,#67186,#67187),.UNSPECIFIED.,.F.,.F.)
B_SPLINE_CURVE_WITH_KNOTS((6,1,1,1,1,1,1,1,1,1,1,1,1,1,1,1,1,1,1,1,1,1,
1,1,1,1,1,1,1,1,1,1,1,1,1,1,1,1,1,1,1,1,1,1,1,1,1,1,1,1,1,1,1,1,1,1,1,1,
1,1,1,1,1,1,1,6),(-1.,-0.984615384615383,-0.969230769230768,-0.953846153846152,
-0.938461538461537,-0.923076923076922,-0.907692307692306,-0.892307692307691,
-0.876923076923076,-0.86153846153846,-0.846153846153845,-0.83076923076923,
-0.815384615384614,-0.799999999999999,-0.784615384615384,-0.769230769230768,
-0.753846153846153,-0.738461538461538,-0.723076923076922,-0.707692307692307,
-0.692307692307692,-0.676923076923076,-0.661538461538461,-0.646153846153846,
-0.63076923076923,-0.615384615384615,-0.6,-0.584615384615384,-0.569230769230769,
-0.553846153846154,-0.538461538461538,-0.523076923076923,-0.507692307692308,
-0.492307692307692,-0.476923076923077,-0.461538461538462,-0.446153846153846,
-0.430769230769231,-0.415384615384615,-0.4,-0.384615384615385,-0.369230769230769,
-0.353846153846154,-0.338461538461538,-0.323076923076923,-0.307692307692308,
-0.292307692307692,-0.276923076923077,-0.261538461538462,-0.246153846153846,
-0.230769230769231,-0.215384615384615,-0.2,-0.184615384615385,-0.169230769230769,
-0.153846153846154,-0.138461538461538,-0.123076923076923,-0.107692307692308,
-0.0923076923076923,-0.0769230769230769,-0.0615384615384615,-0.0461538461538462,
-0.0307692307692308,-0.0153846153846154,-0.00577184337450876),
 .UNSPECIFIED.)
CURVE()
GEOMETRIC_REPRESENTATION_ITEM()
RATIONAL_B_SPLINE_CURVE((1.,1.,1.,1.,1.,1.,1.,1.,1.,1.,1.,1.,1.,1.,1.,1.,
1.,1.,1.,1.,1.,1.,1.,1.,1.,1.,1.,1.,1.,1.,1.,1.,1.,1.,1.,1.,1.,1.,1.,1.,
1.,1.,1.,1.,1.,1.,1.,1.,1.,1.,1.,1.,1.,1.,1.,1.,1.,1.,1.,1.,1.,1.,1.,1.,
1.,1.,1.,1.,1.,1.))
REPRESENTATION_ITEM('')
);
#464=(
BOUNDED_CURVE()
B_SPLINE_CURVE(5,(#67338,#67339,#67340,#67341,#67342,#67343,#67344,#67345,
#67346,#67347,#67348,#67349,#67350,#67351,#67352,#67353,#67354,#67355,#67356,
#67357,#67358,#67359,#67360,#67361,#67362,#67363,#67364,#67365,#67366,#67367,
#67368,#67369,#67370,#67371,#67372,#67373,#67374,#67375,#67376,#67377,#67378,
#67379,#67380,#67381,#67382,#67383,#67384,#67385,#67386,#67387,#67388,#67389,
#67390,#67391,#67392,#67393,#67394,#67395,#67396,#67397,#67398,#67399,#67400,
#67401,#67402,#67403,#67404,#67405,#67406,#67407),.UNSPECIFIED.,.F.,.F.)
B_SPLINE_CURVE_WITH_KNOTS((6,1,1,1,1,1,1,1,1,1,1,1,1,1,1,1,1,1,1,1,1,1,
1,1,1,1,1,1,1,1,1,1,1,1,1,1,1,1,1,1,1,1,1,1,1,1,1,1,1,1,1,1,1,1,1,1,1,1,
1,1,1,1,1,1,1,6),(-0.99422815673966,-0.984615384615383,-0.969230769230768,
-0.953846153846152,-0.938461538461537,-0.923076923076922,-0.907692307692306,
-0.892307692307691,-0.876923076923076,-0.86153846153846,-0.846153846153845,
-0.83076923076923,-0.815384615384614,-0.799999999999999,-0.784615384615384,
-0.769230769230768,-0.753846153846153,-0.738461538461538,-0.723076923076922,
-0.707692307692307,-0.692307692307692,-0.676923076923076,-0.661538461538461,
-0.646153846153846,-0.63076923076923,-0.615384615384615,-0.6,-0.584615384615384,
-0.569230769230769,-0.553846153846154,-0.538461538461538,-0.523076923076923,
-0.507692307692308,-0.492307692307692,-0.476923076923077,-0.461538461538462,
-0.446153846153846,-0.430769230769231,-0.415384615384615,-0.4,-0.384615384615385,
-0.369230769230769,-0.353846153846154,-0.338461538461538,-0.323076923076923,
-0.307692307692308,-0.292307692307692,-0.276923076923077,-0.261538461538462,
-0.246153846153846,-0.230769230769231,-0.215384615384615,-0.2,-0.184615384615385,
-0.169230769230769,-0.153846153846154,-0.138461538461538,-0.123076923076923,
-0.107692307692308,-0.0923076923076923,-0.0769230769230769,-0.0615384615384615,
-0.0461538461538462,-0.0307692307692308,-0.0153846153846154,0.),
 .UNSPECIFIED.)
CURVE()
GEOMETRIC_REPRESENTATION_ITEM()
RATIONAL_B_SPLINE_CURVE((1.,1.,1.,1.,1.,1.,1.,1.,1.,1.,1.,1.,1.,1.,1.,1.,
1.,1.,1.,1.,1.,1.,1.,1.,1.,1.,1.,1.,1.,1.,1.,1.,1.,1.,1.,1.,1.,1.,1.,1.,
1.,1.,1.,1.,1.,1.,1.,1.,1.,1.,1.,1.,1.,1.,1.,1.,1.,1.,1.,1.,1.,1.,1.,1.,
1.,1.,1.,1.,1.,1.))
REPRESENTATION_ITEM('')
);
#465=(
BOUNDED_CURVE()
B_SPLINE_CURVE(5,(#67560,#67561,#67562,#67563,#67564,#67565,#67566,#67567,
#67568,#67569,#67570,#67571,#67572,#67573,#67574,#67575,#67576,#67577,#67578,
#67579,#67580,#67581,#67582,#67583,#67584,#67585,#67586,#67587,#67588,#67589,
#67590,#67591,#67592,#67593,#67594,#67595,#67596,#67597,#67598,#67599,#67600,
#67601,#67602,#67603,#67604,#67605,#67606,#67607,#67608,#67609,#67610,#67611,
#67612,#67613,#67614,#67615,#67616,#67617,#67618,#67619,#67620,#67621,#67622,
#67623,#67624,#67625,#67626,#67627,#67628,#67629),.UNSPECIFIED.,.F.,.F.)
B_SPLINE_CURVE_WITH_KNOTS((6,1,1,1,1,1,1,1,1,1,1,1,1,1,1,1,1,1,1,1,1,1,
1,1,1,1,1,1,1,1,1,1,1,1,1,1,1,1,1,1,1,1,1,1,1,1,1,1,1,1,1,1,1,1,1,1,1,1,
1,1,1,1,1,1,1,6),(-1.,-0.984615384615383,-0.969230769230768,-0.953846153846152,
-0.938461538461537,-0.923076923076922,-0.907692307692306,-0.892307692307691,
-0.876923076923076,-0.86153846153846,-0.846153846153845,-0.83076923076923,
-0.815384615384614,-0.799999999999999,-0.784615384615384,-0.769230769230768,
-0.753846153846153,-0.738461538461538,-0.723076923076922,-0.707692307692307,
-0.692307692307692,-0.676923076923076,-0.661538461538461,-0.646153846153846,
-0.63076923076923,-0.615384615384615,-0.6,-0.584615384615384,-0.569230769230769,
-0.553846153846154,-0.538461538461538,-0.523076923076923,-0.507692307692308,
-0.492307692307692,-0.476923076923077,-0.461538461538462,-0.446153846153846,
-0.430769230769231,-0.415384615384615,-0.4,-0.384615384615385,-0.369230769230769,
-0.353846153846154,-0.338461538461538,-0.323076923076923,-0.307692307692308,
-0.292307692307692,-0.276923076923077,-0.261538461538462,-0.246153846153846,
-0.230769230769231,-0.215384615384615,-0.2,-0.184615384615385,-0.169230769230769,
-0.153846153846154,-0.138461538461538,-0.123076923076923,-0.107692307692308,
-0.0923076923076923,-0.0769230769230769,-0.0615384615384615,-0.0461538461538462,
-0.0307692307692308,-0.0153846153846154,-0.00577184337451051),
 .UNSPECIFIED.)
CURVE()
GEOMETRIC_REPRESENTATION_ITEM()
RATIONAL_B_SPLINE_CURVE((1.,1.,1.,1.,1.,1.,1.,1.,1.,1.,1.,1.,1.,1.,1.,1.,
1.,1.,1.,1.,1.,1.,1.,1.,1.,1.,1.,1.,1.,1.,1.,1.,1.,1.,1.,1.,1.,1.,1.,1.,
1.,1.,1.,1.,1.,1.,1.,1.,1.,1.,1.,1.,1.,1.,1.,1.,1.,1.,1.,1.,1.,1.,1.,1.,
1.,1.,1.,1.,1.,1.))
REPRESENTATION_ITEM('')
);
#466=(
BOUNDED_CURVE()
B_SPLINE_CURVE(5,(#67780,#67781,#67782,#67783,#67784,#67785,#67786,#67787,
#67788,#67789,#67790,#67791,#67792,#67793,#67794,#67795,#67796,#67797,#67798,
#67799,#67800,#67801,#67802,#67803,#67804,#67805,#67806,#67807,#67808,#67809,
#67810,#67811,#67812,#67813,#67814,#67815,#67816,#67817,#67818,#67819,#67820,
#67821,#67822,#67823,#67824,#67825,#67826,#67827,#67828,#67829,#67830,#67831,
#67832,#67833,#67834,#67835,#67836,#67837,#67838,#67839,#67840,#67841,#67842,
#67843,#67844,#67845,#67846,#67847,#67848,#67849),.UNSPECIFIED.,.F.,.F.)
B_SPLINE_CURVE_WITH_KNOTS((6,1,1,1,1,1,1,1,1,1,1,1,1,1,1,1,1,1,1,1,1,1,
1,1,1,1,1,1,1,1,1,1,1,1,1,1,1,1,1,1,1,1,1,1,1,1,1,1,1,1,1,1,1,1,1,1,1,1,
1,1,1,1,1,1,1,6),(-0.994228156739678,-0.984615384615383,-0.969230769230768,
-0.953846153846152,-0.938461538461537,-0.923076923076922,-0.907692307692306,
-0.892307692307691,-0.876923076923076,-0.86153846153846,-0.846153846153845,
-0.83076923076923,-0.815384615384614,-0.799999999999999,-0.784615384615384,
-0.769230769230768,-0.753846153846153,-0.738461538461538,-0.723076923076922,
-0.707692307692307,-0.692307692307692,-0.676923076923076,-0.661538461538461,
-0.646153846153846,-0.63076923076923,-0.615384615384615,-0.6,-0.584615384615384,
-0.569230769230769,-0.553846153846154,-0.538461538461538,-0.523076923076923,
-0.507692307692308,-0.492307692307692,-0.476923076923077,-0.461538461538462,
-0.446153846153846,-0.430769230769231,-0.415384615384615,-0.4,-0.384615384615385,
-0.369230769230769,-0.353846153846154,-0.338461538461538,-0.323076923076923,
-0.307692307692308,-0.292307692307692,-0.276923076923077,-0.261538461538462,
-0.246153846153846,-0.230769230769231,-0.215384615384615,-0.2,-0.184615384615385,
-0.169230769230769,-0.153846153846154,-0.138461538461538,-0.123076923076923,
-0.107692307692308,-0.0923076923076923,-0.0769230769230769,-0.0615384615384615,
-0.0461538461538462,-0.0307692307692308,-0.0153846153846154,0.),
 .UNSPECIFIED.)
CURVE()
GEOMETRIC_REPRESENTATION_ITEM()
RATIONAL_B_SPLINE_CURVE((1.,1.,1.,1.,1.,1.,1.,1.,1.,1.,1.,1.,1.,1.,1.,1.,
1.,1.,1.,1.,1.,1.,1.,1.,1.,1.,1.,1.,1.,1.,1.,1.,1.,1.,1.,1.,1.,1.,1.,1.,
1.,1.,1.,1.,1.,1.,1.,1.,1.,1.,1.,1.,1.,1.,1.,1.,1.,1.,1.,1.,1.,1.,1.,1.,
1.,1.,1.,1.,1.,1.))
REPRESENTATION_ITEM('')
);
#467=(
BOUNDED_CURVE()
B_SPLINE_CURVE(5,(#68002,#68003,#68004,#68005,#68006,#68007,#68008,#68009,
#68010,#68011,#68012,#68013,#68014,#68015,#68016,#68017,#68018,#68019,#68020,
#68021,#68022,#68023,#68024,#68025,#68026,#68027,#68028,#68029,#68030,#68031,
#68032,#68033,#68034,#68035,#68036,#68037,#68038,#68039,#68040,#68041,#68042,
#68043,#68044,#68045,#68046,#68047,#68048,#68049,#68050,#68051,#68052,#68053,
#68054,#68055,#68056,#68057,#68058,#68059,#68060,#68061,#68062,#68063,#68064,
#68065,#68066,#68067,#68068,#68069,#68070,#68071),.UNSPECIFIED.,.F.,.F.)
B_SPLINE_CURVE_WITH_KNOTS((6,1,1,1,1,1,1,1,1,1,1,1,1,1,1,1,1,1,1,1,1,1,
1,1,1,1,1,1,1,1,1,1,1,1,1,1,1,1,1,1,1,1,1,1,1,1,1,1,1,1,1,1,1,1,1,1,1,1,
1,1,1,1,1,1,1,6),(-1.,-0.984615384615383,-0.969230769230768,-0.953846153846152,
-0.938461538461537,-0.923076923076922,-0.907692307692306,-0.892307692307691,
-0.876923076923076,-0.86153846153846,-0.846153846153845,-0.83076923076923,
-0.815384615384614,-0.799999999999999,-0.784615384615384,-0.769230769230768,
-0.753846153846153,-0.738461538461538,-0.723076923076922,-0.707692307692307,
-0.692307692307692,-0.676923076923076,-0.661538461538461,-0.646153846153846,
-0.63076923076923,-0.615384615384615,-0.6,-0.584615384615384,-0.569230769230769,
-0.553846153846154,-0.538461538461538,-0.523076923076923,-0.507692307692308,
-0.492307692307692,-0.476923076923077,-0.461538461538462,-0.446153846153846,
-0.430769230769231,-0.415384615384615,-0.4,-0.384615384615385,-0.369230769230769,
-0.353846153846154,-0.338461538461538,-0.323076923076923,-0.307692307692308,
-0.292307692307692,-0.276923076923077,-0.261538461538462,-0.246153846153846,
-0.230769230769231,-0.215384615384615,-0.2,-0.184615384615385,-0.169230769230769,
-0.153846153846154,-0.138461538461538,-0.123076923076923,-0.107692307692308,
-0.0923076923076923,-0.0769230769230769,-0.0615384615384615,-0.0461538461538462,
-0.0307692307692308,-0.0153846153846154,-0.0057718433745179),
 .UNSPECIFIED.)
CURVE()
GEOMETRIC_REPRESENTATION_ITEM()
RATIONAL_B_SPLINE_CURVE((1.,1.,1.,1.,1.,1.,1.,1.,1.,1.,1.,1.,1.,1.,1.,1.,
1.,1.,1.,1.,1.,1.,1.,1.,1.,1.,1.,1.,1.,1.,1.,1.,1.,1.,1.,1.,1.,1.,1.,1.,
1.,1.,1.,1.,1.,1.,1.,1.,1.,1.,1.,1.,1.,1.,1.,1.,1.,1.,1.,1.,1.,1.,1.,1.,
1.,1.,1.,1.,1.,1.))
REPRESENTATION_ITEM('')
);
#468=(
BOUNDED_CURVE()
B_SPLINE_CURVE(5,(#68222,#68223,#68224,#68225,#68226,#68227,#68228,#68229,
#68230,#68231,#68232,#68233,#68234,#68235,#68236,#68237,#68238,#68239,#68240,
#68241,#68242,#68243,#68244,#68245,#68246,#68247,#68248,#68249,#68250,#68251,
#68252,#68253,#68254,#68255,#68256,#68257,#68258,#68259,#68260,#68261,#68262,
#68263,#68264,#68265,#68266,#68267,#68268,#68269,#68270,#68271,#68272,#68273,
#68274,#68275,#68276,#68277,#68278,#68279,#68280,#68281,#68282,#68283,#68284,
#68285,#68286,#68287,#68288,#68289,#68290,#68291),.UNSPECIFIED.,.F.,.F.)
B_SPLINE_CURVE_WITH_KNOTS((6,1,1,1,1,1,1,1,1,1,1,1,1,1,1,1,1,1,1,1,1,1,
1,1,1,1,1,1,1,1,1,1,1,1,1,1,1,1,1,1,1,1,1,1,1,1,1,1,1,1,1,1,1,1,1,1,1,1,
1,1,1,1,1,1,1,6),(-0.99422815673967,-0.984615384615383,-0.969230769230768,
-0.953846153846152,-0.938461538461537,-0.923076923076922,-0.907692307692306,
-0.892307692307691,-0.876923076923076,-0.86153846153846,-0.846153846153845,
-0.83076923076923,-0.815384615384614,-0.799999999999999,-0.784615384615384,
-0.769230769230768,-0.753846153846153,-0.738461538461538,-0.723076923076922,
-0.707692307692307,-0.692307692307692,-0.676923076923076,-0.661538461538461,
-0.646153846153846,-0.63076923076923,-0.615384615384615,-0.6,-0.584615384615384,
-0.569230769230769,-0.553846153846154,-0.538461538461538,-0.523076923076923,
-0.507692307692308,-0.492307692307692,-0.476923076923077,-0.461538461538462,
-0.446153846153846,-0.430769230769231,-0.415384615384615,-0.4,-0.384615384615385,
-0.369230769230769,-0.353846153846154,-0.338461538461538,-0.323076923076923,
-0.307692307692308,-0.292307692307692,-0.276923076923077,-0.261538461538462,
-0.246153846153846,-0.230769230769231,-0.215384615384615,-0.2,-0.184615384615385,
-0.169230769230769,-0.153846153846154,-0.138461538461538,-0.123076923076923,
-0.107692307692308,-0.0923076923076923,-0.0769230769230769,-0.0615384615384615,
-0.0461538461538462,-0.0307692307692308,-0.0153846153846154,0.),
 .UNSPECIFIED.)
CURVE()
GEOMETRIC_REPRESENTATION_ITEM()
RATIONAL_B_SPLINE_CURVE((1.,1.,1.,1.,1.,1.,1.,1.,1.,1.,1.,1.,1.,1.,1.,1.,
1.,1.,1.,1.,1.,1.,1.,1.,1.,1.,1.,1.,1.,1.,1.,1.,1.,1.,1.,1.,1.,1.,1.,1.,
1.,1.,1.,1.,1.,1.,1.,1.,1.,1.,1.,1.,1.,1.,1.,1.,1.,1.,1.,1.,1.,1.,1.,1.,
1.,1.,1.,1.,1.,1.))
REPRESENTATION_ITEM('')
);
#469=(
BOUNDED_CURVE()
B_SPLINE_CURVE(5,(#68444,#68445,#68446,#68447,#68448,#68449,#68450,#68451,
#68452,#68453,#68454,#68455,#68456,#68457,#68458,#68459,#68460,#68461,#68462,
#68463,#68464,#68465,#68466,#68467,#68468,#68469,#68470,#68471,#68472,#68473,
#68474,#68475,#68476,#68477,#68478,#68479,#68480,#68481,#68482,#68483,#68484,
#68485,#68486,#68487,#68488,#68489,#68490,#68491,#68492,#68493,#68494,#68495,
#68496,#68497,#68498,#68499,#68500,#68501,#68502,#68503,#68504,#68505,#68506,
#68507,#68508,#68509,#68510,#68511,#68512,#68513),.UNSPECIFIED.,.F.,.F.)
B_SPLINE_CURVE_WITH_KNOTS((6,1,1,1,1,1,1,1,1,1,1,1,1,1,1,1,1,1,1,1,1,1,
1,1,1,1,1,1,1,1,1,1,1,1,1,1,1,1,1,1,1,1,1,1,1,1,1,1,1,1,1,1,1,1,1,1,1,1,
1,1,1,1,1,1,1,6),(-1.,-0.984615384615383,-0.969230769230768,-0.953846153846152,
-0.938461538461537,-0.923076923076922,-0.907692307692306,-0.892307692307691,
-0.876923076923076,-0.86153846153846,-0.846153846153845,-0.83076923076923,
-0.815384615384614,-0.799999999999999,-0.784615384615384,-0.769230769230768,
-0.753846153846153,-0.738461538461538,-0.723076923076922,-0.707692307692307,
-0.692307692307692,-0.676923076923076,-0.661538461538461,-0.646153846153846,
-0.63076923076923,-0.615384615384615,-0.6,-0.584615384615384,-0.569230769230769,
-0.553846153846154,-0.538461538461538,-0.523076923076923,-0.507692307692308,
-0.492307692307692,-0.476923076923077,-0.461538461538462,-0.446153846153846,
-0.430769230769231,-0.415384615384615,-0.4,-0.384615384615385,-0.369230769230769,
-0.353846153846154,-0.338461538461538,-0.323076923076923,-0.307692307692308,
-0.292307692307692,-0.276923076923077,-0.261538461538462,-0.246153846153846,
-0.230769230769231,-0.215384615384615,-0.2,-0.184615384615385,-0.169230769230769,
-0.153846153846154,-0.138461538461538,-0.123076923076923,-0.107692307692308,
-0.0923076923076923,-0.0769230769230769,-0.0615384615384615,-0.0461538461538462,
-0.0307692307692308,-0.0153846153846154,-0.00577184337452479),
 .UNSPECIFIED.)
CURVE()
GEOMETRIC_REPRESENTATION_ITEM()
RATIONAL_B_SPLINE_CURVE((1.,1.,1.,1.,1.,1.,1.,1.,1.,1.,1.,1.,1.,1.,1.,1.,
1.,1.,1.,1.,1.,1.,1.,1.,1.,1.,1.,1.,1.,1.,1.,1.,1.,1.,1.,1.,1.,1.,1.,1.,
1.,1.,1.,1.,1.,1.,1.,1.,1.,1.,1.,1.,1.,1.,1.,1.,1.,1.,1.,1.,1.,1.,1.,1.,
1.,1.,1.,1.,1.,1.))
REPRESENTATION_ITEM('')
);
#470=(
BOUNDED_CURVE()
B_SPLINE_CURVE(5,(#68664,#68665,#68666,#68667,#68668,#68669,#68670,#68671,
#68672,#68673,#68674,#68675,#68676,#68677,#68678,#68679,#68680,#68681,#68682,
#68683,#68684,#68685,#68686,#68687,#68688,#68689,#68690,#68691,#68692,#68693,
#68694,#68695,#68696,#68697,#68698,#68699,#68700,#68701,#68702,#68703,#68704,
#68705,#68706,#68707,#68708,#68709,#68710,#68711,#68712,#68713,#68714,#68715,
#68716,#68717,#68718,#68719,#68720,#68721,#68722,#68723,#68724,#68725,#68726,
#68727,#68728,#68729,#68730,#68731,#68732,#68733),.UNSPECIFIED.,.F.,.F.)
B_SPLINE_CURVE_WITH_KNOTS((6,1,1,1,1,1,1,1,1,1,1,1,1,1,1,1,1,1,1,1,1,1,
1,1,1,1,1,1,1,1,1,1,1,1,1,1,1,1,1,1,1,1,1,1,1,1,1,1,1,1,1,1,1,1,1,1,1,1,
1,1,1,1,1,1,1,6),(-0.99422815673967,-0.984615384615383,-0.969230769230768,
-0.953846153846152,-0.938461538461537,-0.923076923076922,-0.907692307692306,
-0.892307692307691,-0.876923076923076,-0.86153846153846,-0.846153846153845,
-0.83076923076923,-0.815384615384614,-0.799999999999999,-0.784615384615384,
-0.769230769230768,-0.753846153846153,-0.738461538461538,-0.723076923076922,
-0.707692307692307,-0.692307692307692,-0.676923076923076,-0.661538461538461,
-0.646153846153846,-0.63076923076923,-0.615384615384615,-0.6,-0.584615384615384,
-0.569230769230769,-0.553846153846154,-0.538461538461538,-0.523076923076923,
-0.507692307692308,-0.492307692307692,-0.476923076923077,-0.461538461538462,
-0.446153846153846,-0.430769230769231,-0.415384615384615,-0.4,-0.384615384615385,
-0.369230769230769,-0.353846153846154,-0.338461538461538,-0.323076923076923,
-0.307692307692308,-0.292307692307692,-0.276923076923077,-0.261538461538462,
-0.246153846153846,-0.230769230769231,-0.215384615384615,-0.2,-0.184615384615385,
-0.169230769230769,-0.153846153846154,-0.138461538461538,-0.123076923076923,
-0.107692307692308,-0.0923076923076923,-0.0769230769230769,-0.0615384615384615,
-0.0461538461538462,-0.0307692307692308,-0.0153846153846154,0.),
 .UNSPECIFIED.)
CURVE()
GEOMETRIC_REPRESENTATION_ITEM()
RATIONAL_B_SPLINE_CURVE((1.,1.,1.,1.,1.,1.,1.,1.,1.,1.,1.,1.,1.,1.,1.,1.,
1.,1.,1.,1.,1.,1.,1.,1.,1.,1.,1.,1.,1.,1.,1.,1.,1.,1.,1.,1.,1.,1.,1.,1.,
1.,1.,1.,1.,1.,1.,1.,1.,1.,1.,1.,1.,1.,1.,1.,1.,1.,1.,1.,1.,1.,1.,1.,1.,
1.,1.,1.,1.,1.,1.))
REPRESENTATION_ITEM('')
);
#471=(
BOUNDED_CURVE()
B_SPLINE_CURVE(5,(#68886,#68887,#68888,#68889,#68890,#68891,#68892,#68893,
#68894,#68895,#68896,#68897,#68898,#68899,#68900,#68901,#68902,#68903,#68904,
#68905,#68906,#68907,#68908,#68909,#68910,#68911,#68912,#68913,#68914,#68915,
#68916,#68917,#68918,#68919,#68920,#68921,#68922,#68923,#68924,#68925,#68926,
#68927,#68928,#68929,#68930,#68931,#68932,#68933,#68934,#68935,#68936,#68937,
#68938,#68939,#68940,#68941,#68942,#68943,#68944,#68945,#68946,#68947,#68948,
#68949,#68950,#68951,#68952,#68953,#68954,#68955),.UNSPECIFIED.,.F.,.F.)
B_SPLINE_CURVE_WITH_KNOTS((6,1,1,1,1,1,1,1,1,1,1,1,1,1,1,1,1,1,1,1,1,1,
1,1,1,1,1,1,1,1,1,1,1,1,1,1,1,1,1,1,1,1,1,1,1,1,1,1,1,1,1,1,1,1,1,1,1,1,
1,1,1,1,1,1,1,6),(-1.,-0.984615384615383,-0.969230769230768,-0.953846153846152,
-0.938461538461537,-0.923076923076922,-0.907692307692306,-0.892307692307691,
-0.876923076923076,-0.86153846153846,-0.846153846153845,-0.83076923076923,
-0.815384615384614,-0.799999999999999,-0.784615384615384,-0.769230769230768,
-0.753846153846153,-0.738461538461538,-0.723076923076922,-0.707692307692307,
-0.692307692307692,-0.676923076923076,-0.661538461538461,-0.646153846153846,
-0.63076923076923,-0.615384615384615,-0.6,-0.584615384615384,-0.569230769230769,
-0.553846153846154,-0.538461538461538,-0.523076923076923,-0.507692307692308,
-0.492307692307692,-0.476923076923077,-0.461538461538462,-0.446153846153846,
-0.430769230769231,-0.415384615384615,-0.4,-0.384615384615385,-0.369230769230769,
-0.353846153846154,-0.338461538461538,-0.323076923076923,-0.307692307692308,
-0.292307692307692,-0.276923076923077,-0.261538461538462,-0.246153846153846,
-0.230769230769231,-0.215384615384615,-0.2,-0.184615384615385,-0.169230769230769,
-0.153846153846154,-0.138461538461538,-0.123076923076923,-0.107692307692308,
-0.0923076923076923,-0.0769230769230769,-0.0615384615384615,-0.0461538461538462,
-0.0307692307692308,-0.0153846153846154,-0.0057718433745009),
 .UNSPECIFIED.)
CURVE()
GEOMETRIC_REPRESENTATION_ITEM()
RATIONAL_B_SPLINE_CURVE((1.,1.,1.,1.,1.,1.,1.,1.,1.,1.,1.,1.,1.,1.,1.,1.,
1.,1.,1.,1.,1.,1.,1.,1.,1.,1.,1.,1.,1.,1.,1.,1.,1.,1.,1.,1.,1.,1.,1.,1.,
1.,1.,1.,1.,1.,1.,1.,1.,1.,1.,1.,1.,1.,1.,1.,1.,1.,1.,1.,1.,1.,1.,1.,1.,
1.,1.,1.,1.,1.,1.))
REPRESENTATION_ITEM('')
);
#472=(
BOUNDED_CURVE()
B_SPLINE_CURVE(5,(#69106,#69107,#69108,#69109,#69110,#69111,#69112,#69113,
#69114,#69115,#69116,#69117,#69118,#69119,#69120,#69121,#69122,#69123,#69124,
#69125,#69126,#69127,#69128,#69129,#69130,#69131,#69132,#69133,#69134,#69135,
#69136,#69137,#69138,#69139,#69140,#69141,#69142,#69143,#69144,#69145,#69146,
#69147,#69148,#69149,#69150,#69151,#69152,#69153,#69154,#69155,#69156,#69157,
#69158,#69159,#69160,#69161,#69162,#69163,#69164,#69165,#69166,#69167,#69168,
#69169,#69170,#69171,#69172,#69173,#69174,#69175),.UNSPECIFIED.,.F.,.F.)
B_SPLINE_CURVE_WITH_KNOTS((6,1,1,1,1,1,1,1,1,1,1,1,1,1,1,1,1,1,1,1,1,1,
1,1,1,1,1,1,1,1,1,1,1,1,1,1,1,1,1,1,1,1,1,1,1,1,1,1,1,1,1,1,1,1,1,1,1,1,
1,1,1,1,1,1,1,6),(-0.99422815673967,-0.984615384615383,-0.969230769230768,
-0.953846153846152,-0.938461538461537,-0.923076923076922,-0.907692307692306,
-0.892307692307691,-0.876923076923076,-0.86153846153846,-0.846153846153845,
-0.83076923076923,-0.815384615384614,-0.799999999999999,-0.784615384615384,
-0.769230769230768,-0.753846153846153,-0.738461538461538,-0.723076923076922,
-0.707692307692307,-0.692307692307692,-0.676923076923076,-0.661538461538461,
-0.646153846153846,-0.63076923076923,-0.615384615384615,-0.6,-0.584615384615384,
-0.569230769230769,-0.553846153846154,-0.538461538461538,-0.523076923076923,
-0.507692307692308,-0.492307692307692,-0.476923076923077,-0.461538461538462,
-0.446153846153846,-0.430769230769231,-0.415384615384615,-0.4,-0.384615384615385,
-0.369230769230769,-0.353846153846154,-0.338461538461538,-0.323076923076923,
-0.307692307692308,-0.292307692307692,-0.276923076923077,-0.261538461538462,
-0.246153846153846,-0.230769230769231,-0.215384615384615,-0.2,-0.184615384615385,
-0.169230769230769,-0.153846153846154,-0.138461538461538,-0.123076923076923,
-0.107692307692308,-0.0923076923076923,-0.0769230769230769,-0.0615384615384615,
-0.0461538461538462,-0.0307692307692308,-0.0153846153846154,0.),
 .UNSPECIFIED.)
CURVE()
GEOMETRIC_REPRESENTATION_ITEM()
RATIONAL_B_SPLINE_CURVE((1.,1.,1.,1.,1.,1.,1.,1.,1.,1.,1.,1.,1.,1.,1.,1.,
1.,1.,1.,1.,1.,1.,1.,1.,1.,1.,1.,1.,1.,1.,1.,1.,1.,1.,1.,1.,1.,1.,1.,1.,
1.,1.,1.,1.,1.,1.,1.,1.,1.,1.,1.,1.,1.,1.,1.,1.,1.,1.,1.,1.,1.,1.,1.,1.,
1.,1.,1.,1.,1.,1.))
REPRESENTATION_ITEM('')
);
#473=(
BOUNDED_CURVE()
B_SPLINE_CURVE(5,(#69328,#69329,#69330,#69331,#69332,#69333,#69334,#69335,
#69336,#69337,#69338,#69339,#69340,#69341,#69342,#69343,#69344,#69345,#69346,
#69347,#69348,#69349,#69350,#69351,#69352,#69353,#69354,#69355,#69356,#69357,
#69358,#69359,#69360,#69361,#69362,#69363,#69364,#69365,#69366,#69367,#69368,
#69369,#69370,#69371,#69372,#69373,#69374,#69375,#69376,#69377,#69378,#69379,
#69380,#69381,#69382,#69383,#69384,#69385,#69386,#69387,#69388,#69389,#69390,
#69391,#69392,#69393,#69394,#69395,#69396,#69397),.UNSPECIFIED.,.F.,.F.)
B_SPLINE_CURVE_WITH_KNOTS((6,1,1,1,1,1,1,1,1,1,1,1,1,1,1,1,1,1,1,1,1,1,
1,1,1,1,1,1,1,1,1,1,1,1,1,1,1,1,1,1,1,1,1,1,1,1,1,1,1,1,1,1,1,1,1,1,1,1,
1,1,1,1,1,1,1,6),(-1.,-0.984615384615383,-0.969230769230768,-0.953846153846152,
-0.938461538461537,-0.923076923076922,-0.907692307692306,-0.892307692307691,
-0.876923076923076,-0.86153846153846,-0.846153846153845,-0.83076923076923,
-0.815384615384614,-0.799999999999999,-0.784615384615384,-0.769230769230768,
-0.753846153846153,-0.738461538461538,-0.723076923076922,-0.707692307692307,
-0.692307692307692,-0.676923076923076,-0.661538461538461,-0.646153846153846,
-0.63076923076923,-0.615384615384615,-0.6,-0.584615384615384,-0.569230769230769,
-0.553846153846154,-0.538461538461538,-0.523076923076923,-0.507692307692308,
-0.492307692307692,-0.476923076923077,-0.461538461538462,-0.446153846153846,
-0.430769230769231,-0.415384615384615,-0.4,-0.384615384615385,-0.369230769230769,
-0.353846153846154,-0.338461538461538,-0.323076923076923,-0.307692307692308,
-0.292307692307692,-0.276923076923077,-0.261538461538462,-0.246153846153846,
-0.230769230769231,-0.215384615384615,-0.2,-0.184615384615385,-0.169230769230769,
-0.153846153846154,-0.138461538461538,-0.123076923076923,-0.107692307692308,
-0.0923076923076923,-0.0769230769230769,-0.0615384615384615,-0.0461538461538462,
-0.0307692307692308,-0.0153846153846154,-0.00577184337450701),
 .UNSPECIFIED.)
CURVE()
GEOMETRIC_REPRESENTATION_ITEM()
RATIONAL_B_SPLINE_CURVE((1.,1.,1.,1.,1.,1.,1.,1.,1.,1.,1.,1.,1.,1.,1.,1.,
1.,1.,1.,1.,1.,1.,1.,1.,1.,1.,1.,1.,1.,1.,1.,1.,1.,1.,1.,1.,1.,1.,1.,1.,
1.,1.,1.,1.,1.,1.,1.,1.,1.,1.,1.,1.,1.,1.,1.,1.,1.,1.,1.,1.,1.,1.,1.,1.,
1.,1.,1.,1.,1.,1.))
REPRESENTATION_ITEM('')
);
#474=(
BOUNDED_CURVE()
B_SPLINE_CURVE(5,(#69548,#69549,#69550,#69551,#69552,#69553,#69554,#69555,
#69556,#69557,#69558,#69559,#69560,#69561,#69562,#69563,#69564,#69565,#69566,
#69567,#69568,#69569,#69570,#69571,#69572,#69573,#69574,#69575,#69576,#69577,
#69578,#69579,#69580,#69581,#69582,#69583,#69584,#69585,#69586,#69587,#69588,
#69589,#69590,#69591,#69592,#69593,#69594,#69595,#69596,#69597,#69598,#69599,
#69600,#69601,#69602,#69603,#69604,#69605,#69606,#69607,#69608,#69609,#69610,
#69611,#69612,#69613,#69614,#69615,#69616,#69617),.UNSPECIFIED.,.F.,.F.)
B_SPLINE_CURVE_WITH_KNOTS((6,1,1,1,1,1,1,1,1,1,1,1,1,1,1,1,1,1,1,1,1,1,
1,1,1,1,1,1,1,1,1,1,1,1,1,1,1,1,1,1,1,1,1,1,1,1,1,1,1,1,1,1,1,1,1,1,1,1,
1,1,1,1,1,1,1,6),(-0.994228156739689,-0.984615384615383,-0.969230769230768,
-0.953846153846152,-0.938461538461537,-0.923076923076922,-0.907692307692306,
-0.892307692307691,-0.876923076923076,-0.86153846153846,-0.846153846153845,
-0.83076923076923,-0.815384615384614,-0.799999999999999,-0.784615384615384,
-0.769230769230768,-0.753846153846153,-0.738461538461538,-0.723076923076922,
-0.707692307692307,-0.692307692307692,-0.676923076923076,-0.661538461538461,
-0.646153846153846,-0.63076923076923,-0.615384615384615,-0.6,-0.584615384615384,
-0.569230769230769,-0.553846153846154,-0.538461538461538,-0.523076923076923,
-0.507692307692308,-0.492307692307692,-0.476923076923077,-0.461538461538462,
-0.446153846153846,-0.430769230769231,-0.415384615384615,-0.4,-0.384615384615385,
-0.369230769230769,-0.353846153846154,-0.338461538461538,-0.323076923076923,
-0.307692307692308,-0.292307692307692,-0.276923076923077,-0.261538461538462,
-0.246153846153846,-0.230769230769231,-0.215384615384615,-0.2,-0.184615384615385,
-0.169230769230769,-0.153846153846154,-0.138461538461538,-0.123076923076923,
-0.107692307692308,-0.0923076923076923,-0.0769230769230769,-0.0615384615384615,
-0.0461538461538462,-0.0307692307692308,-0.0153846153846154,0.),
 .UNSPECIFIED.)
CURVE()
GEOMETRIC_REPRESENTATION_ITEM()
RATIONAL_B_SPLINE_CURVE((1.,1.,1.,1.,1.,1.,1.,1.,1.,1.,1.,1.,1.,1.,1.,1.,
1.,1.,1.,1.,1.,1.,1.,1.,1.,1.,1.,1.,1.,1.,1.,1.,1.,1.,1.,1.,1.,1.,1.,1.,
1.,1.,1.,1.,1.,1.,1.,1.,1.,1.,1.,1.,1.,1.,1.,1.,1.,1.,1.,1.,1.,1.,1.,1.,
1.,1.,1.,1.,1.,1.))
REPRESENTATION_ITEM('')
);
#475=(
BOUNDED_CURVE()
B_SPLINE_CURVE(5,(#69770,#69771,#69772,#69773,#69774,#69775,#69776,#69777,
#69778,#69779,#69780,#69781,#69782,#69783,#69784,#69785,#69786,#69787,#69788,
#69789,#69790,#69791,#69792,#69793,#69794,#69795,#69796,#69797,#69798,#69799,
#69800,#69801,#69802,#69803,#69804,#69805,#69806,#69807,#69808,#69809,#69810,
#69811,#69812,#69813,#69814,#69815,#69816,#69817,#69818,#69819,#69820,#69821,
#69822,#69823,#69824,#69825,#69826,#69827,#69828,#69829,#69830,#69831,#69832,
#69833,#69834,#69835,#69836,#69837,#69838,#69839),.UNSPECIFIED.,.F.,.F.)
B_SPLINE_CURVE_WITH_KNOTS((6,1,1,1,1,1,1,1,1,1,1,1,1,1,1,1,1,1,1,1,1,1,
1,1,1,1,1,1,1,1,1,1,1,1,1,1,1,1,1,1,1,1,1,1,1,1,1,1,1,1,1,1,1,1,1,1,1,1,
1,1,1,1,1,1,1,6),(-1.,-0.984615384615383,-0.969230769230768,-0.953846153846152,
-0.938461538461537,-0.923076923076922,-0.907692307692306,-0.892307692307691,
-0.876923076923076,-0.86153846153846,-0.846153846153845,-0.83076923076923,
-0.815384615384614,-0.799999999999999,-0.784615384615384,-0.769230769230768,
-0.753846153846153,-0.738461538461538,-0.723076923076922,-0.707692307692307,
-0.692307692307692,-0.676923076923076,-0.661538461538461,-0.646153846153846,
-0.63076923076923,-0.615384615384615,-0.6,-0.584615384615384,-0.569230769230769,
-0.553846153846154,-0.538461538461538,-0.523076923076923,-0.507692307692308,
-0.492307692307692,-0.476923076923077,-0.461538461538462,-0.446153846153846,
-0.430769230769231,-0.415384615384615,-0.4,-0.384615384615385,-0.369230769230769,
-0.353846153846154,-0.338461538461538,-0.323076923076923,-0.307692307692308,
-0.292307692307692,-0.276923076923077,-0.261538461538462,-0.246153846153846,
-0.230769230769231,-0.215384615384615,-0.2,-0.184615384615385,-0.169230769230769,
-0.153846153846154,-0.138461538461538,-0.123076923076923,-0.107692307692308,
-0.0923076923076923,-0.0769230769230769,-0.0615384615384615,-0.0461538461538462,
-0.0307692307692308,-0.0153846153846154,-0.00577184337452382),
 .UNSPECIFIED.)
CURVE()
GEOMETRIC_REPRESENTATION_ITEM()
RATIONAL_B_SPLINE_CURVE((1.,1.,1.,1.,1.,1.,1.,1.,1.,1.,1.,1.,1.,1.,1.,1.,
1.,1.,1.,1.,1.,1.,1.,1.,1.,1.,1.,1.,1.,1.,1.,1.,1.,1.,1.,1.,1.,1.,1.,1.,
1.,1.,1.,1.,1.,1.,1.,1.,1.,1.,1.,1.,1.,1.,1.,1.,1.,1.,1.,1.,1.,1.,1.,1.,
1.,1.,1.,1.,1.,1.))
REPRESENTATION_ITEM('')
);
#476=(
BOUNDED_CURVE()
B_SPLINE_CURVE(5,(#69990,#69991,#69992,#69993,#69994,#69995,#69996,#69997,
#69998,#69999,#70000,#70001,#70002,#70003,#70004,#70005,#70006,#70007,#70008,
#70009,#70010,#70011,#70012,#70013,#70014,#70015,#70016,#70017,#70018,#70019,
#70020,#70021,#70022,#70023,#70024,#70025,#70026,#70027,#70028,#70029,#70030,
#70031,#70032,#70033,#70034,#70035,#70036,#70037,#70038,#70039,#70040,#70041,
#70042,#70043,#70044,#70045,#70046,#70047,#70048,#70049,#70050,#70051,#70052,
#70053,#70054,#70055,#70056,#70057,#70058,#70059),.UNSPECIFIED.,.F.,.F.)
B_SPLINE_CURVE_WITH_KNOTS((6,1,1,1,1,1,1,1,1,1,1,1,1,1,1,1,1,1,1,1,1,1,
1,1,1,1,1,1,1,1,1,1,1,1,1,1,1,1,1,1,1,1,1,1,1,1,1,1,1,1,1,1,1,1,1,1,1,1,
1,1,1,1,1,1,1,6),(-0.994228156739677,-0.984615384615383,-0.969230769230768,
-0.953846153846152,-0.938461538461537,-0.923076923076922,-0.907692307692306,
-0.892307692307691,-0.876923076923076,-0.86153846153846,-0.846153846153845,
-0.83076923076923,-0.815384615384614,-0.799999999999999,-0.784615384615384,
-0.769230769230768,-0.753846153846153,-0.738461538461538,-0.723076923076922,
-0.707692307692307,-0.692307692307692,-0.676923076923076,-0.661538461538461,
-0.646153846153846,-0.63076923076923,-0.615384615384615,-0.6,-0.584615384615384,
-0.569230769230769,-0.553846153846154,-0.538461538461538,-0.523076923076923,
-0.507692307692308,-0.492307692307692,-0.476923076923077,-0.461538461538462,
-0.446153846153846,-0.430769230769231,-0.415384615384615,-0.4,-0.384615384615385,
-0.369230769230769,-0.353846153846154,-0.338461538461538,-0.323076923076923,
-0.307692307692308,-0.292307692307692,-0.276923076923077,-0.261538461538462,
-0.246153846153846,-0.230769230769231,-0.215384615384615,-0.2,-0.184615384615385,
-0.169230769230769,-0.153846153846154,-0.138461538461538,-0.123076923076923,
-0.107692307692308,-0.0923076923076923,-0.0769230769230769,-0.0615384615384615,
-0.0461538461538462,-0.0307692307692308,-0.0153846153846154,0.),
 .UNSPECIFIED.)
CURVE()
GEOMETRIC_REPRESENTATION_ITEM()
RATIONAL_B_SPLINE_CURVE((1.,1.,1.,1.,1.,1.,1.,1.,1.,1.,1.,1.,1.,1.,1.,1.,
1.,1.,1.,1.,1.,1.,1.,1.,1.,1.,1.,1.,1.,1.,1.,1.,1.,1.,1.,1.,1.,1.,1.,1.,
1.,1.,1.,1.,1.,1.,1.,1.,1.,1.,1.,1.,1.,1.,1.,1.,1.,1.,1.,1.,1.,1.,1.,1.,
1.,1.,1.,1.,1.,1.))
REPRESENTATION_ITEM('')
);
#477=(
BOUNDED_CURVE()
B_SPLINE_CURVE(5,(#70212,#70213,#70214,#70215,#70216,#70217,#70218,#70219,
#70220,#70221,#70222,#70223,#70224,#70225,#70226,#70227,#70228,#70229,#70230,
#70231,#70232,#70233,#70234,#70235,#70236,#70237,#70238,#70239,#70240,#70241,
#70242,#70243,#70244,#70245,#70246,#70247,#70248,#70249,#70250,#70251,#70252,
#70253,#70254,#70255,#70256,#70257,#70258,#70259,#70260,#70261,#70262,#70263,
#70264,#70265,#70266,#70267,#70268,#70269,#70270,#70271,#70272,#70273,#70274,
#70275,#70276,#70277,#70278,#70279,#70280,#70281),.UNSPECIFIED.,.F.,.F.)
B_SPLINE_CURVE_WITH_KNOTS((6,1,1,1,1,1,1,1,1,1,1,1,1,1,1,1,1,1,1,1,1,1,
1,1,1,1,1,1,1,1,1,1,1,1,1,1,1,1,1,1,1,1,1,1,1,1,1,1,1,1,1,1,1,1,1,1,1,1,
1,1,1,1,1,1,1,6),(-1.,-0.984615384615383,-0.969230769230768,-0.953846153846152,
-0.938461538461537,-0.923076923076922,-0.907692307692306,-0.892307692307691,
-0.876923076923076,-0.86153846153846,-0.846153846153845,-0.83076923076923,
-0.815384615384614,-0.799999999999999,-0.784615384615384,-0.769230769230768,
-0.753846153846153,-0.738461538461538,-0.723076923076922,-0.707692307692307,
-0.692307692307692,-0.676923076923076,-0.661538461538461,-0.646153846153846,
-0.63076923076923,-0.615384615384615,-0.6,-0.584615384615384,-0.569230769230769,
-0.553846153846154,-0.538461538461538,-0.523076923076923,-0.507692307692308,
-0.492307692307692,-0.476923076923077,-0.461538461538462,-0.446153846153846,
-0.430769230769231,-0.415384615384615,-0.4,-0.384615384615385,-0.369230769230769,
-0.353846153846154,-0.338461538461538,-0.323076923076923,-0.307692307692308,
-0.292307692307692,-0.276923076923077,-0.261538461538462,-0.246153846153846,
-0.230769230769231,-0.215384615384615,-0.2,-0.184615384615385,-0.169230769230769,
-0.153846153846154,-0.138461538461538,-0.123076923076923,-0.107692307692308,
-0.0923076923076923,-0.0769230769230769,-0.0615384615384615,-0.0461538461538462,
-0.0307692307692308,-0.0153846153846154,-0.0057718433744938),
 .UNSPECIFIED.)
CURVE()
GEOMETRIC_REPRESENTATION_ITEM()
RATIONAL_B_SPLINE_CURVE((1.,1.,1.,1.,1.,1.,1.,1.,1.,1.,1.,1.,1.,1.,1.,1.,
1.,1.,1.,1.,1.,1.,1.,1.,1.,1.,1.,1.,1.,1.,1.,1.,1.,1.,1.,1.,1.,1.,1.,1.,
1.,1.,1.,1.,1.,1.,1.,1.,1.,1.,1.,1.,1.,1.,1.,1.,1.,1.,1.,1.,1.,1.,1.,1.,
1.,1.,1.,1.,1.,1.))
REPRESENTATION_ITEM('')
);
#478=(
BOUNDED_CURVE()
B_SPLINE_CURVE(5,(#70432,#70433,#70434,#70435,#70436,#70437,#70438,#70439,
#70440,#70441,#70442,#70443,#70444,#70445,#70446,#70447,#70448,#70449,#70450,
#70451,#70452,#70453,#70454,#70455,#70456,#70457,#70458,#70459,#70460,#70461,
#70462,#70463,#70464,#70465,#70466,#70467,#70468,#70469,#70470,#70471,#70472,
#70473,#70474,#70475,#70476,#70477,#70478,#70479,#70480,#70481,#70482,#70483,
#70484,#70485,#70486,#70487,#70488,#70489,#70490,#70491,#70492,#70493,#70494,
#70495,#70496,#70497,#70498,#70499,#70500,#70501),.UNSPECIFIED.,.F.,.F.)
B_SPLINE_CURVE_WITH_KNOTS((6,1,1,1,1,1,1,1,1,1,1,1,1,1,1,1,1,1,1,1,1,1,
1,1,1,1,1,1,1,1,1,1,1,1,1,1,1,1,1,1,1,1,1,1,1,1,1,1,1,1,1,1,1,1,1,1,1,1,
1,1,1,1,1,1,1,6),(-0.994228156739743,-0.984615384615383,-0.969230769230768,
-0.953846153846152,-0.938461538461537,-0.923076923076922,-0.907692307692306,
-0.892307692307691,-0.876923076923076,-0.86153846153846,-0.846153846153845,
-0.83076923076923,-0.815384615384614,-0.799999999999999,-0.784615384615384,
-0.769230769230768,-0.753846153846153,-0.738461538461538,-0.723076923076922,
-0.707692307692307,-0.692307692307692,-0.676923076923076,-0.661538461538461,
-0.646153846153846,-0.63076923076923,-0.615384615384615,-0.6,-0.584615384615384,
-0.569230769230769,-0.553846153846154,-0.538461538461538,-0.523076923076923,
-0.507692307692308,-0.492307692307692,-0.476923076923077,-0.461538461538462,
-0.446153846153846,-0.430769230769231,-0.415384615384615,-0.4,-0.384615384615385,
-0.369230769230769,-0.353846153846154,-0.338461538461538,-0.323076923076923,
-0.307692307692308,-0.292307692307692,-0.276923076923077,-0.261538461538462,
-0.246153846153846,-0.230769230769231,-0.215384615384615,-0.2,-0.184615384615385,
-0.169230769230769,-0.153846153846154,-0.138461538461538,-0.123076923076923,
-0.107692307692308,-0.0923076923076923,-0.0769230769230769,-0.0615384615384615,
-0.0461538461538462,-0.0307692307692308,-0.0153846153846154,0.),
 .UNSPECIFIED.)
CURVE()
GEOMETRIC_REPRESENTATION_ITEM()
RATIONAL_B_SPLINE_CURVE((1.,1.,1.,1.,1.,1.,1.,1.,1.,1.,1.,1.,1.,1.,1.,1.,
1.,1.,1.,1.,1.,1.,1.,1.,1.,1.,1.,1.,1.,1.,1.,1.,1.,1.,1.,1.,1.,1.,1.,1.,
1.,1.,1.,1.,1.,1.,1.,1.,1.,1.,1.,1.,1.,1.,1.,1.,1.,1.,1.,1.,1.,1.,1.,1.,
1.,1.,1.,1.,1.,1.))
REPRESENTATION_ITEM('')
);
#479=(
BOUNDED_CURVE()
B_SPLINE_CURVE(5,(#70654,#70655,#70656,#70657,#70658,#70659,#70660,#70661,
#70662,#70663,#70664,#70665,#70666,#70667,#70668,#70669,#70670,#70671,#70672,
#70673,#70674,#70675,#70676,#70677,#70678,#70679,#70680,#70681,#70682,#70683,
#70684,#70685,#70686,#70687,#70688,#70689,#70690,#70691,#70692,#70693,#70694,
#70695,#70696,#70697,#70698,#70699,#70700,#70701,#70702,#70703,#70704,#70705,
#70706,#70707,#70708,#70709,#70710,#70711,#70712,#70713,#70714,#70715,#70716,
#70717,#70718,#70719,#70720,#70721,#70722,#70723),.UNSPECIFIED.,.F.,.F.)
B_SPLINE_CURVE_WITH_KNOTS((6,1,1,1,1,1,1,1,1,1,1,1,1,1,1,1,1,1,1,1,1,1,
1,1,1,1,1,1,1,1,1,1,1,1,1,1,1,1,1,1,1,1,1,1,1,1,1,1,1,1,1,1,1,1,1,1,1,1,
1,1,1,1,1,1,1,6),(-1.,-0.984615384615383,-0.969230769230768,-0.953846153846152,
-0.938461538461537,-0.923076923076922,-0.907692307692306,-0.892307692307691,
-0.876923076923076,-0.86153846153846,-0.846153846153845,-0.83076923076923,
-0.815384615384614,-0.799999999999999,-0.784615384615384,-0.769230769230768,
-0.753846153846153,-0.738461538461538,-0.723076923076922,-0.707692307692307,
-0.692307692307692,-0.676923076923076,-0.661538461538461,-0.646153846153846,
-0.63076923076923,-0.615384615384615,-0.6,-0.584615384615384,-0.569230769230769,
-0.553846153846154,-0.538461538461538,-0.523076923076923,-0.507692307692308,
-0.492307692307692,-0.476923076923077,-0.461538461538462,-0.446153846153846,
-0.430769230769231,-0.415384615384615,-0.4,-0.384615384615385,-0.369230769230769,
-0.353846153846154,-0.338461538461538,-0.323076923076923,-0.307692307692308,
-0.292307692307692,-0.276923076923077,-0.261538461538462,-0.246153846153846,
-0.230769230769231,-0.215384615384615,-0.2,-0.184615384615385,-0.169230769230769,
-0.153846153846154,-0.138461538461538,-0.123076923076923,-0.107692307692308,
-0.0923076923076923,-0.0769230769230769,-0.0615384615384615,-0.0461538461538462,
-0.0307692307692308,-0.0153846153846154,-0.0057718433745291),
 .UNSPECIFIED.)
CURVE()
GEOMETRIC_REPRESENTATION_ITEM()
RATIONAL_B_SPLINE_CURVE((1.,1.,1.,1.,1.,1.,1.,1.,1.,1.,1.,1.,1.,1.,1.,1.,
1.,1.,1.,1.,1.,1.,1.,1.,1.,1.,1.,1.,1.,1.,1.,1.,1.,1.,1.,1.,1.,1.,1.,1.,
1.,1.,1.,1.,1.,1.,1.,1.,1.,1.,1.,1.,1.,1.,1.,1.,1.,1.,1.,1.,1.,1.,1.,1.,
1.,1.,1.,1.,1.,1.))
REPRESENTATION_ITEM('')
);
#480=(
BOUNDED_CURVE()
B_SPLINE_CURVE(5,(#70874,#70875,#70876,#70877,#70878,#70879,#70880,#70881,
#70882,#70883,#70884,#70885,#70886,#70887,#70888,#70889,#70890,#70891,#70892,
#70893,#70894,#70895,#70896,#70897,#70898,#70899,#70900,#70901,#70902,#70903,
#70904,#70905,#70906,#70907,#70908,#70909,#70910,#70911,#70912,#70913,#70914,
#70915,#70916,#70917,#70918,#70919,#70920,#70921,#70922,#70923,#70924,#70925,
#70926,#70927,#70928,#70929,#70930,#70931,#70932,#70933,#70934,#70935,#70936,
#70937,#70938,#70939,#70940,#70941,#70942,#70943),.UNSPECIFIED.,.F.,.F.)
B_SPLINE_CURVE_WITH_KNOTS((6,1,1,1,1,1,1,1,1,1,1,1,1,1,1,1,1,1,1,1,1,1,
1,1,1,1,1,1,1,1,1,1,1,1,1,1,1,1,1,1,1,1,1,1,1,1,1,1,1,1,1,1,1,1,1,1,1,1,
1,1,1,1,1,1,1,6),(-0.994228156739665,-0.984615384615383,-0.969230769230768,
-0.953846153846152,-0.938461538461537,-0.923076923076922,-0.907692307692306,
-0.892307692307691,-0.876923076923076,-0.86153846153846,-0.846153846153845,
-0.83076923076923,-0.815384615384614,-0.799999999999999,-0.784615384615384,
-0.769230769230768,-0.753846153846153,-0.738461538461538,-0.723076923076922,
-0.707692307692307,-0.692307692307692,-0.676923076923076,-0.661538461538461,
-0.646153846153846,-0.63076923076923,-0.615384615384615,-0.6,-0.584615384615384,
-0.569230769230769,-0.553846153846154,-0.538461538461538,-0.523076923076923,
-0.507692307692308,-0.492307692307692,-0.476923076923077,-0.461538461538462,
-0.446153846153846,-0.430769230769231,-0.415384615384615,-0.4,-0.384615384615385,
-0.369230769230769,-0.353846153846154,-0.338461538461538,-0.323076923076923,
-0.307692307692308,-0.292307692307692,-0.276923076923077,-0.261538461538462,
-0.246153846153846,-0.230769230769231,-0.215384615384615,-0.2,-0.184615384615385,
-0.169230769230769,-0.153846153846154,-0.138461538461538,-0.123076923076923,
-0.107692307692308,-0.0923076923076923,-0.0769230769230769,-0.0615384615384615,
-0.0461538461538462,-0.0307692307692308,-0.0153846153846154,0.),
 .UNSPECIFIED.)
CURVE()
GEOMETRIC_REPRESENTATION_ITEM()
RATIONAL_B_SPLINE_CURVE((1.,1.,1.,1.,1.,1.,1.,1.,1.,1.,1.,1.,1.,1.,1.,1.,
1.,1.,1.,1.,1.,1.,1.,1.,1.,1.,1.,1.,1.,1.,1.,1.,1.,1.,1.,1.,1.,1.,1.,1.,
1.,1.,1.,1.,1.,1.,1.,1.,1.,1.,1.,1.,1.,1.,1.,1.,1.,1.,1.,1.,1.,1.,1.,1.,
1.,1.,1.,1.,1.,1.))
REPRESENTATION_ITEM('')
);
#481=(
BOUNDED_CURVE()
B_SPLINE_CURVE(5,(#71096,#71097,#71098,#71099,#71100,#71101,#71102,#71103,
#71104,#71105,#71106,#71107,#71108,#71109,#71110,#71111,#71112,#71113,#71114,
#71115,#71116,#71117,#71118,#71119,#71120,#71121,#71122,#71123,#71124,#71125,
#71126,#71127,#71128,#71129,#71130,#71131,#71132,#71133,#71134,#71135,#71136,
#71137,#71138,#71139,#71140,#71141,#71142,#71143,#71144,#71145,#71146,#71147,
#71148,#71149,#71150,#71151,#71152,#71153,#71154,#71155,#71156,#71157,#71158,
#71159,#71160,#71161,#71162,#71163,#71164,#71165),.UNSPECIFIED.,.F.,.F.)
B_SPLINE_CURVE_WITH_KNOTS((6,1,1,1,1,1,1,1,1,1,1,1,1,1,1,1,1,1,1,1,1,1,
1,1,1,1,1,1,1,1,1,1,1,1,1,1,1,1,1,1,1,1,1,1,1,1,1,1,1,1,1,1,1,1,1,1,1,1,
1,1,1,1,1,1,1,6),(-1.,-0.984615384615383,-0.969230769230768,-0.953846153846152,
-0.938461538461537,-0.923076923076922,-0.907692307692306,-0.892307692307691,
-0.876923076923076,-0.86153846153846,-0.846153846153845,-0.83076923076923,
-0.815384615384614,-0.799999999999999,-0.784615384615384,-0.769230769230768,
-0.753846153846153,-0.738461538461538,-0.723076923076922,-0.707692307692307,
-0.692307692307692,-0.676923076923076,-0.661538461538461,-0.646153846153846,
-0.63076923076923,-0.615384615384615,-0.6,-0.584615384615384,-0.569230769230769,
-0.553846153846154,-0.538461538461538,-0.523076923076923,-0.507692307692308,
-0.492307692307692,-0.476923076923077,-0.461538461538462,-0.446153846153846,
-0.430769230769231,-0.415384615384615,-0.4,-0.384615384615385,-0.369230769230769,
-0.353846153846154,-0.338461538461538,-0.323076923076923,-0.307692307692308,
-0.292307692307692,-0.276923076923077,-0.261538461538462,-0.246153846153846,
-0.230769230769231,-0.215384615384615,-0.2,-0.184615384615385,-0.169230769230769,
-0.153846153846154,-0.138461538461538,-0.123076923076923,-0.107692307692308,
-0.0923076923076923,-0.0769230769230769,-0.0615384615384615,-0.0461538461538462,
-0.0307692307692308,-0.0153846153846154,-0.00577184337450666),
 .UNSPECIFIED.)
CURVE()
GEOMETRIC_REPRESENTATION_ITEM()
RATIONAL_B_SPLINE_CURVE((1.,1.,1.,1.,1.,1.,1.,1.,1.,1.,1.,1.,1.,1.,1.,1.,
1.,1.,1.,1.,1.,1.,1.,1.,1.,1.,1.,1.,1.,1.,1.,1.,1.,1.,1.,1.,1.,1.,1.,1.,
1.,1.,1.,1.,1.,1.,1.,1.,1.,1.,1.,1.,1.,1.,1.,1.,1.,1.,1.,1.,1.,1.,1.,1.,
1.,1.,1.,1.,1.,1.))
REPRESENTATION_ITEM('')
);
#482=(
BOUNDED_CURVE()
B_SPLINE_CURVE(5,(#71316,#71317,#71318,#71319,#71320,#71321,#71322,#71323,
#71324,#71325,#71326,#71327,#71328,#71329,#71330,#71331,#71332,#71333,#71334,
#71335,#71336,#71337,#71338,#71339,#71340,#71341,#71342,#71343,#71344,#71345,
#71346,#71347,#71348,#71349,#71350,#71351,#71352,#71353,#71354,#71355,#71356,
#71357,#71358,#71359,#71360,#71361,#71362,#71363,#71364,#71365,#71366,#71367,
#71368,#71369,#71370,#71371,#71372,#71373,#71374,#71375,#71376,#71377,#71378,
#71379,#71380,#71381,#71382,#71383,#71384,#71385),.UNSPECIFIED.,.F.,.F.)
B_SPLINE_CURVE_WITH_KNOTS((6,1,1,1,1,1,1,1,1,1,1,1,1,1,1,1,1,1,1,1,1,1,
1,1,1,1,1,1,1,1,1,1,1,1,1,1,1,1,1,1,1,1,1,1,1,1,1,1,1,1,1,1,1,1,1,1,1,1,
1,1,1,1,1,1,1,6),(-0.994228156739758,-0.984615384615383,-0.969230769230768,
-0.953846153846152,-0.938461538461537,-0.923076923076922,-0.907692307692306,
-0.892307692307691,-0.876923076923076,-0.86153846153846,-0.846153846153845,
-0.83076923076923,-0.815384615384614,-0.799999999999999,-0.784615384615384,
-0.769230769230768,-0.753846153846153,-0.738461538461538,-0.723076923076922,
-0.707692307692307,-0.692307692307692,-0.676923076923076,-0.661538461538461,
-0.646153846153846,-0.63076923076923,-0.615384615384615,-0.6,-0.584615384615384,
-0.569230769230769,-0.553846153846154,-0.538461538461538,-0.523076923076923,
-0.507692307692308,-0.492307692307692,-0.476923076923077,-0.461538461538462,
-0.446153846153846,-0.430769230769231,-0.415384615384615,-0.4,-0.384615384615385,
-0.369230769230769,-0.353846153846154,-0.338461538461538,-0.323076923076923,
-0.307692307692308,-0.292307692307692,-0.276923076923077,-0.261538461538462,
-0.246153846153846,-0.230769230769231,-0.215384615384615,-0.2,-0.184615384615385,
-0.169230769230769,-0.153846153846154,-0.138461538461538,-0.123076923076923,
-0.107692307692308,-0.0923076923076923,-0.0769230769230769,-0.0615384615384615,
-0.0461538461538462,-0.0307692307692308,-0.0153846153846154,0.),
 .UNSPECIFIED.)
CURVE()
GEOMETRIC_REPRESENTATION_ITEM()
RATIONAL_B_SPLINE_CURVE((1.,1.,1.,1.,1.,1.,1.,1.,1.,1.,1.,1.,1.,1.,1.,1.,
1.,1.,1.,1.,1.,1.,1.,1.,1.,1.,1.,1.,1.,1.,1.,1.,1.,1.,1.,1.,1.,1.,1.,1.,
1.,1.,1.,1.,1.,1.,1.,1.,1.,1.,1.,1.,1.,1.,1.,1.,1.,1.,1.,1.,1.,1.,1.,1.,
1.,1.,1.,1.,1.,1.))
REPRESENTATION_ITEM('')
);
#483=(
BOUNDED_CURVE()
B_SPLINE_CURVE(5,(#71538,#71539,#71540,#71541,#71542,#71543,#71544,#71545,
#71546,#71547,#71548,#71549,#71550,#71551,#71552,#71553,#71554,#71555,#71556,
#71557,#71558,#71559,#71560,#71561,#71562,#71563,#71564,#71565,#71566,#71567,
#71568,#71569,#71570,#71571,#71572,#71573,#71574,#71575,#71576,#71577,#71578,
#71579,#71580,#71581,#71582,#71583,#71584,#71585,#71586,#71587,#71588,#71589,
#71590,#71591,#71592,#71593,#71594,#71595,#71596,#71597,#71598,#71599,#71600,
#71601,#71602,#71603,#71604,#71605,#71606,#71607),.UNSPECIFIED.,.F.,.F.)
B_SPLINE_CURVE_WITH_KNOTS((6,1,1,1,1,1,1,1,1,1,1,1,1,1,1,1,1,1,1,1,1,1,
1,1,1,1,1,1,1,1,1,1,1,1,1,1,1,1,1,1,1,1,1,1,1,1,1,1,1,1,1,1,1,1,1,1,1,1,
1,1,1,1,1,1,1,6),(-1.,-0.984615384615383,-0.969230769230768,-0.953846153846152,
-0.938461538461537,-0.923076923076922,-0.907692307692306,-0.892307692307691,
-0.876923076923076,-0.86153846153846,-0.846153846153845,-0.83076923076923,
-0.815384615384614,-0.799999999999999,-0.784615384615384,-0.769230769230768,
-0.753846153846153,-0.738461538461538,-0.723076923076922,-0.707692307692307,
-0.692307692307692,-0.676923076923076,-0.661538461538461,-0.646153846153846,
-0.63076923076923,-0.615384615384615,-0.6,-0.584615384615384,-0.569230769230769,
-0.553846153846154,-0.538461538461538,-0.523076923076923,-0.507692307692308,
-0.492307692307692,-0.476923076923077,-0.461538461538462,-0.446153846153846,
-0.430769230769231,-0.415384615384615,-0.4,-0.384615384615385,-0.369230769230769,
-0.353846153846154,-0.338461538461538,-0.323076923076923,-0.307692307692308,
-0.292307692307692,-0.276923076923077,-0.261538461538462,-0.246153846153846,
-0.230769230769231,-0.215384615384615,-0.2,-0.184615384615385,-0.169230769230769,
-0.153846153846154,-0.138461538461538,-0.123076923076923,-0.107692307692308,
-0.0923076923076923,-0.0769230769230769,-0.0615384615384615,-0.0461538461538462,
-0.0307692307692308,-0.0153846153846154,-0.00577184337451981),
 .UNSPECIFIED.)
CURVE()
GEOMETRIC_REPRESENTATION_ITEM()
RATIONAL_B_SPLINE_CURVE((1.,1.,1.,1.,1.,1.,1.,1.,1.,1.,1.,1.,1.,1.,1.,1.,
1.,1.,1.,1.,1.,1.,1.,1.,1.,1.,1.,1.,1.,1.,1.,1.,1.,1.,1.,1.,1.,1.,1.,1.,
1.,1.,1.,1.,1.,1.,1.,1.,1.,1.,1.,1.,1.,1.,1.,1.,1.,1.,1.,1.,1.,1.,1.,1.,
1.,1.,1.,1.,1.,1.))
REPRESENTATION_ITEM('')
);
#484=(
BOUNDED_CURVE()
B_SPLINE_CURVE(5,(#71758,#71759,#71760,#71761,#71762,#71763,#71764,#71765,
#71766,#71767,#71768,#71769,#71770,#71771,#71772,#71773,#71774,#71775,#71776,
#71777,#71778,#71779,#71780,#71781,#71782,#71783,#71784,#71785,#71786,#71787,
#71788,#71789,#71790,#71791,#71792,#71793,#71794,#71795,#71796,#71797,#71798,
#71799,#71800,#71801,#71802,#71803,#71804,#71805,#71806,#71807,#71808,#71809,
#71810,#71811,#71812,#71813,#71814,#71815,#71816,#71817,#71818,#71819,#71820,
#71821,#71822,#71823,#71824,#71825,#71826,#71827),.UNSPECIFIED.,.F.,.F.)
B_SPLINE_CURVE_WITH_KNOTS((6,1,1,1,1,1,1,1,1,1,1,1,1,1,1,1,1,1,1,1,1,1,
1,1,1,1,1,1,1,1,1,1,1,1,1,1,1,1,1,1,1,1,1,1,1,1,1,1,1,1,1,1,1,1,1,1,1,1,
1,1,1,1,1,1,1,6),(-0.994228156739659,-0.984615384615383,-0.969230769230768,
-0.953846153846152,-0.938461538461537,-0.923076923076922,-0.907692307692306,
-0.892307692307691,-0.876923076923076,-0.86153846153846,-0.846153846153845,
-0.83076923076923,-0.815384615384614,-0.799999999999999,-0.784615384615384,
-0.769230769230768,-0.753846153846153,-0.738461538461538,-0.723076923076922,
-0.707692307692307,-0.692307692307692,-0.676923076923076,-0.661538461538461,
-0.646153846153846,-0.63076923076923,-0.615384615384615,-0.6,-0.584615384615384,
-0.569230769230769,-0.553846153846154,-0.538461538461538,-0.523076923076923,
-0.507692307692308,-0.492307692307692,-0.476923076923077,-0.461538461538462,
-0.446153846153846,-0.430769230769231,-0.415384615384615,-0.4,-0.384615384615385,
-0.369230769230769,-0.353846153846154,-0.338461538461538,-0.323076923076923,
-0.307692307692308,-0.292307692307692,-0.276923076923077,-0.261538461538462,
-0.246153846153846,-0.230769230769231,-0.215384615384615,-0.2,-0.184615384615385,
-0.169230769230769,-0.153846153846154,-0.138461538461538,-0.123076923076923,
-0.107692307692308,-0.0923076923076923,-0.0769230769230769,-0.0615384615384615,
-0.0461538461538462,-0.0307692307692308,-0.0153846153846154,0.),
 .UNSPECIFIED.)
CURVE()
GEOMETRIC_REPRESENTATION_ITEM()
RATIONAL_B_SPLINE_CURVE((1.,1.,1.,1.,1.,1.,1.,1.,1.,1.,1.,1.,1.,1.,1.,1.,
1.,1.,1.,1.,1.,1.,1.,1.,1.,1.,1.,1.,1.,1.,1.,1.,1.,1.,1.,1.,1.,1.,1.,1.,
1.,1.,1.,1.,1.,1.,1.,1.,1.,1.,1.,1.,1.,1.,1.,1.,1.,1.,1.,1.,1.,1.,1.,1.,
1.,1.,1.,1.,1.,1.))
REPRESENTATION_ITEM('')
);
#485=(
BOUNDED_CURVE()
B_SPLINE_CURVE(5,(#71980,#71981,#71982,#71983,#71984,#71985,#71986,#71987,
#71988,#71989,#71990,#71991,#71992,#71993,#71994,#71995,#71996,#71997,#71998,
#71999,#72000,#72001,#72002,#72003,#72004,#72005,#72006,#72007,#72008,#72009,
#72010,#72011,#72012,#72013,#72014,#72015,#72016,#72017,#72018,#72019,#72020,
#72021,#72022,#72023,#72024,#72025,#72026,#72027,#72028,#72029,#72030,#72031,
#72032,#72033,#72034,#72035,#72036,#72037,#72038,#72039,#72040,#72041,#72042,
#72043,#72044,#72045,#72046,#72047,#72048,#72049),.UNSPECIFIED.,.F.,.F.)
B_SPLINE_CURVE_WITH_KNOTS((6,1,1,1,1,1,1,1,1,1,1,1,1,1,1,1,1,1,1,1,1,1,
1,1,1,1,1,1,1,1,1,1,1,1,1,1,1,1,1,1,1,1,1,1,1,1,1,1,1,1,1,1,1,1,1,1,1,1,
1,1,1,1,1,1,1,6),(-1.,-0.984615384615383,-0.969230769230768,-0.953846153846152,
-0.938461538461537,-0.923076923076922,-0.907692307692306,-0.892307692307691,
-0.876923076923076,-0.86153846153846,-0.846153846153845,-0.83076923076923,
-0.815384615384614,-0.799999999999999,-0.784615384615384,-0.769230769230768,
-0.753846153846153,-0.738461538461538,-0.723076923076922,-0.707692307692307,
-0.692307692307692,-0.676923076923076,-0.661538461538461,-0.646153846153846,
-0.63076923076923,-0.615384615384615,-0.6,-0.584615384615384,-0.569230769230769,
-0.553846153846154,-0.538461538461538,-0.523076923076923,-0.507692307692308,
-0.492307692307692,-0.476923076923077,-0.461538461538462,-0.446153846153846,
-0.430769230769231,-0.415384615384615,-0.4,-0.384615384615385,-0.369230769230769,
-0.353846153846154,-0.338461538461538,-0.323076923076923,-0.307692307692308,
-0.292307692307692,-0.276923076923077,-0.261538461538462,-0.246153846153846,
-0.230769230769231,-0.215384615384615,-0.2,-0.184615384615385,-0.169230769230769,
-0.153846153846154,-0.138461538461538,-0.123076923076923,-0.107692307692308,
-0.0923076923076923,-0.0769230769230769,-0.0615384615384615,-0.0461538461538462,
-0.0307692307692308,-0.0153846153846154,-0.00577184337450306),
 .UNSPECIFIED.)
CURVE()
GEOMETRIC_REPRESENTATION_ITEM()
RATIONAL_B_SPLINE_CURVE((1.,1.,1.,1.,1.,1.,1.,1.,1.,1.,1.,1.,1.,1.,1.,1.,
1.,1.,1.,1.,1.,1.,1.,1.,1.,1.,1.,1.,1.,1.,1.,1.,1.,1.,1.,1.,1.,1.,1.,1.,
1.,1.,1.,1.,1.,1.,1.,1.,1.,1.,1.,1.,1.,1.,1.,1.,1.,1.,1.,1.,1.,1.,1.,1.,
1.,1.,1.,1.,1.,1.))
REPRESENTATION_ITEM('')
);
#486=(
BOUNDED_CURVE()
B_SPLINE_CURVE(5,(#72200,#72201,#72202,#72203,#72204,#72205,#72206,#72207,
#72208,#72209,#72210,#72211,#72212,#72213,#72214,#72215,#72216,#72217,#72218,
#72219,#72220,#72221,#72222,#72223,#72224,#72225,#72226,#72227,#72228,#72229,
#72230,#72231,#72232,#72233,#72234,#72235,#72236,#72237,#72238,#72239,#72240,
#72241,#72242,#72243,#72244,#72245,#72246,#72247,#72248,#72249,#72250,#72251,
#72252,#72253,#72254,#72255,#72256,#72257,#72258,#72259,#72260,#72261,#72262,
#72263,#72264,#72265,#72266,#72267,#72268,#72269),.UNSPECIFIED.,.F.,.F.)
B_SPLINE_CURVE_WITH_KNOTS((6,1,1,1,1,1,1,1,1,1,1,1,1,1,1,1,1,1,1,1,1,1,
1,1,1,1,1,1,1,1,1,1,1,1,1,1,1,1,1,1,1,1,1,1,1,1,1,1,1,1,1,1,1,1,1,1,1,1,
1,1,1,1,1,1,1,6),(-0.994228156739675,-0.984615384615383,-0.969230769230768,
-0.953846153846152,-0.938461538461537,-0.923076923076922,-0.907692307692306,
-0.892307692307691,-0.876923076923076,-0.86153846153846,-0.846153846153845,
-0.83076923076923,-0.815384615384614,-0.799999999999999,-0.784615384615384,
-0.769230769230768,-0.753846153846153,-0.738461538461538,-0.723076923076922,
-0.707692307692307,-0.692307692307692,-0.676923076923076,-0.661538461538461,
-0.646153846153846,-0.63076923076923,-0.615384615384615,-0.6,-0.584615384615384,
-0.569230769230769,-0.553846153846154,-0.538461538461538,-0.523076923076923,
-0.507692307692308,-0.492307692307692,-0.476923076923077,-0.461538461538462,
-0.446153846153846,-0.430769230769231,-0.415384615384615,-0.4,-0.384615384615385,
-0.369230769230769,-0.353846153846154,-0.338461538461538,-0.323076923076923,
-0.307692307692308,-0.292307692307692,-0.276923076923077,-0.261538461538462,
-0.246153846153846,-0.230769230769231,-0.215384615384615,-0.2,-0.184615384615385,
-0.169230769230769,-0.153846153846154,-0.138461538461538,-0.123076923076923,
-0.107692307692308,-0.0923076923076923,-0.0769230769230769,-0.0615384615384615,
-0.0461538461538462,-0.0307692307692308,-0.0153846153846154,0.),
 .UNSPECIFIED.)
CURVE()
GEOMETRIC_REPRESENTATION_ITEM()
RATIONAL_B_SPLINE_CURVE((1.,1.,1.,1.,1.,1.,1.,1.,1.,1.,1.,1.,1.,1.,1.,1.,
1.,1.,1.,1.,1.,1.,1.,1.,1.,1.,1.,1.,1.,1.,1.,1.,1.,1.,1.,1.,1.,1.,1.,1.,
1.,1.,1.,1.,1.,1.,1.,1.,1.,1.,1.,1.,1.,1.,1.,1.,1.,1.,1.,1.,1.,1.,1.,1.,
1.,1.,1.,1.,1.,1.))
REPRESENTATION_ITEM('')
);
#487=(
BOUNDED_CURVE()
B_SPLINE_CURVE(5,(#72422,#72423,#72424,#72425,#72426,#72427,#72428,#72429,
#72430,#72431,#72432,#72433,#72434,#72435,#72436,#72437,#72438,#72439,#72440,
#72441,#72442,#72443,#72444,#72445,#72446,#72447,#72448,#72449,#72450,#72451,
#72452,#72453,#72454,#72455,#72456,#72457,#72458,#72459,#72460,#72461,#72462,
#72463,#72464,#72465,#72466,#72467,#72468,#72469,#72470,#72471,#72472,#72473,
#72474,#72475,#72476,#72477,#72478,#72479,#72480,#72481,#72482,#72483,#72484,
#72485,#72486,#72487,#72488,#72489,#72490,#72491),.UNSPECIFIED.,.F.,.F.)
B_SPLINE_CURVE_WITH_KNOTS((6,1,1,1,1,1,1,1,1,1,1,1,1,1,1,1,1,1,1,1,1,1,
1,1,1,1,1,1,1,1,1,1,1,1,1,1,1,1,1,1,1,1,1,1,1,1,1,1,1,1,1,1,1,1,1,1,1,1,
1,1,1,1,1,1,1,6),(-1.,-0.984615384615383,-0.969230769230768,-0.953846153846152,
-0.938461538461537,-0.923076923076922,-0.907692307692306,-0.892307692307691,
-0.876923076923076,-0.86153846153846,-0.846153846153845,-0.83076923076923,
-0.815384615384614,-0.799999999999999,-0.784615384615384,-0.769230769230768,
-0.753846153846153,-0.738461538461538,-0.723076923076922,-0.707692307692307,
-0.692307692307692,-0.676923076923076,-0.661538461538461,-0.646153846153846,
-0.63076923076923,-0.615384615384615,-0.6,-0.584615384615384,-0.569230769230769,
-0.553846153846154,-0.538461538461538,-0.523076923076923,-0.507692307692308,
-0.492307692307692,-0.476923076923077,-0.461538461538462,-0.446153846153846,
-0.430769230769231,-0.415384615384615,-0.4,-0.384615384615385,-0.369230769230769,
-0.353846153846154,-0.338461538461538,-0.323076923076923,-0.307692307692308,
-0.292307692307692,-0.276923076923077,-0.261538461538462,-0.246153846153846,
-0.230769230769231,-0.215384615384615,-0.2,-0.184615384615385,-0.169230769230769,
-0.153846153846154,-0.138461538461538,-0.123076923076923,-0.107692307692308,
-0.0923076923076923,-0.0769230769230769,-0.0615384615384615,-0.0461538461538462,
-0.0307692307692308,-0.0153846153846154,-0.00577184337450328),
 .UNSPECIFIED.)
CURVE()
GEOMETRIC_REPRESENTATION_ITEM()
RATIONAL_B_SPLINE_CURVE((1.,1.,1.,1.,1.,1.,1.,1.,1.,1.,1.,1.,1.,1.,1.,1.,
1.,1.,1.,1.,1.,1.,1.,1.,1.,1.,1.,1.,1.,1.,1.,1.,1.,1.,1.,1.,1.,1.,1.,1.,
1.,1.,1.,1.,1.,1.,1.,1.,1.,1.,1.,1.,1.,1.,1.,1.,1.,1.,1.,1.,1.,1.,1.,1.,
1.,1.,1.,1.,1.,1.))
REPRESENTATION_ITEM('')
);
#488=(
BOUNDED_CURVE()
B_SPLINE_CURVE(5,(#72644,#72645,#72646,#72647,#72648,#72649,#72650,#72651,
#72652,#72653,#72654,#72655,#72656,#72657,#72658,#72659,#72660,#72661,#72662,
#72663,#72664,#72665,#72666,#72667,#72668,#72669,#72670,#72671,#72672,#72673,
#72674,#72675,#72676,#72677,#72678,#72679,#72680,#72681,#72682,#72683,#72684,
#72685,#72686,#72687,#72688,#72689,#72690,#72691,#72692,#72693,#72694,#72695,
#72696,#72697,#72698,#72699,#72700,#72701,#72702,#72703,#72704,#72705,#72706,
#72707,#72708,#72709,#72710,#72711,#72712,#72713),.UNSPECIFIED.,.F.,.F.)
B_SPLINE_CURVE_WITH_KNOTS((6,1,1,1,1,1,1,1,1,1,1,1,1,1,1,1,1,1,1,1,1,1,
1,1,1,1,1,1,1,1,1,1,1,1,1,1,1,1,1,1,1,1,1,1,1,1,1,1,1,1,1,1,1,1,1,1,1,1,
1,1,1,1,1,1,1,6),(-0.994228156739672,-0.984615384615383,-0.969230769230768,
-0.953846153846152,-0.938461538461537,-0.923076923076922,-0.907692307692306,
-0.892307692307691,-0.876923076923076,-0.86153846153846,-0.846153846153845,
-0.83076923076923,-0.815384615384614,-0.799999999999999,-0.784615384615384,
-0.769230769230768,-0.753846153846153,-0.738461538461538,-0.723076923076922,
-0.707692307692307,-0.692307692307692,-0.676923076923076,-0.661538461538461,
-0.646153846153846,-0.63076923076923,-0.615384615384615,-0.6,-0.584615384615384,
-0.569230769230769,-0.553846153846154,-0.538461538461538,-0.523076923076923,
-0.507692307692308,-0.492307692307692,-0.476923076923077,-0.461538461538462,
-0.446153846153846,-0.430769230769231,-0.415384615384615,-0.4,-0.384615384615385,
-0.369230769230769,-0.353846153846154,-0.338461538461538,-0.323076923076923,
-0.307692307692308,-0.292307692307692,-0.276923076923077,-0.261538461538462,
-0.246153846153846,-0.230769230769231,-0.215384615384615,-0.2,-0.184615384615385,
-0.169230769230769,-0.153846153846154,-0.138461538461538,-0.123076923076923,
-0.107692307692308,-0.0923076923076923,-0.0769230769230769,-0.0615384615384615,
-0.0461538461538462,-0.0307692307692308,-0.0153846153846154,0.),
 .UNSPECIFIED.)
CURVE()
GEOMETRIC_REPRESENTATION_ITEM()
RATIONAL_B_SPLINE_CURVE((1.,1.,1.,1.,1.,1.,1.,1.,1.,1.,1.,1.,1.,1.,1.,1.,
1.,1.,1.,1.,1.,1.,1.,1.,1.,1.,1.,1.,1.,1.,1.,1.,1.,1.,1.,1.,1.,1.,1.,1.,
1.,1.,1.,1.,1.,1.,1.,1.,1.,1.,1.,1.,1.,1.,1.,1.,1.,1.,1.,1.,1.,1.,1.,1.,
1.,1.,1.,1.,1.,1.))
REPRESENTATION_ITEM('')
);
#489=(
BOUNDED_CURVE()
B_SPLINE_CURVE(5,(#72872,#72873,#72874,#72875,#72876,#72877,#72878,#72879,
#72880,#72881,#72882,#72883,#72884,#72885,#72886,#72887,#72888,#72889,#72890,
#72891,#72892,#72893,#72894,#72895,#72896,#72897,#72898,#72899,#72900,#72901,
#72902,#72903,#72904,#72905,#72906,#72907,#72908,#72909,#72910,#72911,#72912,
#72913,#72914,#72915,#72916,#72917,#72918,#72919,#72920,#72921,#72922,#72923,
#72924,#72925,#72926,#72927,#72928,#72929,#72930,#72931,#72932,#72933,#72934,
#72935,#72936,#72937,#72938,#72939,#72940,#72941),.UNSPECIFIED.,.F.,.F.)
B_SPLINE_CURVE_WITH_KNOTS((6,1,1,1,1,1,1,1,1,1,1,1,1,1,1,1,1,1,1,1,1,1,
1,1,1,1,1,1,1,1,1,1,1,1,1,1,1,1,1,1,1,1,1,1,1,1,1,1,1,1,1,1,1,1,1,1,1,1,
1,1,1,1,1,1,1,6),(-0.994228156739704,-0.984615384615383,-0.969230769230768,
-0.953846153846152,-0.938461538461537,-0.923076923076922,-0.907692307692306,
-0.892307692307691,-0.876923076923076,-0.86153846153846,-0.846153846153845,
-0.83076923076923,-0.815384615384614,-0.799999999999999,-0.784615384615384,
-0.769230769230768,-0.753846153846153,-0.738461538461538,-0.723076923076922,
-0.707692307692307,-0.692307692307692,-0.676923076923076,-0.661538461538461,
-0.646153846153846,-0.63076923076923,-0.615384615384615,-0.6,-0.584615384615384,
-0.569230769230769,-0.553846153846154,-0.538461538461538,-0.523076923076923,
-0.507692307692308,-0.492307692307692,-0.476923076923077,-0.461538461538462,
-0.446153846153846,-0.430769230769231,-0.415384615384615,-0.4,-0.384615384615385,
-0.369230769230769,-0.353846153846154,-0.338461538461538,-0.323076923076923,
-0.307692307692308,-0.292307692307692,-0.276923076923077,-0.261538461538462,
-0.246153846153846,-0.230769230769231,-0.215384615384615,-0.2,-0.184615384615385,
-0.169230769230769,-0.153846153846154,-0.138461538461538,-0.123076923076923,
-0.107692307692308,-0.0923076923076923,-0.0769230769230769,-0.0615384615384615,
-0.0461538461538462,-0.0307692307692308,-0.0153846153846154,0.),
 .UNSPECIFIED.)
CURVE()
GEOMETRIC_REPRESENTATION_ITEM()
RATIONAL_B_SPLINE_CURVE((1.,1.,1.,1.,1.,1.,1.,1.,1.,1.,1.,1.,1.,1.,1.,1.,
1.,1.,1.,1.,1.,1.,1.,1.,1.,1.,1.,1.,1.,1.,1.,1.,1.,1.,1.,1.,1.,1.,1.,1.,
1.,1.,1.,1.,1.,1.,1.,1.,1.,1.,1.,1.,1.,1.,1.,1.,1.,1.,1.,1.,1.,1.,1.,1.,
1.,1.,1.,1.,1.,1.))
REPRESENTATION_ITEM('')
);
#490=(
BOUNDED_CURVE()
B_SPLINE_CURVE(5,(#73083,#73084,#73085,#73086,#73087,#73088,#73089,#73090,
#73091,#73092,#73093,#73094,#73095,#73096,#73097,#73098,#73099,#73100,#73101,
#73102,#73103,#73104,#73105,#73106,#73107,#73108,#73109,#73110,#73111,#73112,
#73113,#73114,#73115,#73116,#73117,#73118,#73119,#73120,#73121,#73122,#73123,
#73124,#73125,#73126,#73127,#73128,#73129,#73130,#73131,#73132,#73133,#73134,
#73135,#73136,#73137,#73138,#73139,#73140,#73141,#73142,#73143,#73144,#73145,
#73146,#73147,#73148,#73149,#73150,#73151,#73152),.UNSPECIFIED.,.F.,.F.)
B_SPLINE_CURVE_WITH_KNOTS((6,1,1,1,1,1,1,1,1,1,1,1,1,1,1,1,1,1,1,1,1,1,
1,1,1,1,1,1,1,1,1,1,1,1,1,1,1,1,1,1,1,1,1,1,1,1,1,1,1,1,1,1,1,1,1,1,1,1,
1,1,1,1,1,1,1,6),(-1.,-0.984615384615383,-0.969230769230768,-0.953846153846152,
-0.938461538461537,-0.923076923076922,-0.907692307692306,-0.892307692307691,
-0.876923076923076,-0.86153846153846,-0.846153846153845,-0.83076923076923,
-0.815384615384614,-0.799999999999999,-0.784615384615384,-0.769230769230768,
-0.753846153846153,-0.738461538461538,-0.723076923076922,-0.707692307692307,
-0.692307692307692,-0.676923076923076,-0.661538461538461,-0.646153846153846,
-0.63076923076923,-0.615384615384615,-0.6,-0.584615384615384,-0.569230769230769,
-0.553846153846154,-0.538461538461538,-0.523076923076923,-0.507692307692308,
-0.492307692307692,-0.476923076923077,-0.461538461538462,-0.446153846153846,
-0.430769230769231,-0.415384615384615,-0.4,-0.384615384615385,-0.369230769230769,
-0.353846153846154,-0.338461538461538,-0.323076923076923,-0.307692307692308,
-0.292307692307692,-0.276923076923077,-0.261538461538462,-0.246153846153846,
-0.230769230769231,-0.215384615384615,-0.2,-0.184615384615385,-0.169230769230769,
-0.153846153846154,-0.138461538461538,-0.123076923076923,-0.107692307692308,
-0.0923076923076923,-0.0769230769230769,-0.0615384615384615,-0.0461538461538462,
-0.0307692307692308,-0.0153846153846154,-0.00577184337451611),
 .UNSPECIFIED.)
CURVE()
GEOMETRIC_REPRESENTATION_ITEM()
RATIONAL_B_SPLINE_CURVE((1.,1.,1.,1.,1.,1.,1.,1.,1.,1.,1.,1.,1.,1.,1.,1.,
1.,1.,1.,1.,1.,1.,1.,1.,1.,1.,1.,1.,1.,1.,1.,1.,1.,1.,1.,1.,1.,1.,1.,1.,
1.,1.,1.,1.,1.,1.,1.,1.,1.,1.,1.,1.,1.,1.,1.,1.,1.,1.,1.,1.,1.,1.,1.,1.,
1.,1.,1.,1.,1.,1.))
REPRESENTATION_ITEM('')
);
#987=B_SPLINE_CURVE_WITH_KNOTS('',3,(#55619,#55620,#55621,#55622,#55623,
#55624),.UNSPECIFIED.,.F.,.F.,(4,2,4),(0.,1.,2.),.UNSPECIFIED.);
#988=B_SPLINE_CURVE_WITH_KNOTS('',3,(#55838,#55839,#55840,#55841,#55842,
#55843),.UNSPECIFIED.,.F.,.F.,(4,2,4),(0.,1.,2.),.UNSPECIFIED.);
#989=B_SPLINE_CURVE_WITH_KNOTS('',3,(#55921,#55922,#55923,#55924,#55925,
#55926),.UNSPECIFIED.,.F.,.F.,(4,2,4),(0.,1.,2.),.UNSPECIFIED.);
#990=B_SPLINE_CURVE_WITH_KNOTS('',3,(#56280,#56281,#56282,#56283,#56284,
#56285),.UNSPECIFIED.,.F.,.F.,(4,2,4),(0.,1.,2.),.UNSPECIFIED.);
#991=B_SPLINE_CURVE_WITH_KNOTS('',3,(#56363,#56364,#56365,#56366,#56367,
#56368),.UNSPECIFIED.,.F.,.F.,(4,2,4),(0.,1.,2.),.UNSPECIFIED.);
#992=B_SPLINE_CURVE_WITH_KNOTS('',3,(#56722,#56723,#56724,#56725,#56726,
#56727),.UNSPECIFIED.,.F.,.F.,(4,2,4),(0.,1.,2.),.UNSPECIFIED.);
#993=B_SPLINE_CURVE_WITH_KNOTS('',3,(#56805,#56806,#56807,#56808,#56809,
#56810),.UNSPECIFIED.,.F.,.F.,(4,2,4),(0.,1.,2.),.UNSPECIFIED.);
#994=B_SPLINE_CURVE_WITH_KNOTS('',3,(#57164,#57165,#57166,#57167,#57168,
#57169),.UNSPECIFIED.,.F.,.F.,(4,2,4),(0.,1.,2.),.UNSPECIFIED.);
#995=B_SPLINE_CURVE_WITH_KNOTS('',3,(#57247,#57248,#57249,#57250,#57251,
#57252),.UNSPECIFIED.,.F.,.F.,(4,2,4),(0.,1.,2.),.UNSPECIFIED.);
#996=B_SPLINE_CURVE_WITH_KNOTS('',3,(#57606,#57607,#57608,#57609,#57610,
#57611),.UNSPECIFIED.,.F.,.F.,(4,2,4),(0.,1.,2.),.UNSPECIFIED.);
#997=B_SPLINE_CURVE_WITH_KNOTS('',3,(#57689,#57690,#57691,#57692,#57693,
#57694),.UNSPECIFIED.,.F.,.F.,(4,2,4),(0.,1.,2.),.UNSPECIFIED.);
#998=B_SPLINE_CURVE_WITH_KNOTS('',3,(#58048,#58049,#58050,#58051,#58052,
#58053),.UNSPECIFIED.,.F.,.F.,(4,2,4),(0.,1.,2.),.UNSPECIFIED.);
#999=B_SPLINE_CURVE_WITH_KNOTS('',3,(#58131,#58132,#58133,#58134,#58135,
#58136),.UNSPECIFIED.,.F.,.F.,(4,2,4),(0.,1.,2.),.UNSPECIFIED.);
#1000=B_SPLINE_CURVE_WITH_KNOTS('',3,(#58490,#58491,#58492,#58493,#58494,
#58495),.UNSPECIFIED.,.F.,.F.,(4,2,4),(0.,1.,2.),.UNSPECIFIED.);
#1001=B_SPLINE_CURVE_WITH_KNOTS('',3,(#58573,#58574,#58575,#58576,#58577,
#58578),.UNSPECIFIED.,.F.,.F.,(4,2,4),(0.,1.,2.),.UNSPECIFIED.);
#1002=B_SPLINE_CURVE_WITH_KNOTS('',3,(#58932,#58933,#58934,#58935,#58936,
#58937),.UNSPECIFIED.,.F.,.F.,(4,2,4),(0.,1.,2.),.UNSPECIFIED.);
#1003=B_SPLINE_CURVE_WITH_KNOTS('',3,(#59015,#59016,#59017,#59018,#59019,
#59020),.UNSPECIFIED.,.F.,.F.,(4,2,4),(0.,1.,2.),.UNSPECIFIED.);
#1004=B_SPLINE_CURVE_WITH_KNOTS('',3,(#59374,#59375,#59376,#59377,#59378,
#59379),.UNSPECIFIED.,.F.,.F.,(4,2,4),(0.,1.,2.),.UNSPECIFIED.);
#1005=B_SPLINE_CURVE_WITH_KNOTS('',3,(#59457,#59458,#59459,#59460,#59461,
#59462),.UNSPECIFIED.,.F.,.F.,(4,2,4),(0.,1.,2.),.UNSPECIFIED.);
#1006=B_SPLINE_CURVE_WITH_KNOTS('',3,(#59816,#59817,#59818,#59819,#59820,
#59821),.UNSPECIFIED.,.F.,.F.,(4,2,4),(0.,1.,2.),.UNSPECIFIED.);
#1007=B_SPLINE_CURVE_WITH_KNOTS('',3,(#59899,#59900,#59901,#59902,#59903,
#59904),.UNSPECIFIED.,.F.,.F.,(4,2,4),(0.,1.,2.),.UNSPECIFIED.);
#1008=B_SPLINE_CURVE_WITH_KNOTS('',3,(#60258,#60259,#60260,#60261,#60262,
#60263),.UNSPECIFIED.,.F.,.F.,(4,2,4),(0.,1.,2.),.UNSPECIFIED.);
#1009=B_SPLINE_CURVE_WITH_KNOTS('',3,(#60341,#60342,#60343,#60344,#60345,
#60346),.UNSPECIFIED.,.F.,.F.,(4,2,4),(0.,1.,2.),.UNSPECIFIED.);
#1010=B_SPLINE_CURVE_WITH_KNOTS('',3,(#60700,#60701,#60702,#60703,#60704,
#60705),.UNSPECIFIED.,.F.,.F.,(4,2,4),(0.,1.,2.),.UNSPECIFIED.);
#1011=B_SPLINE_CURVE_WITH_KNOTS('',3,(#60783,#60784,#60785,#60786,#60787,
#60788),.UNSPECIFIED.,.F.,.F.,(4,2,4),(0.,1.,2.),.UNSPECIFIED.);
#1012=B_SPLINE_CURVE_WITH_KNOTS('',3,(#61142,#61143,#61144,#61145,#61146,
#61147),.UNSPECIFIED.,.F.,.F.,(4,2,4),(0.,1.,2.),.UNSPECIFIED.);
#1013=B_SPLINE_CURVE_WITH_KNOTS('',3,(#61225,#61226,#61227,#61228,#61229,
#61230),.UNSPECIFIED.,.F.,.F.,(4,2,4),(0.,1.,2.),.UNSPECIFIED.);
#1014=B_SPLINE_CURVE_WITH_KNOTS('',3,(#61584,#61585,#61586,#61587,#61588,
#61589),.UNSPECIFIED.,.F.,.F.,(4,2,4),(0.,1.,2.),.UNSPECIFIED.);
#1015=B_SPLINE_CURVE_WITH_KNOTS('',3,(#61667,#61668,#61669,#61670,#61671,
#61672),.UNSPECIFIED.,.F.,.F.,(4,2,4),(0.,1.,2.),.UNSPECIFIED.);
#1016=B_SPLINE_CURVE_WITH_KNOTS('',3,(#62026,#62027,#62028,#62029,#62030,
#62031),.UNSPECIFIED.,.F.,.F.,(4,2,4),(0.,1.,2.),.UNSPECIFIED.);
#1017=B_SPLINE_CURVE_WITH_KNOTS('',3,(#62109,#62110,#62111,#62112,#62113,
#62114),.UNSPECIFIED.,.F.,.F.,(4,2,4),(0.,1.,2.),.UNSPECIFIED.);
#1018=B_SPLINE_CURVE_WITH_KNOTS('',3,(#62468,#62469,#62470,#62471,#62472,
#62473),.UNSPECIFIED.,.F.,.F.,(4,2,4),(0.,1.,2.),.UNSPECIFIED.);
#1019=B_SPLINE_CURVE_WITH_KNOTS('',3,(#62551,#62552,#62553,#62554,#62555,
#62556),.UNSPECIFIED.,.F.,.F.,(4,2,4),(0.,1.,2.),.UNSPECIFIED.);
#1020=B_SPLINE_CURVE_WITH_KNOTS('',3,(#62910,#62911,#62912,#62913,#62914,
#62915),.UNSPECIFIED.,.F.,.F.,(4,2,4),(0.,1.,2.),.UNSPECIFIED.);
#1021=B_SPLINE_CURVE_WITH_KNOTS('',3,(#62993,#62994,#62995,#62996,#62997,
#62998),.UNSPECIFIED.,.F.,.F.,(4,2,4),(0.,1.,2.),.UNSPECIFIED.);
#1022=B_SPLINE_CURVE_WITH_KNOTS('',3,(#63352,#63353,#63354,#63355,#63356,
#63357),.UNSPECIFIED.,.F.,.F.,(4,2,4),(0.,1.,2.),.UNSPECIFIED.);
#1023=B_SPLINE_CURVE_WITH_KNOTS('',3,(#63435,#63436,#63437,#63438,#63439,
#63440),.UNSPECIFIED.,.F.,.F.,(4,2,4),(0.,1.,2.),.UNSPECIFIED.);
#1024=B_SPLINE_CURVE_WITH_KNOTS('',3,(#63794,#63795,#63796,#63797,#63798,
#63799),.UNSPECIFIED.,.F.,.F.,(4,2,4),(0.,1.,2.),.UNSPECIFIED.);
#1025=B_SPLINE_CURVE_WITH_KNOTS('',3,(#63877,#63878,#63879,#63880,#63881,
#63882),.UNSPECIFIED.,.F.,.F.,(4,2,4),(0.,1.,2.),.UNSPECIFIED.);
#1026=B_SPLINE_CURVE_WITH_KNOTS('',3,(#64236,#64237,#64238,#64239,#64240,
#64241),.UNSPECIFIED.,.F.,.F.,(4,2,4),(0.,1.,2.),.UNSPECIFIED.);
#1027=B_SPLINE_CURVE_WITH_KNOTS('',3,(#64319,#64320,#64321,#64322,#64323,
#64324),.UNSPECIFIED.,.F.,.F.,(4,2,4),(0.,1.,2.),.UNSPECIFIED.);
#1028=B_SPLINE_CURVE_WITH_KNOTS('',3,(#64678,#64679,#64680,#64681,#64682,
#64683),.UNSPECIFIED.,.F.,.F.,(4,2,4),(0.,1.,2.),.UNSPECIFIED.);
#1029=B_SPLINE_CURVE_WITH_KNOTS('',3,(#64761,#64762,#64763,#64764,#64765,
#64766),.UNSPECIFIED.,.F.,.F.,(4,2,4),(0.,1.,2.),.UNSPECIFIED.);
#1030=B_SPLINE_CURVE_WITH_KNOTS('',3,(#65120,#65121,#65122,#65123,#65124,
#65125),.UNSPECIFIED.,.F.,.F.,(4,2,4),(0.,1.,2.),.UNSPECIFIED.);
#1031=B_SPLINE_CURVE_WITH_KNOTS('',3,(#65203,#65204,#65205,#65206,#65207,
#65208),.UNSPECIFIED.,.F.,.F.,(4,2,4),(0.,1.,2.),.UNSPECIFIED.);
#1032=B_SPLINE_CURVE_WITH_KNOTS('',3,(#65562,#65563,#65564,#65565,#65566,
#65567),.UNSPECIFIED.,.F.,.F.,(4,2,4),(0.,1.,2.),.UNSPECIFIED.);
#1033=B_SPLINE_CURVE_WITH_KNOTS('',3,(#65645,#65646,#65647,#65648,#65649,
#65650),.UNSPECIFIED.,.F.,.F.,(4,2,4),(0.,1.,2.),.UNSPECIFIED.);
#1034=B_SPLINE_CURVE_WITH_KNOTS('',3,(#66004,#66005,#66006,#66007,#66008,
#66009),.UNSPECIFIED.,.F.,.F.,(4,2,4),(0.,1.,2.),.UNSPECIFIED.);
#1035=B_SPLINE_CURVE_WITH_KNOTS('',3,(#66087,#66088,#66089,#66090,#66091,
#66092),.UNSPECIFIED.,.F.,.F.,(4,2,4),(0.,1.,2.),.UNSPECIFIED.);
#1036=B_SPLINE_CURVE_WITH_KNOTS('',3,(#66446,#66447,#66448,#66449,#66450,
#66451),.UNSPECIFIED.,.F.,.F.,(4,2,4),(0.,1.,2.),.UNSPECIFIED.);
#1037=B_SPLINE_CURVE_WITH_KNOTS('',3,(#66529,#66530,#66531,#66532,#66533,
#66534),.UNSPECIFIED.,.F.,.F.,(4,2,4),(0.,1.,2.),.UNSPECIFIED.);
#1038=B_SPLINE_CURVE_WITH_KNOTS('',3,(#66888,#66889,#66890,#66891,#66892,
#66893),.UNSPECIFIED.,.F.,.F.,(4,2,4),(0.,1.,2.),.UNSPECIFIED.);
#1039=B_SPLINE_CURVE_WITH_KNOTS('',3,(#66971,#66972,#66973,#66974,#66975,
#66976),.UNSPECIFIED.,.F.,.F.,(4,2,4),(0.,1.,2.),.UNSPECIFIED.);
#1040=B_SPLINE_CURVE_WITH_KNOTS('',3,(#67330,#67331,#67332,#67333,#67334,
#67335),.UNSPECIFIED.,.F.,.F.,(4,2,4),(0.,1.,2.),.UNSPECIFIED.);
#1041=B_SPLINE_CURVE_WITH_KNOTS('',3,(#67413,#67414,#67415,#67416,#67417,
#67418),.UNSPECIFIED.,.F.,.F.,(4,2,4),(0.,1.,2.),.UNSPECIFIED.);
#1042=B_SPLINE_CURVE_WITH_KNOTS('',3,(#67772,#67773,#67774,#67775,#67776,
#67777),.UNSPECIFIED.,.F.,.F.,(4,2,4),(0.,1.,2.),.UNSPECIFIED.);
#1043=B_SPLINE_CURVE_WITH_KNOTS('',3,(#67855,#67856,#67857,#67858,#67859,
#67860),.UNSPECIFIED.,.F.,.F.,(4,2,4),(0.,1.,2.),.UNSPECIFIED.);
#1044=B_SPLINE_CURVE_WITH_KNOTS('',3,(#68214,#68215,#68216,#68217,#68218,
#68219),.UNSPECIFIED.,.F.,.F.,(4,2,4),(0.,1.,2.),.UNSPECIFIED.);
#1045=B_SPLINE_CURVE_WITH_KNOTS('',3,(#68297,#68298,#68299,#68300,#68301,
#68302),.UNSPECIFIED.,.F.,.F.,(4,2,4),(0.,1.,2.),.UNSPECIFIED.);
#1046=B_SPLINE_CURVE_WITH_KNOTS('',3,(#68656,#68657,#68658,#68659,#68660,
#68661),.UNSPECIFIED.,.F.,.F.,(4,2,4),(0.,1.,2.),.UNSPECIFIED.);
#1047=B_SPLINE_CURVE_WITH_KNOTS('',3,(#68739,#68740,#68741,#68742,#68743,
#68744),.UNSPECIFIED.,.F.,.F.,(4,2,4),(0.,1.,2.),.UNSPECIFIED.);
#1048=B_SPLINE_CURVE_WITH_KNOTS('',3,(#69098,#69099,#69100,#69101,#69102,
#69103),.UNSPECIFIED.,.F.,.F.,(4,2,4),(0.,1.,2.),.UNSPECIFIED.);
#1049=B_SPLINE_CURVE_WITH_KNOTS('',3,(#69181,#69182,#69183,#69184,#69185,
#69186),.UNSPECIFIED.,.F.,.F.,(4,2,4),(0.,1.,2.),.UNSPECIFIED.);
#1050=B_SPLINE_CURVE_WITH_KNOTS('',3,(#69540,#69541,#69542,#69543,#69544,
#69545),.UNSPECIFIED.,.F.,.F.,(4,2,4),(0.,1.,2.),.UNSPECIFIED.);
#1051=B_SPLINE_CURVE_WITH_KNOTS('',3,(#69623,#69624,#69625,#69626,#69627,
#69628),.UNSPECIFIED.,.F.,.F.,(4,2,4),(0.,1.,2.),.UNSPECIFIED.);
#1052=B_SPLINE_CURVE_WITH_KNOTS('',3,(#69982,#69983,#69984,#69985,#69986,
#69987),.UNSPECIFIED.,.F.,.F.,(4,2,4),(0.,1.,2.),.UNSPECIFIED.);
#1053=B_SPLINE_CURVE_WITH_KNOTS('',3,(#70065,#70066,#70067,#70068,#70069,
#70070),.UNSPECIFIED.,.F.,.F.,(4,2,4),(0.,1.,2.),.UNSPECIFIED.);
#1054=B_SPLINE_CURVE_WITH_KNOTS('',3,(#70424,#70425,#70426,#70427,#70428,
#70429),.UNSPECIFIED.,.F.,.F.,(4,2,4),(0.,1.,2.),.UNSPECIFIED.);
#1055=B_SPLINE_CURVE_WITH_KNOTS('',3,(#70507,#70508,#70509,#70510,#70511,
#70512),.UNSPECIFIED.,.F.,.F.,(4,2,4),(0.,1.,2.),.UNSPECIFIED.);
#1056=B_SPLINE_CURVE_WITH_KNOTS('',3,(#70866,#70867,#70868,#70869,#70870,
#70871),.UNSPECIFIED.,.F.,.F.,(4,2,4),(0.,1.,2.),.UNSPECIFIED.);
#1057=B_SPLINE_CURVE_WITH_KNOTS('',3,(#70949,#70950,#70951,#70952,#70953,
#70954),.UNSPECIFIED.,.F.,.F.,(4,2,4),(0.,1.,2.),.UNSPECIFIED.);
#1058=B_SPLINE_CURVE_WITH_KNOTS('',3,(#71308,#71309,#71310,#71311,#71312,
#71313),.UNSPECIFIED.,.F.,.F.,(4,2,4),(0.,1.,2.),.UNSPECIFIED.);
#1059=B_SPLINE_CURVE_WITH_KNOTS('',3,(#71391,#71392,#71393,#71394,#71395,
#71396),.UNSPECIFIED.,.F.,.F.,(4,2,4),(0.,1.,2.),.UNSPECIFIED.);
#1060=B_SPLINE_CURVE_WITH_KNOTS('',3,(#71750,#71751,#71752,#71753,#71754,
#71755),.UNSPECIFIED.,.F.,.F.,(4,2,4),(0.,1.,2.),.UNSPECIFIED.);
#1061=B_SPLINE_CURVE_WITH_KNOTS('',3,(#71833,#71834,#71835,#71836,#71837,
#71838),.UNSPECIFIED.,.F.,.F.,(4,2,4),(0.,1.,2.),.UNSPECIFIED.);
#1062=B_SPLINE_CURVE_WITH_KNOTS('',3,(#72192,#72193,#72194,#72195,#72196,
#72197),.UNSPECIFIED.,.F.,.F.,(4,2,4),(0.,1.,2.),.UNSPECIFIED.);
#1063=B_SPLINE_CURVE_WITH_KNOTS('',3,(#72275,#72276,#72277,#72278,#72279,
#72280),.UNSPECIFIED.,.F.,.F.,(4,2,4),(0.,1.,2.),.UNSPECIFIED.);
#1064=B_SPLINE_CURVE_WITH_KNOTS('',3,(#72638,#72639,#72640,#72641,#72642,
#72643),.UNSPECIFIED.,.F.,.F.,(4,2,4),(0.,1.,2.),.UNSPECIFIED.);
#1065=B_SPLINE_CURVE_WITH_KNOTS('',3,(#72717,#72718,#72719,#72720,#72721,
#72722),.UNSPECIFIED.,.F.,.F.,(4,2,4),(0.,1.,2.),.UNSPECIFIED.);
#1066=B_SPLINE_CURVE_WITH_KNOTS('',3,(#72864,#72865,#72866,#72867,#72868,
#72869),.UNSPECIFIED.,.F.,.F.,(4,2,4),(0.,1.,2.),.UNSPECIFIED.);
#1176=SHAPE_REPRESENTATION_RELATIONSHIP('SRR','None',#73668,#1232);
#1232=ADVANCED_BREP_SHAPE_REPRESENTATION('',(#1372),#73364);
#1303=STYLED_ITEM('',(#73981),#1372);
#1372=MANIFOLD_SOLID_BREP('Body1',#16193);
#1599=FACE_BOUND('',#3879,.T.);
#1600=FACE_BOUND('',#3883,.T.);
#1601=FACE_BOUND('',#4044,.T.);
#1946=PLANE('',#18246);
#1947=PLANE('',#18247);
#1948=PLANE('',#18248);
#1949=PLANE('',#18249);
#1950=PLANE('',#18296);
#1951=PLANE('',#18297);
#1952=PLANE('',#18300);
#1953=PLANE('',#18303);
#1954=PLANE('',#18306);
#1955=PLANE('',#18309);
#1956=PLANE('',#18312);
#1957=PLANE('',#18315);
#1958=PLANE('',#18318);
#1959=PLANE('',#18321);
#1960=PLANE('',#18324);
#1961=PLANE('',#18327);
#1962=PLANE('',#18330);
#1963=PLANE('',#18333);
#1964=PLANE('',#18336);
#1965=PLANE('',#18339);
#1966=PLANE('',#18342);
#1967=PLANE('',#18345);
#1968=PLANE('',#18348);
#1969=PLANE('',#18351);
#1970=PLANE('',#18354);
#1971=PLANE('',#18357);
#1972=PLANE('',#18360);
#1973=PLANE('',#18363);
#1974=PLANE('',#18366);
#1975=PLANE('',#18369);
#1976=PLANE('',#18372);
#1977=PLANE('',#18375);
#1978=PLANE('',#18378);
#1979=PLANE('',#18381);
#1980=PLANE('',#18384);
#1981=PLANE('',#18387);
#1982=PLANE('',#18390);
#1983=PLANE('',#18393);
#1984=PLANE('',#18396);
#1985=PLANE('',#18399);
#1986=PLANE('',#18402);
#1987=PLANE('',#18405);
#1988=PLANE('',#18408);
#1989=PLANE('',#18411);
#1990=PLANE('',#18414);
#1991=PLANE('',#18415);
#2737=FACE_OUTER_BOUND('',#3875,.T.);
#2738=FACE_OUTER_BOUND('',#3876,.T.);
#2739=FACE_OUTER_BOUND('',#3877,.T.);
#2740=FACE_OUTER_BOUND('',#3878,.T.);
#2741=FACE_OUTER_BOUND('',#3880,.T.);
#2742=FACE_OUTER_BOUND('',#3881,.T.);
#2743=FACE_OUTER_BOUND('',#3882,.T.);
#2744=FACE_OUTER_BOUND('',#3884,.T.);
#2745=FACE_OUTER_BOUND('',#3885,.T.);
#2746=FACE_OUTER_BOUND('',#3886,.T.);
#2747=FACE_OUTER_BOUND('',#3887,.T.);
#2748=FACE_OUTER_BOUND('',#3888,.T.);
#2749=FACE_OUTER_BOUND('',#3889,.T.);
#2750=FACE_OUTER_BOUND('',#3890,.T.);
#2751=FACE_OUTER_BOUND('',#3891,.T.);
#2752=FACE_OUTER_BOUND('',#3892,.T.);
#2753=FACE_OUTER_BOUND('',#3893,.T.);
#2754=FACE_OUTER_BOUND('',#3894,.T.);
#2755=FACE_OUTER_BOUND('',#3895,.T.);
#2756=FACE_OUTER_BOUND('',#3896,.T.);
#2757=FACE_OUTER_BOUND('',#3897,.T.);
#2758=FACE_OUTER_BOUND('',#3898,.T.);
#2759=FACE_OUTER_BOUND('',#3899,.T.);
#2760=FACE_OUTER_BOUND('',#3900,.T.);
#2761=FACE_OUTER_BOUND('',#3901,.T.);
#2762=FACE_OUTER_BOUND('',#3902,.T.);
#2763=FACE_OUTER_BOUND('',#3903,.T.);
#2764=FACE_OUTER_BOUND('',#3904,.T.);
#2765=FACE_OUTER_BOUND('',#3905,.T.);
#2766=FACE_OUTER_BOUND('',#3906,.T.);
#2767=FACE_OUTER_BOUND('',#3907,.T.);
#2768=FACE_OUTER_BOUND('',#3908,.T.);
#2769=FACE_OUTER_BOUND('',#3909,.T.);
#2770=FACE_OUTER_BOUND('',#3910,.T.);
#2771=FACE_OUTER_BOUND('',#3911,.T.);
#2772=FACE_OUTER_BOUND('',#3912,.T.);
#2773=FACE_OUTER_BOUND('',#3913,.T.);
#2774=FACE_OUTER_BOUND('',#3914,.T.);
#2775=FACE_OUTER_BOUND('',#3915,.T.);
#2776=FACE_OUTER_BOUND('',#3916,.T.);
#2777=FACE_OUTER_BOUND('',#3917,.T.);
#2778=FACE_OUTER_BOUND('',#3918,.T.);
#2779=FACE_OUTER_BOUND('',#3919,.T.);
#2780=FACE_OUTER_BOUND('',#3920,.T.);
#2781=FACE_OUTER_BOUND('',#3921,.T.);
#2782=FACE_OUTER_BOUND('',#3922,.T.);
#2783=FACE_OUTER_BOUND('',#3923,.T.);
#2784=FACE_OUTER_BOUND('',#3924,.T.);
#2785=FACE_OUTER_BOUND('',#3925,.T.);
#2786=FACE_OUTER_BOUND('',#3926,.T.);
#2787=FACE_OUTER_BOUND('',#3927,.T.);
#2788=FACE_OUTER_BOUND('',#3928,.T.);
#2789=FACE_OUTER_BOUND('',#3929,.T.);
#2790=FACE_OUTER_BOUND('',#3930,.T.);
#2791=FACE_OUTER_BOUND('',#3931,.T.);
#2792=FACE_OUTER_BOUND('',#3932,.T.);
#2793=FACE_OUTER_BOUND('',#3933,.T.);
#2794=FACE_OUTER_BOUND('',#3934,.T.);
#2795=FACE_OUTER_BOUND('',#3935,.T.);
#2796=FACE_OUTER_BOUND('',#3936,.T.);
#2797=FACE_OUTER_BOUND('',#3937,.T.);
#2798=FACE_OUTER_BOUND('',#3938,.T.);
#2799=FACE_OUTER_BOUND('',#3939,.T.);
#2800=FACE_OUTER_BOUND('',#3940,.T.);
#2801=FACE_OUTER_BOUND('',#3941,.T.);
#2802=FACE_OUTER_BOUND('',#3942,.T.);
#2803=FACE_OUTER_BOUND('',#3943,.T.);
#2804=FACE_OUTER_BOUND('',#3944,.T.);
#2805=FACE_OUTER_BOUND('',#3945,.T.);
#2806=FACE_OUTER_BOUND('',#3946,.T.);
#2807=FACE_OUTER_BOUND('',#3947,.T.);
#2808=FACE_OUTER_BOUND('',#3948,.T.);
#2809=FACE_OUTER_BOUND('',#3949,.T.);
#2810=FACE_OUTER_BOUND('',#3950,.T.);
#2811=FACE_OUTER_BOUND('',#3951,.T.);
#2812=FACE_OUTER_BOUND('',#3952,.T.);
#2813=FACE_OUTER_BOUND('',#3953,.T.);
#2814=FACE_OUTER_BOUND('',#3954,.T.);
#2815=FACE_OUTER_BOUND('',#3955,.T.);
#2816=FACE_OUTER_BOUND('',#3956,.T.);
#2817=FACE_OUTER_BOUND('',#3957,.T.);
#2818=FACE_OUTER_BOUND('',#3958,.T.);
#2819=FACE_OUTER_BOUND('',#3959,.T.);
#2820=FACE_OUTER_BOUND('',#3960,.T.);
#2821=FACE_OUTER_BOUND('',#3961,.T.);
#2822=FACE_OUTER_BOUND('',#3962,.T.);
#2823=FACE_OUTER_BOUND('',#3963,.T.);
#2824=FACE_OUTER_BOUND('',#3964,.T.);
#2825=FACE_OUTER_BOUND('',#3965,.T.);
#2826=FACE_OUTER_BOUND('',#3966,.T.);
#2827=FACE_OUTER_BOUND('',#3967,.T.);
#2828=FACE_OUTER_BOUND('',#3968,.T.);
#2829=FACE_OUTER_BOUND('',#3969,.T.);
#2830=FACE_OUTER_BOUND('',#3970,.T.);
#2831=FACE_OUTER_BOUND('',#3971,.T.);
#2832=FACE_OUTER_BOUND('',#3972,.T.);
#2833=FACE_OUTER_BOUND('',#3973,.T.);
#2834=FACE_OUTER_BOUND('',#3974,.T.);
#2835=FACE_OUTER_BOUND('',#3975,.T.);
#2836=FACE_OUTER_BOUND('',#3976,.T.);
#2837=FACE_OUTER_BOUND('',#3977,.T.);
#2838=FACE_OUTER_BOUND('',#3978,.T.);
#2839=FACE_OUTER_BOUND('',#3979,.T.);
#2840=FACE_OUTER_BOUND('',#3980,.T.);
#2841=FACE_OUTER_BOUND('',#3981,.T.);
#2842=FACE_OUTER_BOUND('',#3982,.T.);
#2843=FACE_OUTER_BOUND('',#3983,.T.);
#2844=FACE_OUTER_BOUND('',#3984,.T.);
#2845=FACE_OUTER_BOUND('',#3985,.T.);
#2846=FACE_OUTER_BOUND('',#3986,.T.);
#2847=FACE_OUTER_BOUND('',#3987,.T.);
#2848=FACE_OUTER_BOUND('',#3988,.T.);
#2849=FACE_OUTER_BOUND('',#3989,.T.);
#2850=FACE_OUTER_BOUND('',#3990,.T.);
#2851=FACE_OUTER_BOUND('',#3991,.T.);
#2852=FACE_OUTER_BOUND('',#3992,.T.);
#2853=FACE_OUTER_BOUND('',#3993,.T.);
#2854=FACE_OUTER_BOUND('',#3994,.T.);
#2855=FACE_OUTER_BOUND('',#3995,.T.);
#2856=FACE_OUTER_BOUND('',#3996,.T.);
#2857=FACE_OUTER_BOUND('',#3997,.T.);
#2858=FACE_OUTER_BOUND('',#3998,.T.);
#2859=FACE_OUTER_BOUND('',#3999,.T.);
#2860=FACE_OUTER_BOUND('',#4000,.T.);
#2861=FACE_OUTER_BOUND('',#4001,.T.);
#2862=FACE_OUTER_BOUND('',#4002,.T.);
#2863=FACE_OUTER_BOUND('',#4003,.T.);
#2864=FACE_OUTER_BOUND('',#4004,.T.);
#2865=FACE_OUTER_BOUND('',#4005,.T.);
#2866=FACE_OUTER_BOUND('',#4006,.T.);
#2867=FACE_OUTER_BOUND('',#4007,.T.);
#2868=FACE_OUTER_BOUND('',#4008,.T.);
#2869=FACE_OUTER_BOUND('',#4009,.T.);
#2870=FACE_OUTER_BOUND('',#4010,.T.);
#2871=FACE_OUTER_BOUND('',#4011,.T.);
#2872=FACE_OUTER_BOUND('',#4012,.T.);
#2873=FACE_OUTER_BOUND('',#4013,.T.);
#2874=FACE_OUTER_BOUND('',#4014,.T.);
#2875=FACE_OUTER_BOUND('',#4015,.T.);
#2876=FACE_OUTER_BOUND('',#4016,.T.);
#2877=FACE_OUTER_BOUND('',#4017,.T.);
#2878=FACE_OUTER_BOUND('',#4018,.T.);
#2879=FACE_OUTER_BOUND('',#4019,.T.);
#2880=FACE_OUTER_BOUND('',#4020,.T.);
#2881=FACE_OUTER_BOUND('',#4021,.T.);
#2882=FACE_OUTER_BOUND('',#4022,.T.);
#2883=FACE_OUTER_BOUND('',#4023,.T.);
#2884=FACE_OUTER_BOUND('',#4024,.T.);
#2885=FACE_OUTER_BOUND('',#4025,.T.);
#2886=FACE_OUTER_BOUND('',#4026,.T.);
#2887=FACE_OUTER_BOUND('',#4027,.T.);
#2888=FACE_OUTER_BOUND('',#4028,.T.);
#2889=FACE_OUTER_BOUND('',#4029,.T.);
#2890=FACE_OUTER_BOUND('',#4030,.T.);
#2891=FACE_OUTER_BOUND('',#4031,.T.);
#2892=FACE_OUTER_BOUND('',#4032,.T.);
#2893=FACE_OUTER_BOUND('',#4033,.T.);
#2894=FACE_OUTER_BOUND('',#4034,.T.);
#2895=FACE_OUTER_BOUND('',#4035,.T.);
#2896=FACE_OUTER_BOUND('',#4036,.T.);
#2897=FACE_OUTER_BOUND('',#4037,.T.);
#2898=FACE_OUTER_BOUND('',#4038,.T.);
#2899=FACE_OUTER_BOUND('',#4039,.T.);
#2900=FACE_OUTER_BOUND('',#4040,.T.);
#2901=FACE_OUTER_BOUND('',#4041,.T.);
#2902=FACE_OUTER_BOUND('',#4042,.T.);
#2903=FACE_OUTER_BOUND('',#4043,.T.);
#2904=FACE_OUTER_BOUND('',#4045,.T.);
#3875=EDGE_LOOP('',(#13869,#13870,#13871,#13872));
#3876=EDGE_LOOP('',(#13873,#13874,#13875,#13876));
#3877=EDGE_LOOP('',(#13877,#13878,#13879,#13880));
#3878=EDGE_LOOP('',(#13881,#13882,#13883,#13884,#13885,#13886,#13887,#13888,
#13889,#13890,#13891,#13892,#13893,#13894,#13895,#13896,#13897,#13898,#13899,
#13900,#13901,#13902,#13903,#13904,#13905,#13906,#13907,#13908,#13909,#13910,
#13911,#13912,#13913,#13914,#13915,#13916,#13917,#13918,#13919,#13920,#13921,
#13922,#13923,#13924,#13925,#13926,#13927,#13928,#13929,#13930,#13931,#13932,
#13933,#13934,#13935,#13936,#13937,#13938,#13939,#13940,#13941,#13942,#13943,
#13944,#13945,#13946,#13947,#13948,#13949,#13950,#13951,#13952,#13953,#13954,
#13955,#13956,#13957,#13958,#13959,#13960,#13961,#13962,#13963,#13964,#13965,
#13966,#13967,#13968,#13969,#13970,#13971,#13972,#13973,#13974,#13975,#13976,
#13977,#13978,#13979,#13980,#13981,#13982,#13983,#13984,#13985,#13986,#13987,
#13988,#13989,#13990,#13991,#13992,#13993,#13994,#13995,#13996,#13997,#13998,
#13999,#14000,#14001,#14002,#14003,#14004,#14005,#14006,#14007,#14008,#14009,
#14010,#14011,#14012,#14013,#14014,#14015,#14016,#14017,#14018,#14019,#14020,
#14021,#14022,#14023,#14024,#14025,#14026,#14027,#14028,#14029,#14030,#14031,
#14032,#14033,#14034,#14035,#14036,#14037,#14038,#14039,#14040));
#3879=EDGE_LOOP('',(#14041,#14042,#14043,#14044));
#3880=EDGE_LOOP('',(#14045,#14046,#14047,#14048));
#3881=EDGE_LOOP('',(#14049,#14050,#14051,#14052));
#3882=EDGE_LOOP('',(#14053));
#3883=EDGE_LOOP('',(#14054,#14055,#14056,#14057));
#3884=EDGE_LOOP('',(#14058,#14059,#14060,#14061));
#3885=EDGE_LOOP('',(#14062,#14063,#14064,#14065));
#3886=EDGE_LOOP('',(#14066,#14067,#14068,#14069));
#3887=EDGE_LOOP('',(#14070,#14071,#14072,#14073));
#3888=EDGE_LOOP('',(#14074,#14075,#14076,#14077));
#3889=EDGE_LOOP('',(#14078,#14079,#14080,#14081));
#3890=EDGE_LOOP('',(#14082,#14083,#14084,#14085));
#3891=EDGE_LOOP('',(#14086,#14087,#14088,#14089));
#3892=EDGE_LOOP('',(#14090,#14091,#14092,#14093));
#3893=EDGE_LOOP('',(#14094,#14095,#14096,#14097));
#3894=EDGE_LOOP('',(#14098,#14099,#14100,#14101));
#3895=EDGE_LOOP('',(#14102,#14103,#14104,#14105));
#3896=EDGE_LOOP('',(#14106,#14107,#14108,#14109));
#3897=EDGE_LOOP('',(#14110,#14111,#14112,#14113));
#3898=EDGE_LOOP('',(#14114,#14115,#14116,#14117));
#3899=EDGE_LOOP('',(#14118,#14119,#14120,#14121));
#3900=EDGE_LOOP('',(#14122,#14123,#14124,#14125));
#3901=EDGE_LOOP('',(#14126,#14127,#14128,#14129));
#3902=EDGE_LOOP('',(#14130,#14131,#14132,#14133));
#3903=EDGE_LOOP('',(#14134,#14135,#14136,#14137));
#3904=EDGE_LOOP('',(#14138,#14139,#14140,#14141));
#3905=EDGE_LOOP('',(#14142,#14143,#14144,#14145));
#3906=EDGE_LOOP('',(#14146,#14147,#14148,#14149));
#3907=EDGE_LOOP('',(#14150,#14151,#14152,#14153));
#3908=EDGE_LOOP('',(#14154,#14155,#14156,#14157));
#3909=EDGE_LOOP('',(#14158,#14159,#14160,#14161));
#3910=EDGE_LOOP('',(#14162,#14163,#14164,#14165));
#3911=EDGE_LOOP('',(#14166,#14167,#14168,#14169));
#3912=EDGE_LOOP('',(#14170,#14171,#14172,#14173));
#3913=EDGE_LOOP('',(#14174,#14175,#14176,#14177));
#3914=EDGE_LOOP('',(#14178,#14179,#14180,#14181));
#3915=EDGE_LOOP('',(#14182,#14183,#14184,#14185));
#3916=EDGE_LOOP('',(#14186,#14187,#14188,#14189));
#3917=EDGE_LOOP('',(#14190,#14191,#14192,#14193));
#3918=EDGE_LOOP('',(#14194,#14195,#14196,#14197));
#3919=EDGE_LOOP('',(#14198,#14199,#14200,#14201));
#3920=EDGE_LOOP('',(#14202,#14203,#14204,#14205));
#3921=EDGE_LOOP('',(#14206,#14207,#14208,#14209));
#3922=EDGE_LOOP('',(#14210,#14211,#14212,#14213));
#3923=EDGE_LOOP('',(#14214,#14215,#14216,#14217));
#3924=EDGE_LOOP('',(#14218,#14219,#14220,#14221));
#3925=EDGE_LOOP('',(#14222,#14223,#14224,#14225));
#3926=EDGE_LOOP('',(#14226,#14227,#14228,#14229));
#3927=EDGE_LOOP('',(#14230,#14231,#14232,#14233));
#3928=EDGE_LOOP('',(#14234,#14235,#14236,#14237));
#3929=EDGE_LOOP('',(#14238,#14239,#14240,#14241));
#3930=EDGE_LOOP('',(#14242,#14243,#14244,#14245));
#3931=EDGE_LOOP('',(#14246,#14247,#14248,#14249));
#3932=EDGE_LOOP('',(#14250,#14251,#14252,#14253));
#3933=EDGE_LOOP('',(#14254,#14255,#14256,#14257));
#3934=EDGE_LOOP('',(#14258,#14259,#14260,#14261));
#3935=EDGE_LOOP('',(#14262,#14263,#14264,#14265));
#3936=EDGE_LOOP('',(#14266,#14267,#14268,#14269));
#3937=EDGE_LOOP('',(#14270,#14271,#14272,#14273));
#3938=EDGE_LOOP('',(#14274,#14275,#14276,#14277));
#3939=EDGE_LOOP('',(#14278,#14279,#14280,#14281));
#3940=EDGE_LOOP('',(#14282,#14283,#14284,#14285));
#3941=EDGE_LOOP('',(#14286,#14287,#14288,#14289));
#3942=EDGE_LOOP('',(#14290,#14291,#14292,#14293));
#3943=EDGE_LOOP('',(#14294,#14295,#14296,#14297));
#3944=EDGE_LOOP('',(#14298,#14299,#14300,#14301));
#3945=EDGE_LOOP('',(#14302,#14303,#14304,#14305));
#3946=EDGE_LOOP('',(#14306,#14307,#14308,#14309));
#3947=EDGE_LOOP('',(#14310,#14311,#14312,#14313));
#3948=EDGE_LOOP('',(#14314,#14315,#14316,#14317));
#3949=EDGE_LOOP('',(#14318,#14319,#14320,#14321));
#3950=EDGE_LOOP('',(#14322,#14323,#14324,#14325));
#3951=EDGE_LOOP('',(#14326,#14327,#14328,#14329));
#3952=EDGE_LOOP('',(#14330,#14331,#14332,#14333));
#3953=EDGE_LOOP('',(#14334,#14335,#14336,#14337));
#3954=EDGE_LOOP('',(#14338,#14339,#14340,#14341));
#3955=EDGE_LOOP('',(#14342,#14343,#14344,#14345));
#3956=EDGE_LOOP('',(#14346,#14347,#14348,#14349));
#3957=EDGE_LOOP('',(#14350,#14351,#14352,#14353));
#3958=EDGE_LOOP('',(#14354,#14355,#14356,#14357));
#3959=EDGE_LOOP('',(#14358,#14359,#14360,#14361));
#3960=EDGE_LOOP('',(#14362,#14363,#14364,#14365));
#3961=EDGE_LOOP('',(#14366,#14367,#14368,#14369));
#3962=EDGE_LOOP('',(#14370,#14371,#14372,#14373));
#3963=EDGE_LOOP('',(#14374,#14375,#14376,#14377));
#3964=EDGE_LOOP('',(#14378,#14379,#14380,#14381));
#3965=EDGE_LOOP('',(#14382,#14383,#14384,#14385));
#3966=EDGE_LOOP('',(#14386,#14387,#14388,#14389));
#3967=EDGE_LOOP('',(#14390,#14391,#14392,#14393));
#3968=EDGE_LOOP('',(#14394,#14395,#14396,#14397));
#3969=EDGE_LOOP('',(#14398,#14399,#14400,#14401));
#3970=EDGE_LOOP('',(#14402,#14403,#14404,#14405));
#3971=EDGE_LOOP('',(#14406,#14407,#14408,#14409));
#3972=EDGE_LOOP('',(#14410,#14411,#14412,#14413));
#3973=EDGE_LOOP('',(#14414,#14415,#14416,#14417));
#3974=EDGE_LOOP('',(#14418,#14419,#14420,#14421));
#3975=EDGE_LOOP('',(#14422,#14423,#14424,#14425));
#3976=EDGE_LOOP('',(#14426,#14427,#14428,#14429));
#3977=EDGE_LOOP('',(#14430,#14431,#14432,#14433));
#3978=EDGE_LOOP('',(#14434,#14435,#14436,#14437));
#3979=EDGE_LOOP('',(#14438,#14439,#14440,#14441));
#3980=EDGE_LOOP('',(#14442,#14443,#14444,#14445));
#3981=EDGE_LOOP('',(#14446,#14447,#14448,#14449));
#3982=EDGE_LOOP('',(#14450,#14451,#14452,#14453));
#3983=EDGE_LOOP('',(#14454,#14455,#14456,#14457));
#3984=EDGE_LOOP('',(#14458,#14459,#14460,#14461));
#3985=EDGE_LOOP('',(#14462,#14463,#14464,#14465));
#3986=EDGE_LOOP('',(#14466,#14467,#14468,#14469));
#3987=EDGE_LOOP('',(#14470,#14471,#14472,#14473));
#3988=EDGE_LOOP('',(#14474,#14475,#14476,#14477));
#3989=EDGE_LOOP('',(#14478,#14479,#14480,#14481));
#3990=EDGE_LOOP('',(#14482,#14483,#14484,#14485));
#3991=EDGE_LOOP('',(#14486,#14487,#14488,#14489));
#3992=EDGE_LOOP('',(#14490,#14491,#14492,#14493));
#3993=EDGE_LOOP('',(#14494,#14495,#14496,#14497));
#3994=EDGE_LOOP('',(#14498,#14499,#14500,#14501));
#3995=EDGE_LOOP('',(#14502,#14503,#14504,#14505));
#3996=EDGE_LOOP('',(#14506,#14507,#14508,#14509));
#3997=EDGE_LOOP('',(#14510,#14511,#14512,#14513));
#3998=EDGE_LOOP('',(#14514,#14515,#14516,#14517));
#3999=EDGE_LOOP('',(#14518,#14519,#14520,#14521));
#4000=EDGE_LOOP('',(#14522,#14523,#14524,#14525));
#4001=EDGE_LOOP('',(#14526,#14527,#14528,#14529));
#4002=EDGE_LOOP('',(#14530,#14531,#14532,#14533));
#4003=EDGE_LOOP('',(#14534,#14535,#14536,#14537));
#4004=EDGE_LOOP('',(#14538,#14539,#14540,#14541));
#4005=EDGE_LOOP('',(#14542,#14543,#14544,#14545));
#4006=EDGE_LOOP('',(#14546,#14547,#14548,#14549));
#4007=EDGE_LOOP('',(#14550,#14551,#14552,#14553));
#4008=EDGE_LOOP('',(#14554,#14555,#14556,#14557));
#4009=EDGE_LOOP('',(#14558,#14559,#14560,#14561));
#4010=EDGE_LOOP('',(#14562,#14563,#14564,#14565));
#4011=EDGE_LOOP('',(#14566,#14567,#14568,#14569));
#4012=EDGE_LOOP('',(#14570,#14571,#14572,#14573));
#4013=EDGE_LOOP('',(#14574,#14575,#14576,#14577));
#4014=EDGE_LOOP('',(#14578,#14579,#14580,#14581));
#4015=EDGE_LOOP('',(#14582,#14583,#14584,#14585));
#4016=EDGE_LOOP('',(#14586,#14587,#14588,#14589));
#4017=EDGE_LOOP('',(#14590,#14591,#14592,#14593));
#4018=EDGE_LOOP('',(#14594,#14595,#14596,#14597));
#4019=EDGE_LOOP('',(#14598,#14599,#14600,#14601));
#4020=EDGE_LOOP('',(#14602,#14603,#14604,#14605));
#4021=EDGE_LOOP('',(#14606,#14607,#14608,#14609));
#4022=EDGE_LOOP('',(#14610,#14611,#14612,#14613));
#4023=EDGE_LOOP('',(#14614,#14615,#14616,#14617));
#4024=EDGE_LOOP('',(#14618,#14619,#14620,#14621));
#4025=EDGE_LOOP('',(#14622,#14623,#14624,#14625));
#4026=EDGE_LOOP('',(#14626,#14627,#14628,#14629));
#4027=EDGE_LOOP('',(#14630,#14631,#14632,#14633));
#4028=EDGE_LOOP('',(#14634,#14635,#14636,#14637));
#4029=EDGE_LOOP('',(#14638,#14639,#14640,#14641));
#4030=EDGE_LOOP('',(#14642,#14643,#14644,#14645));
#4031=EDGE_LOOP('',(#14646,#14647,#14648,#14649));
#4032=EDGE_LOOP('',(#14650,#14651,#14652,#14653));
#4033=EDGE_LOOP('',(#14654,#14655,#14656,#14657));
#4034=EDGE_LOOP('',(#14658,#14659,#14660,#14661));
#4035=EDGE_LOOP('',(#14662,#14663,#14664,#14665));
#4036=EDGE_LOOP('',(#14666,#14667,#14668,#14669));
#4037=EDGE_LOOP('',(#14670,#14671,#14672,#14673));
#4038=EDGE_LOOP('',(#14674,#14675,#14676,#14677));
#4039=EDGE_LOOP('',(#14678,#14679,#14680,#14681));
#4040=EDGE_LOOP('',(#14682,#14683,#14684,#14685));
#4041=EDGE_LOOP('',(#14686,#14687,#14688,#14689));
#4042=EDGE_LOOP('',(#14690,#14691,#14692,#14693));
#4043=EDGE_LOOP('',(#14694,#14695,#14696,#14697,#14698,#14699,#14700,#14701,
#14702,#14703,#14704,#14705,#14706,#14707,#14708,#14709,#14710,#14711,#14712,
#14713,#14714,#14715,#14716,#14717,#14718,#14719,#14720,#14721,#14722,#14723,
#14724,#14725,#14726,#14727,#14728,#14729,#14730,#14731,#14732,#14733,#14734,
#14735,#14736,#14737,#14738,#14739,#14740,#14741,#14742,#14743,#14744,#14745,
#14746,#14747,#14748,#14749,#14750,#14751,#14752,#14753,#14754,#14755,#14756,
#14757,#14758,#14759,#14760,#14761,#14762,#14763,#14764,#14765,#14766,#14767,
#14768,#14769,#14770,#14771,#14772,#14773,#14774,#14775,#14776,#14777,#14778,
#14779,#14780,#14781,#14782,#14783,#14784,#14785,#14786,#14787,#14788,#14789,
#14790,#14791,#14792,#14793,#14794,#14795,#14796,#14797,#14798,#14799,#14800,
#14801,#14802,#14803,#14804,#14805,#14806,#14807,#14808,#14809,#14810,#14811,
#14812,#14813,#14814,#14815,#14816,#14817,#14818,#14819,#14820,#14821,#14822,
#14823,#14824,#14825,#14826,#14827,#14828,#14829,#14830,#14831,#14832,#14833,
#14834,#14835,#14836,#14837,#14838,#14839,#14840,#14841,#14842,#14843,#14844,
#14845,#14846,#14847,#14848,#14849,#14850,#14851,#14852,#14853));
#4044=EDGE_LOOP('',(#14854));
#4045=EDGE_LOOP('',(#14855,#14856,#14857,#14858));
#4885=LINE('',#49609,#5909);
#4886=LINE('',#49611,#5910);
#4887=LINE('',#49613,#5911);
#4888=LINE('',#49614,#5912);
#4889=LINE('',#49617,#5913);
#4890=LINE('',#49619,#5914);
#4891=LINE('',#49620,#5915);
#4892=LINE('',#49623,#5916);
#4893=LINE('',#49625,#5917);
#4894=LINE('',#49626,#5918);
#4895=LINE('',#49703,#5919);
#4896=LINE('',#49849,#5920);
#4897=LINE('',#49995,#5921);
#4898=LINE('',#50141,#5922);
#4899=LINE('',#50287,#5923);
#4900=LINE('',#50433,#5924);
#4901=LINE('',#50579,#5925);
#4902=LINE('',#50725,#5926);
#4903=LINE('',#50871,#5927);
#4904=LINE('',#51017,#5928);
#4905=LINE('',#51163,#5929);
#4906=LINE('',#51309,#5930);
#4907=LINE('',#51455,#5931);
#4908=LINE('',#51601,#5932);
#4909=LINE('',#51747,#5933);
#4910=LINE('',#51893,#5934);
#4911=LINE('',#52039,#5935);
#4912=LINE('',#52185,#5936);
#4913=LINE('',#52331,#5937);
#4914=LINE('',#52477,#5938);
#4915=LINE('',#52623,#5939);
#4916=LINE('',#52769,#5940);
#4917=LINE('',#52915,#5941);
#4918=LINE('',#53061,#5942);
#4919=LINE('',#53207,#5943);
#4920=LINE('',#53353,#5944);
#4921=LINE('',#53499,#5945);
#4922=LINE('',#53645,#5946);
#4923=LINE('',#53791,#5947);
#4924=LINE('',#53937,#5948);
#4925=LINE('',#54083,#5949);
#4926=LINE('',#54229,#5950);
#4927=LINE('',#54375,#5951);
#4928=LINE('',#54521,#5952);
#4929=LINE('',#54667,#5953);
#4930=LINE('',#54813,#5954);
#4931=LINE('',#54959,#5955);
#4932=LINE('',#55105,#5956);
#4933=LINE('',#55251,#5957);
#4934=LINE('',#55397,#5958);
#4935=LINE('',#55475,#5959);
#4936=LINE('',#55696,#5960);
#4937=LINE('',#55845,#5961);
#4938=LINE('',#55917,#5962);
#4939=LINE('',#56138,#5963);
#4940=LINE('',#56287,#5964);
#4941=LINE('',#56359,#5965);
#4942=LINE('',#56580,#5966);
#4943=LINE('',#56729,#5967);
#4944=LINE('',#56801,#5968);
#4945=LINE('',#57022,#5969);
#4946=LINE('',#57171,#5970);
#4947=LINE('',#57243,#5971);
#4948=LINE('',#57464,#5972);
#4949=LINE('',#57613,#5973);
#4950=LINE('',#57685,#5974);
#4951=LINE('',#57906,#5975);
#4952=LINE('',#58055,#5976);
#4953=LINE('',#58127,#5977);
#4954=LINE('',#58348,#5978);
#4955=LINE('',#58497,#5979);
#4956=LINE('',#58569,#5980);
#4957=LINE('',#58790,#5981);
#4958=LINE('',#58939,#5982);
#4959=LINE('',#59011,#5983);
#4960=LINE('',#59232,#5984);
#4961=LINE('',#59381,#5985);
#4962=LINE('',#59453,#5986);
#4963=LINE('',#59674,#5987);
#4964=LINE('',#59823,#5988);
#4965=LINE('',#59895,#5989);
#4966=LINE('',#60116,#5990);
#4967=LINE('',#60265,#5991);
#4968=LINE('',#60337,#5992);
#4969=LINE('',#60558,#5993);
#4970=LINE('',#60707,#5994);
#4971=LINE('',#60779,#5995);
#4972=LINE('',#61000,#5996);
#4973=LINE('',#61149,#5997);
#4974=LINE('',#61221,#5998);
#4975=LINE('',#61442,#5999);
#4976=LINE('',#61591,#6000);
#4977=LINE('',#61663,#6001);
#4978=LINE('',#61884,#6002);
#4979=LINE('',#62033,#6003);
#4980=LINE('',#62105,#6004);
#4981=LINE('',#62326,#6005);
#4982=LINE('',#62475,#6006);
#4983=LINE('',#62547,#6007);
#4984=LINE('',#62768,#6008);
#4985=LINE('',#62917,#6009);
#4986=LINE('',#62989,#6010);
#4987=LINE('',#63210,#6011);
#4988=LINE('',#63359,#6012);
#4989=LINE('',#63431,#6013);
#4990=LINE('',#63652,#6014);
#4991=LINE('',#63801,#6015);
#4992=LINE('',#63873,#6016);
#4993=LINE('',#64094,#6017);
#4994=LINE('',#64243,#6018);
#4995=LINE('',#64315,#6019);
#4996=LINE('',#64536,#6020);
#4997=LINE('',#64685,#6021);
#4998=LINE('',#64757,#6022);
#4999=LINE('',#64978,#6023);
#5000=LINE('',#65127,#6024);
#5001=LINE('',#65199,#6025);
#5002=LINE('',#65420,#6026);
#5003=LINE('',#65569,#6027);
#5004=LINE('',#65641,#6028);
#5005=LINE('',#65862,#6029);
#5006=LINE('',#66011,#6030);
#5007=LINE('',#66083,#6031);
#5008=LINE('',#66304,#6032);
#5009=LINE('',#66453,#6033);
#5010=LINE('',#66525,#6034);
#5011=LINE('',#66746,#6035);
#5012=LINE('',#66895,#6036);
#5013=LINE('',#66967,#6037);
#5014=LINE('',#67188,#6038);
#5015=LINE('',#67337,#6039);
#5016=LINE('',#67409,#6040);
#5017=LINE('',#67630,#6041);
#5018=LINE('',#67779,#6042);
#5019=LINE('',#67851,#6043);
#5020=LINE('',#68072,#6044);
#5021=LINE('',#68221,#6045);
#5022=LINE('',#68293,#6046);
#5023=LINE('',#68514,#6047);
#5024=LINE('',#68663,#6048);
#5025=LINE('',#68735,#6049);
#5026=LINE('',#68956,#6050);
#5027=LINE('',#69105,#6051);
#5028=LINE('',#69177,#6052);
#5029=LINE('',#69398,#6053);
#5030=LINE('',#69547,#6054);
#5031=LINE('',#69619,#6055);
#5032=LINE('',#69840,#6056);
#5033=LINE('',#69989,#6057);
#5034=LINE('',#70061,#6058);
#5035=LINE('',#70282,#6059);
#5036=LINE('',#70431,#6060);
#5037=LINE('',#70503,#6061);
#5038=LINE('',#70724,#6062);
#5039=LINE('',#70873,#6063);
#5040=LINE('',#70945,#6064);
#5041=LINE('',#71166,#6065);
#5042=LINE('',#71315,#6066);
#5043=LINE('',#71387,#6067);
#5044=LINE('',#71608,#6068);
#5045=LINE('',#71757,#6069);
#5046=LINE('',#71829,#6070);
#5047=LINE('',#72050,#6071);
#5048=LINE('',#72199,#6072);
#5049=LINE('',#72271,#6073);
#5050=LINE('',#72492,#6074);
#5051=LINE('',#72495,#6075);
#5052=LINE('',#72496,#6076);
#5053=LINE('',#72871,#6077);
#5054=LINE('',#73153,#6078);
#5055=LINE('',#73155,#6079);
#5909=VECTOR('',#22157,1.);
#5910=VECTOR('',#22158,1.);
#5911=VECTOR('',#22159,1.);
#5912=VECTOR('',#22160,1.);
#5913=VECTOR('',#22163,1.);
#5914=VECTOR('',#22164,1.);
#5915=VECTOR('',#22165,1.);
#5916=VECTOR('',#22168,1.);
#5917=VECTOR('',#22169,1.);
#5918=VECTOR('',#22170,1.);
#5919=VECTOR('',#22175,1.);
#5920=VECTOR('',#22178,1.);
#5921=VECTOR('',#22181,1.);
#5922=VECTOR('',#22184,1.);
#5923=VECTOR('',#22187,1.);
#5924=VECTOR('',#22190,1.);
#5925=VECTOR('',#22193,1.);
#5926=VECTOR('',#22196,1.);
#5927=VECTOR('',#22199,1.);
#5928=VECTOR('',#22202,1.);
#5929=VECTOR('',#22205,1.);
#5930=VECTOR('',#22208,1.);
#5931=VECTOR('',#22211,1.);
#5932=VECTOR('',#22214,1.);
#5933=VECTOR('',#22217,1.);
#5934=VECTOR('',#22220,1.);
#5935=VECTOR('',#22223,1.);
#5936=VECTOR('',#22226,1.);
#5937=VECTOR('',#22229,1.);
#5938=VECTOR('',#22232,1.);
#5939=VECTOR('',#22235,1.);
#5940=VECTOR('',#22238,1.);
#5941=VECTOR('',#22241,1.);
#5942=VECTOR('',#22244,1.);
#5943=VECTOR('',#22247,1.);
#5944=VECTOR('',#22250,1.);
#5945=VECTOR('',#22253,1.);
#5946=VECTOR('',#22256,1.);
#5947=VECTOR('',#22259,1.);
#5948=VECTOR('',#22262,1.);
#5949=VECTOR('',#22265,1.);
#5950=VECTOR('',#22268,1.);
#5951=VECTOR('',#22271,1.);
#5952=VECTOR('',#22274,1.);
#5953=VECTOR('',#22277,1.);
#5954=VECTOR('',#22280,1.);
#5955=VECTOR('',#22283,1.);
#5956=VECTOR('',#22286,1.);
#5957=VECTOR('',#22289,1.);
#5958=VECTOR('',#22292,1.);
#5959=VECTOR('',#22303,2.);
#5960=VECTOR('',#22308,1.);
#5961=VECTOR('',#22309,1.);
#5962=VECTOR('',#22312,1.);
#5963=VECTOR('',#22317,1.);
#5964=VECTOR('',#22318,1.);
#5965=VECTOR('',#22321,1.);
#5966=VECTOR('',#22326,1.);
#5967=VECTOR('',#22327,1.);
#5968=VECTOR('',#22330,1.);
#5969=VECTOR('',#22335,1.);
#5970=VECTOR('',#22336,1.);
#5971=VECTOR('',#22339,1.);
#5972=VECTOR('',#22344,1.);
#5973=VECTOR('',#22345,1.);
#5974=VECTOR('',#22348,1.);
#5975=VECTOR('',#22353,1.);
#5976=VECTOR('',#22354,1.);
#5977=VECTOR('',#22357,1.);
#5978=VECTOR('',#22362,1.);
#5979=VECTOR('',#22363,1.);
#5980=VECTOR('',#22366,1.);
#5981=VECTOR('',#22371,1.);
#5982=VECTOR('',#22372,1.);
#5983=VECTOR('',#22375,1.);
#5984=VECTOR('',#22380,1.);
#5985=VECTOR('',#22381,1.);
#5986=VECTOR('',#22384,1.);
#5987=VECTOR('',#22389,1.);
#5988=VECTOR('',#22390,1.);
#5989=VECTOR('',#22393,1.);
#5990=VECTOR('',#22398,1.);
#5991=VECTOR('',#22399,1.);
#5992=VECTOR('',#22402,1.);
#5993=VECTOR('',#22407,1.);
#5994=VECTOR('',#22408,1.);
#5995=VECTOR('',#22411,1.);
#5996=VECTOR('',#22416,1.);
#5997=VECTOR('',#22417,1.);
#5998=VECTOR('',#22420,1.);
#5999=VECTOR('',#22425,1.);
#6000=VECTOR('',#22426,1.);
#6001=VECTOR('',#22429,1.);
#6002=VECTOR('',#22434,1.);
#6003=VECTOR('',#22435,1.);
#6004=VECTOR('',#22438,1.);
#6005=VECTOR('',#22443,1.);
#6006=VECTOR('',#22444,1.);
#6007=VECTOR('',#22447,1.);
#6008=VECTOR('',#22452,1.);
#6009=VECTOR('',#22453,1.);
#6010=VECTOR('',#22456,1.);
#6011=VECTOR('',#22461,1.);
#6012=VECTOR('',#22462,1.);
#6013=VECTOR('',#22465,1.);
#6014=VECTOR('',#22470,1.);
#6015=VECTOR('',#22471,1.);
#6016=VECTOR('',#22474,1.);
#6017=VECTOR('',#22479,1.);
#6018=VECTOR('',#22480,1.);
#6019=VECTOR('',#22483,1.);
#6020=VECTOR('',#22488,1.);
#6021=VECTOR('',#22489,1.);
#6022=VECTOR('',#22492,1.);
#6023=VECTOR('',#22497,1.);
#6024=VECTOR('',#22498,1.);
#6025=VECTOR('',#22501,1.);
#6026=VECTOR('',#22506,1.);
#6027=VECTOR('',#22507,1.);
#6028=VECTOR('',#22510,1.);
#6029=VECTOR('',#22515,1.);
#6030=VECTOR('',#22516,1.);
#6031=VECTOR('',#22519,1.);
#6032=VECTOR('',#22524,1.);
#6033=VECTOR('',#22525,1.);
#6034=VECTOR('',#22528,1.);
#6035=VECTOR('',#22533,1.);
#6036=VECTOR('',#22534,1.);
#6037=VECTOR('',#22537,1.);
#6038=VECTOR('',#22542,1.);
#6039=VECTOR('',#22543,1.);
#6040=VECTOR('',#22546,1.);
#6041=VECTOR('',#22551,1.);
#6042=VECTOR('',#22552,1.);
#6043=VECTOR('',#22555,1.);
#6044=VECTOR('',#22560,1.);
#6045=VECTOR('',#22561,1.);
#6046=VECTOR('',#22564,1.);
#6047=VECTOR('',#22569,1.);
#6048=VECTOR('',#22570,1.);
#6049=VECTOR('',#22573,1.);
#6050=VECTOR('',#22578,1.);
#6051=VECTOR('',#22579,1.);
#6052=VECTOR('',#22582,1.);
#6053=VECTOR('',#22587,1.);
#6054=VECTOR('',#22588,1.);
#6055=VECTOR('',#22591,1.);
#6056=VECTOR('',#22596,1.);
#6057=VECTOR('',#22597,1.);
#6058=VECTOR('',#22600,1.);
#6059=VECTOR('',#22605,1.);
#6060=VECTOR('',#22606,1.);
#6061=VECTOR('',#22609,1.);
#6062=VECTOR('',#22614,1.);
#6063=VECTOR('',#22615,1.);
#6064=VECTOR('',#22618,1.);
#6065=VECTOR('',#22623,1.);
#6066=VECTOR('',#22624,1.);
#6067=VECTOR('',#22627,1.);
#6068=VECTOR('',#22632,1.);
#6069=VECTOR('',#22633,1.);
#6070=VECTOR('',#22636,1.);
#6071=VECTOR('',#22641,1.);
#6072=VECTOR('',#22642,1.);
#6073=VECTOR('',#22645,1.);
#6074=VECTOR('',#22650,1.);
#6075=VECTOR('',#22653,1.);
#6076=VECTOR('',#22654,1.);
#6077=VECTOR('',#22659,1.);
#6078=VECTOR('',#22660,1.);
#6079=VECTOR('',#22663,1.);
#6740=CIRCLE('',#18250,3.75);
#6741=CIRCLE('',#18251,3.75);
#6742=CIRCLE('',#18252,3.75);
#6743=CIRCLE('',#18253,3.75);
#6744=CIRCLE('',#18254,3.75);
#6745=CIRCLE('',#18255,3.75);
#6746=CIRCLE('',#18256,3.75);
#6747=CIRCLE('',#18257,3.75);
#6748=CIRCLE('',#18258,3.75);
#6749=CIRCLE('',#18259,3.75);
#6750=CIRCLE('',#18260,3.75);
#6751=CIRCLE('',#18261,3.75);
#6752=CIRCLE('',#18262,3.75);
#6753=CIRCLE('',#18263,3.75);
#6754=CIRCLE('',#18264,3.75);
#6755=CIRCLE('',#18265,3.75);
#6756=CIRCLE('',#18266,3.75);
#6757=CIRCLE('',#18267,3.75);
#6758=CIRCLE('',#18268,3.75);
#6759=CIRCLE('',#18269,3.75);
#6760=CIRCLE('',#18270,3.75);
#6761=CIRCLE('',#18271,3.75);
#6762=CIRCLE('',#18272,3.75);
#6763=CIRCLE('',#18273,3.75);
#6764=CIRCLE('',#18274,3.75);
#6765=CIRCLE('',#18275,3.75);
#6766=CIRCLE('',#18276,3.75);
#6767=CIRCLE('',#18277,3.75);
#6768=CIRCLE('',#18278,3.75);
#6769=CIRCLE('',#18279,3.75);
#6770=CIRCLE('',#18280,3.75);
#6771=CIRCLE('',#18281,3.75);
#6772=CIRCLE('',#18282,3.75);
#6773=CIRCLE('',#18283,3.75);
#6774=CIRCLE('',#18284,3.75);
#6775=CIRCLE('',#18285,3.75);
#6776=CIRCLE('',#18286,3.75);
#6777=CIRCLE('',#18287,3.75);
#6778=CIRCLE('',#18288,3.75);
#6779=CIRCLE('',#18289,3.75);
#6780=CIRCLE('',#18290,1.);
#6781=CIRCLE('',#18292,1.);
#6782=CIRCLE('',#18294,2.);
#6783=CIRCLE('',#18295,2.);
#6784=CIRCLE('',#18299,3.75);
#6785=CIRCLE('',#18302,3.75);
#6786=CIRCLE('',#18305,3.75);
#6787=CIRCLE('',#18308,3.75);
#6788=CIRCLE('',#18311,3.75);
#6789=CIRCLE('',#18314,3.75);
#6790=CIRCLE('',#18317,3.75);
#6791=CIRCLE('',#18320,3.75);
#6792=CIRCLE('',#18323,3.75);
#6793=CIRCLE('',#18326,3.75);
#6794=CIRCLE('',#18329,3.75);
#6795=CIRCLE('',#18332,3.75);
#6796=CIRCLE('',#18335,3.75);
#6797=CIRCLE('',#18338,3.75);
#6798=CIRCLE('',#18341,3.75);
#6799=CIRCLE('',#18344,3.75);
#6800=CIRCLE('',#18347,3.75);
#6801=CIRCLE('',#18350,3.75);
#6802=CIRCLE('',#18353,3.75);
#6803=CIRCLE('',#18356,3.75);
#6804=CIRCLE('',#18359,3.75);
#6805=CIRCLE('',#18362,3.75);
#6806=CIRCLE('',#18365,3.75);
#6807=CIRCLE('',#18368,3.75);
#6808=CIRCLE('',#18371,3.75);
#6809=CIRCLE('',#18374,3.75);
#6810=CIRCLE('',#18377,3.75);
#6811=CIRCLE('',#18380,3.75);
#6812=CIRCLE('',#18383,3.75);
#6813=CIRCLE('',#18386,3.75);
#6814=CIRCLE('',#18389,3.75);
#6815=CIRCLE('',#18392,3.75);
#6816=CIRCLE('',#18395,3.75);
#6817=CIRCLE('',#18398,3.75);
#6818=CIRCLE('',#18401,3.75);
#6819=CIRCLE('',#18404,3.75);
#6820=CIRCLE('',#18407,3.75);
#6821=CIRCLE('',#18410,3.75);
#6822=CIRCLE('',#18413,3.75);
#6823=CIRCLE('',#18416,3.75);
#7961=VERTEX_POINT('',#49607);
#7962=VERTEX_POINT('',#49608);
#7963=VERTEX_POINT('',#49610);
#7964=VERTEX_POINT('',#49612);
#7965=VERTEX_POINT('',#49616);
#7966=VERTEX_POINT('',#49618);
#7967=VERTEX_POINT('',#49622);
#7968=VERTEX_POINT('',#49624);
#7969=VERTEX_POINT('',#49628);
#7970=VERTEX_POINT('',#49629);
#7971=VERTEX_POINT('',#49631);
#7972=VERTEX_POINT('',#49702);
#7973=VERTEX_POINT('',#49704);
#7974=VERTEX_POINT('',#49775);
#7975=VERTEX_POINT('',#49777);
#7976=VERTEX_POINT('',#49848);
#7977=VERTEX_POINT('',#49850);
#7978=VERTEX_POINT('',#49921);
#7979=VERTEX_POINT('',#49923);
#7980=VERTEX_POINT('',#49994);
#7981=VERTEX_POINT('',#49996);
#7982=VERTEX_POINT('',#50067);
#7983=VERTEX_POINT('',#50069);
#7984=VERTEX_POINT('',#50140);
#7985=VERTEX_POINT('',#50142);
#7986=VERTEX_POINT('',#50213);
#7987=VERTEX_POINT('',#50215);
#7988=VERTEX_POINT('',#50286);
#7989=VERTEX_POINT('',#50288);
#7990=VERTEX_POINT('',#50359);
#7991=VERTEX_POINT('',#50361);
#7992=VERTEX_POINT('',#50432);
#7993=VERTEX_POINT('',#50434);
#7994=VERTEX_POINT('',#50505);
#7995=VERTEX_POINT('',#50507);
#7996=VERTEX_POINT('',#50578);
#7997=VERTEX_POINT('',#50580);
#7998=VERTEX_POINT('',#50651);
#7999=VERTEX_POINT('',#50653);
#8000=VERTEX_POINT('',#50724);
#8001=VERTEX_POINT('',#50726);
#8002=VERTEX_POINT('',#50797);
#8003=VERTEX_POINT('',#50799);
#8004=VERTEX_POINT('',#50870);
#8005=VERTEX_POINT('',#50872);
#8006=VERTEX_POINT('',#50943);
#8007=VERTEX_POINT('',#50945);
#8008=VERTEX_POINT('',#51016);
#8009=VERTEX_POINT('',#51018);
#8010=VERTEX_POINT('',#51089);
#8011=VERTEX_POINT('',#51091);
#8012=VERTEX_POINT('',#51162);
#8013=VERTEX_POINT('',#51164);
#8014=VERTEX_POINT('',#51235);
#8015=VERTEX_POINT('',#51237);
#8016=VERTEX_POINT('',#51308);
#8017=VERTEX_POINT('',#51310);
#8018=VERTEX_POINT('',#51381);
#8019=VERTEX_POINT('',#51383);
#8020=VERTEX_POINT('',#51454);
#8021=VERTEX_POINT('',#51456);
#8022=VERTEX_POINT('',#51527);
#8023=VERTEX_POINT('',#51529);
#8024=VERTEX_POINT('',#51600);
#8025=VERTEX_POINT('',#51602);
#8026=VERTEX_POINT('',#51673);
#8027=VERTEX_POINT('',#51675);
#8028=VERTEX_POINT('',#51746);
#8029=VERTEX_POINT('',#51748);
#8030=VERTEX_POINT('',#51819);
#8031=VERTEX_POINT('',#51821);
#8032=VERTEX_POINT('',#51892);
#8033=VERTEX_POINT('',#51894);
#8034=VERTEX_POINT('',#51965);
#8035=VERTEX_POINT('',#51967);
#8036=VERTEX_POINT('',#52038);
#8037=VERTEX_POINT('',#52040);
#8038=VERTEX_POINT('',#52111);
#8039=VERTEX_POINT('',#52113);
#8040=VERTEX_POINT('',#52184);
#8041=VERTEX_POINT('',#52186);
#8042=VERTEX_POINT('',#52257);
#8043=VERTEX_POINT('',#52259);
#8044=VERTEX_POINT('',#52330);
#8045=VERTEX_POINT('',#52332);
#8046=VERTEX_POINT('',#52403);
#8047=VERTEX_POINT('',#52405);
#8048=VERTEX_POINT('',#52476);
#8049=VERTEX_POINT('',#52478);
#8050=VERTEX_POINT('',#52549);
#8051=VERTEX_POINT('',#52551);
#8052=VERTEX_POINT('',#52622);
#8053=VERTEX_POINT('',#52624);
#8054=VERTEX_POINT('',#52695);
#8055=VERTEX_POINT('',#52697);
#8056=VERTEX_POINT('',#52768);
#8057=VERTEX_POINT('',#52770);
#8058=VERTEX_POINT('',#52841);
#8059=VERTEX_POINT('',#52843);
#8060=VERTEX_POINT('',#52914);
#8061=VERTEX_POINT('',#52916);
#8062=VERTEX_POINT('',#52987);
#8063=VERTEX_POINT('',#52989);
#8064=VERTEX_POINT('',#53060);
#8065=VERTEX_POINT('',#53062);
#8066=VERTEX_POINT('',#53133);
#8067=VERTEX_POINT('',#53135);
#8068=VERTEX_POINT('',#53206);
#8069=VERTEX_POINT('',#53208);
#8070=VERTEX_POINT('',#53279);
#8071=VERTEX_POINT('',#53281);
#8072=VERTEX_POINT('',#53352);
#8073=VERTEX_POINT('',#53354);
#8074=VERTEX_POINT('',#53425);
#8075=VERTEX_POINT('',#53427);
#8076=VERTEX_POINT('',#53498);
#8077=VERTEX_POINT('',#53500);
#8078=VERTEX_POINT('',#53571);
#8079=VERTEX_POINT('',#53573);
#8080=VERTEX_POINT('',#53644);
#8081=VERTEX_POINT('',#53646);
#8082=VERTEX_POINT('',#53717);
#8083=VERTEX_POINT('',#53719);
#8084=VERTEX_POINT('',#53790);
#8085=VERTEX_POINT('',#53792);
#8086=VERTEX_POINT('',#53863);
#8087=VERTEX_POINT('',#53865);
#8088=VERTEX_POINT('',#53936);
#8089=VERTEX_POINT('',#53938);
#8090=VERTEX_POINT('',#54009);
#8091=VERTEX_POINT('',#54011);
#8092=VERTEX_POINT('',#54082);
#8093=VERTEX_POINT('',#54084);
#8094=VERTEX_POINT('',#54155);
#8095=VERTEX_POINT('',#54157);
#8096=VERTEX_POINT('',#54228);
#8097=VERTEX_POINT('',#54230);
#8098=VERTEX_POINT('',#54301);
#8099=VERTEX_POINT('',#54303);
#8100=VERTEX_POINT('',#54374);
#8101=VERTEX_POINT('',#54376);
#8102=VERTEX_POINT('',#54447);
#8103=VERTEX_POINT('',#54449);
#8104=VERTEX_POINT('',#54520);
#8105=VERTEX_POINT('',#54522);
#8106=VERTEX_POINT('',#54593);
#8107=VERTEX_POINT('',#54595);
#8108=VERTEX_POINT('',#54666);
#8109=VERTEX_POINT('',#54668);
#8110=VERTEX_POINT('',#54739);
#8111=VERTEX_POINT('',#54741);
#8112=VERTEX_POINT('',#54812);
#8113=VERTEX_POINT('',#54814);
#8114=VERTEX_POINT('',#54885);
#8115=VERTEX_POINT('',#54887);
#8116=VERTEX_POINT('',#54958);
#8117=VERTEX_POINT('',#54960);
#8118=VERTEX_POINT('',#55031);
#8119=VERTEX_POINT('',#55033);
#8120=VERTEX_POINT('',#55104);
#8121=VERTEX_POINT('',#55106);
#8122=VERTEX_POINT('',#55177);
#8123=VERTEX_POINT('',#55179);
#8124=VERTEX_POINT('',#55250);
#8125=VERTEX_POINT('',#55252);
#8126=VERTEX_POINT('',#55323);
#8127=VERTEX_POINT('',#55325);
#8128=VERTEX_POINT('',#55396);
#8129=VERTEX_POINT('',#55472);
#8130=VERTEX_POINT('',#55474);
#8131=VERTEX_POINT('',#55618);
#8132=VERTEX_POINT('',#55625);
#8133=VERTEX_POINT('',#55837);
#8134=VERTEX_POINT('',#55844);
#8135=VERTEX_POINT('',#55919);
#8136=VERTEX_POINT('',#56067);
#8137=VERTEX_POINT('',#56279);
#8138=VERTEX_POINT('',#56286);
#8139=VERTEX_POINT('',#56361);
#8140=VERTEX_POINT('',#56509);
#8141=VERTEX_POINT('',#56721);
#8142=VERTEX_POINT('',#56728);
#8143=VERTEX_POINT('',#56803);
#8144=VERTEX_POINT('',#56951);
#8145=VERTEX_POINT('',#57163);
#8146=VERTEX_POINT('',#57170);
#8147=VERTEX_POINT('',#57245);
#8148=VERTEX_POINT('',#57393);
#8149=VERTEX_POINT('',#57605);
#8150=VERTEX_POINT('',#57612);
#8151=VERTEX_POINT('',#57687);
#8152=VERTEX_POINT('',#57835);
#8153=VERTEX_POINT('',#58047);
#8154=VERTEX_POINT('',#58054);
#8155=VERTEX_POINT('',#58129);
#8156=VERTEX_POINT('',#58277);
#8157=VERTEX_POINT('',#58489);
#8158=VERTEX_POINT('',#58496);
#8159=VERTEX_POINT('',#58571);
#8160=VERTEX_POINT('',#58719);
#8161=VERTEX_POINT('',#58931);
#8162=VERTEX_POINT('',#58938);
#8163=VERTEX_POINT('',#59013);
#8164=VERTEX_POINT('',#59161);
#8165=VERTEX_POINT('',#59373);
#8166=VERTEX_POINT('',#59380);
#8167=VERTEX_POINT('',#59455);
#8168=VERTEX_POINT('',#59603);
#8169=VERTEX_POINT('',#59815);
#8170=VERTEX_POINT('',#59822);
#8171=VERTEX_POINT('',#59897);
#8172=VERTEX_POINT('',#60045);
#8173=VERTEX_POINT('',#60257);
#8174=VERTEX_POINT('',#60264);
#8175=VERTEX_POINT('',#60339);
#8176=VERTEX_POINT('',#60487);
#8177=VERTEX_POINT('',#60699);
#8178=VERTEX_POINT('',#60706);
#8179=VERTEX_POINT('',#60781);
#8180=VERTEX_POINT('',#60929);
#8181=VERTEX_POINT('',#61141);
#8182=VERTEX_POINT('',#61148);
#8183=VERTEX_POINT('',#61223);
#8184=VERTEX_POINT('',#61371);
#8185=VERTEX_POINT('',#61583);
#8186=VERTEX_POINT('',#61590);
#8187=VERTEX_POINT('',#61665);
#8188=VERTEX_POINT('',#61813);
#8189=VERTEX_POINT('',#62025);
#8190=VERTEX_POINT('',#62032);
#8191=VERTEX_POINT('',#62107);
#8192=VERTEX_POINT('',#62255);
#8193=VERTEX_POINT('',#62467);
#8194=VERTEX_POINT('',#62474);
#8195=VERTEX_POINT('',#62549);
#8196=VERTEX_POINT('',#62697);
#8197=VERTEX_POINT('',#62909);
#8198=VERTEX_POINT('',#62916);
#8199=VERTEX_POINT('',#62991);
#8200=VERTEX_POINT('',#63139);
#8201=VERTEX_POINT('',#63351);
#8202=VERTEX_POINT('',#63358);
#8203=VERTEX_POINT('',#63433);
#8204=VERTEX_POINT('',#63581);
#8205=VERTEX_POINT('',#63793);
#8206=VERTEX_POINT('',#63800);
#8207=VERTEX_POINT('',#63875);
#8208=VERTEX_POINT('',#64023);
#8209=VERTEX_POINT('',#64235);
#8210=VERTEX_POINT('',#64242);
#8211=VERTEX_POINT('',#64317);
#8212=VERTEX_POINT('',#64465);
#8213=VERTEX_POINT('',#64677);
#8214=VERTEX_POINT('',#64684);
#8215=VERTEX_POINT('',#64759);
#8216=VERTEX_POINT('',#64907);
#8217=VERTEX_POINT('',#65119);
#8218=VERTEX_POINT('',#65126);
#8219=VERTEX_POINT('',#65201);
#8220=VERTEX_POINT('',#65349);
#8221=VERTEX_POINT('',#65561);
#8222=VERTEX_POINT('',#65568);
#8223=VERTEX_POINT('',#65643);
#8224=VERTEX_POINT('',#65791);
#8225=VERTEX_POINT('',#66003);
#8226=VERTEX_POINT('',#66010);
#8227=VERTEX_POINT('',#66085);
#8228=VERTEX_POINT('',#66233);
#8229=VERTEX_POINT('',#66445);
#8230=VERTEX_POINT('',#66452);
#8231=VERTEX_POINT('',#66527);
#8232=VERTEX_POINT('',#66675);
#8233=VERTEX_POINT('',#66887);
#8234=VERTEX_POINT('',#66894);
#8235=VERTEX_POINT('',#66969);
#8236=VERTEX_POINT('',#67117);
#8237=VERTEX_POINT('',#67329);
#8238=VERTEX_POINT('',#67336);
#8239=VERTEX_POINT('',#67411);
#8240=VERTEX_POINT('',#67559);
#8241=VERTEX_POINT('',#67771);
#8242=VERTEX_POINT('',#67778);
#8243=VERTEX_POINT('',#67853);
#8244=VERTEX_POINT('',#68001);
#8245=VERTEX_POINT('',#68213);
#8246=VERTEX_POINT('',#68220);
#8247=VERTEX_POINT('',#68295);
#8248=VERTEX_POINT('',#68443);
#8249=VERTEX_POINT('',#68655);
#8250=VERTEX_POINT('',#68662);
#8251=VERTEX_POINT('',#68737);
#8252=VERTEX_POINT('',#68885);
#8253=VERTEX_POINT('',#69097);
#8254=VERTEX_POINT('',#69104);
#8255=VERTEX_POINT('',#69179);
#8256=VERTEX_POINT('',#69327);
#8257=VERTEX_POINT('',#69539);
#8258=VERTEX_POINT('',#69546);
#8259=VERTEX_POINT('',#69621);
#8260=VERTEX_POINT('',#69769);
#8261=VERTEX_POINT('',#69981);
#8262=VERTEX_POINT('',#69988);
#8263=VERTEX_POINT('',#70063);
#8264=VERTEX_POINT('',#70211);
#8265=VERTEX_POINT('',#70423);
#8266=VERTEX_POINT('',#70430);
#8267=VERTEX_POINT('',#70505);
#8268=VERTEX_POINT('',#70653);
#8269=VERTEX_POINT('',#70865);
#8270=VERTEX_POINT('',#70872);
#8271=VERTEX_POINT('',#70947);
#8272=VERTEX_POINT('',#71095);
#8273=VERTEX_POINT('',#71307);
#8274=VERTEX_POINT('',#71314);
#8275=VERTEX_POINT('',#71389);
#8276=VERTEX_POINT('',#71537);
#8277=VERTEX_POINT('',#71749);
#8278=VERTEX_POINT('',#71756);
#8279=VERTEX_POINT('',#71831);
#8280=VERTEX_POINT('',#71979);
#8281=VERTEX_POINT('',#72191);
#8282=VERTEX_POINT('',#72198);
#8283=VERTEX_POINT('',#72273);
#8284=VERTEX_POINT('',#72421);
#8285=VERTEX_POINT('',#72494);
#8286=VERTEX_POINT('',#72637);
#8287=VERTEX_POINT('',#72715);
#8288=VERTEX_POINT('',#72863);
#8289=VERTEX_POINT('',#72870);
#8290=VERTEX_POINT('',#73082);
#9988=EDGE_CURVE('',#7961,#7962,#4885,.T.);
#9989=EDGE_CURVE('',#7963,#7961,#4886,.T.);
#9990=EDGE_CURVE('',#7964,#7963,#4887,.T.);
#9991=EDGE_CURVE('',#7962,#7964,#4888,.T.);
#9992=EDGE_CURVE('',#7965,#7961,#4889,.T.);
#9993=EDGE_CURVE('',#7965,#7966,#4890,.T.);
#9994=EDGE_CURVE('',#7963,#7966,#4891,.T.);
#9995=EDGE_CURVE('',#7967,#7965,#4892,.T.);
#9996=EDGE_CURVE('',#7968,#7967,#4893,.T.);
#9997=EDGE_CURVE('',#7966,#7968,#4894,.T.);
#9998=EDGE_CURVE('',#7969,#7970,#6740,.T.);
#9999=EDGE_CURVE('',#7970,#7971,#331,.T.);
#10000=EDGE_CURVE('',#7971,#7972,#4895,.T.);
#10001=EDGE_CURVE('',#7972,#7973,#332,.T.);
#10002=EDGE_CURVE('',#7973,#7974,#6741,.T.);
#10003=EDGE_CURVE('',#7974,#7975,#333,.T.);
#10004=EDGE_CURVE('',#7975,#7976,#4896,.T.);
#10005=EDGE_CURVE('',#7976,#7977,#334,.T.);
#10006=EDGE_CURVE('',#7977,#7978,#6742,.T.);
#10007=EDGE_CURVE('',#7978,#7979,#335,.T.);
#10008=EDGE_CURVE('',#7979,#7980,#4897,.T.);
#10009=EDGE_CURVE('',#7980,#7981,#336,.T.);
#10010=EDGE_CURVE('',#7981,#7982,#6743,.T.);
#10011=EDGE_CURVE('',#7982,#7983,#337,.T.);
#10012=EDGE_CURVE('',#7983,#7984,#4898,.T.);
#10013=EDGE_CURVE('',#7984,#7985,#338,.T.);
#10014=EDGE_CURVE('',#7985,#7986,#6744,.T.);
#10015=EDGE_CURVE('',#7986,#7987,#339,.T.);
#10016=EDGE_CURVE('',#7987,#7988,#4899,.T.);
#10017=EDGE_CURVE('',#7988,#7989,#340,.T.);
#10018=EDGE_CURVE('',#7989,#7990,#6745,.T.);
#10019=EDGE_CURVE('',#7990,#7991,#341,.T.);
#10020=EDGE_CURVE('',#7991,#7992,#4900,.T.);
#10021=EDGE_CURVE('',#7992,#7993,#342,.T.);
#10022=EDGE_CURVE('',#7993,#7994,#6746,.T.);
#10023=EDGE_CURVE('',#7994,#7995,#343,.T.);
#10024=EDGE_CURVE('',#7995,#7996,#4901,.T.);
#10025=EDGE_CURVE('',#7996,#7997,#344,.T.);
#10026=EDGE_CURVE('',#7997,#7998,#6747,.T.);
#10027=EDGE_CURVE('',#7998,#7999,#345,.T.);
#10028=EDGE_CURVE('',#7999,#8000,#4902,.T.);
#10029=EDGE_CURVE('',#8000,#8001,#346,.T.);
#10030=EDGE_CURVE('',#8001,#8002,#6748,.T.);
#10031=EDGE_CURVE('',#8002,#8003,#347,.T.);
#10032=EDGE_CURVE('',#8003,#8004,#4903,.T.);
#10033=EDGE_CURVE('',#8004,#8005,#348,.T.);
#10034=EDGE_CURVE('',#8005,#8006,#6749,.T.);
#10035=EDGE_CURVE('',#8006,#8007,#349,.T.);
#10036=EDGE_CURVE('',#8007,#8008,#4904,.T.);
#10037=EDGE_CURVE('',#8008,#8009,#350,.T.);
#10038=EDGE_CURVE('',#8009,#8010,#6750,.T.);
#10039=EDGE_CURVE('',#8010,#8011,#351,.T.);
#10040=EDGE_CURVE('',#8011,#8012,#4905,.T.);
#10041=EDGE_CURVE('',#8012,#8013,#352,.T.);
#10042=EDGE_CURVE('',#8013,#8014,#6751,.T.);
#10043=EDGE_CURVE('',#8014,#8015,#353,.T.);
#10044=EDGE_CURVE('',#8015,#8016,#4906,.T.);
#10045=EDGE_CURVE('',#8016,#8017,#354,.T.);
#10046=EDGE_CURVE('',#8017,#8018,#6752,.T.);
#10047=EDGE_CURVE('',#8018,#8019,#355,.T.);
#10048=EDGE_CURVE('',#8019,#8020,#4907,.T.);
#10049=EDGE_CURVE('',#8020,#8021,#356,.T.);
#10050=EDGE_CURVE('',#8021,#8022,#6753,.T.);
#10051=EDGE_CURVE('',#8022,#8023,#357,.T.);
#10052=EDGE_CURVE('',#8023,#8024,#4908,.T.);
#10053=EDGE_CURVE('',#8024,#8025,#358,.T.);
#10054=EDGE_CURVE('',#8025,#8026,#6754,.T.);
#10055=EDGE_CURVE('',#8026,#8027,#359,.T.);
#10056=EDGE_CURVE('',#8027,#8028,#4909,.T.);
#10057=EDGE_CURVE('',#8028,#8029,#360,.T.);
#10058=EDGE_CURVE('',#8029,#8030,#6755,.T.);
#10059=EDGE_CURVE('',#8030,#8031,#361,.T.);
#10060=EDGE_CURVE('',#8031,#8032,#4910,.T.);
#10061=EDGE_CURVE('',#8032,#8033,#362,.T.);
#10062=EDGE_CURVE('',#8033,#8034,#6756,.T.);
#10063=EDGE_CURVE('',#8034,#8035,#363,.T.);
#10064=EDGE_CURVE('',#8035,#8036,#4911,.T.);
#10065=EDGE_CURVE('',#8036,#8037,#364,.T.);
#10066=EDGE_CURVE('',#8037,#8038,#6757,.T.);
#10067=EDGE_CURVE('',#8038,#8039,#365,.T.);
#10068=EDGE_CURVE('',#8039,#8040,#4912,.T.);
#10069=EDGE_CURVE('',#8040,#8041,#366,.T.);
#10070=EDGE_CURVE('',#8041,#8042,#6758,.T.);
#10071=EDGE_CURVE('',#8042,#8043,#367,.T.);
#10072=EDGE_CURVE('',#8043,#8044,#4913,.T.);
#10073=EDGE_CURVE('',#8044,#8045,#368,.T.);
#10074=EDGE_CURVE('',#8045,#8046,#6759,.T.);
#10075=EDGE_CURVE('',#8046,#8047,#369,.T.);
#10076=EDGE_CURVE('',#8047,#8048,#4914,.T.);
#10077=EDGE_CURVE('',#8048,#8049,#370,.T.);
#10078=EDGE_CURVE('',#8049,#8050,#6760,.T.);
#10079=EDGE_CURVE('',#8050,#8051,#371,.T.);
#10080=EDGE_CURVE('',#8051,#8052,#4915,.T.);
#10081=EDGE_CURVE('',#8052,#8053,#372,.T.);
#10082=EDGE_CURVE('',#8053,#8054,#6761,.T.);
#10083=EDGE_CURVE('',#8054,#8055,#373,.T.);
#10084=EDGE_CURVE('',#8055,#8056,#4916,.T.);
#10085=EDGE_CURVE('',#8056,#8057,#374,.T.);
#10086=EDGE_CURVE('',#8057,#8058,#6762,.T.);
#10087=EDGE_CURVE('',#8058,#8059,#375,.T.);
#10088=EDGE_CURVE('',#8059,#8060,#4917,.T.);
#10089=EDGE_CURVE('',#8060,#8061,#376,.T.);
#10090=EDGE_CURVE('',#8061,#8062,#6763,.T.);
#10091=EDGE_CURVE('',#8062,#8063,#377,.T.);
#10092=EDGE_CURVE('',#8063,#8064,#4918,.T.);
#10093=EDGE_CURVE('',#8064,#8065,#378,.T.);
#10094=EDGE_CURVE('',#8065,#8066,#6764,.T.);
#10095=EDGE_CURVE('',#8066,#8067,#379,.T.);
#10096=EDGE_CURVE('',#8067,#8068,#4919,.T.);
#10097=EDGE_CURVE('',#8068,#8069,#380,.T.);
#10098=EDGE_CURVE('',#8069,#8070,#6765,.T.);
#10099=EDGE_CURVE('',#8070,#8071,#381,.T.);
#10100=EDGE_CURVE('',#8071,#8072,#4920,.T.);
#10101=EDGE_CURVE('',#8072,#8073,#382,.T.);
#10102=EDGE_CURVE('',#8073,#8074,#6766,.T.);
#10103=EDGE_CURVE('',#8074,#8075,#383,.T.);
#10104=EDGE_CURVE('',#8075,#8076,#4921,.T.);
#10105=EDGE_CURVE('',#8076,#8077,#384,.T.);
#10106=EDGE_CURVE('',#8077,#8078,#6767,.T.);
#10107=EDGE_CURVE('',#8078,#8079,#385,.T.);
#10108=EDGE_CURVE('',#8079,#8080,#4922,.T.);
#10109=EDGE_CURVE('',#8080,#8081,#386,.T.);
#10110=EDGE_CURVE('',#8081,#8082,#6768,.T.);
#10111=EDGE_CURVE('',#8082,#8083,#387,.T.);
#10112=EDGE_CURVE('',#8083,#8084,#4923,.T.);
#10113=EDGE_CURVE('',#8084,#8085,#388,.T.);
#10114=EDGE_CURVE('',#8085,#8086,#6769,.T.);
#10115=EDGE_CURVE('',#8086,#8087,#389,.T.);
#10116=EDGE_CURVE('',#8087,#8088,#4924,.T.);
#10117=EDGE_CURVE('',#8088,#8089,#390,.T.);
#10118=EDGE_CURVE('',#8089,#8090,#6770,.T.);
#10119=EDGE_CURVE('',#8090,#8091,#391,.T.);
#10120=EDGE_CURVE('',#8091,#8092,#4925,.T.);
#10121=EDGE_CURVE('',#8092,#8093,#392,.T.);
#10122=EDGE_CURVE('',#8093,#8094,#6771,.T.);
#10123=EDGE_CURVE('',#8094,#8095,#393,.T.);
#10124=EDGE_CURVE('',#8095,#8096,#4926,.T.);
#10125=EDGE_CURVE('',#8096,#8097,#394,.T.);
#10126=EDGE_CURVE('',#8097,#8098,#6772,.T.);
#10127=EDGE_CURVE('',#8098,#8099,#395,.T.);
#10128=EDGE_CURVE('',#8099,#8100,#4927,.T.);
#10129=EDGE_CURVE('',#8100,#8101,#396,.T.);
#10130=EDGE_CURVE('',#8101,#8102,#6773,.T.);
#10131=EDGE_CURVE('',#8102,#8103,#397,.T.);
#10132=EDGE_CURVE('',#8103,#8104,#4928,.T.);
#10133=EDGE_CURVE('',#8104,#8105,#398,.T.);
#10134=EDGE_CURVE('',#8105,#8106,#6774,.T.);
#10135=EDGE_CURVE('',#8106,#8107,#399,.T.);
#10136=EDGE_CURVE('',#8107,#8108,#4929,.T.);
#10137=EDGE_CURVE('',#8108,#8109,#400,.T.);
#10138=EDGE_CURVE('',#8109,#8110,#6775,.T.);
#10139=EDGE_CURVE('',#8110,#8111,#401,.T.);
#10140=EDGE_CURVE('',#8111,#8112,#4930,.T.);
#10141=EDGE_CURVE('',#8112,#8113,#402,.T.);
#10142=EDGE_CURVE('',#8113,#8114,#6776,.T.);
#10143=EDGE_CURVE('',#8114,#8115,#403,.T.);
#10144=EDGE_CURVE('',#8115,#8116,#4931,.T.);
#10145=EDGE_CURVE('',#8116,#8117,#404,.T.);
#10146=EDGE_CURVE('',#8117,#8118,#6777,.T.);
#10147=EDGE_CURVE('',#8118,#8119,#405,.T.);
#10148=EDGE_CURVE('',#8119,#8120,#4932,.T.);
#10149=EDGE_CURVE('',#8120,#8121,#406,.T.);
#10150=EDGE_CURVE('',#8121,#8122,#6778,.T.);
#10151=EDGE_CURVE('',#8122,#8123,#407,.T.);
#10152=EDGE_CURVE('',#8123,#8124,#4933,.T.);
#10153=EDGE_CURVE('',#8124,#8125,#408,.T.);
#10154=EDGE_CURVE('',#8125,#8126,#6779,.T.);
#10155=EDGE_CURVE('',#8126,#8127,#409,.T.);
#10156=EDGE_CURVE('',#8127,#8128,#4934,.T.);
#10157=EDGE_CURVE('',#8128,#7969,#410,.T.);
#10158=EDGE_CURVE('',#7968,#7964,#6780,.T.);
#10159=EDGE_CURVE('',#7962,#7967,#6781,.T.);
#10160=EDGE_CURVE('',#8129,#8129,#6782,.T.);
#10161=EDGE_CURVE('',#8129,#8130,#4935,.T.);
#10162=EDGE_CURVE('',#8130,#8130,#6783,.T.);
#10163=EDGE_CURVE('',#8131,#8126,#987,.T.);
#10164=EDGE_CURVE('',#8132,#8131,#411,.T.);
#10165=EDGE_CURVE('',#8127,#8132,#4936,.T.);
#10166=EDGE_CURVE('',#7969,#8133,#988,.T.);
#10167=EDGE_CURVE('',#8128,#8134,#4937,.T.);
#10168=EDGE_CURVE('',#8133,#8134,#412,.T.);
#10169=EDGE_CURVE('',#8134,#8132,#4938,.T.);
#10170=EDGE_CURVE('',#8135,#8133,#6784,.T.);
#10171=EDGE_CURVE('',#8135,#7970,#989,.T.);
#10172=EDGE_CURVE('',#8136,#8135,#413,.T.);
#10173=EDGE_CURVE('',#7971,#8136,#4939,.T.);
#10174=EDGE_CURVE('',#7973,#8137,#990,.T.);
#10175=EDGE_CURVE('',#7972,#8138,#4940,.T.);
#10176=EDGE_CURVE('',#8137,#8138,#414,.T.);
#10177=EDGE_CURVE('',#8138,#8136,#4941,.T.);
#10178=EDGE_CURVE('',#8139,#8137,#6785,.T.);
#10179=EDGE_CURVE('',#8139,#7974,#991,.T.);
#10180=EDGE_CURVE('',#8140,#8139,#415,.T.);
#10181=EDGE_CURVE('',#7975,#8140,#4942,.T.);
#10182=EDGE_CURVE('',#7977,#8141,#992,.T.);
#10183=EDGE_CURVE('',#7976,#8142,#4943,.T.);
#10184=EDGE_CURVE('',#8141,#8142,#416,.T.);
#10185=EDGE_CURVE('',#8142,#8140,#4944,.T.);
#10186=EDGE_CURVE('',#8143,#8141,#6786,.T.);
#10187=EDGE_CURVE('',#8143,#7978,#993,.T.);
#10188=EDGE_CURVE('',#8144,#8143,#417,.T.);
#10189=EDGE_CURVE('',#7979,#8144,#4945,.T.);
#10190=EDGE_CURVE('',#7981,#8145,#994,.T.);
#10191=EDGE_CURVE('',#7980,#8146,#4946,.T.);
#10192=EDGE_CURVE('',#8145,#8146,#418,.T.);
#10193=EDGE_CURVE('',#8146,#8144,#4947,.T.);
#10194=EDGE_CURVE('',#8147,#8145,#6787,.T.);
#10195=EDGE_CURVE('',#8147,#7982,#995,.T.);
#10196=EDGE_CURVE('',#8148,#8147,#419,.T.);
#10197=EDGE_CURVE('',#7983,#8148,#4948,.T.);
#10198=EDGE_CURVE('',#7985,#8149,#996,.T.);
#10199=EDGE_CURVE('',#7984,#8150,#4949,.T.);
#10200=EDGE_CURVE('',#8149,#8150,#420,.T.);
#10201=EDGE_CURVE('',#8150,#8148,#4950,.T.);
#10202=EDGE_CURVE('',#8151,#8149,#6788,.T.);
#10203=EDGE_CURVE('',#8151,#7986,#997,.T.);
#10204=EDGE_CURVE('',#8152,#8151,#421,.T.);
#10205=EDGE_CURVE('',#7987,#8152,#4951,.T.);
#10206=EDGE_CURVE('',#7989,#8153,#998,.T.);
#10207=EDGE_CURVE('',#7988,#8154,#4952,.T.);
#10208=EDGE_CURVE('',#8153,#8154,#422,.T.);
#10209=EDGE_CURVE('',#8154,#8152,#4953,.T.);
#10210=EDGE_CURVE('',#8155,#8153,#6789,.T.);
#10211=EDGE_CURVE('',#8155,#7990,#999,.T.);
#10212=EDGE_CURVE('',#8156,#8155,#423,.T.);
#10213=EDGE_CURVE('',#7991,#8156,#4954,.T.);
#10214=EDGE_CURVE('',#7993,#8157,#1000,.T.);
#10215=EDGE_CURVE('',#7992,#8158,#4955,.T.);
#10216=EDGE_CURVE('',#8157,#8158,#424,.T.);
#10217=EDGE_CURVE('',#8158,#8156,#4956,.T.);
#10218=EDGE_CURVE('',#8159,#8157,#6790,.T.);
#10219=EDGE_CURVE('',#8159,#7994,#1001,.T.);
#10220=EDGE_CURVE('',#8160,#8159,#425,.T.);
#10221=EDGE_CURVE('',#7995,#8160,#4957,.T.);
#10222=EDGE_CURVE('',#7997,#8161,#1002,.T.);
#10223=EDGE_CURVE('',#7996,#8162,#4958,.T.);
#10224=EDGE_CURVE('',#8161,#8162,#426,.T.);
#10225=EDGE_CURVE('',#8162,#8160,#4959,.T.);
#10226=EDGE_CURVE('',#8163,#8161,#6791,.T.);
#10227=EDGE_CURVE('',#8163,#7998,#1003,.T.);
#10228=EDGE_CURVE('',#8164,#8163,#427,.T.);
#10229=EDGE_CURVE('',#7999,#8164,#4960,.T.);
#10230=EDGE_CURVE('',#8001,#8165,#1004,.T.);
#10231=EDGE_CURVE('',#8000,#8166,#4961,.T.);
#10232=EDGE_CURVE('',#8165,#8166,#428,.T.);
#10233=EDGE_CURVE('',#8166,#8164,#4962,.T.);
#10234=EDGE_CURVE('',#8167,#8165,#6792,.T.);
#10235=EDGE_CURVE('',#8167,#8002,#1005,.T.);
#10236=EDGE_CURVE('',#8168,#8167,#429,.T.);
#10237=EDGE_CURVE('',#8003,#8168,#4963,.T.);
#10238=EDGE_CURVE('',#8005,#8169,#1006,.T.);
#10239=EDGE_CURVE('',#8004,#8170,#4964,.T.);
#10240=EDGE_CURVE('',#8169,#8170,#430,.T.);
#10241=EDGE_CURVE('',#8170,#8168,#4965,.T.);
#10242=EDGE_CURVE('',#8171,#8169,#6793,.T.);
#10243=EDGE_CURVE('',#8171,#8006,#1007,.T.);
#10244=EDGE_CURVE('',#8172,#8171,#431,.T.);
#10245=EDGE_CURVE('',#8007,#8172,#4966,.T.);
#10246=EDGE_CURVE('',#8009,#8173,#1008,.T.);
#10247=EDGE_CURVE('',#8008,#8174,#4967,.T.);
#10248=EDGE_CURVE('',#8173,#8174,#432,.T.);
#10249=EDGE_CURVE('',#8174,#8172,#4968,.T.);
#10250=EDGE_CURVE('',#8175,#8173,#6794,.T.);
#10251=EDGE_CURVE('',#8175,#8010,#1009,.T.);
#10252=EDGE_CURVE('',#8176,#8175,#433,.T.);
#10253=EDGE_CURVE('',#8011,#8176,#4969,.T.);
#10254=EDGE_CURVE('',#8013,#8177,#1010,.T.);
#10255=EDGE_CURVE('',#8012,#8178,#4970,.T.);
#10256=EDGE_CURVE('',#8177,#8178,#434,.T.);
#10257=EDGE_CURVE('',#8178,#8176,#4971,.T.);
#10258=EDGE_CURVE('',#8179,#8177,#6795,.T.);
#10259=EDGE_CURVE('',#8179,#8014,#1011,.T.);
#10260=EDGE_CURVE('',#8180,#8179,#435,.T.);
#10261=EDGE_CURVE('',#8015,#8180,#4972,.T.);
#10262=EDGE_CURVE('',#8017,#8181,#1012,.T.);
#10263=EDGE_CURVE('',#8016,#8182,#4973,.T.);
#10264=EDGE_CURVE('',#8181,#8182,#436,.T.);
#10265=EDGE_CURVE('',#8182,#8180,#4974,.T.);
#10266=EDGE_CURVE('',#8183,#8181,#6796,.T.);
#10267=EDGE_CURVE('',#8183,#8018,#1013,.T.);
#10268=EDGE_CURVE('',#8184,#8183,#437,.T.);
#10269=EDGE_CURVE('',#8019,#8184,#4975,.T.);
#10270=EDGE_CURVE('',#8021,#8185,#1014,.T.);
#10271=EDGE_CURVE('',#8020,#8186,#4976,.T.);
#10272=EDGE_CURVE('',#8185,#8186,#438,.T.);
#10273=EDGE_CURVE('',#8186,#8184,#4977,.T.);
#10274=EDGE_CURVE('',#8187,#8185,#6797,.T.);
#10275=EDGE_CURVE('',#8187,#8022,#1015,.T.);
#10276=EDGE_CURVE('',#8188,#8187,#439,.T.);
#10277=EDGE_CURVE('',#8023,#8188,#4978,.T.);
#10278=EDGE_CURVE('',#8025,#8189,#1016,.T.);
#10279=EDGE_CURVE('',#8024,#8190,#4979,.T.);
#10280=EDGE_CURVE('',#8189,#8190,#440,.T.);
#10281=EDGE_CURVE('',#8190,#8188,#4980,.T.);
#10282=EDGE_CURVE('',#8191,#8189,#6798,.T.);
#10283=EDGE_CURVE('',#8191,#8026,#1017,.T.);
#10284=EDGE_CURVE('',#8192,#8191,#441,.T.);
#10285=EDGE_CURVE('',#8027,#8192,#4981,.T.);
#10286=EDGE_CURVE('',#8029,#8193,#1018,.T.);
#10287=EDGE_CURVE('',#8028,#8194,#4982,.T.);
#10288=EDGE_CURVE('',#8193,#8194,#442,.T.);
#10289=EDGE_CURVE('',#8194,#8192,#4983,.T.);
#10290=EDGE_CURVE('',#8195,#8193,#6799,.T.);
#10291=EDGE_CURVE('',#8195,#8030,#1019,.T.);
#10292=EDGE_CURVE('',#8196,#8195,#443,.T.);
#10293=EDGE_CURVE('',#8031,#8196,#4984,.T.);
#10294=EDGE_CURVE('',#8033,#8197,#1020,.T.);
#10295=EDGE_CURVE('',#8032,#8198,#4985,.T.);
#10296=EDGE_CURVE('',#8197,#8198,#444,.T.);
#10297=EDGE_CURVE('',#8198,#8196,#4986,.T.);
#10298=EDGE_CURVE('',#8199,#8197,#6800,.T.);
#10299=EDGE_CURVE('',#8199,#8034,#1021,.T.);
#10300=EDGE_CURVE('',#8200,#8199,#445,.T.);
#10301=EDGE_CURVE('',#8035,#8200,#4987,.T.);
#10302=EDGE_CURVE('',#8037,#8201,#1022,.T.);
#10303=EDGE_CURVE('',#8036,#8202,#4988,.T.);
#10304=EDGE_CURVE('',#8201,#8202,#446,.T.);
#10305=EDGE_CURVE('',#8202,#8200,#4989,.T.);
#10306=EDGE_CURVE('',#8203,#8201,#6801,.T.);
#10307=EDGE_CURVE('',#8203,#8038,#1023,.T.);
#10308=EDGE_CURVE('',#8204,#8203,#447,.T.);
#10309=EDGE_CURVE('',#8039,#8204,#4990,.T.);
#10310=EDGE_CURVE('',#8041,#8205,#1024,.T.);
#10311=EDGE_CURVE('',#8040,#8206,#4991,.T.);
#10312=EDGE_CURVE('',#8205,#8206,#448,.T.);
#10313=EDGE_CURVE('',#8206,#8204,#4992,.T.);
#10314=EDGE_CURVE('',#8207,#8205,#6802,.T.);
#10315=EDGE_CURVE('',#8207,#8042,#1025,.T.);
#10316=EDGE_CURVE('',#8208,#8207,#449,.T.);
#10317=EDGE_CURVE('',#8043,#8208,#4993,.T.);
#10318=EDGE_CURVE('',#8045,#8209,#1026,.T.);
#10319=EDGE_CURVE('',#8044,#8210,#4994,.T.);
#10320=EDGE_CURVE('',#8209,#8210,#450,.T.);
#10321=EDGE_CURVE('',#8210,#8208,#4995,.T.);
#10322=EDGE_CURVE('',#8211,#8209,#6803,.T.);
#10323=EDGE_CURVE('',#8211,#8046,#1027,.T.);
#10324=EDGE_CURVE('',#8212,#8211,#451,.T.);
#10325=EDGE_CURVE('',#8047,#8212,#4996,.T.);
#10326=EDGE_CURVE('',#8049,#8213,#1028,.T.);
#10327=EDGE_CURVE('',#8048,#8214,#4997,.T.);
#10328=EDGE_CURVE('',#8213,#8214,#452,.T.);
#10329=EDGE_CURVE('',#8214,#8212,#4998,.T.);
#10330=EDGE_CURVE('',#8215,#8213,#6804,.T.);
#10331=EDGE_CURVE('',#8215,#8050,#1029,.T.);
#10332=EDGE_CURVE('',#8216,#8215,#453,.T.);
#10333=EDGE_CURVE('',#8051,#8216,#4999,.T.);
#10334=EDGE_CURVE('',#8053,#8217,#1030,.T.);
#10335=EDGE_CURVE('',#8052,#8218,#5000,.T.);
#10336=EDGE_CURVE('',#8217,#8218,#454,.T.);
#10337=EDGE_CURVE('',#8218,#8216,#5001,.T.);
#10338=EDGE_CURVE('',#8219,#8217,#6805,.T.);
#10339=EDGE_CURVE('',#8219,#8054,#1031,.T.);
#10340=EDGE_CURVE('',#8220,#8219,#455,.T.);
#10341=EDGE_CURVE('',#8055,#8220,#5002,.T.);
#10342=EDGE_CURVE('',#8057,#8221,#1032,.T.);
#10343=EDGE_CURVE('',#8056,#8222,#5003,.T.);
#10344=EDGE_CURVE('',#8221,#8222,#456,.T.);
#10345=EDGE_CURVE('',#8222,#8220,#5004,.T.);
#10346=EDGE_CURVE('',#8223,#8221,#6806,.T.);
#10347=EDGE_CURVE('',#8223,#8058,#1033,.T.);
#10348=EDGE_CURVE('',#8224,#8223,#457,.T.);
#10349=EDGE_CURVE('',#8059,#8224,#5005,.T.);
#10350=EDGE_CURVE('',#8061,#8225,#1034,.T.);
#10351=EDGE_CURVE('',#8060,#8226,#5006,.T.);
#10352=EDGE_CURVE('',#8225,#8226,#458,.T.);
#10353=EDGE_CURVE('',#8226,#8224,#5007,.T.);
#10354=EDGE_CURVE('',#8227,#8225,#6807,.T.);
#10355=EDGE_CURVE('',#8227,#8062,#1035,.T.);
#10356=EDGE_CURVE('',#8228,#8227,#459,.T.);
#10357=EDGE_CURVE('',#8063,#8228,#5008,.T.);
#10358=EDGE_CURVE('',#8065,#8229,#1036,.T.);
#10359=EDGE_CURVE('',#8064,#8230,#5009,.T.);
#10360=EDGE_CURVE('',#8229,#8230,#460,.T.);
#10361=EDGE_CURVE('',#8230,#8228,#5010,.T.);
#10362=EDGE_CURVE('',#8231,#8229,#6808,.T.);
#10363=EDGE_CURVE('',#8231,#8066,#1037,.T.);
#10364=EDGE_CURVE('',#8232,#8231,#461,.T.);
#10365=EDGE_CURVE('',#8067,#8232,#5011,.T.);
#10366=EDGE_CURVE('',#8069,#8233,#1038,.T.);
#10367=EDGE_CURVE('',#8068,#8234,#5012,.T.);
#10368=EDGE_CURVE('',#8233,#8234,#462,.T.);
#10369=EDGE_CURVE('',#8234,#8232,#5013,.T.);
#10370=EDGE_CURVE('',#8235,#8233,#6809,.T.);
#10371=EDGE_CURVE('',#8235,#8070,#1039,.T.);
#10372=EDGE_CURVE('',#8236,#8235,#463,.T.);
#10373=EDGE_CURVE('',#8071,#8236,#5014,.T.);
#10374=EDGE_CURVE('',#8073,#8237,#1040,.T.);
#10375=EDGE_CURVE('',#8072,#8238,#5015,.T.);
#10376=EDGE_CURVE('',#8237,#8238,#464,.T.);
#10377=EDGE_CURVE('',#8238,#8236,#5016,.T.);
#10378=EDGE_CURVE('',#8239,#8237,#6810,.T.);
#10379=EDGE_CURVE('',#8239,#8074,#1041,.T.);
#10380=EDGE_CURVE('',#8240,#8239,#465,.T.);
#10381=EDGE_CURVE('',#8075,#8240,#5017,.T.);
#10382=EDGE_CURVE('',#8077,#8241,#1042,.T.);
#10383=EDGE_CURVE('',#8076,#8242,#5018,.T.);
#10384=EDGE_CURVE('',#8241,#8242,#466,.T.);
#10385=EDGE_CURVE('',#8242,#8240,#5019,.T.);
#10386=EDGE_CURVE('',#8243,#8241,#6811,.T.);
#10387=EDGE_CURVE('',#8243,#8078,#1043,.T.);
#10388=EDGE_CURVE('',#8244,#8243,#467,.T.);
#10389=EDGE_CURVE('',#8079,#8244,#5020,.T.);
#10390=EDGE_CURVE('',#8081,#8245,#1044,.T.);
#10391=EDGE_CURVE('',#8080,#8246,#5021,.T.);
#10392=EDGE_CURVE('',#8245,#8246,#468,.T.);
#10393=EDGE_CURVE('',#8246,#8244,#5022,.T.);
#10394=EDGE_CURVE('',#8247,#8245,#6812,.T.);
#10395=EDGE_CURVE('',#8247,#8082,#1045,.T.);
#10396=EDGE_CURVE('',#8248,#8247,#469,.T.);
#10397=EDGE_CURVE('',#8083,#8248,#5023,.T.);
#10398=EDGE_CURVE('',#8085,#8249,#1046,.T.);
#10399=EDGE_CURVE('',#8084,#8250,#5024,.T.);
#10400=EDGE_CURVE('',#8249,#8250,#470,.T.);
#10401=EDGE_CURVE('',#8250,#8248,#5025,.T.);
#10402=EDGE_CURVE('',#8251,#8249,#6813,.T.);
#10403=EDGE_CURVE('',#8251,#8086,#1047,.T.);
#10404=EDGE_CURVE('',#8252,#8251,#471,.T.);
#10405=EDGE_CURVE('',#8087,#8252,#5026,.T.);
#10406=EDGE_CURVE('',#8089,#8253,#1048,.T.);
#10407=EDGE_CURVE('',#8088,#8254,#5027,.T.);
#10408=EDGE_CURVE('',#8253,#8254,#472,.T.);
#10409=EDGE_CURVE('',#8254,#8252,#5028,.T.);
#10410=EDGE_CURVE('',#8255,#8253,#6814,.T.);
#10411=EDGE_CURVE('',#8255,#8090,#1049,.T.);
#10412=EDGE_CURVE('',#8256,#8255,#473,.T.);
#10413=EDGE_CURVE('',#8091,#8256,#5029,.T.);
#10414=EDGE_CURVE('',#8093,#8257,#1050,.T.);
#10415=EDGE_CURVE('',#8092,#8258,#5030,.T.);
#10416=EDGE_CURVE('',#8257,#8258,#474,.T.);
#10417=EDGE_CURVE('',#8258,#8256,#5031,.T.);
#10418=EDGE_CURVE('',#8259,#8257,#6815,.T.);
#10419=EDGE_CURVE('',#8259,#8094,#1051,.T.);
#10420=EDGE_CURVE('',#8260,#8259,#475,.T.);
#10421=EDGE_CURVE('',#8095,#8260,#5032,.T.);
#10422=EDGE_CURVE('',#8097,#8261,#1052,.T.);
#10423=EDGE_CURVE('',#8096,#8262,#5033,.T.);
#10424=EDGE_CURVE('',#8261,#8262,#476,.T.);
#10425=EDGE_CURVE('',#8262,#8260,#5034,.T.);
#10426=EDGE_CURVE('',#8263,#8261,#6816,.T.);
#10427=EDGE_CURVE('',#8263,#8098,#1053,.T.);
#10428=EDGE_CURVE('',#8264,#8263,#477,.T.);
#10429=EDGE_CURVE('',#8099,#8264,#5035,.T.);
#10430=EDGE_CURVE('',#8101,#8265,#1054,.T.);
#10431=EDGE_CURVE('',#8100,#8266,#5036,.T.);
#10432=EDGE_CURVE('',#8265,#8266,#478,.T.);
#10433=EDGE_CURVE('',#8266,#8264,#5037,.T.);
#10434=EDGE_CURVE('',#8267,#8265,#6817,.T.);
#10435=EDGE_CURVE('',#8267,#8102,#1055,.T.);
#10436=EDGE_CURVE('',#8268,#8267,#479,.T.);
#10437=EDGE_CURVE('',#8103,#8268,#5038,.T.);
#10438=EDGE_CURVE('',#8105,#8269,#1056,.T.);
#10439=EDGE_CURVE('',#8104,#8270,#5039,.T.);
#10440=EDGE_CURVE('',#8269,#8270,#480,.T.);
#10441=EDGE_CURVE('',#8270,#8268,#5040,.T.);
#10442=EDGE_CURVE('',#8271,#8269,#6818,.T.);
#10443=EDGE_CURVE('',#8271,#8106,#1057,.T.);
#10444=EDGE_CURVE('',#8272,#8271,#481,.T.);
#10445=EDGE_CURVE('',#8107,#8272,#5041,.T.);
#10446=EDGE_CURVE('',#8109,#8273,#1058,.T.);
#10447=EDGE_CURVE('',#8108,#8274,#5042,.T.);
#10448=EDGE_CURVE('',#8273,#8274,#482,.T.);
#10449=EDGE_CURVE('',#8274,#8272,#5043,.T.);
#10450=EDGE_CURVE('',#8275,#8273,#6819,.T.);
#10451=EDGE_CURVE('',#8275,#8110,#1059,.T.);
#10452=EDGE_CURVE('',#8276,#8275,#483,.T.);
#10453=EDGE_CURVE('',#8111,#8276,#5044,.T.);
#10454=EDGE_CURVE('',#8113,#8277,#1060,.T.);
#10455=EDGE_CURVE('',#8112,#8278,#5045,.T.);
#10456=EDGE_CURVE('',#8277,#8278,#484,.T.);
#10457=EDGE_CURVE('',#8278,#8276,#5046,.T.);
#10458=EDGE_CURVE('',#8279,#8277,#6820,.T.);
#10459=EDGE_CURVE('',#8279,#8114,#1061,.T.);
#10460=EDGE_CURVE('',#8280,#8279,#485,.T.);
#10461=EDGE_CURVE('',#8115,#8280,#5047,.T.);
#10462=EDGE_CURVE('',#8117,#8281,#1062,.T.);
#10463=EDGE_CURVE('',#8116,#8282,#5048,.T.);
#10464=EDGE_CURVE('',#8281,#8282,#486,.T.);
#10465=EDGE_CURVE('',#8282,#8280,#5049,.T.);
#10466=EDGE_CURVE('',#8283,#8281,#6821,.T.);
#10467=EDGE_CURVE('',#8283,#8118,#1063,.T.);
#10468=EDGE_CURVE('',#8284,#8283,#487,.T.);
#10469=EDGE_CURVE('',#8119,#8284,#5050,.T.);
#10470=EDGE_CURVE('',#8285,#8284,#5051,.T.);
#10471=EDGE_CURVE('',#8120,#8285,#5052,.T.);
#10472=EDGE_CURVE('',#8121,#8286,#1064,.T.);
#10473=EDGE_CURVE('',#8286,#8285,#488,.T.);
#10474=EDGE_CURVE('',#8287,#8286,#6822,.T.);
#10475=EDGE_CURVE('',#8287,#8122,#1065,.T.);
#10476=EDGE_CURVE('',#8125,#8288,#1066,.T.);
#10477=EDGE_CURVE('',#8124,#8289,#5053,.T.);
#10478=EDGE_CURVE('',#8288,#8289,#489,.T.);
#10479=EDGE_CURVE('',#8290,#8287,#490,.T.);
#10480=EDGE_CURVE('',#8123,#8290,#5054,.T.);
#10481=EDGE_CURVE('',#8289,#8290,#5055,.T.);
#10482=EDGE_CURVE('',#8131,#8288,#6823,.T.);
#13869=ORIENTED_EDGE('',*,*,#9988,.F.);
#13870=ORIENTED_EDGE('',*,*,#9989,.F.);
#13871=ORIENTED_EDGE('',*,*,#9990,.F.);
#13872=ORIENTED_EDGE('',*,*,#9991,.F.);
#13873=ORIENTED_EDGE('',*,*,#9992,.F.);
#13874=ORIENTED_EDGE('',*,*,#9993,.T.);
#13875=ORIENTED_EDGE('',*,*,#9994,.F.);
#13876=ORIENTED_EDGE('',*,*,#9989,.T.);
#13877=ORIENTED_EDGE('',*,*,#9995,.F.);
#13878=ORIENTED_EDGE('',*,*,#9996,.F.);
#13879=ORIENTED_EDGE('',*,*,#9997,.F.);
#13880=ORIENTED_EDGE('',*,*,#9993,.F.);
#13881=ORIENTED_EDGE('',*,*,#9998,.T.);
#13882=ORIENTED_EDGE('',*,*,#9999,.T.);
#13883=ORIENTED_EDGE('',*,*,#10000,.T.);
#13884=ORIENTED_EDGE('',*,*,#10001,.T.);
#13885=ORIENTED_EDGE('',*,*,#10002,.T.);
#13886=ORIENTED_EDGE('',*,*,#10003,.T.);
#13887=ORIENTED_EDGE('',*,*,#10004,.T.);
#13888=ORIENTED_EDGE('',*,*,#10005,.T.);
#13889=ORIENTED_EDGE('',*,*,#10006,.T.);
#13890=ORIENTED_EDGE('',*,*,#10007,.T.);
#13891=ORIENTED_EDGE('',*,*,#10008,.T.);
#13892=ORIENTED_EDGE('',*,*,#10009,.T.);
#13893=ORIENTED_EDGE('',*,*,#10010,.T.);
#13894=ORIENTED_EDGE('',*,*,#10011,.T.);
#13895=ORIENTED_EDGE('',*,*,#10012,.T.);
#13896=ORIENTED_EDGE('',*,*,#10013,.T.);
#13897=ORIENTED_EDGE('',*,*,#10014,.T.);
#13898=ORIENTED_EDGE('',*,*,#10015,.T.);
#13899=ORIENTED_EDGE('',*,*,#10016,.T.);
#13900=ORIENTED_EDGE('',*,*,#10017,.T.);
#13901=ORIENTED_EDGE('',*,*,#10018,.T.);
#13902=ORIENTED_EDGE('',*,*,#10019,.T.);
#13903=ORIENTED_EDGE('',*,*,#10020,.T.);
#13904=ORIENTED_EDGE('',*,*,#10021,.T.);
#13905=ORIENTED_EDGE('',*,*,#10022,.T.);
#13906=ORIENTED_EDGE('',*,*,#10023,.T.);
#13907=ORIENTED_EDGE('',*,*,#10024,.T.);
#13908=ORIENTED_EDGE('',*,*,#10025,.T.);
#13909=ORIENTED_EDGE('',*,*,#10026,.T.);
#13910=ORIENTED_EDGE('',*,*,#10027,.T.);
#13911=ORIENTED_EDGE('',*,*,#10028,.T.);
#13912=ORIENTED_EDGE('',*,*,#10029,.T.);
#13913=ORIENTED_EDGE('',*,*,#10030,.T.);
#13914=ORIENTED_EDGE('',*,*,#10031,.T.);
#13915=ORIENTED_EDGE('',*,*,#10032,.T.);
#13916=ORIENTED_EDGE('',*,*,#10033,.T.);
#13917=ORIENTED_EDGE('',*,*,#10034,.T.);
#13918=ORIENTED_EDGE('',*,*,#10035,.T.);
#13919=ORIENTED_EDGE('',*,*,#10036,.T.);
#13920=ORIENTED_EDGE('',*,*,#10037,.T.);
#13921=ORIENTED_EDGE('',*,*,#10038,.T.);
#13922=ORIENTED_EDGE('',*,*,#10039,.T.);
#13923=ORIENTED_EDGE('',*,*,#10040,.T.);
#13924=ORIENTED_EDGE('',*,*,#10041,.T.);
#13925=ORIENTED_EDGE('',*,*,#10042,.T.);
#13926=ORIENTED_EDGE('',*,*,#10043,.T.);
#13927=ORIENTED_EDGE('',*,*,#10044,.T.);
#13928=ORIENTED_EDGE('',*,*,#10045,.T.);
#13929=ORIENTED_EDGE('',*,*,#10046,.T.);
#13930=ORIENTED_EDGE('',*,*,#10047,.T.);
#13931=ORIENTED_EDGE('',*,*,#10048,.T.);
#13932=ORIENTED_EDGE('',*,*,#10049,.T.);
#13933=ORIENTED_EDGE('',*,*,#10050,.T.);
#13934=ORIENTED_EDGE('',*,*,#10051,.T.);
#13935=ORIENTED_EDGE('',*,*,#10052,.T.);
#13936=ORIENTED_EDGE('',*,*,#10053,.T.);
#13937=ORIENTED_EDGE('',*,*,#10054,.T.);
#13938=ORIENTED_EDGE('',*,*,#10055,.T.);
#13939=ORIENTED_EDGE('',*,*,#10056,.T.);
#13940=ORIENTED_EDGE('',*,*,#10057,.T.);
#13941=ORIENTED_EDGE('',*,*,#10058,.T.);
#13942=ORIENTED_EDGE('',*,*,#10059,.T.);
#13943=ORIENTED_EDGE('',*,*,#10060,.T.);
#13944=ORIENTED_EDGE('',*,*,#10061,.T.);
#13945=ORIENTED_EDGE('',*,*,#10062,.T.);
#13946=ORIENTED_EDGE('',*,*,#10063,.T.);
#13947=ORIENTED_EDGE('',*,*,#10064,.T.);
#13948=ORIENTED_EDGE('',*,*,#10065,.T.);
#13949=ORIENTED_EDGE('',*,*,#10066,.T.);
#13950=ORIENTED_EDGE('',*,*,#10067,.T.);
#13951=ORIENTED_EDGE('',*,*,#10068,.T.);
#13952=ORIENTED_EDGE('',*,*,#10069,.T.);
#13953=ORIENTED_EDGE('',*,*,#10070,.T.);
#13954=ORIENTED_EDGE('',*,*,#10071,.T.);
#13955=ORIENTED_EDGE('',*,*,#10072,.T.);
#13956=ORIENTED_EDGE('',*,*,#10073,.T.);
#13957=ORIENTED_EDGE('',*,*,#10074,.T.);
#13958=ORIENTED_EDGE('',*,*,#10075,.T.);
#13959=ORIENTED_EDGE('',*,*,#10076,.T.);
#13960=ORIENTED_EDGE('',*,*,#10077,.T.);
#13961=ORIENTED_EDGE('',*,*,#10078,.T.);
#13962=ORIENTED_EDGE('',*,*,#10079,.T.);
#13963=ORIENTED_EDGE('',*,*,#10080,.T.);
#13964=ORIENTED_EDGE('',*,*,#10081,.T.);
#13965=ORIENTED_EDGE('',*,*,#10082,.T.);
#13966=ORIENTED_EDGE('',*,*,#10083,.T.);
#13967=ORIENTED_EDGE('',*,*,#10084,.T.);
#13968=ORIENTED_EDGE('',*,*,#10085,.T.);
#13969=ORIENTED_EDGE('',*,*,#10086,.T.);
#13970=ORIENTED_EDGE('',*,*,#10087,.T.);
#13971=ORIENTED_EDGE('',*,*,#10088,.T.);
#13972=ORIENTED_EDGE('',*,*,#10089,.T.);
#13973=ORIENTED_EDGE('',*,*,#10090,.T.);
#13974=ORIENTED_EDGE('',*,*,#10091,.T.);
#13975=ORIENTED_EDGE('',*,*,#10092,.T.);
#13976=ORIENTED_EDGE('',*,*,#10093,.T.);
#13977=ORIENTED_EDGE('',*,*,#10094,.T.);
#13978=ORIENTED_EDGE('',*,*,#10095,.T.);
#13979=ORIENTED_EDGE('',*,*,#10096,.T.);
#13980=ORIENTED_EDGE('',*,*,#10097,.T.);
#13981=ORIENTED_EDGE('',*,*,#10098,.T.);
#13982=ORIENTED_EDGE('',*,*,#10099,.T.);
#13983=ORIENTED_EDGE('',*,*,#10100,.T.);
#13984=ORIENTED_EDGE('',*,*,#10101,.T.);
#13985=ORIENTED_EDGE('',*,*,#10102,.T.);
#13986=ORIENTED_EDGE('',*,*,#10103,.T.);
#13987=ORIENTED_EDGE('',*,*,#10104,.T.);
#13988=ORIENTED_EDGE('',*,*,#10105,.T.);
#13989=ORIENTED_EDGE('',*,*,#10106,.T.);
#13990=ORIENTED_EDGE('',*,*,#10107,.T.);
#13991=ORIENTED_EDGE('',*,*,#10108,.T.);
#13992=ORIENTED_EDGE('',*,*,#10109,.T.);
#13993=ORIENTED_EDGE('',*,*,#10110,.T.);
#13994=ORIENTED_EDGE('',*,*,#10111,.T.);
#13995=ORIENTED_EDGE('',*,*,#10112,.T.);
#13996=ORIENTED_EDGE('',*,*,#10113,.T.);
#13997=ORIENTED_EDGE('',*,*,#10114,.T.);
#13998=ORIENTED_EDGE('',*,*,#10115,.T.);
#13999=ORIENTED_EDGE('',*,*,#10116,.T.);
#14000=ORIENTED_EDGE('',*,*,#10117,.T.);
#14001=ORIENTED_EDGE('',*,*,#10118,.T.);
#14002=ORIENTED_EDGE('',*,*,#10119,.T.);
#14003=ORIENTED_EDGE('',*,*,#10120,.T.);
#14004=ORIENTED_EDGE('',*,*,#10121,.T.);
#14005=ORIENTED_EDGE('',*,*,#10122,.T.);
#14006=ORIENTED_EDGE('',*,*,#10123,.T.);
#14007=ORIENTED_EDGE('',*,*,#10124,.T.);
#14008=ORIENTED_EDGE('',*,*,#10125,.T.);
#14009=ORIENTED_EDGE('',*,*,#10126,.T.);
#14010=ORIENTED_EDGE('',*,*,#10127,.T.);
#14011=ORIENTED_EDGE('',*,*,#10128,.T.);
#14012=ORIENTED_EDGE('',*,*,#10129,.T.);
#14013=ORIENTED_EDGE('',*,*,#10130,.T.);
#14014=ORIENTED_EDGE('',*,*,#10131,.T.);
#14015=ORIENTED_EDGE('',*,*,#10132,.T.);
#14016=ORIENTED_EDGE('',*,*,#10133,.T.);
#14017=ORIENTED_EDGE('',*,*,#10134,.T.);
#14018=ORIENTED_EDGE('',*,*,#10135,.T.);
#14019=ORIENTED_EDGE('',*,*,#10136,.T.);
#14020=ORIENTED_EDGE('',*,*,#10137,.T.);
#14021=ORIENTED_EDGE('',*,*,#10138,.T.);
#14022=ORIENTED_EDGE('',*,*,#10139,.T.);
#14023=ORIENTED_EDGE('',*,*,#10140,.T.);
#14024=ORIENTED_EDGE('',*,*,#10141,.T.);
#14025=ORIENTED_EDGE('',*,*,#10142,.T.);
#14026=ORIENTED_EDGE('',*,*,#10143,.T.);
#14027=ORIENTED_EDGE('',*,*,#10144,.T.);
#14028=ORIENTED_EDGE('',*,*,#10145,.T.);
#14029=ORIENTED_EDGE('',*,*,#10146,.T.);
#14030=ORIENTED_EDGE('',*,*,#10147,.T.);
#14031=ORIENTED_EDGE('',*,*,#10148,.T.);
#14032=ORIENTED_EDGE('',*,*,#10149,.T.);
#14033=ORIENTED_EDGE('',*,*,#10150,.T.);
#14034=ORIENTED_EDGE('',*,*,#10151,.T.);
#14035=ORIENTED_EDGE('',*,*,#10152,.T.);
#14036=ORIENTED_EDGE('',*,*,#10153,.T.);
#14037=ORIENTED_EDGE('',*,*,#10154,.T.);
#14038=ORIENTED_EDGE('',*,*,#10155,.T.);
#14039=ORIENTED_EDGE('',*,*,#10156,.T.);
#14040=ORIENTED_EDGE('',*,*,#10157,.T.);
#14041=ORIENTED_EDGE('',*,*,#9990,.T.);
#14042=ORIENTED_EDGE('',*,*,#9994,.T.);
#14043=ORIENTED_EDGE('',*,*,#9997,.T.);
#14044=ORIENTED_EDGE('',*,*,#10158,.T.);
#14045=ORIENTED_EDGE('',*,*,#9991,.T.);
#14046=ORIENTED_EDGE('',*,*,#10158,.F.);
#14047=ORIENTED_EDGE('',*,*,#9996,.T.);
#14048=ORIENTED_EDGE('',*,*,#10159,.F.);
#14049=ORIENTED_EDGE('',*,*,#10160,.F.);
#14050=ORIENTED_EDGE('',*,*,#10161,.T.);
#14051=ORIENTED_EDGE('',*,*,#10162,.F.);
#14052=ORIENTED_EDGE('',*,*,#10161,.F.);
#14053=ORIENTED_EDGE('',*,*,#10160,.T.);
#14054=ORIENTED_EDGE('',*,*,#9988,.T.);
#14055=ORIENTED_EDGE('',*,*,#10159,.T.);
#14056=ORIENTED_EDGE('',*,*,#9995,.T.);
#14057=ORIENTED_EDGE('',*,*,#9992,.T.);
#14058=ORIENTED_EDGE('',*,*,#10163,.F.);
#14059=ORIENTED_EDGE('',*,*,#10164,.F.);
#14060=ORIENTED_EDGE('',*,*,#10165,.F.);
#14061=ORIENTED_EDGE('',*,*,#10155,.F.);
#14062=ORIENTED_EDGE('',*,*,#10166,.F.);
#14063=ORIENTED_EDGE('',*,*,#10157,.F.);
#14064=ORIENTED_EDGE('',*,*,#10167,.T.);
#14065=ORIENTED_EDGE('',*,*,#10168,.F.);
#14066=ORIENTED_EDGE('',*,*,#10165,.T.);
#14067=ORIENTED_EDGE('',*,*,#10169,.F.);
#14068=ORIENTED_EDGE('',*,*,#10167,.F.);
#14069=ORIENTED_EDGE('',*,*,#10156,.F.);
#14070=ORIENTED_EDGE('',*,*,#10166,.T.);
#14071=ORIENTED_EDGE('',*,*,#10170,.F.);
#14072=ORIENTED_EDGE('',*,*,#10171,.T.);
#14073=ORIENTED_EDGE('',*,*,#9998,.F.);
#14074=ORIENTED_EDGE('',*,*,#10171,.F.);
#14075=ORIENTED_EDGE('',*,*,#10172,.F.);
#14076=ORIENTED_EDGE('',*,*,#10173,.F.);
#14077=ORIENTED_EDGE('',*,*,#9999,.F.);
#14078=ORIENTED_EDGE('',*,*,#10174,.F.);
#14079=ORIENTED_EDGE('',*,*,#10001,.F.);
#14080=ORIENTED_EDGE('',*,*,#10175,.T.);
#14081=ORIENTED_EDGE('',*,*,#10176,.F.);
#14082=ORIENTED_EDGE('',*,*,#10173,.T.);
#14083=ORIENTED_EDGE('',*,*,#10177,.F.);
#14084=ORIENTED_EDGE('',*,*,#10175,.F.);
#14085=ORIENTED_EDGE('',*,*,#10000,.F.);
#14086=ORIENTED_EDGE('',*,*,#10174,.T.);
#14087=ORIENTED_EDGE('',*,*,#10178,.F.);
#14088=ORIENTED_EDGE('',*,*,#10179,.T.);
#14089=ORIENTED_EDGE('',*,*,#10002,.F.);
#14090=ORIENTED_EDGE('',*,*,#10179,.F.);
#14091=ORIENTED_EDGE('',*,*,#10180,.F.);
#14092=ORIENTED_EDGE('',*,*,#10181,.F.);
#14093=ORIENTED_EDGE('',*,*,#10003,.F.);
#14094=ORIENTED_EDGE('',*,*,#10182,.F.);
#14095=ORIENTED_EDGE('',*,*,#10005,.F.);
#14096=ORIENTED_EDGE('',*,*,#10183,.T.);
#14097=ORIENTED_EDGE('',*,*,#10184,.F.);
#14098=ORIENTED_EDGE('',*,*,#10181,.T.);
#14099=ORIENTED_EDGE('',*,*,#10185,.F.);
#14100=ORIENTED_EDGE('',*,*,#10183,.F.);
#14101=ORIENTED_EDGE('',*,*,#10004,.F.);
#14102=ORIENTED_EDGE('',*,*,#10182,.T.);
#14103=ORIENTED_EDGE('',*,*,#10186,.F.);
#14104=ORIENTED_EDGE('',*,*,#10187,.T.);
#14105=ORIENTED_EDGE('',*,*,#10006,.F.);
#14106=ORIENTED_EDGE('',*,*,#10187,.F.);
#14107=ORIENTED_EDGE('',*,*,#10188,.F.);
#14108=ORIENTED_EDGE('',*,*,#10189,.F.);
#14109=ORIENTED_EDGE('',*,*,#10007,.F.);
#14110=ORIENTED_EDGE('',*,*,#10190,.F.);
#14111=ORIENTED_EDGE('',*,*,#10009,.F.);
#14112=ORIENTED_EDGE('',*,*,#10191,.T.);
#14113=ORIENTED_EDGE('',*,*,#10192,.F.);
#14114=ORIENTED_EDGE('',*,*,#10189,.T.);
#14115=ORIENTED_EDGE('',*,*,#10193,.F.);
#14116=ORIENTED_EDGE('',*,*,#10191,.F.);
#14117=ORIENTED_EDGE('',*,*,#10008,.F.);
#14118=ORIENTED_EDGE('',*,*,#10190,.T.);
#14119=ORIENTED_EDGE('',*,*,#10194,.F.);
#14120=ORIENTED_EDGE('',*,*,#10195,.T.);
#14121=ORIENTED_EDGE('',*,*,#10010,.F.);
#14122=ORIENTED_EDGE('',*,*,#10195,.F.);
#14123=ORIENTED_EDGE('',*,*,#10196,.F.);
#14124=ORIENTED_EDGE('',*,*,#10197,.F.);
#14125=ORIENTED_EDGE('',*,*,#10011,.F.);
#14126=ORIENTED_EDGE('',*,*,#10198,.F.);
#14127=ORIENTED_EDGE('',*,*,#10013,.F.);
#14128=ORIENTED_EDGE('',*,*,#10199,.T.);
#14129=ORIENTED_EDGE('',*,*,#10200,.F.);
#14130=ORIENTED_EDGE('',*,*,#10197,.T.);
#14131=ORIENTED_EDGE('',*,*,#10201,.F.);
#14132=ORIENTED_EDGE('',*,*,#10199,.F.);
#14133=ORIENTED_EDGE('',*,*,#10012,.F.);
#14134=ORIENTED_EDGE('',*,*,#10198,.T.);
#14135=ORIENTED_EDGE('',*,*,#10202,.F.);
#14136=ORIENTED_EDGE('',*,*,#10203,.T.);
#14137=ORIENTED_EDGE('',*,*,#10014,.F.);
#14138=ORIENTED_EDGE('',*,*,#10203,.F.);
#14139=ORIENTED_EDGE('',*,*,#10204,.F.);
#14140=ORIENTED_EDGE('',*,*,#10205,.F.);
#14141=ORIENTED_EDGE('',*,*,#10015,.F.);
#14142=ORIENTED_EDGE('',*,*,#10206,.F.);
#14143=ORIENTED_EDGE('',*,*,#10017,.F.);
#14144=ORIENTED_EDGE('',*,*,#10207,.T.);
#14145=ORIENTED_EDGE('',*,*,#10208,.F.);
#14146=ORIENTED_EDGE('',*,*,#10205,.T.);
#14147=ORIENTED_EDGE('',*,*,#10209,.F.);
#14148=ORIENTED_EDGE('',*,*,#10207,.F.);
#14149=ORIENTED_EDGE('',*,*,#10016,.F.);
#14150=ORIENTED_EDGE('',*,*,#10206,.T.);
#14151=ORIENTED_EDGE('',*,*,#10210,.F.);
#14152=ORIENTED_EDGE('',*,*,#10211,.T.);
#14153=ORIENTED_EDGE('',*,*,#10018,.F.);
#14154=ORIENTED_EDGE('',*,*,#10211,.F.);
#14155=ORIENTED_EDGE('',*,*,#10212,.F.);
#14156=ORIENTED_EDGE('',*,*,#10213,.F.);
#14157=ORIENTED_EDGE('',*,*,#10019,.F.);
#14158=ORIENTED_EDGE('',*,*,#10214,.F.);
#14159=ORIENTED_EDGE('',*,*,#10021,.F.);
#14160=ORIENTED_EDGE('',*,*,#10215,.T.);
#14161=ORIENTED_EDGE('',*,*,#10216,.F.);
#14162=ORIENTED_EDGE('',*,*,#10213,.T.);
#14163=ORIENTED_EDGE('',*,*,#10217,.F.);
#14164=ORIENTED_EDGE('',*,*,#10215,.F.);
#14165=ORIENTED_EDGE('',*,*,#10020,.F.);
#14166=ORIENTED_EDGE('',*,*,#10214,.T.);
#14167=ORIENTED_EDGE('',*,*,#10218,.F.);
#14168=ORIENTED_EDGE('',*,*,#10219,.T.);
#14169=ORIENTED_EDGE('',*,*,#10022,.F.);
#14170=ORIENTED_EDGE('',*,*,#10219,.F.);
#14171=ORIENTED_EDGE('',*,*,#10220,.F.);
#14172=ORIENTED_EDGE('',*,*,#10221,.F.);
#14173=ORIENTED_EDGE('',*,*,#10023,.F.);
#14174=ORIENTED_EDGE('',*,*,#10222,.F.);
#14175=ORIENTED_EDGE('',*,*,#10025,.F.);
#14176=ORIENTED_EDGE('',*,*,#10223,.T.);
#14177=ORIENTED_EDGE('',*,*,#10224,.F.);
#14178=ORIENTED_EDGE('',*,*,#10221,.T.);
#14179=ORIENTED_EDGE('',*,*,#10225,.F.);
#14180=ORIENTED_EDGE('',*,*,#10223,.F.);
#14181=ORIENTED_EDGE('',*,*,#10024,.F.);
#14182=ORIENTED_EDGE('',*,*,#10222,.T.);
#14183=ORIENTED_EDGE('',*,*,#10226,.F.);
#14184=ORIENTED_EDGE('',*,*,#10227,.T.);
#14185=ORIENTED_EDGE('',*,*,#10026,.F.);
#14186=ORIENTED_EDGE('',*,*,#10227,.F.);
#14187=ORIENTED_EDGE('',*,*,#10228,.F.);
#14188=ORIENTED_EDGE('',*,*,#10229,.F.);
#14189=ORIENTED_EDGE('',*,*,#10027,.F.);
#14190=ORIENTED_EDGE('',*,*,#10230,.F.);
#14191=ORIENTED_EDGE('',*,*,#10029,.F.);
#14192=ORIENTED_EDGE('',*,*,#10231,.T.);
#14193=ORIENTED_EDGE('',*,*,#10232,.F.);
#14194=ORIENTED_EDGE('',*,*,#10229,.T.);
#14195=ORIENTED_EDGE('',*,*,#10233,.F.);
#14196=ORIENTED_EDGE('',*,*,#10231,.F.);
#14197=ORIENTED_EDGE('',*,*,#10028,.F.);
#14198=ORIENTED_EDGE('',*,*,#10230,.T.);
#14199=ORIENTED_EDGE('',*,*,#10234,.F.);
#14200=ORIENTED_EDGE('',*,*,#10235,.T.);
#14201=ORIENTED_EDGE('',*,*,#10030,.F.);
#14202=ORIENTED_EDGE('',*,*,#10235,.F.);
#14203=ORIENTED_EDGE('',*,*,#10236,.F.);
#14204=ORIENTED_EDGE('',*,*,#10237,.F.);
#14205=ORIENTED_EDGE('',*,*,#10031,.F.);
#14206=ORIENTED_EDGE('',*,*,#10238,.F.);
#14207=ORIENTED_EDGE('',*,*,#10033,.F.);
#14208=ORIENTED_EDGE('',*,*,#10239,.T.);
#14209=ORIENTED_EDGE('',*,*,#10240,.F.);
#14210=ORIENTED_EDGE('',*,*,#10237,.T.);
#14211=ORIENTED_EDGE('',*,*,#10241,.F.);
#14212=ORIENTED_EDGE('',*,*,#10239,.F.);
#14213=ORIENTED_EDGE('',*,*,#10032,.F.);
#14214=ORIENTED_EDGE('',*,*,#10238,.T.);
#14215=ORIENTED_EDGE('',*,*,#10242,.F.);
#14216=ORIENTED_EDGE('',*,*,#10243,.T.);
#14217=ORIENTED_EDGE('',*,*,#10034,.F.);
#14218=ORIENTED_EDGE('',*,*,#10243,.F.);
#14219=ORIENTED_EDGE('',*,*,#10244,.F.);
#14220=ORIENTED_EDGE('',*,*,#10245,.F.);
#14221=ORIENTED_EDGE('',*,*,#10035,.F.);
#14222=ORIENTED_EDGE('',*,*,#10246,.F.);
#14223=ORIENTED_EDGE('',*,*,#10037,.F.);
#14224=ORIENTED_EDGE('',*,*,#10247,.T.);
#14225=ORIENTED_EDGE('',*,*,#10248,.F.);
#14226=ORIENTED_EDGE('',*,*,#10245,.T.);
#14227=ORIENTED_EDGE('',*,*,#10249,.F.);
#14228=ORIENTED_EDGE('',*,*,#10247,.F.);
#14229=ORIENTED_EDGE('',*,*,#10036,.F.);
#14230=ORIENTED_EDGE('',*,*,#10246,.T.);
#14231=ORIENTED_EDGE('',*,*,#10250,.F.);
#14232=ORIENTED_EDGE('',*,*,#10251,.T.);
#14233=ORIENTED_EDGE('',*,*,#10038,.F.);
#14234=ORIENTED_EDGE('',*,*,#10251,.F.);
#14235=ORIENTED_EDGE('',*,*,#10252,.F.);
#14236=ORIENTED_EDGE('',*,*,#10253,.F.);
#14237=ORIENTED_EDGE('',*,*,#10039,.F.);
#14238=ORIENTED_EDGE('',*,*,#10254,.F.);
#14239=ORIENTED_EDGE('',*,*,#10041,.F.);
#14240=ORIENTED_EDGE('',*,*,#10255,.T.);
#14241=ORIENTED_EDGE('',*,*,#10256,.F.);
#14242=ORIENTED_EDGE('',*,*,#10253,.T.);
#14243=ORIENTED_EDGE('',*,*,#10257,.F.);
#14244=ORIENTED_EDGE('',*,*,#10255,.F.);
#14245=ORIENTED_EDGE('',*,*,#10040,.F.);
#14246=ORIENTED_EDGE('',*,*,#10254,.T.);
#14247=ORIENTED_EDGE('',*,*,#10258,.F.);
#14248=ORIENTED_EDGE('',*,*,#10259,.T.);
#14249=ORIENTED_EDGE('',*,*,#10042,.F.);
#14250=ORIENTED_EDGE('',*,*,#10259,.F.);
#14251=ORIENTED_EDGE('',*,*,#10260,.F.);
#14252=ORIENTED_EDGE('',*,*,#10261,.F.);
#14253=ORIENTED_EDGE('',*,*,#10043,.F.);
#14254=ORIENTED_EDGE('',*,*,#10262,.F.);
#14255=ORIENTED_EDGE('',*,*,#10045,.F.);
#14256=ORIENTED_EDGE('',*,*,#10263,.T.);
#14257=ORIENTED_EDGE('',*,*,#10264,.F.);
#14258=ORIENTED_EDGE('',*,*,#10261,.T.);
#14259=ORIENTED_EDGE('',*,*,#10265,.F.);
#14260=ORIENTED_EDGE('',*,*,#10263,.F.);
#14261=ORIENTED_EDGE('',*,*,#10044,.F.);
#14262=ORIENTED_EDGE('',*,*,#10262,.T.);
#14263=ORIENTED_EDGE('',*,*,#10266,.F.);
#14264=ORIENTED_EDGE('',*,*,#10267,.T.);
#14265=ORIENTED_EDGE('',*,*,#10046,.F.);
#14266=ORIENTED_EDGE('',*,*,#10267,.F.);
#14267=ORIENTED_EDGE('',*,*,#10268,.F.);
#14268=ORIENTED_EDGE('',*,*,#10269,.F.);
#14269=ORIENTED_EDGE('',*,*,#10047,.F.);
#14270=ORIENTED_EDGE('',*,*,#10270,.F.);
#14271=ORIENTED_EDGE('',*,*,#10049,.F.);
#14272=ORIENTED_EDGE('',*,*,#10271,.T.);
#14273=ORIENTED_EDGE('',*,*,#10272,.F.);
#14274=ORIENTED_EDGE('',*,*,#10269,.T.);
#14275=ORIENTED_EDGE('',*,*,#10273,.F.);
#14276=ORIENTED_EDGE('',*,*,#10271,.F.);
#14277=ORIENTED_EDGE('',*,*,#10048,.F.);
#14278=ORIENTED_EDGE('',*,*,#10270,.T.);
#14279=ORIENTED_EDGE('',*,*,#10274,.F.);
#14280=ORIENTED_EDGE('',*,*,#10275,.T.);
#14281=ORIENTED_EDGE('',*,*,#10050,.F.);
#14282=ORIENTED_EDGE('',*,*,#10275,.F.);
#14283=ORIENTED_EDGE('',*,*,#10276,.F.);
#14284=ORIENTED_EDGE('',*,*,#10277,.F.);
#14285=ORIENTED_EDGE('',*,*,#10051,.F.);
#14286=ORIENTED_EDGE('',*,*,#10278,.F.);
#14287=ORIENTED_EDGE('',*,*,#10053,.F.);
#14288=ORIENTED_EDGE('',*,*,#10279,.T.);
#14289=ORIENTED_EDGE('',*,*,#10280,.F.);
#14290=ORIENTED_EDGE('',*,*,#10277,.T.);
#14291=ORIENTED_EDGE('',*,*,#10281,.F.);
#14292=ORIENTED_EDGE('',*,*,#10279,.F.);
#14293=ORIENTED_EDGE('',*,*,#10052,.F.);
#14294=ORIENTED_EDGE('',*,*,#10278,.T.);
#14295=ORIENTED_EDGE('',*,*,#10282,.F.);
#14296=ORIENTED_EDGE('',*,*,#10283,.T.);
#14297=ORIENTED_EDGE('',*,*,#10054,.F.);
#14298=ORIENTED_EDGE('',*,*,#10283,.F.);
#14299=ORIENTED_EDGE('',*,*,#10284,.F.);
#14300=ORIENTED_EDGE('',*,*,#10285,.F.);
#14301=ORIENTED_EDGE('',*,*,#10055,.F.);
#14302=ORIENTED_EDGE('',*,*,#10286,.F.);
#14303=ORIENTED_EDGE('',*,*,#10057,.F.);
#14304=ORIENTED_EDGE('',*,*,#10287,.T.);
#14305=ORIENTED_EDGE('',*,*,#10288,.F.);
#14306=ORIENTED_EDGE('',*,*,#10285,.T.);
#14307=ORIENTED_EDGE('',*,*,#10289,.F.);
#14308=ORIENTED_EDGE('',*,*,#10287,.F.);
#14309=ORIENTED_EDGE('',*,*,#10056,.F.);
#14310=ORIENTED_EDGE('',*,*,#10286,.T.);
#14311=ORIENTED_EDGE('',*,*,#10290,.F.);
#14312=ORIENTED_EDGE('',*,*,#10291,.T.);
#14313=ORIENTED_EDGE('',*,*,#10058,.F.);
#14314=ORIENTED_EDGE('',*,*,#10291,.F.);
#14315=ORIENTED_EDGE('',*,*,#10292,.F.);
#14316=ORIENTED_EDGE('',*,*,#10293,.F.);
#14317=ORIENTED_EDGE('',*,*,#10059,.F.);
#14318=ORIENTED_EDGE('',*,*,#10294,.F.);
#14319=ORIENTED_EDGE('',*,*,#10061,.F.);
#14320=ORIENTED_EDGE('',*,*,#10295,.T.);
#14321=ORIENTED_EDGE('',*,*,#10296,.F.);
#14322=ORIENTED_EDGE('',*,*,#10293,.T.);
#14323=ORIENTED_EDGE('',*,*,#10297,.F.);
#14324=ORIENTED_EDGE('',*,*,#10295,.F.);
#14325=ORIENTED_EDGE('',*,*,#10060,.F.);
#14326=ORIENTED_EDGE('',*,*,#10294,.T.);
#14327=ORIENTED_EDGE('',*,*,#10298,.F.);
#14328=ORIENTED_EDGE('',*,*,#10299,.T.);
#14329=ORIENTED_EDGE('',*,*,#10062,.F.);
#14330=ORIENTED_EDGE('',*,*,#10299,.F.);
#14331=ORIENTED_EDGE('',*,*,#10300,.F.);
#14332=ORIENTED_EDGE('',*,*,#10301,.F.);
#14333=ORIENTED_EDGE('',*,*,#10063,.F.);
#14334=ORIENTED_EDGE('',*,*,#10302,.F.);
#14335=ORIENTED_EDGE('',*,*,#10065,.F.);
#14336=ORIENTED_EDGE('',*,*,#10303,.T.);
#14337=ORIENTED_EDGE('',*,*,#10304,.F.);
#14338=ORIENTED_EDGE('',*,*,#10301,.T.);
#14339=ORIENTED_EDGE('',*,*,#10305,.F.);
#14340=ORIENTED_EDGE('',*,*,#10303,.F.);
#14341=ORIENTED_EDGE('',*,*,#10064,.F.);
#14342=ORIENTED_EDGE('',*,*,#10302,.T.);
#14343=ORIENTED_EDGE('',*,*,#10306,.F.);
#14344=ORIENTED_EDGE('',*,*,#10307,.T.);
#14345=ORIENTED_EDGE('',*,*,#10066,.F.);
#14346=ORIENTED_EDGE('',*,*,#10307,.F.);
#14347=ORIENTED_EDGE('',*,*,#10308,.F.);
#14348=ORIENTED_EDGE('',*,*,#10309,.F.);
#14349=ORIENTED_EDGE('',*,*,#10067,.F.);
#14350=ORIENTED_EDGE('',*,*,#10310,.F.);
#14351=ORIENTED_EDGE('',*,*,#10069,.F.);
#14352=ORIENTED_EDGE('',*,*,#10311,.T.);
#14353=ORIENTED_EDGE('',*,*,#10312,.F.);
#14354=ORIENTED_EDGE('',*,*,#10309,.T.);
#14355=ORIENTED_EDGE('',*,*,#10313,.F.);
#14356=ORIENTED_EDGE('',*,*,#10311,.F.);
#14357=ORIENTED_EDGE('',*,*,#10068,.F.);
#14358=ORIENTED_EDGE('',*,*,#10310,.T.);
#14359=ORIENTED_EDGE('',*,*,#10314,.F.);
#14360=ORIENTED_EDGE('',*,*,#10315,.T.);
#14361=ORIENTED_EDGE('',*,*,#10070,.F.);
#14362=ORIENTED_EDGE('',*,*,#10315,.F.);
#14363=ORIENTED_EDGE('',*,*,#10316,.F.);
#14364=ORIENTED_EDGE('',*,*,#10317,.F.);
#14365=ORIENTED_EDGE('',*,*,#10071,.F.);
#14366=ORIENTED_EDGE('',*,*,#10318,.F.);
#14367=ORIENTED_EDGE('',*,*,#10073,.F.);
#14368=ORIENTED_EDGE('',*,*,#10319,.T.);
#14369=ORIENTED_EDGE('',*,*,#10320,.F.);
#14370=ORIENTED_EDGE('',*,*,#10317,.T.);
#14371=ORIENTED_EDGE('',*,*,#10321,.F.);
#14372=ORIENTED_EDGE('',*,*,#10319,.F.);
#14373=ORIENTED_EDGE('',*,*,#10072,.F.);
#14374=ORIENTED_EDGE('',*,*,#10318,.T.);
#14375=ORIENTED_EDGE('',*,*,#10322,.F.);
#14376=ORIENTED_EDGE('',*,*,#10323,.T.);
#14377=ORIENTED_EDGE('',*,*,#10074,.F.);
#14378=ORIENTED_EDGE('',*,*,#10323,.F.);
#14379=ORIENTED_EDGE('',*,*,#10324,.F.);
#14380=ORIENTED_EDGE('',*,*,#10325,.F.);
#14381=ORIENTED_EDGE('',*,*,#10075,.F.);
#14382=ORIENTED_EDGE('',*,*,#10326,.F.);
#14383=ORIENTED_EDGE('',*,*,#10077,.F.);
#14384=ORIENTED_EDGE('',*,*,#10327,.T.);
#14385=ORIENTED_EDGE('',*,*,#10328,.F.);
#14386=ORIENTED_EDGE('',*,*,#10325,.T.);
#14387=ORIENTED_EDGE('',*,*,#10329,.F.);
#14388=ORIENTED_EDGE('',*,*,#10327,.F.);
#14389=ORIENTED_EDGE('',*,*,#10076,.F.);
#14390=ORIENTED_EDGE('',*,*,#10326,.T.);
#14391=ORIENTED_EDGE('',*,*,#10330,.F.);
#14392=ORIENTED_EDGE('',*,*,#10331,.T.);
#14393=ORIENTED_EDGE('',*,*,#10078,.F.);
#14394=ORIENTED_EDGE('',*,*,#10331,.F.);
#14395=ORIENTED_EDGE('',*,*,#10332,.F.);
#14396=ORIENTED_EDGE('',*,*,#10333,.F.);
#14397=ORIENTED_EDGE('',*,*,#10079,.F.);
#14398=ORIENTED_EDGE('',*,*,#10334,.F.);
#14399=ORIENTED_EDGE('',*,*,#10081,.F.);
#14400=ORIENTED_EDGE('',*,*,#10335,.T.);
#14401=ORIENTED_EDGE('',*,*,#10336,.F.);
#14402=ORIENTED_EDGE('',*,*,#10333,.T.);
#14403=ORIENTED_EDGE('',*,*,#10337,.F.);
#14404=ORIENTED_EDGE('',*,*,#10335,.F.);
#14405=ORIENTED_EDGE('',*,*,#10080,.F.);
#14406=ORIENTED_EDGE('',*,*,#10334,.T.);
#14407=ORIENTED_EDGE('',*,*,#10338,.F.);
#14408=ORIENTED_EDGE('',*,*,#10339,.T.);
#14409=ORIENTED_EDGE('',*,*,#10082,.F.);
#14410=ORIENTED_EDGE('',*,*,#10339,.F.);
#14411=ORIENTED_EDGE('',*,*,#10340,.F.);
#14412=ORIENTED_EDGE('',*,*,#10341,.F.);
#14413=ORIENTED_EDGE('',*,*,#10083,.F.);
#14414=ORIENTED_EDGE('',*,*,#10342,.F.);
#14415=ORIENTED_EDGE('',*,*,#10085,.F.);
#14416=ORIENTED_EDGE('',*,*,#10343,.T.);
#14417=ORIENTED_EDGE('',*,*,#10344,.F.);
#14418=ORIENTED_EDGE('',*,*,#10341,.T.);
#14419=ORIENTED_EDGE('',*,*,#10345,.F.);
#14420=ORIENTED_EDGE('',*,*,#10343,.F.);
#14421=ORIENTED_EDGE('',*,*,#10084,.F.);
#14422=ORIENTED_EDGE('',*,*,#10342,.T.);
#14423=ORIENTED_EDGE('',*,*,#10346,.F.);
#14424=ORIENTED_EDGE('',*,*,#10347,.T.);
#14425=ORIENTED_EDGE('',*,*,#10086,.F.);
#14426=ORIENTED_EDGE('',*,*,#10347,.F.);
#14427=ORIENTED_EDGE('',*,*,#10348,.F.);
#14428=ORIENTED_EDGE('',*,*,#10349,.F.);
#14429=ORIENTED_EDGE('',*,*,#10087,.F.);
#14430=ORIENTED_EDGE('',*,*,#10350,.F.);
#14431=ORIENTED_EDGE('',*,*,#10089,.F.);
#14432=ORIENTED_EDGE('',*,*,#10351,.T.);
#14433=ORIENTED_EDGE('',*,*,#10352,.F.);
#14434=ORIENTED_EDGE('',*,*,#10349,.T.);
#14435=ORIENTED_EDGE('',*,*,#10353,.F.);
#14436=ORIENTED_EDGE('',*,*,#10351,.F.);
#14437=ORIENTED_EDGE('',*,*,#10088,.F.);
#14438=ORIENTED_EDGE('',*,*,#10350,.T.);
#14439=ORIENTED_EDGE('',*,*,#10354,.F.);
#14440=ORIENTED_EDGE('',*,*,#10355,.T.);
#14441=ORIENTED_EDGE('',*,*,#10090,.F.);
#14442=ORIENTED_EDGE('',*,*,#10355,.F.);
#14443=ORIENTED_EDGE('',*,*,#10356,.F.);
#14444=ORIENTED_EDGE('',*,*,#10357,.F.);
#14445=ORIENTED_EDGE('',*,*,#10091,.F.);
#14446=ORIENTED_EDGE('',*,*,#10358,.F.);
#14447=ORIENTED_EDGE('',*,*,#10093,.F.);
#14448=ORIENTED_EDGE('',*,*,#10359,.T.);
#14449=ORIENTED_EDGE('',*,*,#10360,.F.);
#14450=ORIENTED_EDGE('',*,*,#10357,.T.);
#14451=ORIENTED_EDGE('',*,*,#10361,.F.);
#14452=ORIENTED_EDGE('',*,*,#10359,.F.);
#14453=ORIENTED_EDGE('',*,*,#10092,.F.);
#14454=ORIENTED_EDGE('',*,*,#10358,.T.);
#14455=ORIENTED_EDGE('',*,*,#10362,.F.);
#14456=ORIENTED_EDGE('',*,*,#10363,.T.);
#14457=ORIENTED_EDGE('',*,*,#10094,.F.);
#14458=ORIENTED_EDGE('',*,*,#10363,.F.);
#14459=ORIENTED_EDGE('',*,*,#10364,.F.);
#14460=ORIENTED_EDGE('',*,*,#10365,.F.);
#14461=ORIENTED_EDGE('',*,*,#10095,.F.);
#14462=ORIENTED_EDGE('',*,*,#10366,.F.);
#14463=ORIENTED_EDGE('',*,*,#10097,.F.);
#14464=ORIENTED_EDGE('',*,*,#10367,.T.);
#14465=ORIENTED_EDGE('',*,*,#10368,.F.);
#14466=ORIENTED_EDGE('',*,*,#10365,.T.);
#14467=ORIENTED_EDGE('',*,*,#10369,.F.);
#14468=ORIENTED_EDGE('',*,*,#10367,.F.);
#14469=ORIENTED_EDGE('',*,*,#10096,.F.);
#14470=ORIENTED_EDGE('',*,*,#10366,.T.);
#14471=ORIENTED_EDGE('',*,*,#10370,.F.);
#14472=ORIENTED_EDGE('',*,*,#10371,.T.);
#14473=ORIENTED_EDGE('',*,*,#10098,.F.);
#14474=ORIENTED_EDGE('',*,*,#10371,.F.);
#14475=ORIENTED_EDGE('',*,*,#10372,.F.);
#14476=ORIENTED_EDGE('',*,*,#10373,.F.);
#14477=ORIENTED_EDGE('',*,*,#10099,.F.);
#14478=ORIENTED_EDGE('',*,*,#10374,.F.);
#14479=ORIENTED_EDGE('',*,*,#10101,.F.);
#14480=ORIENTED_EDGE('',*,*,#10375,.T.);
#14481=ORIENTED_EDGE('',*,*,#10376,.F.);
#14482=ORIENTED_EDGE('',*,*,#10373,.T.);
#14483=ORIENTED_EDGE('',*,*,#10377,.F.);
#14484=ORIENTED_EDGE('',*,*,#10375,.F.);
#14485=ORIENTED_EDGE('',*,*,#10100,.F.);
#14486=ORIENTED_EDGE('',*,*,#10374,.T.);
#14487=ORIENTED_EDGE('',*,*,#10378,.F.);
#14488=ORIENTED_EDGE('',*,*,#10379,.T.);
#14489=ORIENTED_EDGE('',*,*,#10102,.F.);
#14490=ORIENTED_EDGE('',*,*,#10379,.F.);
#14491=ORIENTED_EDGE('',*,*,#10380,.F.);
#14492=ORIENTED_EDGE('',*,*,#10381,.F.);
#14493=ORIENTED_EDGE('',*,*,#10103,.F.);
#14494=ORIENTED_EDGE('',*,*,#10382,.F.);
#14495=ORIENTED_EDGE('',*,*,#10105,.F.);
#14496=ORIENTED_EDGE('',*,*,#10383,.T.);
#14497=ORIENTED_EDGE('',*,*,#10384,.F.);
#14498=ORIENTED_EDGE('',*,*,#10381,.T.);
#14499=ORIENTED_EDGE('',*,*,#10385,.F.);
#14500=ORIENTED_EDGE('',*,*,#10383,.F.);
#14501=ORIENTED_EDGE('',*,*,#10104,.F.);
#14502=ORIENTED_EDGE('',*,*,#10382,.T.);
#14503=ORIENTED_EDGE('',*,*,#10386,.F.);
#14504=ORIENTED_EDGE('',*,*,#10387,.T.);
#14505=ORIENTED_EDGE('',*,*,#10106,.F.);
#14506=ORIENTED_EDGE('',*,*,#10387,.F.);
#14507=ORIENTED_EDGE('',*,*,#10388,.F.);
#14508=ORIENTED_EDGE('',*,*,#10389,.F.);
#14509=ORIENTED_EDGE('',*,*,#10107,.F.);
#14510=ORIENTED_EDGE('',*,*,#10390,.F.);
#14511=ORIENTED_EDGE('',*,*,#10109,.F.);
#14512=ORIENTED_EDGE('',*,*,#10391,.T.);
#14513=ORIENTED_EDGE('',*,*,#10392,.F.);
#14514=ORIENTED_EDGE('',*,*,#10389,.T.);
#14515=ORIENTED_EDGE('',*,*,#10393,.F.);
#14516=ORIENTED_EDGE('',*,*,#10391,.F.);
#14517=ORIENTED_EDGE('',*,*,#10108,.F.);
#14518=ORIENTED_EDGE('',*,*,#10390,.T.);
#14519=ORIENTED_EDGE('',*,*,#10394,.F.);
#14520=ORIENTED_EDGE('',*,*,#10395,.T.);
#14521=ORIENTED_EDGE('',*,*,#10110,.F.);
#14522=ORIENTED_EDGE('',*,*,#10395,.F.);
#14523=ORIENTED_EDGE('',*,*,#10396,.F.);
#14524=ORIENTED_EDGE('',*,*,#10397,.F.);
#14525=ORIENTED_EDGE('',*,*,#10111,.F.);
#14526=ORIENTED_EDGE('',*,*,#10398,.F.);
#14527=ORIENTED_EDGE('',*,*,#10113,.F.);
#14528=ORIENTED_EDGE('',*,*,#10399,.T.);
#14529=ORIENTED_EDGE('',*,*,#10400,.F.);
#14530=ORIENTED_EDGE('',*,*,#10397,.T.);
#14531=ORIENTED_EDGE('',*,*,#10401,.F.);
#14532=ORIENTED_EDGE('',*,*,#10399,.F.);
#14533=ORIENTED_EDGE('',*,*,#10112,.F.);
#14534=ORIENTED_EDGE('',*,*,#10398,.T.);
#14535=ORIENTED_EDGE('',*,*,#10402,.F.);
#14536=ORIENTED_EDGE('',*,*,#10403,.T.);
#14537=ORIENTED_EDGE('',*,*,#10114,.F.);
#14538=ORIENTED_EDGE('',*,*,#10403,.F.);
#14539=ORIENTED_EDGE('',*,*,#10404,.F.);
#14540=ORIENTED_EDGE('',*,*,#10405,.F.);
#14541=ORIENTED_EDGE('',*,*,#10115,.F.);
#14542=ORIENTED_EDGE('',*,*,#10406,.F.);
#14543=ORIENTED_EDGE('',*,*,#10117,.F.);
#14544=ORIENTED_EDGE('',*,*,#10407,.T.);
#14545=ORIENTED_EDGE('',*,*,#10408,.F.);
#14546=ORIENTED_EDGE('',*,*,#10405,.T.);
#14547=ORIENTED_EDGE('',*,*,#10409,.F.);
#14548=ORIENTED_EDGE('',*,*,#10407,.F.);
#14549=ORIENTED_EDGE('',*,*,#10116,.F.);
#14550=ORIENTED_EDGE('',*,*,#10406,.T.);
#14551=ORIENTED_EDGE('',*,*,#10410,.F.);
#14552=ORIENTED_EDGE('',*,*,#10411,.T.);
#14553=ORIENTED_EDGE('',*,*,#10118,.F.);
#14554=ORIENTED_EDGE('',*,*,#10411,.F.);
#14555=ORIENTED_EDGE('',*,*,#10412,.F.);
#14556=ORIENTED_EDGE('',*,*,#10413,.F.);
#14557=ORIENTED_EDGE('',*,*,#10119,.F.);
#14558=ORIENTED_EDGE('',*,*,#10414,.F.);
#14559=ORIENTED_EDGE('',*,*,#10121,.F.);
#14560=ORIENTED_EDGE('',*,*,#10415,.T.);
#14561=ORIENTED_EDGE('',*,*,#10416,.F.);
#14562=ORIENTED_EDGE('',*,*,#10413,.T.);
#14563=ORIENTED_EDGE('',*,*,#10417,.F.);
#14564=ORIENTED_EDGE('',*,*,#10415,.F.);
#14565=ORIENTED_EDGE('',*,*,#10120,.F.);
#14566=ORIENTED_EDGE('',*,*,#10414,.T.);
#14567=ORIENTED_EDGE('',*,*,#10418,.F.);
#14568=ORIENTED_EDGE('',*,*,#10419,.T.);
#14569=ORIENTED_EDGE('',*,*,#10122,.F.);
#14570=ORIENTED_EDGE('',*,*,#10419,.F.);
#14571=ORIENTED_EDGE('',*,*,#10420,.F.);
#14572=ORIENTED_EDGE('',*,*,#10421,.F.);
#14573=ORIENTED_EDGE('',*,*,#10123,.F.);
#14574=ORIENTED_EDGE('',*,*,#10422,.F.);
#14575=ORIENTED_EDGE('',*,*,#10125,.F.);
#14576=ORIENTED_EDGE('',*,*,#10423,.T.);
#14577=ORIENTED_EDGE('',*,*,#10424,.F.);
#14578=ORIENTED_EDGE('',*,*,#10421,.T.);
#14579=ORIENTED_EDGE('',*,*,#10425,.F.);
#14580=ORIENTED_EDGE('',*,*,#10423,.F.);
#14581=ORIENTED_EDGE('',*,*,#10124,.F.);
#14582=ORIENTED_EDGE('',*,*,#10422,.T.);
#14583=ORIENTED_EDGE('',*,*,#10426,.F.);
#14584=ORIENTED_EDGE('',*,*,#10427,.T.);
#14585=ORIENTED_EDGE('',*,*,#10126,.F.);
#14586=ORIENTED_EDGE('',*,*,#10427,.F.);
#14587=ORIENTED_EDGE('',*,*,#10428,.F.);
#14588=ORIENTED_EDGE('',*,*,#10429,.F.);
#14589=ORIENTED_EDGE('',*,*,#10127,.F.);
#14590=ORIENTED_EDGE('',*,*,#10430,.F.);
#14591=ORIENTED_EDGE('',*,*,#10129,.F.);
#14592=ORIENTED_EDGE('',*,*,#10431,.T.);
#14593=ORIENTED_EDGE('',*,*,#10432,.F.);
#14594=ORIENTED_EDGE('',*,*,#10429,.T.);
#14595=ORIENTED_EDGE('',*,*,#10433,.F.);
#14596=ORIENTED_EDGE('',*,*,#10431,.F.);
#14597=ORIENTED_EDGE('',*,*,#10128,.F.);
#14598=ORIENTED_EDGE('',*,*,#10430,.T.);
#14599=ORIENTED_EDGE('',*,*,#10434,.F.);
#14600=ORIENTED_EDGE('',*,*,#10435,.T.);
#14601=ORIENTED_EDGE('',*,*,#10130,.F.);
#14602=ORIENTED_EDGE('',*,*,#10435,.F.);
#14603=ORIENTED_EDGE('',*,*,#10436,.F.);
#14604=ORIENTED_EDGE('',*,*,#10437,.F.);
#14605=ORIENTED_EDGE('',*,*,#10131,.F.);
#14606=ORIENTED_EDGE('',*,*,#10438,.F.);
#14607=ORIENTED_EDGE('',*,*,#10133,.F.);
#14608=ORIENTED_EDGE('',*,*,#10439,.T.);
#14609=ORIENTED_EDGE('',*,*,#10440,.F.);
#14610=ORIENTED_EDGE('',*,*,#10437,.T.);
#14611=ORIENTED_EDGE('',*,*,#10441,.F.);
#14612=ORIENTED_EDGE('',*,*,#10439,.F.);
#14613=ORIENTED_EDGE('',*,*,#10132,.F.);
#14614=ORIENTED_EDGE('',*,*,#10438,.T.);
#14615=ORIENTED_EDGE('',*,*,#10442,.F.);
#14616=ORIENTED_EDGE('',*,*,#10443,.T.);
#14617=ORIENTED_EDGE('',*,*,#10134,.F.);
#14618=ORIENTED_EDGE('',*,*,#10443,.F.);
#14619=ORIENTED_EDGE('',*,*,#10444,.F.);
#14620=ORIENTED_EDGE('',*,*,#10445,.F.);
#14621=ORIENTED_EDGE('',*,*,#10135,.F.);
#14622=ORIENTED_EDGE('',*,*,#10446,.F.);
#14623=ORIENTED_EDGE('',*,*,#10137,.F.);
#14624=ORIENTED_EDGE('',*,*,#10447,.T.);
#14625=ORIENTED_EDGE('',*,*,#10448,.F.);
#14626=ORIENTED_EDGE('',*,*,#10445,.T.);
#14627=ORIENTED_EDGE('',*,*,#10449,.F.);
#14628=ORIENTED_EDGE('',*,*,#10447,.F.);
#14629=ORIENTED_EDGE('',*,*,#10136,.F.);
#14630=ORIENTED_EDGE('',*,*,#10446,.T.);
#14631=ORIENTED_EDGE('',*,*,#10450,.F.);
#14632=ORIENTED_EDGE('',*,*,#10451,.T.);
#14633=ORIENTED_EDGE('',*,*,#10138,.F.);
#14634=ORIENTED_EDGE('',*,*,#10451,.F.);
#14635=ORIENTED_EDGE('',*,*,#10452,.F.);
#14636=ORIENTED_EDGE('',*,*,#10453,.F.);
#14637=ORIENTED_EDGE('',*,*,#10139,.F.);
#14638=ORIENTED_EDGE('',*,*,#10454,.F.);
#14639=ORIENTED_EDGE('',*,*,#10141,.F.);
#14640=ORIENTED_EDGE('',*,*,#10455,.T.);
#14641=ORIENTED_EDGE('',*,*,#10456,.F.);
#14642=ORIENTED_EDGE('',*,*,#10453,.T.);
#14643=ORIENTED_EDGE('',*,*,#10457,.F.);
#14644=ORIENTED_EDGE('',*,*,#10455,.F.);
#14645=ORIENTED_EDGE('',*,*,#10140,.F.);
#14646=ORIENTED_EDGE('',*,*,#10454,.T.);
#14647=ORIENTED_EDGE('',*,*,#10458,.F.);
#14648=ORIENTED_EDGE('',*,*,#10459,.T.);
#14649=ORIENTED_EDGE('',*,*,#10142,.F.);
#14650=ORIENTED_EDGE('',*,*,#10459,.F.);
#14651=ORIENTED_EDGE('',*,*,#10460,.F.);
#14652=ORIENTED_EDGE('',*,*,#10461,.F.);
#14653=ORIENTED_EDGE('',*,*,#10143,.F.);
#14654=ORIENTED_EDGE('',*,*,#10462,.F.);
#14655=ORIENTED_EDGE('',*,*,#10145,.F.);
#14656=ORIENTED_EDGE('',*,*,#10463,.T.);
#14657=ORIENTED_EDGE('',*,*,#10464,.F.);
#14658=ORIENTED_EDGE('',*,*,#10461,.T.);
#14659=ORIENTED_EDGE('',*,*,#10465,.F.);
#14660=ORIENTED_EDGE('',*,*,#10463,.F.);
#14661=ORIENTED_EDGE('',*,*,#10144,.F.);
#14662=ORIENTED_EDGE('',*,*,#10462,.T.);
#14663=ORIENTED_EDGE('',*,*,#10466,.F.);
#14664=ORIENTED_EDGE('',*,*,#10467,.T.);
#14665=ORIENTED_EDGE('',*,*,#10146,.F.);
#14666=ORIENTED_EDGE('',*,*,#10467,.F.);
#14667=ORIENTED_EDGE('',*,*,#10468,.F.);
#14668=ORIENTED_EDGE('',*,*,#10469,.F.);
#14669=ORIENTED_EDGE('',*,*,#10147,.F.);
#14670=ORIENTED_EDGE('',*,*,#10469,.T.);
#14671=ORIENTED_EDGE('',*,*,#10470,.F.);
#14672=ORIENTED_EDGE('',*,*,#10471,.F.);
#14673=ORIENTED_EDGE('',*,*,#10148,.F.);
#14674=ORIENTED_EDGE('',*,*,#10472,.F.);
#14675=ORIENTED_EDGE('',*,*,#10149,.F.);
#14676=ORIENTED_EDGE('',*,*,#10471,.T.);
#14677=ORIENTED_EDGE('',*,*,#10473,.F.);
#14678=ORIENTED_EDGE('',*,*,#10472,.T.);
#14679=ORIENTED_EDGE('',*,*,#10474,.F.);
#14680=ORIENTED_EDGE('',*,*,#10475,.T.);
#14681=ORIENTED_EDGE('',*,*,#10150,.F.);
#14682=ORIENTED_EDGE('',*,*,#10476,.F.);
#14683=ORIENTED_EDGE('',*,*,#10153,.F.);
#14684=ORIENTED_EDGE('',*,*,#10477,.T.);
#14685=ORIENTED_EDGE('',*,*,#10478,.F.);
#14686=ORIENTED_EDGE('',*,*,#10475,.F.);
#14687=ORIENTED_EDGE('',*,*,#10479,.F.);
#14688=ORIENTED_EDGE('',*,*,#10480,.F.);
#14689=ORIENTED_EDGE('',*,*,#10151,.F.);
#14690=ORIENTED_EDGE('',*,*,#10480,.T.);
#14691=ORIENTED_EDGE('',*,*,#10481,.F.);
#14692=ORIENTED_EDGE('',*,*,#10477,.F.);
#14693=ORIENTED_EDGE('',*,*,#10152,.F.);
#14694=ORIENTED_EDGE('',*,*,#10168,.T.);
#14695=ORIENTED_EDGE('',*,*,#10169,.T.);
#14696=ORIENTED_EDGE('',*,*,#10164,.T.);
#14697=ORIENTED_EDGE('',*,*,#10482,.T.);
#14698=ORIENTED_EDGE('',*,*,#10478,.T.);
#14699=ORIENTED_EDGE('',*,*,#10481,.T.);
#14700=ORIENTED_EDGE('',*,*,#10479,.T.);
#14701=ORIENTED_EDGE('',*,*,#10474,.T.);
#14702=ORIENTED_EDGE('',*,*,#10473,.T.);
#14703=ORIENTED_EDGE('',*,*,#10470,.T.);
#14704=ORIENTED_EDGE('',*,*,#10468,.T.);
#14705=ORIENTED_EDGE('',*,*,#10466,.T.);
#14706=ORIENTED_EDGE('',*,*,#10464,.T.);
#14707=ORIENTED_EDGE('',*,*,#10465,.T.);
#14708=ORIENTED_EDGE('',*,*,#10460,.T.);
#14709=ORIENTED_EDGE('',*,*,#10458,.T.);
#14710=ORIENTED_EDGE('',*,*,#10456,.T.);
#14711=ORIENTED_EDGE('',*,*,#10457,.T.);
#14712=ORIENTED_EDGE('',*,*,#10452,.T.);
#14713=ORIENTED_EDGE('',*,*,#10450,.T.);
#14714=ORIENTED_EDGE('',*,*,#10448,.T.);
#14715=ORIENTED_EDGE('',*,*,#10449,.T.);
#14716=ORIENTED_EDGE('',*,*,#10444,.T.);
#14717=ORIENTED_EDGE('',*,*,#10442,.T.);
#14718=ORIENTED_EDGE('',*,*,#10440,.T.);
#14719=ORIENTED_EDGE('',*,*,#10441,.T.);
#14720=ORIENTED_EDGE('',*,*,#10436,.T.);
#14721=ORIENTED_EDGE('',*,*,#10434,.T.);
#14722=ORIENTED_EDGE('',*,*,#10432,.T.);
#14723=ORIENTED_EDGE('',*,*,#10433,.T.);
#14724=ORIENTED_EDGE('',*,*,#10428,.T.);
#14725=ORIENTED_EDGE('',*,*,#10426,.T.);
#14726=ORIENTED_EDGE('',*,*,#10424,.T.);
#14727=ORIENTED_EDGE('',*,*,#10425,.T.);
#14728=ORIENTED_EDGE('',*,*,#10420,.T.);
#14729=ORIENTED_EDGE('',*,*,#10418,.T.);
#14730=ORIENTED_EDGE('',*,*,#10416,.T.);
#14731=ORIENTED_EDGE('',*,*,#10417,.T.);
#14732=ORIENTED_EDGE('',*,*,#10412,.T.);
#14733=ORIENTED_EDGE('',*,*,#10410,.T.);
#14734=ORIENTED_EDGE('',*,*,#10408,.T.);
#14735=ORIENTED_EDGE('',*,*,#10409,.T.);
#14736=ORIENTED_EDGE('',*,*,#10404,.T.);
#14737=ORIENTED_EDGE('',*,*,#10402,.T.);
#14738=ORIENTED_EDGE('',*,*,#10400,.T.);
#14739=ORIENTED_EDGE('',*,*,#10401,.T.);
#14740=ORIENTED_EDGE('',*,*,#10396,.T.);
#14741=ORIENTED_EDGE('',*,*,#10394,.T.);
#14742=ORIENTED_EDGE('',*,*,#10392,.T.);
#14743=ORIENTED_EDGE('',*,*,#10393,.T.);
#14744=ORIENTED_EDGE('',*,*,#10388,.T.);
#14745=ORIENTED_EDGE('',*,*,#10386,.T.);
#14746=ORIENTED_EDGE('',*,*,#10384,.T.);
#14747=ORIENTED_EDGE('',*,*,#10385,.T.);
#14748=ORIENTED_EDGE('',*,*,#10380,.T.);
#14749=ORIENTED_EDGE('',*,*,#10378,.T.);
#14750=ORIENTED_EDGE('',*,*,#10376,.T.);
#14751=ORIENTED_EDGE('',*,*,#10377,.T.);
#14752=ORIENTED_EDGE('',*,*,#10372,.T.);
#14753=ORIENTED_EDGE('',*,*,#10370,.T.);
#14754=ORIENTED_EDGE('',*,*,#10368,.T.);
#14755=ORIENTED_EDGE('',*,*,#10369,.T.);
#14756=ORIENTED_EDGE('',*,*,#10364,.T.);
#14757=ORIENTED_EDGE('',*,*,#10362,.T.);
#14758=ORIENTED_EDGE('',*,*,#10360,.T.);
#14759=ORIENTED_EDGE('',*,*,#10361,.T.);
#14760=ORIENTED_EDGE('',*,*,#10356,.T.);
#14761=ORIENTED_EDGE('',*,*,#10354,.T.);
#14762=ORIENTED_EDGE('',*,*,#10352,.T.);
#14763=ORIENTED_EDGE('',*,*,#10353,.T.);
#14764=ORIENTED_EDGE('',*,*,#10348,.T.);
#14765=ORIENTED_EDGE('',*,*,#10346,.T.);
#14766=ORIENTED_EDGE('',*,*,#10344,.T.);
#14767=ORIENTED_EDGE('',*,*,#10345,.T.);
#14768=ORIENTED_EDGE('',*,*,#10340,.T.);
#14769=ORIENTED_EDGE('',*,*,#10338,.T.);
#14770=ORIENTED_EDGE('',*,*,#10336,.T.);
#14771=ORIENTED_EDGE('',*,*,#10337,.T.);
#14772=ORIENTED_EDGE('',*,*,#10332,.T.);
#14773=ORIENTED_EDGE('',*,*,#10330,.T.);
#14774=ORIENTED_EDGE('',*,*,#10328,.T.);
#14775=ORIENTED_EDGE('',*,*,#10329,.T.);
#14776=ORIENTED_EDGE('',*,*,#10324,.T.);
#14777=ORIENTED_EDGE('',*,*,#10322,.T.);
#14778=ORIENTED_EDGE('',*,*,#10320,.T.);
#14779=ORIENTED_EDGE('',*,*,#10321,.T.);
#14780=ORIENTED_EDGE('',*,*,#10316,.T.);
#14781=ORIENTED_EDGE('',*,*,#10314,.T.);
#14782=ORIENTED_EDGE('',*,*,#10312,.T.);
#14783=ORIENTED_EDGE('',*,*,#10313,.T.);
#14784=ORIENTED_EDGE('',*,*,#10308,.T.);
#14785=ORIENTED_EDGE('',*,*,#10306,.T.);
#14786=ORIENTED_EDGE('',*,*,#10304,.T.);
#14787=ORIENTED_EDGE('',*,*,#10305,.T.);
#14788=ORIENTED_EDGE('',*,*,#10300,.T.);
#14789=ORIENTED_EDGE('',*,*,#10298,.T.);
#14790=ORIENTED_EDGE('',*,*,#10296,.T.);
#14791=ORIENTED_EDGE('',*,*,#10297,.T.);
#14792=ORIENTED_EDGE('',*,*,#10292,.T.);
#14793=ORIENTED_EDGE('',*,*,#10290,.T.);
#14794=ORIENTED_EDGE('',*,*,#10288,.T.);
#14795=ORIENTED_EDGE('',*,*,#10289,.T.);
#14796=ORIENTED_EDGE('',*,*,#10284,.T.);
#14797=ORIENTED_EDGE('',*,*,#10282,.T.);
#14798=ORIENTED_EDGE('',*,*,#10280,.T.);
#14799=ORIENTED_EDGE('',*,*,#10281,.T.);
#14800=ORIENTED_EDGE('',*,*,#10276,.T.);
#14801=ORIENTED_EDGE('',*,*,#10274,.T.);
#14802=ORIENTED_EDGE('',*,*,#10272,.T.);
#14803=ORIENTED_EDGE('',*,*,#10273,.T.);
#14804=ORIENTED_EDGE('',*,*,#10268,.T.);
#14805=ORIENTED_EDGE('',*,*,#10266,.T.);
#14806=ORIENTED_EDGE('',*,*,#10264,.T.);
#14807=ORIENTED_EDGE('',*,*,#10265,.T.);
#14808=ORIENTED_EDGE('',*,*,#10260,.T.);
#14809=ORIENTED_EDGE('',*,*,#10258,.T.);
#14810=ORIENTED_EDGE('',*,*,#10256,.T.);
#14811=ORIENTED_EDGE('',*,*,#10257,.T.);
#14812=ORIENTED_EDGE('',*,*,#10252,.T.);
#14813=ORIENTED_EDGE('',*,*,#10250,.T.);
#14814=ORIENTED_EDGE('',*,*,#10248,.T.);
#14815=ORIENTED_EDGE('',*,*,#10249,.T.);
#14816=ORIENTED_EDGE('',*,*,#10244,.T.);
#14817=ORIENTED_EDGE('',*,*,#10242,.T.);
#14818=ORIENTED_EDGE('',*,*,#10240,.T.);
#14819=ORIENTED_EDGE('',*,*,#10241,.T.);
#14820=ORIENTED_EDGE('',*,*,#10236,.T.);
#14821=ORIENTED_EDGE('',*,*,#10234,.T.);
#14822=ORIENTED_EDGE('',*,*,#10232,.T.);
#14823=ORIENTED_EDGE('',*,*,#10233,.T.);
#14824=ORIENTED_EDGE('',*,*,#10228,.T.);
#14825=ORIENTED_EDGE('',*,*,#10226,.T.);
#14826=ORIENTED_EDGE('',*,*,#10224,.T.);
#14827=ORIENTED_EDGE('',*,*,#10225,.T.);
#14828=ORIENTED_EDGE('',*,*,#10220,.T.);
#14829=ORIENTED_EDGE('',*,*,#10218,.T.);
#14830=ORIENTED_EDGE('',*,*,#10216,.T.);
#14831=ORIENTED_EDGE('',*,*,#10217,.T.);
#14832=ORIENTED_EDGE('',*,*,#10212,.T.);
#14833=ORIENTED_EDGE('',*,*,#10210,.T.);
#14834=ORIENTED_EDGE('',*,*,#10208,.T.);
#14835=ORIENTED_EDGE('',*,*,#10209,.T.);
#14836=ORIENTED_EDGE('',*,*,#10204,.T.);
#14837=ORIENTED_EDGE('',*,*,#10202,.T.);
#14838=ORIENTED_EDGE('',*,*,#10200,.T.);
#14839=ORIENTED_EDGE('',*,*,#10201,.T.);
#14840=ORIENTED_EDGE('',*,*,#10196,.T.);
#14841=ORIENTED_EDGE('',*,*,#10194,.T.);
#14842=ORIENTED_EDGE('',*,*,#10192,.T.);
#14843=ORIENTED_EDGE('',*,*,#10193,.T.);
#14844=ORIENTED_EDGE('',*,*,#10188,.T.);
#14845=ORIENTED_EDGE('',*,*,#10186,.T.);
#14846=ORIENTED_EDGE('',*,*,#10184,.T.);
#14847=ORIENTED_EDGE('',*,*,#10185,.T.);
#14848=ORIENTED_EDGE('',*,*,#10180,.T.);
#14849=ORIENTED_EDGE('',*,*,#10178,.T.);
#14850=ORIENTED_EDGE('',*,*,#10176,.T.);
#14851=ORIENTED_EDGE('',*,*,#10177,.T.);
#14852=ORIENTED_EDGE('',*,*,#10172,.T.);
#14853=ORIENTED_EDGE('',*,*,#10170,.T.);
#14854=ORIENTED_EDGE('',*,*,#10162,.T.);
#14855=ORIENTED_EDGE('',*,*,#10163,.T.);
#14856=ORIENTED_EDGE('',*,*,#10154,.F.);
#14857=ORIENTED_EDGE('',*,*,#10476,.T.);
#14858=ORIENTED_EDGE('',*,*,#10482,.F.);
#15167=CYLINDRICAL_SURFACE('',#18291,1.);
#15168=CYLINDRICAL_SURFACE('',#18293,2.);
#15169=CYLINDRICAL_SURFACE('',#18298,3.75);
#15170=CYLINDRICAL_SURFACE('',#18301,3.75);
#15171=CYLINDRICAL_SURFACE('',#18304,3.75);
#15172=CYLINDRICAL_SURFACE('',#18307,3.75);
#15173=CYLINDRICAL_SURFACE('',#18310,3.75);
#15174=CYLINDRICAL_SURFACE('',#18313,3.75);
#15175=CYLINDRICAL_SURFACE('',#18316,3.75);
#15176=CYLINDRICAL_SURFACE('',#18319,3.75);
#15177=CYLINDRICAL_SURFACE('',#18322,3.75);
#15178=CYLINDRICAL_SURFACE('',#18325,3.75);
#15179=CYLINDRICAL_SURFACE('',#18328,3.75);
#15180=CYLINDRICAL_SURFACE('',#18331,3.75);
#15181=CYLINDRICAL_SURFACE('',#18334,3.75);
#15182=CYLINDRICAL_SURFACE('',#18337,3.75);
#15183=CYLINDRICAL_SURFACE('',#18340,3.75);
#15184=CYLINDRICAL_SURFACE('',#18343,3.75);
#15185=CYLINDRICAL_SURFACE('',#18346,3.75);
#15186=CYLINDRICAL_SURFACE('',#18349,3.75);
#15187=CYLINDRICAL_SURFACE('',#18352,3.75);
#15188=CYLINDRICAL_SURFACE('',#18355,3.75);
#15189=CYLINDRICAL_SURFACE('',#18358,3.75);
#15190=CYLINDRICAL_SURFACE('',#18361,3.75);
#15191=CYLINDRICAL_SURFACE('',#18364,3.75);
#15192=CYLINDRICAL_SURFACE('',#18367,3.75);
#15193=CYLINDRICAL_SURFACE('',#18370,3.75);
#15194=CYLINDRICAL_SURFACE('',#18373,3.75);
#15195=CYLINDRICAL_SURFACE('',#18376,3.75);
#15196=CYLINDRICAL_SURFACE('',#18379,3.75);
#15197=CYLINDRICAL_SURFACE('',#18382,3.75);
#15198=CYLINDRICAL_SURFACE('',#18385,3.75);
#15199=CYLINDRICAL_SURFACE('',#18388,3.75);
#15200=CYLINDRICAL_SURFACE('',#18391,3.75);
#15201=CYLINDRICAL_SURFACE('',#18394,3.75);
#15202=CYLINDRICAL_SURFACE('',#18397,3.75);
#15203=CYLINDRICAL_SURFACE('',#18400,3.75);
#15204=CYLINDRICAL_SURFACE('',#18403,3.75);
#15205=CYLINDRICAL_SURFACE('',#18406,3.75);
#15206=CYLINDRICAL_SURFACE('',#18409,3.75);
#15207=CYLINDRICAL_SURFACE('',#18412,3.75);
#15208=CYLINDRICAL_SURFACE('',#18417,3.75);
#15944=ADVANCED_FACE('',(#2737),#1946,.F.);
#15945=ADVANCED_FACE('',(#2738),#1947,.F.);
#15946=ADVANCED_FACE('',(#2739),#1948,.F.);
#15947=ADVANCED_FACE('',(#2740,#1599),#1949,.F.);
#15948=ADVANCED_FACE('',(#2741),#15167,.F.);
#15949=ADVANCED_FACE('',(#2742),#15168,.T.);
#15950=ADVANCED_FACE('',(#2743,#1600),#1950,.T.);
#15951=ADVANCED_FACE('',(#2744),#91,.T.);
#15952=ADVANCED_FACE('',(#2745),#92,.T.);
#15953=ADVANCED_FACE('',(#2746),#1951,.T.);
#15954=ADVANCED_FACE('',(#2747),#15169,.T.);
#15955=ADVANCED_FACE('',(#2748),#93,.T.);
#15956=ADVANCED_FACE('',(#2749),#94,.T.);
#15957=ADVANCED_FACE('',(#2750),#1952,.T.);
#15958=ADVANCED_FACE('',(#2751),#15170,.T.);
#15959=ADVANCED_FACE('',(#2752),#95,.T.);
#15960=ADVANCED_FACE('',(#2753),#96,.T.);
#15961=ADVANCED_FACE('',(#2754),#1953,.T.);
#15962=ADVANCED_FACE('',(#2755),#15171,.T.);
#15963=ADVANCED_FACE('',(#2756),#97,.T.);
#15964=ADVANCED_FACE('',(#2757),#98,.T.);
#15965=ADVANCED_FACE('',(#2758),#1954,.T.);
#15966=ADVANCED_FACE('',(#2759),#15172,.T.);
#15967=ADVANCED_FACE('',(#2760),#99,.T.);
#15968=ADVANCED_FACE('',(#2761),#100,.T.);
#15969=ADVANCED_FACE('',(#2762),#1955,.T.);
#15970=ADVANCED_FACE('',(#2763),#15173,.T.);
#15971=ADVANCED_FACE('',(#2764),#101,.T.);
#15972=ADVANCED_FACE('',(#2765),#102,.T.);
#15973=ADVANCED_FACE('',(#2766),#1956,.T.);
#15974=ADVANCED_FACE('',(#2767),#15174,.T.);
#15975=ADVANCED_FACE('',(#2768),#103,.T.);
#15976=ADVANCED_FACE('',(#2769),#104,.T.);
#15977=ADVANCED_FACE('',(#2770),#1957,.T.);
#15978=ADVANCED_FACE('',(#2771),#15175,.T.);
#15979=ADVANCED_FACE('',(#2772),#105,.T.);
#15980=ADVANCED_FACE('',(#2773),#106,.T.);
#15981=ADVANCED_FACE('',(#2774),#1958,.T.);
#15982=ADVANCED_FACE('',(#2775),#15176,.T.);
#15983=ADVANCED_FACE('',(#2776),#107,.T.);
#15984=ADVANCED_FACE('',(#2777),#108,.T.);
#15985=ADVANCED_FACE('',(#2778),#1959,.T.);
#15986=ADVANCED_FACE('',(#2779),#15177,.T.);
#15987=ADVANCED_FACE('',(#2780),#109,.T.);
#15988=ADVANCED_FACE('',(#2781),#110,.T.);
#15989=ADVANCED_FACE('',(#2782),#1960,.T.);
#15990=ADVANCED_FACE('',(#2783),#15178,.T.);
#15991=ADVANCED_FACE('',(#2784),#111,.T.);
#15992=ADVANCED_FACE('',(#2785),#112,.T.);
#15993=ADVANCED_FACE('',(#2786),#1961,.T.);
#15994=ADVANCED_FACE('',(#2787),#15179,.T.);
#15995=ADVANCED_FACE('',(#2788),#113,.T.);
#15996=ADVANCED_FACE('',(#2789),#114,.T.);
#15997=ADVANCED_FACE('',(#2790),#1962,.T.);
#15998=ADVANCED_FACE('',(#2791),#15180,.T.);
#15999=ADVANCED_FACE('',(#2792),#115,.T.);
#16000=ADVANCED_FACE('',(#2793),#116,.T.);
#16001=ADVANCED_FACE('',(#2794),#1963,.T.);
#16002=ADVANCED_FACE('',(#2795),#15181,.T.);
#16003=ADVANCED_FACE('',(#2796),#117,.T.);
#16004=ADVANCED_FACE('',(#2797),#118,.T.);
#16005=ADVANCED_FACE('',(#2798),#1964,.T.);
#16006=ADVANCED_FACE('',(#2799),#15182,.T.);
#16007=ADVANCED_FACE('',(#2800),#119,.T.);
#16008=ADVANCED_FACE('',(#2801),#120,.T.);
#16009=ADVANCED_FACE('',(#2802),#1965,.T.);
#16010=ADVANCED_FACE('',(#2803),#15183,.T.);
#16011=ADVANCED_FACE('',(#2804),#121,.T.);
#16012=ADVANCED_FACE('',(#2805),#122,.T.);
#16013=ADVANCED_FACE('',(#2806),#1966,.T.);
#16014=ADVANCED_FACE('',(#2807),#15184,.T.);
#16015=ADVANCED_FACE('',(#2808),#123,.T.);
#16016=ADVANCED_FACE('',(#2809),#124,.T.);
#16017=ADVANCED_FACE('',(#2810),#1967,.T.);
#16018=ADVANCED_FACE('',(#2811),#15185,.T.);
#16019=ADVANCED_FACE('',(#2812),#125,.T.);
#16020=ADVANCED_FACE('',(#2813),#126,.T.);
#16021=ADVANCED_FACE('',(#2814),#1968,.T.);
#16022=ADVANCED_FACE('',(#2815),#15186,.T.);
#16023=ADVANCED_FACE('',(#2816),#127,.T.);
#16024=ADVANCED_FACE('',(#2817),#128,.T.);
#16025=ADVANCED_FACE('',(#2818),#1969,.T.);
#16026=ADVANCED_FACE('',(#2819),#15187,.T.);
#16027=ADVANCED_FACE('',(#2820),#129,.T.);
#16028=ADVANCED_FACE('',(#2821),#130,.T.);
#16029=ADVANCED_FACE('',(#2822),#1970,.T.);
#16030=ADVANCED_FACE('',(#2823),#15188,.T.);
#16031=ADVANCED_FACE('',(#2824),#131,.T.);
#16032=ADVANCED_FACE('',(#2825),#132,.T.);
#16033=ADVANCED_FACE('',(#2826),#1971,.T.);
#16034=ADVANCED_FACE('',(#2827),#15189,.T.);
#16035=ADVANCED_FACE('',(#2828),#133,.T.);
#16036=ADVANCED_FACE('',(#2829),#134,.T.);
#16037=ADVANCED_FACE('',(#2830),#1972,.T.);
#16038=ADVANCED_FACE('',(#2831),#15190,.T.);
#16039=ADVANCED_FACE('',(#2832),#135,.T.);
#16040=ADVANCED_FACE('',(#2833),#136,.T.);
#16041=ADVANCED_FACE('',(#2834),#1973,.T.);
#16042=ADVANCED_FACE('',(#2835),#15191,.T.);
#16043=ADVANCED_FACE('',(#2836),#137,.T.);
#16044=ADVANCED_FACE('',(#2837),#138,.T.);
#16045=ADVANCED_FACE('',(#2838),#1974,.T.);
#16046=ADVANCED_FACE('',(#2839),#15192,.T.);
#16047=ADVANCED_FACE('',(#2840),#139,.T.);
#16048=ADVANCED_FACE('',(#2841),#140,.T.);
#16049=ADVANCED_FACE('',(#2842),#1975,.T.);
#16050=ADVANCED_FACE('',(#2843),#15193,.T.);
#16051=ADVANCED_FACE('',(#2844),#141,.T.);
#16052=ADVANCED_FACE('',(#2845),#142,.T.);
#16053=ADVANCED_FACE('',(#2846),#1976,.T.);
#16054=ADVANCED_FACE('',(#2847),#15194,.T.);
#16055=ADVANCED_FACE('',(#2848),#143,.T.);
#16056=ADVANCED_FACE('',(#2849),#144,.T.);
#16057=ADVANCED_FACE('',(#2850),#1977,.T.);
#16058=ADVANCED_FACE('',(#2851),#15195,.T.);
#16059=ADVANCED_FACE('',(#2852),#145,.T.);
#16060=ADVANCED_FACE('',(#2853),#146,.T.);
#16061=ADVANCED_FACE('',(#2854),#1978,.T.);
#16062=ADVANCED_FACE('',(#2855),#15196,.T.);
#16063=ADVANCED_FACE('',(#2856),#147,.T.);
#16064=ADVANCED_FACE('',(#2857),#148,.T.);
#16065=ADVANCED_FACE('',(#2858),#1979,.T.);
#16066=ADVANCED_FACE('',(#2859),#15197,.T.);
#16067=ADVANCED_FACE('',(#2860),#149,.T.);
#16068=ADVANCED_FACE('',(#2861),#150,.T.);
#16069=ADVANCED_FACE('',(#2862),#1980,.T.);
#16070=ADVANCED_FACE('',(#2863),#15198,.T.);
#16071=ADVANCED_FACE('',(#2864),#151,.T.);
#16072=ADVANCED_FACE('',(#2865),#152,.T.);
#16073=ADVANCED_FACE('',(#2866),#1981,.T.);
#16074=ADVANCED_FACE('',(#2867),#15199,.T.);
#16075=ADVANCED_FACE('',(#2868),#153,.T.);
#16076=ADVANCED_FACE('',(#2869),#154,.T.);
#16077=ADVANCED_FACE('',(#2870),#1982,.T.);
#16078=ADVANCED_FACE('',(#2871),#15200,.T.);
#16079=ADVANCED_FACE('',(#2872),#155,.T.);
#16080=ADVANCED_FACE('',(#2873),#156,.T.);
#16081=ADVANCED_FACE('',(#2874),#1983,.T.);
#16082=ADVANCED_FACE('',(#2875),#15201,.T.);
#16083=ADVANCED_FACE('',(#2876),#157,.T.);
#16084=ADVANCED_FACE('',(#2877),#158,.T.);
#16085=ADVANCED_FACE('',(#2878),#1984,.T.);
#16086=ADVANCED_FACE('',(#2879),#15202,.T.);
#16087=ADVANCED_FACE('',(#2880),#159,.T.);
#16088=ADVANCED_FACE('',(#2881),#160,.T.);
#16089=ADVANCED_FACE('',(#2882),#1985,.T.);
#16090=ADVANCED_FACE('',(#2883),#15203,.T.);
#16091=ADVANCED_FACE('',(#2884),#161,.T.);
#16092=ADVANCED_FACE('',(#2885),#162,.T.);
#16093=ADVANCED_FACE('',(#2886),#1986,.T.);
#16094=ADVANCED_FACE('',(#2887),#15204,.T.);
#16095=ADVANCED_FACE('',(#2888),#163,.T.);
#16096=ADVANCED_FACE('',(#2889),#164,.T.);
#16097=ADVANCED_FACE('',(#2890),#1987,.T.);
#16098=ADVANCED_FACE('',(#2891),#15205,.T.);
#16099=ADVANCED_FACE('',(#2892),#165,.T.);
#16100=ADVANCED_FACE('',(#2893),#166,.T.);
#16101=ADVANCED_FACE('',(#2894),#1988,.T.);
#16102=ADVANCED_FACE('',(#2895),#15206,.T.);
#16103=ADVANCED_FACE('',(#2896),#167,.T.);
#16104=ADVANCED_FACE('',(#2897),#1989,.T.);
#16105=ADVANCED_FACE('',(#2898),#168,.T.);
#16106=ADVANCED_FACE('',(#2899),#15207,.T.);
#16107=ADVANCED_FACE('',(#2900),#169,.T.);
#16108=ADVANCED_FACE('',(#2901),#170,.T.);
#16109=ADVANCED_FACE('',(#2902),#1990,.T.);
#16110=ADVANCED_FACE('',(#2903,#1601),#1991,.T.);
#16111=ADVANCED_FACE('',(#2904),#15208,.T.);
#16193=CLOSED_SHELL('',(#15944,#15945,#15946,#15947,#15948,#15949,#15950,
#15951,#15952,#15953,#15954,#15955,#15956,#15957,#15958,#15959,#15960,#15961,
#15962,#15963,#15964,#15965,#15966,#15967,#15968,#15969,#15970,#15971,#15972,
#15973,#15974,#15975,#15976,#15977,#15978,#15979,#15980,#15981,#15982,#15983,
#15984,#15985,#15986,#15987,#15988,#15989,#15990,#15991,#15992,#15993,#15994,
#15995,#15996,#15997,#15998,#15999,#16000,#16001,#16002,#16003,#16004,#16005,
#16006,#16007,#16008,#16009,#16010,#16011,#16012,#16013,#16014,#16015,#16016,
#16017,#16018,#16019,#16020,#16021,#16022,#16023,#16024,#16025,#16026,#16027,
#16028,#16029,#16030,#16031,#16032,#16033,#16034,#16035,#16036,#16037,#16038,
#16039,#16040,#16041,#16042,#16043,#16044,#16045,#16046,#16047,#16048,#16049,
#16050,#16051,#16052,#16053,#16054,#16055,#16056,#16057,#16058,#16059,#16060,
#16061,#16062,#16063,#16064,#16065,#16066,#16067,#16068,#16069,#16070,#16071,
#16072,#16073,#16074,#16075,#16076,#16077,#16078,#16079,#16080,#16081,#16082,
#16083,#16084,#16085,#16086,#16087,#16088,#16089,#16090,#16091,#16092,#16093,
#16094,#16095,#16096,#16097,#16098,#16099,#16100,#16101,#16102,#16103,#16104,
#16105,#16106,#16107,#16108,#16109,#16110,#16111));
#18245=AXIS2_PLACEMENT_3D('',#49605,#22153,#22154);
#18246=AXIS2_PLACEMENT_3D('',#49606,#22155,#22156);
#18247=AXIS2_PLACEMENT_3D('',#49615,#22161,#22162);
#18248=AXIS2_PLACEMENT_3D('',#49621,#22166,#22167);
#18249=AXIS2_PLACEMENT_3D('',#49627,#22171,#22172);
#18250=AXIS2_PLACEMENT_3D('',#49630,#22173,#22174);
#18251=AXIS2_PLACEMENT_3D('',#49776,#22176,#22177);
#18252=AXIS2_PLACEMENT_3D('',#49922,#22179,#22180);
#18253=AXIS2_PLACEMENT_3D('',#50068,#22182,#22183);
#18254=AXIS2_PLACEMENT_3D('',#50214,#22185,#22186);
#18255=AXIS2_PLACEMENT_3D('',#50360,#22188,#22189);
#18256=AXIS2_PLACEMENT_3D('',#50506,#22191,#22192);
#18257=AXIS2_PLACEMENT_3D('',#50652,#22194,#22195);
#18258=AXIS2_PLACEMENT_3D('',#50798,#22197,#22198);
#18259=AXIS2_PLACEMENT_3D('',#50944,#22200,#22201);
#18260=AXIS2_PLACEMENT_3D('',#51090,#22203,#22204);
#18261=AXIS2_PLACEMENT_3D('',#51236,#22206,#22207);
#18262=AXIS2_PLACEMENT_3D('',#51382,#22209,#22210);
#18263=AXIS2_PLACEMENT_3D('',#51528,#22212,#22213);
#18264=AXIS2_PLACEMENT_3D('',#51674,#22215,#22216);
#18265=AXIS2_PLACEMENT_3D('',#51820,#22218,#22219);
#18266=AXIS2_PLACEMENT_3D('',#51966,#22221,#22222);
#18267=AXIS2_PLACEMENT_3D('',#52112,#22224,#22225);
#18268=AXIS2_PLACEMENT_3D('',#52258,#22227,#22228);
#18269=AXIS2_PLACEMENT_3D('',#52404,#22230,#22231);
#18270=AXIS2_PLACEMENT_3D('',#52550,#22233,#22234);
#18271=AXIS2_PLACEMENT_3D('',#52696,#22236,#22237);
#18272=AXIS2_PLACEMENT_3D('',#52842,#22239,#22240);
#18273=AXIS2_PLACEMENT_3D('',#52988,#22242,#22243);
#18274=AXIS2_PLACEMENT_3D('',#53134,#22245,#22246);
#18275=AXIS2_PLACEMENT_3D('',#53280,#22248,#22249);
#18276=AXIS2_PLACEMENT_3D('',#53426,#22251,#22252);
#18277=AXIS2_PLACEMENT_3D('',#53572,#22254,#22255);
#18278=AXIS2_PLACEMENT_3D('',#53718,#22257,#22258);
#18279=AXIS2_PLACEMENT_3D('',#53864,#22260,#22261);
#18280=AXIS2_PLACEMENT_3D('',#54010,#22263,#22264);
#18281=AXIS2_PLACEMENT_3D('',#54156,#22266,#22267);
#18282=AXIS2_PLACEMENT_3D('',#54302,#22269,#22270);
#18283=AXIS2_PLACEMENT_3D('',#54448,#22272,#22273);
#18284=AXIS2_PLACEMENT_3D('',#54594,#22275,#22276);
#18285=AXIS2_PLACEMENT_3D('',#54740,#22278,#22279);
#18286=AXIS2_PLACEMENT_3D('',#54886,#22281,#22282);
#18287=AXIS2_PLACEMENT_3D('',#55032,#22284,#22285);
#18288=AXIS2_PLACEMENT_3D('',#55178,#22287,#22288);
#18289=AXIS2_PLACEMENT_3D('',#55324,#22290,#22291);
#18290=AXIS2_PLACEMENT_3D('',#55468,#22293,#22294);
#18291=AXIS2_PLACEMENT_3D('',#55469,#22295,#22296);
#18292=AXIS2_PLACEMENT_3D('',#55470,#22297,#22298);
#18293=AXIS2_PLACEMENT_3D('',#55471,#22299,#22300);
#18294=AXIS2_PLACEMENT_3D('',#55473,#22301,#22302);
#18295=AXIS2_PLACEMENT_3D('',#55476,#22304,#22305);
#18296=AXIS2_PLACEMENT_3D('',#55477,#22306,#22307);
#18297=AXIS2_PLACEMENT_3D('',#55916,#22310,#22311);
#18298=AXIS2_PLACEMENT_3D('',#55918,#22313,#22314);
#18299=AXIS2_PLACEMENT_3D('',#55920,#22315,#22316);
#18300=AXIS2_PLACEMENT_3D('',#56358,#22319,#22320);
#18301=AXIS2_PLACEMENT_3D('',#56360,#22322,#22323);
#18302=AXIS2_PLACEMENT_3D('',#56362,#22324,#22325);
#18303=AXIS2_PLACEMENT_3D('',#56800,#22328,#22329);
#18304=AXIS2_PLACEMENT_3D('',#56802,#22331,#22332);
#18305=AXIS2_PLACEMENT_3D('',#56804,#22333,#22334);
#18306=AXIS2_PLACEMENT_3D('',#57242,#22337,#22338);
#18307=AXIS2_PLACEMENT_3D('',#57244,#22340,#22341);
#18308=AXIS2_PLACEMENT_3D('',#57246,#22342,#22343);
#18309=AXIS2_PLACEMENT_3D('',#57684,#22346,#22347);
#18310=AXIS2_PLACEMENT_3D('',#57686,#22349,#22350);
#18311=AXIS2_PLACEMENT_3D('',#57688,#22351,#22352);
#18312=AXIS2_PLACEMENT_3D('',#58126,#22355,#22356);
#18313=AXIS2_PLACEMENT_3D('',#58128,#22358,#22359);
#18314=AXIS2_PLACEMENT_3D('',#58130,#22360,#22361);
#18315=AXIS2_PLACEMENT_3D('',#58568,#22364,#22365);
#18316=AXIS2_PLACEMENT_3D('',#58570,#22367,#22368);
#18317=AXIS2_PLACEMENT_3D('',#58572,#22369,#22370);
#18318=AXIS2_PLACEMENT_3D('',#59010,#22373,#22374);
#18319=AXIS2_PLACEMENT_3D('',#59012,#22376,#22377);
#18320=AXIS2_PLACEMENT_3D('',#59014,#22378,#22379);
#18321=AXIS2_PLACEMENT_3D('',#59452,#22382,#22383);
#18322=AXIS2_PLACEMENT_3D('',#59454,#22385,#22386);
#18323=AXIS2_PLACEMENT_3D('',#59456,#22387,#22388);
#18324=AXIS2_PLACEMENT_3D('',#59894,#22391,#22392);
#18325=AXIS2_PLACEMENT_3D('',#59896,#22394,#22395);
#18326=AXIS2_PLACEMENT_3D('',#59898,#22396,#22397);
#18327=AXIS2_PLACEMENT_3D('',#60336,#22400,#22401);
#18328=AXIS2_PLACEMENT_3D('',#60338,#22403,#22404);
#18329=AXIS2_PLACEMENT_3D('',#60340,#22405,#22406);
#18330=AXIS2_PLACEMENT_3D('',#60778,#22409,#22410);
#18331=AXIS2_PLACEMENT_3D('',#60780,#22412,#22413);
#18332=AXIS2_PLACEMENT_3D('',#60782,#22414,#22415);
#18333=AXIS2_PLACEMENT_3D('',#61220,#22418,#22419);
#18334=AXIS2_PLACEMENT_3D('',#61222,#22421,#22422);
#18335=AXIS2_PLACEMENT_3D('',#61224,#22423,#22424);
#18336=AXIS2_PLACEMENT_3D('',#61662,#22427,#22428);
#18337=AXIS2_PLACEMENT_3D('',#61664,#22430,#22431);
#18338=AXIS2_PLACEMENT_3D('',#61666,#22432,#22433);
#18339=AXIS2_PLACEMENT_3D('',#62104,#22436,#22437);
#18340=AXIS2_PLACEMENT_3D('',#62106,#22439,#22440);
#18341=AXIS2_PLACEMENT_3D('',#62108,#22441,#22442);
#18342=AXIS2_PLACEMENT_3D('',#62546,#22445,#22446);
#18343=AXIS2_PLACEMENT_3D('',#62548,#22448,#22449);
#18344=AXIS2_PLACEMENT_3D('',#62550,#22450,#22451);
#18345=AXIS2_PLACEMENT_3D('',#62988,#22454,#22455);
#18346=AXIS2_PLACEMENT_3D('',#62990,#22457,#22458);
#18347=AXIS2_PLACEMENT_3D('',#62992,#22459,#22460);
#18348=AXIS2_PLACEMENT_3D('',#63430,#22463,#22464);
#18349=AXIS2_PLACEMENT_3D('',#63432,#22466,#22467);
#18350=AXIS2_PLACEMENT_3D('',#63434,#22468,#22469);
#18351=AXIS2_PLACEMENT_3D('',#63872,#22472,#22473);
#18352=AXIS2_PLACEMENT_3D('',#63874,#22475,#22476);
#18353=AXIS2_PLACEMENT_3D('',#63876,#22477,#22478);
#18354=AXIS2_PLACEMENT_3D('',#64314,#22481,#22482);
#18355=AXIS2_PLACEMENT_3D('',#64316,#22484,#22485);
#18356=AXIS2_PLACEMENT_3D('',#64318,#22486,#22487);
#18357=AXIS2_PLACEMENT_3D('',#64756,#22490,#22491);
#18358=AXIS2_PLACEMENT_3D('',#64758,#22493,#22494);
#18359=AXIS2_PLACEMENT_3D('',#64760,#22495,#22496);
#18360=AXIS2_PLACEMENT_3D('',#65198,#22499,#22500);
#18361=AXIS2_PLACEMENT_3D('',#65200,#22502,#22503);
#18362=AXIS2_PLACEMENT_3D('',#65202,#22504,#22505);
#18363=AXIS2_PLACEMENT_3D('',#65640,#22508,#22509);
#18364=AXIS2_PLACEMENT_3D('',#65642,#22511,#22512);
#18365=AXIS2_PLACEMENT_3D('',#65644,#22513,#22514);
#18366=AXIS2_PLACEMENT_3D('',#66082,#22517,#22518);
#18367=AXIS2_PLACEMENT_3D('',#66084,#22520,#22521);
#18368=AXIS2_PLACEMENT_3D('',#66086,#22522,#22523);
#18369=AXIS2_PLACEMENT_3D('',#66524,#22526,#22527);
#18370=AXIS2_PLACEMENT_3D('',#66526,#22529,#22530);
#18371=AXIS2_PLACEMENT_3D('',#66528,#22531,#22532);
#18372=AXIS2_PLACEMENT_3D('',#66966,#22535,#22536);
#18373=AXIS2_PLACEMENT_3D('',#66968,#22538,#22539);
#18374=AXIS2_PLACEMENT_3D('',#66970,#22540,#22541);
#18375=AXIS2_PLACEMENT_3D('',#67408,#22544,#22545);
#18376=AXIS2_PLACEMENT_3D('',#67410,#22547,#22548);
#18377=AXIS2_PLACEMENT_3D('',#67412,#22549,#22550);
#18378=AXIS2_PLACEMENT_3D('',#67850,#22553,#22554);
#18379=AXIS2_PLACEMENT_3D('',#67852,#22556,#22557);
#18380=AXIS2_PLACEMENT_3D('',#67854,#22558,#22559);
#18381=AXIS2_PLACEMENT_3D('',#68292,#22562,#22563);
#18382=AXIS2_PLACEMENT_3D('',#68294,#22565,#22566);
#18383=AXIS2_PLACEMENT_3D('',#68296,#22567,#22568);
#18384=AXIS2_PLACEMENT_3D('',#68734,#22571,#22572);
#18385=AXIS2_PLACEMENT_3D('',#68736,#22574,#22575);
#18386=AXIS2_PLACEMENT_3D('',#68738,#22576,#22577);
#18387=AXIS2_PLACEMENT_3D('',#69176,#22580,#22581);
#18388=AXIS2_PLACEMENT_3D('',#69178,#22583,#22584);
#18389=AXIS2_PLACEMENT_3D('',#69180,#22585,#22586);
#18390=AXIS2_PLACEMENT_3D('',#69618,#22589,#22590);
#18391=AXIS2_PLACEMENT_3D('',#69620,#22592,#22593);
#18392=AXIS2_PLACEMENT_3D('',#69622,#22594,#22595);
#18393=AXIS2_PLACEMENT_3D('',#70060,#22598,#22599);
#18394=AXIS2_PLACEMENT_3D('',#70062,#22601,#22602);
#18395=AXIS2_PLACEMENT_3D('',#70064,#22603,#22604);
#18396=AXIS2_PLACEMENT_3D('',#70502,#22607,#22608);
#18397=AXIS2_PLACEMENT_3D('',#70504,#22610,#22611);
#18398=AXIS2_PLACEMENT_3D('',#70506,#22612,#22613);
#18399=AXIS2_PLACEMENT_3D('',#70944,#22616,#22617);
#18400=AXIS2_PLACEMENT_3D('',#70946,#22619,#22620);
#18401=AXIS2_PLACEMENT_3D('',#70948,#22621,#22622);
#18402=AXIS2_PLACEMENT_3D('',#71386,#22625,#22626);
#18403=AXIS2_PLACEMENT_3D('',#71388,#22628,#22629);
#18404=AXIS2_PLACEMENT_3D('',#71390,#22630,#22631);
#18405=AXIS2_PLACEMENT_3D('',#71828,#22634,#22635);
#18406=AXIS2_PLACEMENT_3D('',#71830,#22637,#22638);
#18407=AXIS2_PLACEMENT_3D('',#71832,#22639,#22640);
#18408=AXIS2_PLACEMENT_3D('',#72270,#22643,#22644);
#18409=AXIS2_PLACEMENT_3D('',#72272,#22646,#22647);
#18410=AXIS2_PLACEMENT_3D('',#72274,#22648,#22649);
#18411=AXIS2_PLACEMENT_3D('',#72493,#22651,#22652);
#18412=AXIS2_PLACEMENT_3D('',#72714,#22655,#22656);
#18413=AXIS2_PLACEMENT_3D('',#72716,#22657,#22658);
#18414=AXIS2_PLACEMENT_3D('',#73154,#22661,#22662);
#18415=AXIS2_PLACEMENT_3D('',#73156,#22664,#22665);
#18416=AXIS2_PLACEMENT_3D('',#73157,#22666,#22667);
#18417=AXIS2_PLACEMENT_3D('',#73158,#22668,#22669);
#22153=DIRECTION('axis',(0.,0.,1.));
#22154=DIRECTION('refdir',(1.,0.,0.));
#22155=DIRECTION('center_axis',(1.,0.,0.));
#22156=DIRECTION('ref_axis',(0.,0.,-1.));
#22157=DIRECTION('',(0.,0.,1.));
#22158=DIRECTION('',(0.,1.,0.));
#22159=DIRECTION('',(0.,0.,-1.));
#22160=DIRECTION('',(0.,-1.,0.));
#22161=DIRECTION('center_axis',(0.,0.,-1.));
#22162=DIRECTION('ref_axis',(-1.,0.,0.));
#22163=DIRECTION('',(1.,0.,0.));
#22164=DIRECTION('',(0.,-1.,0.));
#22165=DIRECTION('',(-1.,0.,0.));
#22166=DIRECTION('center_axis',(-1.,0.,0.));
#22167=DIRECTION('ref_axis',(0.,0.,1.));
#22168=DIRECTION('',(0.,0.,-1.));
#22169=DIRECTION('',(0.,1.,0.));
#22170=DIRECTION('',(0.,0.,1.));
#22171=DIRECTION('center_axis',(0.,1.,0.));
#22172=DIRECTION('ref_axis',(1.,0.,0.));
#22173=DIRECTION('center_axis',(0.,-1.,0.));
#22174=DIRECTION('ref_axis',(1.,0.,0.));
#22175=DIRECTION('',(-0.309016994374948,0.,0.951056516295154));
#22176=DIRECTION('center_axis',(0.,-1.,0.));
#22177=DIRECTION('ref_axis',(1.,0.,0.));
#22178=DIRECTION('',(-0.453990499739547,0.,0.891006524188368));
#22179=DIRECTION('center_axis',(0.,-1.,0.));
#22180=DIRECTION('ref_axis',(1.,0.,0.));
#22181=DIRECTION('',(-0.587785252292473,0.,0.809016994374947));
#22182=DIRECTION('center_axis',(0.,-1.,0.));
#22183=DIRECTION('ref_axis',(1.,0.,0.));
#22184=DIRECTION('',(-0.707106781186548,0.,0.707106781186547));
#22185=DIRECTION('center_axis',(0.,-1.,0.));
#22186=DIRECTION('ref_axis',(1.,0.,0.));
#22187=DIRECTION('',(-0.809016994374948,0.,0.587785252292473));
#22188=DIRECTION('center_axis',(0.,-1.,0.));
#22189=DIRECTION('ref_axis',(1.,0.,0.));
#22190=DIRECTION('',(-0.891006524188368,0.,0.453990499739547));
#22191=DIRECTION('center_axis',(0.,-1.,0.));
#22192=DIRECTION('ref_axis',(1.,0.,0.));
#22193=DIRECTION('',(-0.951056516295154,0.,0.309016994374947));
#22194=DIRECTION('center_axis',(0.,-1.,0.));
#22195=DIRECTION('ref_axis',(1.,0.,0.));
#22196=DIRECTION('',(-0.987688340595138,0.,0.156434465040231));
#22197=DIRECTION('center_axis',(0.,-1.,0.));
#22198=DIRECTION('ref_axis',(1.,0.,0.));
#22199=DIRECTION('',(-1.,0.,-1.83697019872103E-16));
#22200=DIRECTION('center_axis',(0.,-1.,0.));
#22201=DIRECTION('ref_axis',(1.,0.,0.));
#22202=DIRECTION('',(-0.987688340595138,0.,-0.156434465040231));
#22203=DIRECTION('center_axis',(0.,-1.,0.));
#22204=DIRECTION('ref_axis',(1.,0.,0.));
#22205=DIRECTION('',(-0.951056516295154,0.,-0.309016994374948));
#22206=DIRECTION('center_axis',(0.,-1.,0.));
#22207=DIRECTION('ref_axis',(1.,0.,0.));
#22208=DIRECTION('',(-0.891006524188368,0.,-0.453990499739547));
#22209=DIRECTION('center_axis',(0.,-1.,0.));
#22210=DIRECTION('ref_axis',(1.,0.,0.));
#22211=DIRECTION('',(-0.809016994374947,0.,-0.587785252292473));
#22212=DIRECTION('center_axis',(0.,-1.,0.));
#22213=DIRECTION('ref_axis',(1.,0.,0.));
#22214=DIRECTION('',(-0.707106781186547,0.,-0.707106781186548));
#22215=DIRECTION('center_axis',(0.,-1.,0.));
#22216=DIRECTION('ref_axis',(1.,0.,0.));
#22217=DIRECTION('',(-0.587785252292473,0.,-0.809016994374948));
#22218=DIRECTION('center_axis',(0.,-1.,0.));
#22219=DIRECTION('ref_axis',(1.,0.,0.));
#22220=DIRECTION('',(-0.453990499739547,0.,-0.891006524188368));
#22221=DIRECTION('center_axis',(0.,-1.,0.));
#22222=DIRECTION('ref_axis',(1.,0.,0.));
#22223=DIRECTION('',(-0.309016994374947,0.,-0.951056516295154));
#22224=DIRECTION('center_axis',(0.,-1.,0.));
#22225=DIRECTION('ref_axis',(1.,0.,0.));
#22226=DIRECTION('',(-0.156434465040231,0.,-0.987688340595138));
#22227=DIRECTION('center_axis',(0.,-1.,0.));
#22228=DIRECTION('ref_axis',(1.,0.,0.));
#22229=DIRECTION('',(1.22464679914735E-16,0.,-1.));
#22230=DIRECTION('center_axis',(0.,-1.,0.));
#22231=DIRECTION('ref_axis',(1.,0.,0.));
#22232=DIRECTION('',(0.156434465040231,0.,-0.987688340595138));
#22233=DIRECTION('center_axis',(0.,-1.,0.));
#22234=DIRECTION('ref_axis',(1.,0.,0.));
#22235=DIRECTION('',(0.309016994374948,0.,-0.951056516295154));
#22236=DIRECTION('center_axis',(0.,-1.,0.));
#22237=DIRECTION('ref_axis',(1.,0.,0.));
#22238=DIRECTION('',(0.453990499739547,0.,-0.891006524188368));
#22239=DIRECTION('center_axis',(0.,-1.,0.));
#22240=DIRECTION('ref_axis',(1.,0.,0.));
#22241=DIRECTION('',(0.587785252292473,0.,-0.809016994374947));
#22242=DIRECTION('center_axis',(0.,-1.,0.));
#22243=DIRECTION('ref_axis',(1.,0.,0.));
#22244=DIRECTION('',(0.707106781186548,0.,-0.707106781186547));
#22245=DIRECTION('center_axis',(0.,-1.,0.));
#22246=DIRECTION('ref_axis',(1.,0.,0.));
#22247=DIRECTION('',(0.809016994374948,0.,-0.587785252292473));
#22248=DIRECTION('center_axis',(0.,-1.,0.));
#22249=DIRECTION('ref_axis',(1.,0.,0.));
#22250=DIRECTION('',(0.891006524188368,0.,-0.453990499739547));
#22251=DIRECTION('center_axis',(0.,-1.,0.));
#22252=DIRECTION('ref_axis',(1.,0.,0.));
#22253=DIRECTION('',(0.951056516295154,0.,-0.309016994374947));
#22254=DIRECTION('center_axis',(0.,-1.,0.));
#22255=DIRECTION('ref_axis',(1.,0.,0.));
#22256=DIRECTION('',(0.987688340595138,0.,-0.156434465040231));
#22257=DIRECTION('center_axis',(0.,-1.,0.));
#22258=DIRECTION('ref_axis',(1.,0.,0.));
#22259=DIRECTION('',(1.,0.,6.12323399573677E-17));
#22260=DIRECTION('center_axis',(0.,-1.,0.));
#22261=DIRECTION('ref_axis',(1.,0.,0.));
#22262=DIRECTION('',(0.987688340595138,0.,0.156434465040231));
#22263=DIRECTION('center_axis',(0.,-1.,0.));
#22264=DIRECTION('ref_axis',(1.,0.,0.));
#22265=DIRECTION('',(0.951056516295154,0.,0.309016994374948));
#22266=DIRECTION('center_axis',(0.,-1.,0.));
#22267=DIRECTION('ref_axis',(1.,0.,0.));
#22268=DIRECTION('',(0.891006524188368,0.,0.453990499739547));
#22269=DIRECTION('center_axis',(0.,-1.,0.));
#22270=DIRECTION('ref_axis',(1.,0.,0.));
#22271=DIRECTION('',(0.809016994374947,0.,0.587785252292473));
#22272=DIRECTION('center_axis',(0.,-1.,0.));
#22273=DIRECTION('ref_axis',(1.,0.,0.));
#22274=DIRECTION('',(0.707106781186547,0.,0.707106781186548));
#22275=DIRECTION('center_axis',(0.,-1.,0.));
#22276=DIRECTION('ref_axis',(1.,0.,0.));
#22277=DIRECTION('',(0.587785252292473,0.,0.809016994374947));
#22278=DIRECTION('center_axis',(0.,-1.,0.));
#22279=DIRECTION('ref_axis',(1.,0.,0.));
#22280=DIRECTION('',(0.453990499739547,0.,0.891006524188368));
#22281=DIRECTION('center_axis',(0.,-1.,0.));
#22282=DIRECTION('ref_axis',(1.,0.,0.));
#22283=DIRECTION('',(0.309016994374947,0.,0.951056516295154));
#22284=DIRECTION('center_axis',(0.,-1.,0.));
#22285=DIRECTION('ref_axis',(1.,0.,0.));
#22286=DIRECTION('',(0.156434465040231,0.,0.987688340595138));
#22287=DIRECTION('center_axis',(0.,-1.,0.));
#22288=DIRECTION('ref_axis',(1.,0.,0.));
#22289=DIRECTION('',(0.,0.,1.));
#22290=DIRECTION('center_axis',(0.,-1.,0.));
#22291=DIRECTION('ref_axis',(1.,0.,0.));
#22292=DIRECTION('',(-0.156434465040231,0.,0.987688340595138));
#22293=DIRECTION('center_axis',(0.,1.,0.));
#22294=DIRECTION('ref_axis',(1.,0.,0.));
#22295=DIRECTION('center_axis',(0.,1.,0.));
#22296=DIRECTION('ref_axis',(6.12323399573677E-17,0.,1.));
#22297=DIRECTION('center_axis',(0.,-1.,0.));
#22298=DIRECTION('ref_axis',(1.,0.,0.));
#22299=DIRECTION('center_axis',(0.,1.,0.));
#22300=DIRECTION('ref_axis',(1.,0.,0.));
#22301=DIRECTION('center_axis',(0.,1.,0.));
#22302=DIRECTION('ref_axis',(1.,0.,0.));
#22303=DIRECTION('',(0.,-1.,0.));
#22304=DIRECTION('center_axis',(0.,-1.,0.));
#22305=DIRECTION('ref_axis',(1.,0.,0.));
#22306=DIRECTION('center_axis',(0.,1.,0.));
#22307=DIRECTION('ref_axis',(1.,0.,0.));
#22308=DIRECTION('',(0.,1.,0.));
#22309=DIRECTION('',(0.,1.,0.));
#22310=DIRECTION('center_axis',(0.987688340595138,0.,0.156434465040231));
#22311=DIRECTION('ref_axis',(0.156434465040231,0.,-0.987688340595138));
#22312=DIRECTION('',(0.156434465040231,0.,-0.987688340595138));
#22313=DIRECTION('center_axis',(0.,1.,0.));
#22314=DIRECTION('ref_axis',(1.,0.,0.));
#22315=DIRECTION('center_axis',(0.,1.,0.));
#22316=DIRECTION('ref_axis',(1.,0.,0.));
#22317=DIRECTION('',(0.,1.,0.));
#22318=DIRECTION('',(0.,1.,0.));
#22319=DIRECTION('center_axis',(0.951056516295154,0.,0.309016994374948));
#22320=DIRECTION('ref_axis',(0.309016994374948,0.,-0.951056516295154));
#22321=DIRECTION('',(0.309016994374948,0.,-0.951056516295154));
#22322=DIRECTION('center_axis',(0.,1.,0.));
#22323=DIRECTION('ref_axis',(1.,0.,0.));
#22324=DIRECTION('center_axis',(0.,1.,0.));
#22325=DIRECTION('ref_axis',(1.,0.,0.));
#22326=DIRECTION('',(0.,1.,0.));
#22327=DIRECTION('',(0.,1.,0.));
#22328=DIRECTION('center_axis',(0.891006524188368,0.,0.453990499739547));
#22329=DIRECTION('ref_axis',(0.453990499739547,0.,-0.891006524188368));
#22330=DIRECTION('',(0.453990499739547,0.,-0.891006524188368));
#22331=DIRECTION('center_axis',(0.,1.,0.));
#22332=DIRECTION('ref_axis',(1.,0.,0.));
#22333=DIRECTION('center_axis',(0.,1.,0.));
#22334=DIRECTION('ref_axis',(1.,0.,0.));
#22335=DIRECTION('',(0.,1.,0.));
#22336=DIRECTION('',(0.,1.,0.));
#22337=DIRECTION('center_axis',(0.809016994374947,0.,0.587785252292473));
#22338=DIRECTION('ref_axis',(0.587785252292473,0.,-0.809016994374947));
#22339=DIRECTION('',(0.587785252292473,0.,-0.809016994374947));
#22340=DIRECTION('center_axis',(0.,1.,0.));
#22341=DIRECTION('ref_axis',(1.,0.,0.));
#22342=DIRECTION('center_axis',(0.,1.,0.));
#22343=DIRECTION('ref_axis',(1.,0.,0.));
#22344=DIRECTION('',(0.,1.,0.));
#22345=DIRECTION('',(0.,1.,0.));
#22346=DIRECTION('center_axis',(0.707106781186547,0.,0.707106781186548));
#22347=DIRECTION('ref_axis',(0.707106781186548,0.,-0.707106781186547));
#22348=DIRECTION('',(0.707106781186548,0.,-0.707106781186547));
#22349=DIRECTION('center_axis',(0.,1.,0.));
#22350=DIRECTION('ref_axis',(1.,0.,0.));
#22351=DIRECTION('center_axis',(0.,1.,0.));
#22352=DIRECTION('ref_axis',(1.,0.,0.));
#22353=DIRECTION('',(0.,1.,0.));
#22354=DIRECTION('',(0.,1.,0.));
#22355=DIRECTION('center_axis',(0.587785252292473,0.,0.809016994374948));
#22356=DIRECTION('ref_axis',(0.809016994374948,0.,-0.587785252292473));
#22357=DIRECTION('',(0.809016994374948,0.,-0.587785252292473));
#22358=DIRECTION('center_axis',(0.,1.,0.));
#22359=DIRECTION('ref_axis',(1.,0.,0.));
#22360=DIRECTION('center_axis',(0.,1.,0.));
#22361=DIRECTION('ref_axis',(1.,0.,0.));
#22362=DIRECTION('',(0.,1.,0.));
#22363=DIRECTION('',(0.,1.,0.));
#22364=DIRECTION('center_axis',(0.453990499739547,0.,0.891006524188368));
#22365=DIRECTION('ref_axis',(0.891006524188368,0.,-0.453990499739547));
#22366=DIRECTION('',(0.891006524188368,0.,-0.453990499739547));
#22367=DIRECTION('center_axis',(0.,1.,0.));
#22368=DIRECTION('ref_axis',(1.,0.,0.));
#22369=DIRECTION('center_axis',(0.,1.,0.));
#22370=DIRECTION('ref_axis',(1.,0.,0.));
#22371=DIRECTION('',(0.,1.,0.));
#22372=DIRECTION('',(0.,1.,0.));
#22373=DIRECTION('center_axis',(0.309016994374947,0.,0.951056516295154));
#22374=DIRECTION('ref_axis',(0.951056516295154,0.,-0.309016994374947));
#22375=DIRECTION('',(0.951056516295154,0.,-0.309016994374947));
#22376=DIRECTION('center_axis',(0.,1.,0.));
#22377=DIRECTION('ref_axis',(1.,0.,0.));
#22378=DIRECTION('center_axis',(0.,1.,0.));
#22379=DIRECTION('ref_axis',(1.,0.,0.));
#22380=DIRECTION('',(0.,1.,0.));
#22381=DIRECTION('',(0.,1.,0.));
#22382=DIRECTION('center_axis',(0.156434465040231,0.,0.987688340595138));
#22383=DIRECTION('ref_axis',(0.987688340595138,0.,-0.156434465040231));
#22384=DIRECTION('',(0.987688340595138,0.,-0.156434465040231));
#22385=DIRECTION('center_axis',(0.,1.,0.));
#22386=DIRECTION('ref_axis',(1.,0.,0.));
#22387=DIRECTION('center_axis',(0.,1.,0.));
#22388=DIRECTION('ref_axis',(1.,0.,0.));
#22389=DIRECTION('',(0.,1.,0.));
#22390=DIRECTION('',(0.,1.,0.));
#22391=DIRECTION('center_axis',(-1.83697019872103E-16,0.,1.));
#22392=DIRECTION('ref_axis',(1.,0.,1.83697019872103E-16));
#22393=DIRECTION('',(1.,0.,1.83697019872103E-16));
#22394=DIRECTION('center_axis',(0.,1.,0.));
#22395=DIRECTION('ref_axis',(1.,0.,0.));
#22396=DIRECTION('center_axis',(0.,1.,0.));
#22397=DIRECTION('ref_axis',(1.,0.,0.));
#22398=DIRECTION('',(0.,1.,0.));
#22399=DIRECTION('',(0.,1.,0.));
#22400=DIRECTION('center_axis',(-0.156434465040231,0.,0.987688340595138));
#22401=DIRECTION('ref_axis',(0.987688340595138,0.,0.156434465040231));
#22402=DIRECTION('',(0.987688340595138,0.,0.156434465040231));
#22403=DIRECTION('center_axis',(0.,1.,0.));
#22404=DIRECTION('ref_axis',(1.,0.,0.));
#22405=DIRECTION('center_axis',(0.,1.,0.));
#22406=DIRECTION('ref_axis',(1.,0.,0.));
#22407=DIRECTION('',(0.,1.,0.));
#22408=DIRECTION('',(0.,1.,0.));
#22409=DIRECTION('center_axis',(-0.309016994374948,0.,0.951056516295154));
#22410=DIRECTION('ref_axis',(0.951056516295154,0.,0.309016994374948));
#22411=DIRECTION('',(0.951056516295154,0.,0.309016994374948));
#22412=DIRECTION('center_axis',(0.,1.,0.));
#22413=DIRECTION('ref_axis',(1.,0.,0.));
#22414=DIRECTION('center_axis',(0.,1.,0.));
#22415=DIRECTION('ref_axis',(1.,0.,0.));
#22416=DIRECTION('',(0.,1.,0.));
#22417=DIRECTION('',(0.,1.,0.));
#22418=DIRECTION('center_axis',(-0.453990499739547,0.,0.891006524188368));
#22419=DIRECTION('ref_axis',(0.891006524188368,0.,0.453990499739547));
#22420=DIRECTION('',(0.891006524188368,0.,0.453990499739547));
#22421=DIRECTION('center_axis',(0.,1.,0.));
#22422=DIRECTION('ref_axis',(1.,0.,0.));
#22423=DIRECTION('center_axis',(0.,1.,0.));
#22424=DIRECTION('ref_axis',(1.,0.,0.));
#22425=DIRECTION('',(0.,1.,0.));
#22426=DIRECTION('',(0.,1.,0.));
#22427=DIRECTION('center_axis',(-0.587785252292473,0.,0.809016994374947));
#22428=DIRECTION('ref_axis',(0.809016994374947,0.,0.587785252292473));
#22429=DIRECTION('',(0.809016994374947,0.,0.587785252292473));
#22430=DIRECTION('center_axis',(0.,1.,0.));
#22431=DIRECTION('ref_axis',(1.,0.,0.));
#22432=DIRECTION('center_axis',(0.,1.,0.));
#22433=DIRECTION('ref_axis',(1.,0.,0.));
#22434=DIRECTION('',(0.,1.,0.));
#22435=DIRECTION('',(0.,1.,0.));
#22436=DIRECTION('center_axis',(-0.707106781186548,0.,0.707106781186547));
#22437=DIRECTION('ref_axis',(0.707106781186547,0.,0.707106781186548));
#22438=DIRECTION('',(0.707106781186547,0.,0.707106781186548));
#22439=DIRECTION('center_axis',(0.,1.,0.));
#22440=DIRECTION('ref_axis',(1.,0.,0.));
#22441=DIRECTION('center_axis',(0.,1.,0.));
#22442=DIRECTION('ref_axis',(1.,0.,0.));
#22443=DIRECTION('',(0.,1.,0.));
#22444=DIRECTION('',(0.,1.,0.));
#22445=DIRECTION('center_axis',(-0.809016994374948,0.,0.587785252292473));
#22446=DIRECTION('ref_axis',(0.587785252292473,0.,0.809016994374948));
#22447=DIRECTION('',(0.587785252292473,0.,0.809016994374948));
#22448=DIRECTION('center_axis',(0.,1.,0.));
#22449=DIRECTION('ref_axis',(1.,0.,0.));
#22450=DIRECTION('center_axis',(0.,1.,0.));
#22451=DIRECTION('ref_axis',(1.,0.,0.));
#22452=DIRECTION('',(0.,1.,0.));
#22453=DIRECTION('',(0.,1.,0.));
#22454=DIRECTION('center_axis',(-0.891006524188368,0.,0.453990499739547));
#22455=DIRECTION('ref_axis',(0.453990499739547,0.,0.891006524188368));
#22456=DIRECTION('',(0.453990499739547,0.,0.891006524188368));
#22457=DIRECTION('center_axis',(0.,1.,0.));
#22458=DIRECTION('ref_axis',(1.,0.,0.));
#22459=DIRECTION('center_axis',(0.,1.,0.));
#22460=DIRECTION('ref_axis',(1.,0.,0.));
#22461=DIRECTION('',(0.,1.,0.));
#22462=DIRECTION('',(0.,1.,0.));
#22463=DIRECTION('center_axis',(-0.951056516295154,0.,0.309016994374947));
#22464=DIRECTION('ref_axis',(0.309016994374947,0.,0.951056516295154));
#22465=DIRECTION('',(0.309016994374947,0.,0.951056516295154));
#22466=DIRECTION('center_axis',(0.,1.,0.));
#22467=DIRECTION('ref_axis',(1.,0.,0.));
#22468=DIRECTION('center_axis',(0.,1.,0.));
#22469=DIRECTION('ref_axis',(1.,0.,0.));
#22470=DIRECTION('',(0.,1.,0.));
#22471=DIRECTION('',(0.,1.,0.));
#22472=DIRECTION('center_axis',(-0.987688340595138,0.,0.156434465040231));
#22473=DIRECTION('ref_axis',(0.156434465040231,0.,0.987688340595138));
#22474=DIRECTION('',(0.156434465040231,0.,0.987688340595138));
#22475=DIRECTION('center_axis',(0.,1.,0.));
#22476=DIRECTION('ref_axis',(1.,0.,0.));
#22477=DIRECTION('center_axis',(0.,1.,0.));
#22478=DIRECTION('ref_axis',(1.,0.,0.));
#22479=DIRECTION('',(0.,1.,0.));
#22480=DIRECTION('',(0.,1.,0.));
#22481=DIRECTION('center_axis',(-1.,0.,-1.22464679914735E-16));
#22482=DIRECTION('ref_axis',(-1.22464679914735E-16,0.,1.));
#22483=DIRECTION('',(-1.22464679914735E-16,0.,1.));
#22484=DIRECTION('center_axis',(0.,1.,0.));
#22485=DIRECTION('ref_axis',(1.,0.,0.));
#22486=DIRECTION('center_axis',(0.,1.,0.));
#22487=DIRECTION('ref_axis',(1.,0.,0.));
#22488=DIRECTION('',(0.,1.,0.));
#22489=DIRECTION('',(0.,1.,0.));
#22490=DIRECTION('center_axis',(-0.987688340595138,0.,-0.156434465040231));
#22491=DIRECTION('ref_axis',(-0.156434465040231,0.,0.987688340595138));
#22492=DIRECTION('',(-0.156434465040231,0.,0.987688340595138));
#22493=DIRECTION('center_axis',(0.,1.,0.));
#22494=DIRECTION('ref_axis',(1.,0.,0.));
#22495=DIRECTION('center_axis',(0.,1.,0.));
#22496=DIRECTION('ref_axis',(1.,0.,0.));
#22497=DIRECTION('',(0.,1.,0.));
#22498=DIRECTION('',(0.,1.,0.));
#22499=DIRECTION('center_axis',(-0.951056516295154,0.,-0.309016994374948));
#22500=DIRECTION('ref_axis',(-0.309016994374948,0.,0.951056516295154));
#22501=DIRECTION('',(-0.309016994374948,0.,0.951056516295154));
#22502=DIRECTION('center_axis',(0.,1.,0.));
#22503=DIRECTION('ref_axis',(1.,0.,0.));
#22504=DIRECTION('center_axis',(0.,1.,0.));
#22505=DIRECTION('ref_axis',(1.,0.,0.));
#22506=DIRECTION('',(0.,1.,0.));
#22507=DIRECTION('',(0.,1.,0.));
#22508=DIRECTION('center_axis',(-0.891006524188368,0.,-0.453990499739547));
#22509=DIRECTION('ref_axis',(-0.453990499739547,0.,0.891006524188368));
#22510=DIRECTION('',(-0.453990499739547,0.,0.891006524188368));
#22511=DIRECTION('center_axis',(0.,1.,0.));
#22512=DIRECTION('ref_axis',(1.,0.,0.));
#22513=DIRECTION('center_axis',(0.,1.,0.));
#22514=DIRECTION('ref_axis',(1.,0.,0.));
#22515=DIRECTION('',(0.,1.,0.));
#22516=DIRECTION('',(0.,1.,0.));
#22517=DIRECTION('center_axis',(-0.809016994374947,0.,-0.587785252292473));
#22518=DIRECTION('ref_axis',(-0.587785252292473,0.,0.809016994374947));
#22519=DIRECTION('',(-0.587785252292473,0.,0.809016994374947));
#22520=DIRECTION('center_axis',(0.,1.,0.));
#22521=DIRECTION('ref_axis',(1.,0.,0.));
#22522=DIRECTION('center_axis',(0.,1.,0.));
#22523=DIRECTION('ref_axis',(1.,0.,0.));
#22524=DIRECTION('',(0.,1.,0.));
#22525=DIRECTION('',(0.,1.,0.));
#22526=DIRECTION('center_axis',(-0.707106781186547,0.,-0.707106781186548));
#22527=DIRECTION('ref_axis',(-0.707106781186548,0.,0.707106781186547));
#22528=DIRECTION('',(-0.707106781186548,0.,0.707106781186547));
#22529=DIRECTION('center_axis',(0.,1.,0.));
#22530=DIRECTION('ref_axis',(1.,0.,0.));
#22531=DIRECTION('center_axis',(0.,1.,0.));
#22532=DIRECTION('ref_axis',(1.,0.,0.));
#22533=DIRECTION('',(0.,1.,0.));
#22534=DIRECTION('',(0.,1.,0.));
#22535=DIRECTION('center_axis',(-0.587785252292473,0.,-0.809016994374948));
#22536=DIRECTION('ref_axis',(-0.809016994374948,0.,0.587785252292473));
#22537=DIRECTION('',(-0.809016994374948,0.,0.587785252292473));
#22538=DIRECTION('center_axis',(0.,1.,0.));
#22539=DIRECTION('ref_axis',(1.,0.,0.));
#22540=DIRECTION('center_axis',(0.,1.,0.));
#22541=DIRECTION('ref_axis',(1.,0.,0.));
#22542=DIRECTION('',(0.,1.,0.));
#22543=DIRECTION('',(0.,1.,0.));
#22544=DIRECTION('center_axis',(-0.453990499739547,0.,-0.891006524188368));
#22545=DIRECTION('ref_axis',(-0.891006524188368,0.,0.453990499739547));
#22546=DIRECTION('',(-0.891006524188368,0.,0.453990499739547));
#22547=DIRECTION('center_axis',(0.,1.,0.));
#22548=DIRECTION('ref_axis',(1.,0.,0.));
#22549=DIRECTION('center_axis',(0.,1.,0.));
#22550=DIRECTION('ref_axis',(1.,0.,0.));
#22551=DIRECTION('',(0.,1.,0.));
#22552=DIRECTION('',(0.,1.,0.));
#22553=DIRECTION('center_axis',(-0.309016994374947,0.,-0.951056516295154));
#22554=DIRECTION('ref_axis',(-0.951056516295154,0.,0.309016994374947));
#22555=DIRECTION('',(-0.951056516295154,0.,0.309016994374947));
#22556=DIRECTION('center_axis',(0.,1.,0.));
#22557=DIRECTION('ref_axis',(1.,0.,0.));
#22558=DIRECTION('center_axis',(0.,1.,0.));
#22559=DIRECTION('ref_axis',(1.,0.,0.));
#22560=DIRECTION('',(0.,1.,0.));
#22561=DIRECTION('',(0.,1.,0.));
#22562=DIRECTION('center_axis',(-0.156434465040231,0.,-0.987688340595138));
#22563=DIRECTION('ref_axis',(-0.987688340595138,0.,0.156434465040231));
#22564=DIRECTION('',(-0.987688340595138,0.,0.156434465040231));
#22565=DIRECTION('center_axis',(0.,1.,0.));
#22566=DIRECTION('ref_axis',(1.,0.,0.));
#22567=DIRECTION('center_axis',(0.,1.,0.));
#22568=DIRECTION('ref_axis',(1.,0.,0.));
#22569=DIRECTION('',(0.,1.,0.));
#22570=DIRECTION('',(0.,1.,0.));
#22571=DIRECTION('center_axis',(6.12323399573677E-17,0.,-1.));
#22572=DIRECTION('ref_axis',(-1.,0.,-6.12323399573677E-17));
#22573=DIRECTION('',(-1.,0.,-6.12323399573677E-17));
#22574=DIRECTION('center_axis',(0.,1.,0.));
#22575=DIRECTION('ref_axis',(1.,0.,0.));
#22576=DIRECTION('center_axis',(0.,1.,0.));
#22577=DIRECTION('ref_axis',(1.,0.,0.));
#22578=DIRECTION('',(0.,1.,0.));
#22579=DIRECTION('',(0.,1.,0.));
#22580=DIRECTION('center_axis',(0.156434465040231,0.,-0.987688340595138));
#22581=DIRECTION('ref_axis',(-0.987688340595138,0.,-0.156434465040231));
#22582=DIRECTION('',(-0.987688340595138,0.,-0.156434465040231));
#22583=DIRECTION('center_axis',(0.,1.,0.));
#22584=DIRECTION('ref_axis',(1.,0.,0.));
#22585=DIRECTION('center_axis',(0.,1.,0.));
#22586=DIRECTION('ref_axis',(1.,0.,0.));
#22587=DIRECTION('',(0.,1.,0.));
#22588=DIRECTION('',(0.,1.,0.));
#22589=DIRECTION('center_axis',(0.309016994374948,0.,-0.951056516295154));
#22590=DIRECTION('ref_axis',(-0.951056516295154,0.,-0.309016994374948));
#22591=DIRECTION('',(-0.951056516295154,0.,-0.309016994374948));
#22592=DIRECTION('center_axis',(0.,1.,0.));
#22593=DIRECTION('ref_axis',(1.,0.,0.));
#22594=DIRECTION('center_axis',(0.,1.,0.));
#22595=DIRECTION('ref_axis',(1.,0.,0.));
#22596=DIRECTION('',(0.,1.,0.));
#22597=DIRECTION('',(0.,1.,0.));
#22598=DIRECTION('center_axis',(0.453990499739547,0.,-0.891006524188368));
#22599=DIRECTION('ref_axis',(-0.891006524188368,0.,-0.453990499739547));
#22600=DIRECTION('',(-0.891006524188368,0.,-0.453990499739547));
#22601=DIRECTION('center_axis',(0.,1.,0.));
#22602=DIRECTION('ref_axis',(1.,0.,0.));
#22603=DIRECTION('center_axis',(0.,1.,0.));
#22604=DIRECTION('ref_axis',(1.,0.,0.));
#22605=DIRECTION('',(0.,1.,0.));
#22606=DIRECTION('',(0.,1.,0.));
#22607=DIRECTION('center_axis',(0.587785252292473,0.,-0.809016994374947));
#22608=DIRECTION('ref_axis',(-0.809016994374947,0.,-0.587785252292473));
#22609=DIRECTION('',(-0.809016994374947,0.,-0.587785252292473));
#22610=DIRECTION('center_axis',(0.,1.,0.));
#22611=DIRECTION('ref_axis',(1.,0.,0.));
#22612=DIRECTION('center_axis',(0.,1.,0.));
#22613=DIRECTION('ref_axis',(1.,0.,0.));
#22614=DIRECTION('',(0.,1.,0.));
#22615=DIRECTION('',(0.,1.,0.));
#22616=DIRECTION('center_axis',(0.707106781186548,0.,-0.707106781186547));
#22617=DIRECTION('ref_axis',(-0.707106781186547,0.,-0.707106781186548));
#22618=DIRECTION('',(-0.707106781186547,0.,-0.707106781186548));
#22619=DIRECTION('center_axis',(0.,1.,0.));
#22620=DIRECTION('ref_axis',(1.,0.,0.));
#22621=DIRECTION('center_axis',(0.,1.,0.));
#22622=DIRECTION('ref_axis',(1.,0.,0.));
#22623=DIRECTION('',(0.,1.,0.));
#22624=DIRECTION('',(0.,1.,0.));
#22625=DIRECTION('center_axis',(0.809016994374947,0.,-0.587785252292473));
#22626=DIRECTION('ref_axis',(-0.587785252292473,0.,-0.809016994374947));
#22627=DIRECTION('',(-0.587785252292473,0.,-0.809016994374947));
#22628=DIRECTION('center_axis',(0.,1.,0.));
#22629=DIRECTION('ref_axis',(1.,0.,0.));
#22630=DIRECTION('center_axis',(0.,1.,0.));
#22631=DIRECTION('ref_axis',(1.,0.,0.));
#22632=DIRECTION('',(0.,1.,0.));
#22633=DIRECTION('',(0.,1.,0.));
#22634=DIRECTION('center_axis',(0.891006524188368,0.,-0.453990499739547));
#22635=DIRECTION('ref_axis',(-0.453990499739547,0.,-0.891006524188368));
#22636=DIRECTION('',(-0.453990499739547,0.,-0.891006524188368));
#22637=DIRECTION('center_axis',(0.,1.,0.));
#22638=DIRECTION('ref_axis',(1.,0.,0.));
#22639=DIRECTION('center_axis',(0.,1.,0.));
#22640=DIRECTION('ref_axis',(1.,0.,0.));
#22641=DIRECTION('',(0.,1.,0.));
#22642=DIRECTION('',(0.,1.,0.));
#22643=DIRECTION('center_axis',(0.951056516295154,0.,-0.309016994374947));
#22644=DIRECTION('ref_axis',(-0.309016994374947,0.,-0.951056516295154));
#22645=DIRECTION('',(-0.309016994374947,0.,-0.951056516295154));
#22646=DIRECTION('center_axis',(0.,1.,0.));
#22647=DIRECTION('ref_axis',(1.,0.,0.));
#22648=DIRECTION('center_axis',(0.,1.,0.));
#22649=DIRECTION('ref_axis',(1.,0.,0.));
#22650=DIRECTION('',(0.,1.,0.));
#22651=DIRECTION('center_axis',(0.987688340595138,0.,-0.156434465040231));
#22652=DIRECTION('ref_axis',(-0.156434465040231,0.,-0.987688340595138));
#22653=DIRECTION('',(-0.156434465040231,0.,-0.987688340595138));
#22654=DIRECTION('',(0.,1.,0.));
#22655=DIRECTION('center_axis',(0.,1.,0.));
#22656=DIRECTION('ref_axis',(1.,0.,0.));
#22657=DIRECTION('center_axis',(0.,1.,0.));
#22658=DIRECTION('ref_axis',(1.,0.,0.));
#22659=DIRECTION('',(0.,1.,0.));
#22660=DIRECTION('',(0.,1.,0.));
#22661=DIRECTION('center_axis',(1.,0.,0.));
#22662=DIRECTION('ref_axis',(0.,0.,-1.));
#22663=DIRECTION('',(0.,0.,-1.));
#22664=DIRECTION('center_axis',(0.,1.,0.));
#22665=DIRECTION('ref_axis',(1.,0.,0.));
#22666=DIRECTION('center_axis',(0.,1.,0.));
#22667=DIRECTION('ref_axis',(1.,0.,0.));
#22668=DIRECTION('center_axis',(0.,1.,0.));
#22669=DIRECTION('ref_axis',(1.,0.,0.));
#49605=CARTESIAN_POINT('',(0.,0.,0.));
#49606=CARTESIAN_POINT('Origin',(0.3,0.,0.));
#49607=CARTESIAN_POINT('',(0.3,2.2,-1.28));
#49608=CARTESIAN_POINT('',(0.3,2.2,-0.953939201416946));
#49609=CARTESIAN_POINT('',(0.3,2.2,0.));
#49610=CARTESIAN_POINT('',(0.3,-1.,-1.28));
#49611=CARTESIAN_POINT('',(0.3,0.,-1.28));
#49612=CARTESIAN_POINT('',(0.3,-1.,-0.953939201416946));
#49613=CARTESIAN_POINT('',(0.3,-1.,0.));
#49614=CARTESIAN_POINT('',(0.3,0.,-0.953939201416946));
#49615=CARTESIAN_POINT('Origin',(0.3,0.,-1.28));
#49616=CARTESIAN_POINT('',(-0.3,2.2,-1.28));
#49617=CARTESIAN_POINT('',(0.15,2.2,-1.28));
#49618=CARTESIAN_POINT('',(-0.3,-1.,-1.28));
#49619=CARTESIAN_POINT('',(-0.3,0.,-1.28));
#49620=CARTESIAN_POINT('',(0.15,-1.,-1.28));
#49621=CARTESIAN_POINT('Origin',(-0.3,0.,-1.28));
#49622=CARTESIAN_POINT('',(-0.3,2.2,-0.953939201416946));
#49623=CARTESIAN_POINT('',(-0.3,2.2,-0.64));
#49624=CARTESIAN_POINT('',(-0.3,-1.,-0.953939201416946));
#49625=CARTESIAN_POINT('',(-0.3,0.,-0.953939201416946));
#49626=CARTESIAN_POINT('',(-0.3,-1.,-0.64));
#49627=CARTESIAN_POINT('Origin',(0.,-1.,0.));
#49628=CARTESIAN_POINT('',(3.66661143271685,-1.,0.786422660831985));
#49629=CARTESIAN_POINT('',(3.62400312501245,-1.,0.963899035117249));
#49630=CARTESIAN_POINT('Origin',(0.,-1.,0.));
#49631=CARTESIAN_POINT('',(4.01728681790024,-1.,1.22531898815164));
#49632=CARTESIAN_POINT('Ctrl Pts',(3.62400312501245,-1.,0.963899035117249));
#49633=CARTESIAN_POINT('Ctrl Pts',(3.6240482887845,-1.,0.963880158555582));
#49634=CARTESIAN_POINT('Ctrl Pts',(3.62424461507588,-1.,0.963861297423241));
#49635=CARTESIAN_POINT('Ctrl Pts',(3.62489305727662,-1.,0.963957782642844));
#49636=CARTESIAN_POINT('Ctrl Pts',(3.62652618145335,-1.,0.964373850166458));
#49637=CARTESIAN_POINT('Ctrl Pts',(3.62988252139846,-1.,0.965395153165294));
#49638=CARTESIAN_POINT('Ctrl Pts',(3.63492122081143,-1.,0.967052554541386));
#49639=CARTESIAN_POINT('Ctrl Pts',(3.64113946505766,-1.,0.969195124675866));
#49640=CARTESIAN_POINT('Ctrl Pts',(3.64819756447455,-1.,0.971722122061341));
#49641=CARTESIAN_POINT('Ctrl Pts',(3.65571576735126,-1.,0.974519971354849));
#49642=CARTESIAN_POINT('Ctrl Pts',(3.66333049637475,-1.,0.977478312751618));
#49643=CARTESIAN_POINT('Ctrl Pts',(3.67074983340361,-1.,0.980505922458267));
#49644=CARTESIAN_POINT('Ctrl Pts',(3.67782408841715,-1.,0.98355079147042));
#49645=CARTESIAN_POINT('Ctrl Pts',(3.68455317926068,-1.,0.986602639863838));
#49646=CARTESIAN_POINT('Ctrl Pts',(3.69102682138846,-1.,0.989676715398559));
#49647=CARTESIAN_POINT('Ctrl Pts',(3.69738123415662,-1.,0.992802218332011));
#49648=CARTESIAN_POINT('Ctrl Pts',(3.70375282282138,-1.,0.996009819772518));
#49649=CARTESIAN_POINT('Ctrl Pts',(3.71022439713938,-1.,0.999317260756531));
#49650=CARTESIAN_POINT('Ctrl Pts',(3.71680667125118,-1.,1.00272423396822));
#49651=CARTESIAN_POINT('Ctrl Pts',(3.72346803750595,-1.,1.0062200073571));
#49652=CARTESIAN_POINT('Ctrl Pts',(3.73015276704426,-1.,1.00978798539496));
#49653=CARTESIAN_POINT('Ctrl Pts',(3.73680245055734,-1.,1.01341114319903));
#49654=CARTESIAN_POINT('Ctrl Pts',(3.74337942504959,-1.,1.01707794311079));
#49655=CARTESIAN_POINT('Ctrl Pts',(3.74987777155834,-1.,1.02078510487428));
#49656=CARTESIAN_POINT('Ctrl Pts',(3.75631037456194,-1.,1.0245342944466));
#49657=CARTESIAN_POINT('Ctrl Pts',(3.76270122291232,-1.,1.02833014458181));
#49658=CARTESIAN_POINT('Ctrl Pts',(3.76907609832522,-1.,1.0321778660492));
#49659=CARTESIAN_POINT('Ctrl Pts',(3.77545283140445,-1.,1.03608074678013));
#49660=CARTESIAN_POINT('Ctrl Pts',(3.78183535008192,-1.,1.04003862055804));
#49661=CARTESIAN_POINT('Ctrl Pts',(3.78821910787195,-1.,1.04404924374426));
#49662=CARTESIAN_POINT('Ctrl Pts',(3.79459440308793,-1.,1.04810913267641));
#49663=CARTESIAN_POINT('Ctrl Pts',(3.80095039790678,-1.,1.05221457990015));
#49664=CARTESIAN_POINT('Ctrl Pts',(3.80727913637784,-1.,1.05636266918643));
#49665=CARTESIAN_POINT('Ctrl Pts',(3.81357866117485,-1.,1.06055206187298));
#49666=CARTESIAN_POINT('Ctrl Pts',(3.81985083953012,-1.,1.06478244038931));
#49667=CARTESIAN_POINT('Ctrl Pts',(3.82609989967278,-1.,1.0690541318036));
#49668=CARTESIAN_POINT('Ctrl Pts',(3.83233071195145,-1.,1.0733676663346));
#49669=CARTESIAN_POINT('Ctrl Pts',(3.83854714117486,-1.,1.07772335353856));
#49670=CARTESIAN_POINT('Ctrl Pts',(3.84475048030615,-1.,1.08212087917986));
#49671=CARTESIAN_POINT('Ctrl Pts',(3.8509402522269,-1.,1.08655950846377));
#49672=CARTESIAN_POINT('Ctrl Pts',(3.85711487933911,-1.,1.09103825516288));
#49673=CARTESIAN_POINT('Ctrl Pts',(3.86327241021242,-1.,1.09555606505012));
#49674=CARTESIAN_POINT('Ctrl Pts',(3.86941120134872,-1.,1.10011198761203));
#49675=CARTESIAN_POINT('Ctrl Pts',(3.87553067187566,-1.,1.10470536603303));
#49676=CARTESIAN_POINT('Ctrl Pts',(3.88163105531791,-1.,1.10933577224029));
#49677=CARTESIAN_POINT('Ctrl Pts',(3.88771308285229,-1.,1.11400292434447));
#49678=CARTESIAN_POINT('Ctrl Pts',(3.89377768340362,-1.,1.11870660794609));
#49679=CARTESIAN_POINT('Ctrl Pts',(3.89982569749978,-1.,1.12344660099029));
#49680=CARTESIAN_POINT('Ctrl Pts',(3.90585753318622,-1.,1.12822258281518));
#49681=CARTESIAN_POINT('Ctrl Pts',(3.91187321145495,-1.,1.13303414693849));
#49682=CARTESIAN_POINT('Ctrl Pts',(3.91787251936688,-1.,1.13788084225511));
#49683=CARTESIAN_POINT('Ctrl Pts',(3.92385513133937,-1.,1.14276220561575));
#49684=CARTESIAN_POINT('Ctrl Pts',(3.92982073294334,-1.,1.14767779451147));
#49685=CARTESIAN_POINT('Ctrl Pts',(3.9357691705651,-1.,1.15262722716391));
#49686=CARTESIAN_POINT('Ctrl Pts',(3.94170046685542,-1.,1.15761018341061));
#49687=CARTESIAN_POINT('Ctrl Pts',(3.9476147478092,-1.,1.16262637999261));
#49688=CARTESIAN_POINT('Ctrl Pts',(3.95351219510062,-1.,1.16767555244495));
#49689=CARTESIAN_POINT('Ctrl Pts',(3.95939299213164,-1.,1.17275743590327));
#49690=CARTESIAN_POINT('Ctrl Pts',(3.96525726357682,-1.,1.17787174135446));
#49691=CARTESIAN_POINT('Ctrl Pts',(3.9711050516465,-1.,1.18301815039596));
#49692=CARTESIAN_POINT('Ctrl Pts',(3.97693634766926,-1.,1.18819633715285));
#49693=CARTESIAN_POINT('Ctrl Pts',(3.98275111052015,-1.,1.19340598349307));
#49694=CARTESIAN_POINT('Ctrl Pts',(3.98854928957287,-1.,1.19864679609596));
#49695=CARTESIAN_POINT('Ctrl Pts',(3.99433084800649,-1.,1.2039185237544));
#49696=CARTESIAN_POINT('Ctrl Pts',(4.00009577952534,-1.,1.20922097030107));
#49697=CARTESIAN_POINT('Ctrl Pts',(4.00584409524937,-1.,1.21455398918813));
#49698=CARTESIAN_POINT('Ctrl Pts',(4.01042947142681,-1.,1.21884478244983));
#49699=CARTESIAN_POINT('Ctrl Pts',(4.01386104434674,-1.,1.22207656456199));
#49700=CARTESIAN_POINT('Ctrl Pts',(4.0161454457032,-1.,1.22423716681447));
#49701=CARTESIAN_POINT('Ctrl Pts',(4.01728681790024,-1.,1.22531898815164));
#49702=CARTESIAN_POINT('',(3.97027773754922,-1.,1.36999806084573));
#49703=CARTESIAN_POINT('',(4.01728681790024,-1.,1.22531898815164));
#49704=CARTESIAN_POINT('',(3.4984457533445,-1.,1.35032489087101));
#49705=CARTESIAN_POINT('Ctrl Pts',(3.97027773754922,-1.,1.36999806084573));
#49706=CARTESIAN_POINT('Ctrl Pts',(3.9687184694131,-1.,1.37020239094614));
#49707=CARTESIAN_POINT('Ctrl Pts',(3.96560037974645,-1.,1.37060761745635));
#49708=CARTESIAN_POINT('Ctrl Pts',(3.96092458506535,-1.,1.3712051561502));
#49709=CARTESIAN_POINT('Ctrl Pts',(3.95469287280914,-1.,1.37198126432386));
#49710=CARTESIAN_POINT('Ctrl Pts',(3.94690771785133,-1.,1.37291699202807));
#49711=CARTESIAN_POINT('Ctrl Pts',(3.93912709040818,-1.,1.37381821967165));
#49712=CARTESIAN_POINT('Ctrl Pts',(3.93135106761844,-1.,1.37468482215751));
#49713=CARTESIAN_POINT('Ctrl Pts',(3.92357976987672,-1.,1.37551664448242));
#49714=CARTESIAN_POINT('Ctrl Pts',(3.91581337462644,-1.,1.37631350505797));
#49715=CARTESIAN_POINT('Ctrl Pts',(3.90805209523486,-1.,1.3770751963402));
#49716=CARTESIAN_POINT('Ctrl Pts',(3.90029615196727,-1.,1.37780148512792));
#49717=CARTESIAN_POINT('Ctrl Pts',(3.89254574338496,-1.,1.3784921128802));
#49718=CARTESIAN_POINT('Ctrl Pts',(3.88480102249277,-1.,1.37914679719383));
#49719=CARTESIAN_POINT('Ctrl Pts',(3.87706205830532,-1.,1.37976523097073));
#49720=CARTESIAN_POINT('Ctrl Pts',(3.86932885813068,-1.,1.38034709213014));
#49721=CARTESIAN_POINT('Ctrl Pts',(3.86160143043959,-1.,1.3808920599299));
#49722=CARTESIAN_POINT('Ctrl Pts',(3.85387983979481,-1.,1.3813998311505));
#49723=CARTESIAN_POINT('Ctrl Pts',(3.84616425605764,-1.,1.38187013346109));
#49724=CARTESIAN_POINT('Ctrl Pts',(3.83845502790746,-1.,1.38230274828822));
#49725=CARTESIAN_POINT('Ctrl Pts',(3.8307526698229,-1.,1.38269750245138));
#49726=CARTESIAN_POINT('Ctrl Pts',(3.82305771743829,-1.,1.38305421262763));
#49727=CARTESIAN_POINT('Ctrl Pts',(3.81537060817811,-1.,1.38337263902782));
#49728=CARTESIAN_POINT('Ctrl Pts',(3.80769156398411,-1.,1.3836524404622));
#49729=CARTESIAN_POINT('Ctrl Pts',(3.80002044322111,-1.,1.38389311766682));
#49730=CARTESIAN_POINT('Ctrl Pts',(3.79235669640841,-1.,1.38409399694566));
#49731=CARTESIAN_POINT('Ctrl Pts',(3.78469969805082,-1.,1.38425435883756));
#49732=CARTESIAN_POINT('Ctrl Pts',(3.77704902230418,-1.,1.38437354551428));
#49733=CARTESIAN_POINT('Ctrl Pts',(3.76940473185779,-1.,1.38445107339518));
#49734=CARTESIAN_POINT('Ctrl Pts',(3.76176768271367,-1.,1.3844867525335));
#49735=CARTESIAN_POINT('Ctrl Pts',(3.7541397631875,-1.,1.38448077997163));
#49736=CARTESIAN_POINT('Ctrl Pts',(3.74652317167876,-1.,1.38443344984394));
#49737=CARTESIAN_POINT('Ctrl Pts',(3.73891976418104,-1.,1.38434489156458));
#49738=CARTESIAN_POINT('Ctrl Pts',(3.73133035859282,-1.,1.38421479111531));
#49739=CARTESIAN_POINT('Ctrl Pts',(3.72375409358803,-1.,1.3840421342895));
#49740=CARTESIAN_POINT('Ctrl Pts',(3.7161876605181,-1.,1.38382489984586));
#49741=CARTESIAN_POINT('Ctrl Pts',(3.70862680753347,-1.,1.38356065402124));
#49742=CARTESIAN_POINT('Ctrl Pts',(3.701067921679,-1.,1.38324717612865));
#49743=CARTESIAN_POINT('Ctrl Pts',(3.69350967899526,-1.,1.38288311171651));
#49744=CARTESIAN_POINT('Ctrl Pts',(3.68595444983837,-1.,1.38246852827182));
#49745=CARTESIAN_POINT('Ctrl Pts',(3.67841038482414,-1.,1.3820057429062));
#49746=CARTESIAN_POINT('Ctrl Pts',(3.67088843112262,-1.,1.38149812653868));
#49747=CARTESIAN_POINT('Ctrl Pts',(3.66339848520857,-1.,1.38094856333552));
#49748=CARTESIAN_POINT('Ctrl Pts',(3.6559455440439,-1.,1.38035791051213));
#49749=CARTESIAN_POINT('Ctrl Pts',(3.64852652756456,-1.,1.37972372481603));
#49750=CARTESIAN_POINT('Ctrl Pts',(3.64112507791141,-1.,1.37903818567359));
#49751=CARTESIAN_POINT('Ctrl Pts',(3.63371727442486,-1.,1.37829035457339));
#49752=CARTESIAN_POINT('Ctrl Pts',(3.62628098665145,-1.,1.37746987919881));
#49753=CARTESIAN_POINT('Ctrl Pts',(3.6188048116042,-1.,1.37657053403107));
#49754=CARTESIAN_POINT('Ctrl Pts',(3.61129546591064,-1.,1.37559314436634));
#49755=CARTESIAN_POINT('Ctrl Pts',(3.60379020123988,-1.,1.37455051379623));
#49756=CARTESIAN_POINT('Ctrl Pts',(3.59634627869048,-1.,1.37346320103157));
#49757=CARTESIAN_POINT('Ctrl Pts',(3.58901853846365,-1.,1.37235053660976));
#49758=CARTESIAN_POINT('Ctrl Pts',(3.58183885982715,-1.,1.37122241663062));
#49759=CARTESIAN_POINT('Ctrl Pts',(3.57479875549486,-1.,1.37007229485659));
#49760=CARTESIAN_POINT('Ctrl Pts',(3.5678208030466,-1.,1.36886584973389));
#49761=CARTESIAN_POINT('Ctrl Pts',(3.56077662028649,-1.,1.36754771771233));
#49762=CARTESIAN_POINT('Ctrl Pts',(3.55353883995949,-1.,1.3660614545677));
#49763=CARTESIAN_POINT('Ctrl Pts',(3.54602591832973,-1.,1.36436666257598));
#49764=CARTESIAN_POINT('Ctrl Pts',(3.53824396424961,-1.,1.36245507339307));
#49765=CARTESIAN_POINT('Ctrl Pts',(3.530344649616,-1.,1.36037259643734));
#49766=CARTESIAN_POINT('Ctrl Pts',(3.52261776116748,-1.,1.35821701528836));
#49767=CARTESIAN_POINT('Ctrl Pts',(3.51542230699556,-1.,1.35611275237152));
#49768=CARTESIAN_POINT('Ctrl Pts',(3.50913227059999,-1.,1.35419113575956));
#49769=CARTESIAN_POINT('Ctrl Pts',(3.50408168106261,-1.,1.35257032843486));
#49770=CARTESIAN_POINT('Ctrl Pts',(3.5007660381649,-1.,1.35142377279517));
#49771=CARTESIAN_POINT('Ctrl Pts',(3.49920025459723,-1.,1.35080045218587));
#49772=CARTESIAN_POINT('Ctrl Pts',(3.49861894124827,-1.,1.35049736560527));
#49773=CARTESIAN_POINT('Ctrl Pts',(3.49847119623846,-1.,1.35036670892966));
#49774=CARTESIAN_POINT('Ctrl Pts',(3.4984457533445,-1.,1.35032489087101));
#49775=CARTESIAN_POINT('',(3.42859860294378,-1.,1.51895082866166));
#49776=CARTESIAN_POINT('Origin',(0.,-1.,0.));
#49777=CARTESIAN_POINT('',(3.77614523045147,-1.,1.83867539237861));
#49778=CARTESIAN_POINT('Ctrl Pts',(3.42859860294378,-1.,1.51895082866166));
#49779=CARTESIAN_POINT('Ctrl Pts',(3.42864616361967,-1.,1.51893924967231));
#49780=CARTESIAN_POINT('Ctrl Pts',(3.42884302333978,-1.,1.51895133295017));
#49781=CARTESIAN_POINT('Ctrl Pts',(3.42946838852728,-1.,1.51914806898539));
#49782=CARTESIAN_POINT('Ctrl Pts',(3.4310163189349,-1.,1.5198144909343));
#49783=CARTESIAN_POINT('Ctrl Pts',(3.43417156977749,-1.,1.52134826724227));
#49784=CARTESIAN_POINT('Ctrl Pts',(3.43888895974182,-1.,1.52377348950429));
#49785=CARTESIAN_POINT('Ctrl Pts',(3.44469547527,-1.,1.52686242875717));
#49786=CARTESIAN_POINT('Ctrl Pts',(3.45127136828667,-1.,1.530462444618));
#49787=CARTESIAN_POINT('Ctrl Pts',(3.45825932955273,-1.,1.53440195378902));
#49788=CARTESIAN_POINT('Ctrl Pts',(3.46531752207222,-1.,1.53851507915533));
#49789=CARTESIAN_POINT('Ctrl Pts',(3.47217189224576,-1.,1.54266605398152));
#49790=CARTESIAN_POINT('Ctrl Pts',(3.47868272898599,-1.,1.54678009290207));
#49791=CARTESIAN_POINT('Ctrl Pts',(3.48485155928414,-1.,1.55084702970382));
#49792=CARTESIAN_POINT('Ctrl Pts',(3.49076460877317,-1.,1.5548959590107));
#49793=CARTESIAN_POINT('Ctrl Pts',(3.49655185179623,-1.,1.55897703097859));
#49794=CARTESIAN_POINT('Ctrl Pts',(3.50234321621607,-1.,1.56314187758689));
#49795=CARTESIAN_POINT('Ctrl Pts',(3.50821771695427,-1.,1.56742097575041));
#49796=CARTESIAN_POINT('Ctrl Pts',(3.51418598431733,-1.,1.57181569799774));
#49797=CARTESIAN_POINT('Ctrl Pts',(3.52021847865961,-1.,1.5763104998818));
#49798=CARTESIAN_POINT('Ctrl Pts',(3.52626275334899,-1.,1.58088027227856));
#49799=CARTESIAN_POINT('Ctrl Pts',(3.53226378147068,-1.,1.58549906268083));
#49800=CARTESIAN_POINT('Ctrl Pts',(3.53818616861045,-1.,1.59014958368725));
#49801=CARTESIAN_POINT('Ctrl Pts',(3.544024581823,-1.,1.5948276694975));
#49802=CARTESIAN_POINT('Ctrl Pts',(3.54979148634426,-1.,1.59953698113444));
#49803=CARTESIAN_POINT('Ctrl Pts',(3.55550985096117,-1.,1.60428584699848));
#49804=CARTESIAN_POINT('Ctrl Pts',(3.56120432482986,-1.,1.60908344685459));
#49805=CARTESIAN_POINT('Ctrl Pts',(3.56689200468404,-1.,1.61393581747522));
#49806=CARTESIAN_POINT('Ctrl Pts',(3.57257679609826,-1.,1.61884340915412));
#49807=CARTESIAN_POINT('Ctrl Pts',(3.57825455954405,-1.,1.62380329464851));
#49808=CARTESIAN_POINT('Ctrl Pts',(3.5839162577435,-1.,1.62881051550748));
#49809=CARTESIAN_POINT('Ctrl Pts',(3.58955176627876,-1.,1.63385971451259));
#49810=CARTESIAN_POINT('Ctrl Pts',(3.59515368334887,-1.,1.63894676675349));
#49811=CARTESIAN_POINT('Ctrl Pts',(3.6007202851384,-1.,1.6440700438558));
#49812=CARTESIAN_POINT('Ctrl Pts',(3.60625346556992,-1.,1.64922952425833));
#49813=CARTESIAN_POINT('Ctrl Pts',(3.61175734965129,-1.,1.65442619244327));
#49814=CARTESIAN_POINT('Ctrl Pts',(3.61723666482457,-1.,1.65966133399186));
#49815=CARTESIAN_POINT('Ctrl Pts',(3.62269517989104,-1.,1.66493585923853));
#49816=CARTESIAN_POINT('Ctrl Pts',(3.62813422105257,-1.,1.67024966008037));
#49817=CARTESIAN_POINT('Ctrl Pts',(3.63355343201211,-1.,1.67560193613145));
#49818=CARTESIAN_POINT('Ctrl Pts',(3.63895140887443,-1.,1.68099146651577));
#49819=CARTESIAN_POINT('Ctrl Pts',(3.64432638915199,-1.,1.68641690471455));
#49820=CARTESIAN_POINT('Ctrl Pts',(3.64967689827393,-1.,1.691877054817));
#49821=CARTESIAN_POINT('Ctrl Pts',(3.65500246526798,-1.,1.69737117722559));
#49822=CARTESIAN_POINT('Ctrl Pts',(3.6603033877491,-1.,1.70289888566904));
#49823=CARTESIAN_POINT('Ctrl Pts',(3.6655804319893,-1.,1.70846001610983));
#49824=CARTESIAN_POINT('Ctrl Pts',(3.67083454901629,-1.,1.71405450210392));
#49825=CARTESIAN_POINT('Ctrl Pts',(3.67606660374665,-1.,1.71968225581787));
#49826=CARTESIAN_POINT('Ctrl Pts',(3.68127704936472,-1.,1.72534302437003));
#49827=CARTESIAN_POINT('Ctrl Pts',(3.68646597019188,-1.,1.73103640956647));
#49828=CARTESIAN_POINT('Ctrl Pts',(3.69163322647906,-1.,1.73676193254493));
#49829=CARTESIAN_POINT('Ctrl Pts',(3.6967785691046,-1.,1.74251908492589));
#49830=CARTESIAN_POINT('Ctrl Pts',(3.70190175673422,-1.,1.74830738046092));
#49831=CARTESIAN_POINT('Ctrl Pts',(3.70700269736876,-1.,1.75412641804148));
#49832=CARTESIAN_POINT('Ctrl Pts',(3.71208146346454,-1.,1.75997588499021));
#49833=CARTESIAN_POINT('Ctrl Pts',(3.71713822377675,-1.,1.76585552124549));
#49834=CARTESIAN_POINT('Ctrl Pts',(3.72217319911429,-1.,1.77176509401846));
#49835=CARTESIAN_POINT('Ctrl Pts',(3.72718661205504,-1.,1.77770437039606));
#49836=CARTESIAN_POINT('Ctrl Pts',(3.73217863095022,-1.,1.78367308442682));
#49837=CARTESIAN_POINT('Ctrl Pts',(3.73714934729962,-1.,1.78967092823139));
#49838=CARTESIAN_POINT('Ctrl Pts',(3.74209880351667,-1.,1.79569757859041));
#49839=CARTESIAN_POINT('Ctrl Pts',(3.74702700874954,-1.,1.80175271485519));
#49840=CARTESIAN_POINT('Ctrl Pts',(3.75193395888069,-1.,1.80783603939662));
#49841=CARTESIAN_POINT('Ctrl Pts',(3.75681965683995,-1.,1.81394729834032));
#49842=CARTESIAN_POINT('Ctrl Pts',(3.76168412709652,-1.,1.82008629694924));
#49843=CARTESIAN_POINT('Ctrl Pts',(3.76652740355856,-1.,1.82625289221933));
#49844=CARTESIAN_POINT('Ctrl Pts',(3.77038509819777,-1.,1.83120816956515));
#49845=CARTESIAN_POINT('Ctrl Pts',(3.77326886065484,-1.,1.83493697935064));
#49846=CARTESIAN_POINT('Ctrl Pts',(3.77518714458232,-1.,1.83742834010821));
#49847=CARTESIAN_POINT('Ctrl Pts',(3.77614523045147,-1.,1.83867539237861));
#49848=CARTESIAN_POINT('',(3.70708211654725,-1.,1.97421938526992));
#49849=CARTESIAN_POINT('',(3.77614523045147,-1.,1.83867539237861));
#49850=CARTESIAN_POINT('',(3.24413672884902,-1.,1.88097764062542));
#49851=CARTESIAN_POINT('Ctrl Pts',(3.70708211654725,-1.,1.97421938526992));
#49852=CARTESIAN_POINT('Ctrl Pts',(3.7055100813194,-1.,1.974177276451));
#49853=CARTESIAN_POINT('Ctrl Pts',(3.70236698911837,-1.,1.97408973726149));
#49854=CARTESIAN_POINT('Ctrl Pts',(3.69765528558292,-1.,1.97394846382289));
#49855=CARTESIAN_POINT('Ctrl Pts',(3.69137888597855,-1.,1.97374016224397));
#49856=CARTESIAN_POINT('Ctrl Pts',(3.68354319913416,-1.,1.97344650303631));
#49857=CARTESIAN_POINT('Ctrl Pts',(3.67571738106175,-1.,1.97311947678035));
#49858=CARTESIAN_POINT('Ctrl Pts',(3.66790152751984,-1.,1.9727589719863));
#49859=CARTESIAN_POINT('Ctrl Pts',(3.66009578166865,-1.,1.97236485439317));
#49860=CARTESIAN_POINT('Ctrl Pts',(3.65230034717364,-1.,1.97193697240645));
#49861=CARTESIAN_POINT('Ctrl Pts',(3.64451546724221,-1.,1.97147515441539));
#49862=CARTESIAN_POINT('Ctrl Pts',(3.63674139590853,-1.,1.97097920454698));
#49863=CARTESIAN_POINT('Ctrl Pts',(3.62897836973397,-1.,1.97044889850518));
#49864=CARTESIAN_POINT('Ctrl Pts',(3.62122658401722,-1.,1.96988398129888));
#49865=CARTESIAN_POINT('Ctrl Pts',(3.61348615496393,-1.,1.96928416040712));
#49866=CARTESIAN_POINT('Ctrl Pts',(3.60575714017676,-1.,1.96864911885775));
#49867=CARTESIAN_POINT('Ctrl Pts',(3.59803959819725,-1.,1.96797854118257));
#49868=CARTESIAN_POINT('Ctrl Pts',(3.5903336402273,-1.,1.96727213799507));
#49869=CARTESIAN_POINT('Ctrl Pts',(3.58263947663884,-1.,1.9665296668894));
#49870=CARTESIAN_POINT('Ctrl Pts',(3.57495748601088,-1.,1.96575096652857));
#49871=CARTESIAN_POINT('Ctrl Pts',(3.56728820357933,-1.,1.96493594634643));
#49872=CARTESIAN_POINT('Ctrl Pts',(3.55963218706201,-1.,1.96408450906868));
#49873=CARTESIAN_POINT('Ctrl Pts',(3.55198990600929,-1.,1.96319648628667));
#49874=CARTESIAN_POINT('Ctrl Pts',(3.54436163300425,-1.,1.96227157573058));
#49875=CARTESIAN_POINT('Ctrl Pts',(3.53674730625759,-1.,1.96130926212661));
#49876=CARTESIAN_POINT('Ctrl Pts',(3.52914648844289,-1.,1.96030879411534));
#49877=CARTESIAN_POINT('Ctrl Pts',(3.52155867431438,-1.,1.95926936324436));
#49878=CARTESIAN_POINT('Ctrl Pts',(3.51398354617772,-1.,1.95819025316768));
#49879=CARTESIAN_POINT('Ctrl Pts',(3.50642124159913,-1.,1.95707099606514));
#49880=CARTESIAN_POINT('Ctrl Pts',(3.49887263575602,-1.,1.9559115382367));
#49881=CARTESIAN_POINT('Ctrl Pts',(3.49133956289154,-1.,1.95471236969653));
#49882=CARTESIAN_POINT('Ctrl Pts',(3.48382414832648,-1.,1.95347412486316));
#49883=CARTESIAN_POINT('Ctrl Pts',(3.47632820495926,-1.,1.95219722189878));
#49884=CARTESIAN_POINT('Ctrl Pts',(3.4688525897419,-1.,1.95088147859876));
#49885=CARTESIAN_POINT('Ctrl Pts',(3.46139661060959,-1.,1.94952575850196));
#49886=CARTESIAN_POINT('Ctrl Pts',(3.45395731584051,-1.,1.94812754766524));
#49887=CARTESIAN_POINT('Ctrl Pts',(3.44653088665685,-1.,1.94668377715332));
#49888=CARTESIAN_POINT('Ctrl Pts',(3.43911410197693,-1.,1.94519168842883));
#49889=CARTESIAN_POINT('Ctrl Pts',(3.43170586602436,-1.,1.94364973660285));
#49890=CARTESIAN_POINT('Ctrl Pts',(3.42430850941497,-1.,1.94205835913692));
#49891=CARTESIAN_POINT('Ctrl Pts',(3.41692971994082,-1.,1.94042111965237));
#49892=CARTESIAN_POINT('Ctrl Pts',(3.40957978266622,-1.,1.93874306008132));
#49893=CARTESIAN_POINT('Ctrl Pts',(3.40226802104093,-1.,1.93702857723089));
#49894=CARTESIAN_POINT('Ctrl Pts',(3.39499923640789,-1.,1.93527929945982));
#49895=CARTESIAN_POINT('Ctrl Pts',(3.38777076883267,-1.,1.93349233176794));
#49896=CARTESIAN_POINT('Ctrl Pts',(3.38056768525577,-1.,1.93165739093292));
#49897=CARTESIAN_POINT('Ctrl Pts',(3.37336807068078,-1.,1.92975993109897));
#49898=CARTESIAN_POINT('Ctrl Pts',(3.36615168657597,-1.,1.92778626543803));
#49899=CARTESIAN_POINT('Ctrl Pts',(3.35890824422976,-1.,1.92572846125763));
#49900=CARTESIAN_POINT('Ctrl Pts',(3.35164424847206,-1.,1.92358838440518));
#49901=CARTESIAN_POINT('Ctrl Pts',(3.34439448941915,-1.,1.92138450828378));
#49902=CARTESIAN_POINT('Ctrl Pts',(3.33721230709948,-1.,1.91914609610173));
#49903=CARTESIAN_POINT('Ctrl Pts',(3.33014884257812,-1.,1.91690081930297));
#49904=CARTESIAN_POINT('Ctrl Pts',(3.32323403454507,-1.,1.91466343916612));
#49905=CARTESIAN_POINT('Ctrl Pts',(3.31646052426395,-1.,1.91242616234459));
#49906=CARTESIAN_POINT('Ctrl Pts',(3.30975721158694,-1.,1.91014297830502));
#49907=CARTESIAN_POINT('Ctrl Pts',(3.30300595568341,-1.,1.90773912171424));
#49908=CARTESIAN_POINT('Ctrl Pts',(3.29608978722258,-1.,1.9051389186417));
#49909=CARTESIAN_POINT('Ctrl Pts',(3.28893448600364,-1.,1.9022897124757));
#49910=CARTESIAN_POINT('Ctrl Pts',(3.28154737912287,-1.,1.89918429230425));
#49911=CARTESIAN_POINT('Ctrl Pts',(3.27407108932908,-1.,1.89589172903662));
#49912=CARTESIAN_POINT('Ctrl Pts',(3.2667765388833,-1.,1.89255393500769));
#49913=CARTESIAN_POINT('Ctrl Pts',(3.2599988519361,-1.,1.88934996203508));
#49914=CARTESIAN_POINT('Ctrl Pts',(3.25408686339298,-1.,1.88646802523372));
#49915=CARTESIAN_POINT('Ctrl Pts',(3.24935200512055,-1.,1.88407708646435));
#49916=CARTESIAN_POINT('Ctrl Pts',(3.24625654410705,-1.,1.88242596600422));
#49917=CARTESIAN_POINT('Ctrl Pts',(3.24480754675942,-1.,1.88156537699118));
#49918=CARTESIAN_POINT('Ctrl Pts',(3.24428080352952,-1.,1.88117508446657));
#49919=CARTESIAN_POINT('Ctrl Pts',(3.2441553167131,-1.,1.88102292397987));
#49920=CARTESIAN_POINT('Ctrl Pts',(3.24413672884902,-1.,1.88097764062542));
#49921=CARTESIAN_POINT('',(3.14877060440425,-1.,2.03660101169564));
#49922=CARTESIAN_POINT('Origin',(0.,-1.,0.));
#49923=CARTESIAN_POINT('',(3.44202241512147,-1.,2.40675750623143));
#49924=CARTESIAN_POINT('Ctrl Pts',(3.14877060440425,-1.,2.03660101169564));
#49925=CARTESIAN_POINT('Ctrl Pts',(3.1488193908823,-1.,2.03659701539175));
#49926=CARTESIAN_POINT('Ctrl Pts',(3.14901193669147,-1.,2.03663974554941));
#49927=CARTESIAN_POINT('Ctrl Pts',(3.14959882629936,-1.,2.03693188810614));
#49928=CARTESIAN_POINT('Ctrl Pts',(3.15102344775396,-1.,2.03783225496023));
#49929=CARTESIAN_POINT('Ctrl Pts',(3.1538999167466,-1.,2.03984073791432));
#49930=CARTESIAN_POINT('Ctrl Pts',(3.15817983946525,-1.,2.04297406404132));
#49931=CARTESIAN_POINT('Ctrl Pts',(3.16343165059235,-1.,2.0469333124766));
#49932=CARTESIAN_POINT('Ctrl Pts',(3.16936341689859,-1.,2.05151770247452));
#49933=CARTESIAN_POINT('Ctrl Pts',(3.17564906975592,-1.,2.05650186773279));
#49934=CARTESIAN_POINT('Ctrl Pts',(3.18197692964677,-1.,2.06166849827143));
#49935=CARTESIAN_POINT('Ctrl Pts',(3.18809755562297,-1.,2.06684062744065));
#49936=CARTESIAN_POINT('Ctrl Pts',(3.19388465568113,-1.,2.07192253497765));
#49937=CARTESIAN_POINT('Ctrl Pts',(3.19934132835879,-1.,2.0769044187063));
#49938=CARTESIAN_POINT('Ctrl Pts',(3.20454818630635,-1.,2.08182850370816));
#49939=CARTESIAN_POINT('Ctrl Pts',(3.20962575845433,-1.,2.08676465517435));
#49940=CARTESIAN_POINT('Ctrl Pts',(3.2146942960168,-1.,2.0917841946046));
#49941=CARTESIAN_POINT('Ctrl Pts',(3.21982707347067,-1.,2.09692958434933));
#49942=CARTESIAN_POINT('Ctrl Pts',(3.22503437553496,-1.,2.10220384298534));
#49943=CARTESIAN_POINT('Ctrl Pts',(3.23028945793334,-1.,2.1075869964248));
#49944=CARTESIAN_POINT('Ctrl Pts',(3.23554444767115,-1.,2.11304604021784));
#49945=CARTESIAN_POINT('Ctrl Pts',(3.24074905517282,-1.,2.11854673326972));
#49946=CARTESIAN_POINT('Ctrl Pts',(3.24587102613347,-1.,2.12406646410943));
#49947=CARTESIAN_POINT('Ctrl Pts',(3.25090574493994,-1.,2.1296002839681));
#49948=CARTESIAN_POINT('Ctrl Pts',(3.25586495065027,-1.,2.13515375878786));
#49949=CARTESIAN_POINT('Ctrl Pts',(3.26077002641868,-1.,2.14073870754258));
#49950=CARTESIAN_POINT('Ctrl Pts',(3.26564388189764,-1.,2.14636805295663));
#49951=CARTESIAN_POINT('Ctrl Pts',(3.27050245897244,-1.,2.15205043199818));
#49952=CARTESIAN_POINT('Ctrl Pts',(3.27534954469206,-1.,2.15778690038359));
#49953=CARTESIAN_POINT('Ctrl Pts',(3.28018150841414,-1.,2.16357391934434));
#49954=CARTESIAN_POINT('Ctrl Pts',(3.2849901997973,-1.,2.16940517773459));
#49955=CARTESIAN_POINT('Ctrl Pts',(3.28976645712566,-1.,2.17527380048422));
#49956=CARTESIAN_POINT('Ctrl Pts',(3.29450361500484,-1.,2.18117455557062));
#49957=CARTESIAN_POINT('Ctrl Pts',(3.29920022557635,-1.,2.18710556500325));
#49958=CARTESIAN_POINT('Ctrl Pts',(3.30385816281831,-1.,2.19306710376112));
#49959=CARTESIAN_POINT('Ctrl Pts',(3.30848134694596,-1.,2.19906078949925));
#49960=CARTESIAN_POINT('Ctrl Pts',(3.3130742460895,-1.,2.20508863150608));
#49961=CARTESIAN_POINT('Ctrl Pts',(3.31764044024231,-1.,2.21115211847872));
#49962=CARTESIAN_POINT('Ctrl Pts',(3.32218125618955,-1.,2.21725135110889));
#49963=CARTESIAN_POINT('Ctrl Pts',(3.32669646722871,-1.,2.22338548312759));
#49964=CARTESIAN_POINT('Ctrl Pts',(3.33118487773593,-1.,2.22955308907221));
#49965=CARTESIAN_POINT('Ctrl Pts',(3.33564495756478,-1.,2.2357525632881));
#49966=CARTESIAN_POINT('Ctrl Pts',(3.34007543738044,-1.,2.24198249391437));
#49967=CARTESIAN_POINT('Ctrl Pts',(3.34447596770768,-1.,2.24824207678288));
#49968=CARTESIAN_POINT('Ctrl Pts',(3.34884690292342,-1.,2.25453097693524));
#49969=CARTESIAN_POINT('Ctrl Pts',(3.35318902552676,-1.,2.26084915222484));
#49970=CARTESIAN_POINT('Ctrl Pts',(3.35750328523077,-1.,2.26719668579921));
#49971=CARTESIAN_POINT('Ctrl Pts',(3.36179055004369,-1.,2.27357362620902));
#49972=CARTESIAN_POINT('Ctrl Pts',(3.36605130712978,-1.,2.27997979457968));
#49973=CARTESIAN_POINT('Ctrl Pts',(3.37028570206357,-1.,2.28641481081045));
#49974=CARTESIAN_POINT('Ctrl Pts',(3.37449367172707,-1.,2.2928781800731));
#49975=CARTESIAN_POINT('Ctrl Pts',(3.37867504959382,-1.,2.29936936127588));
#49976=CARTESIAN_POINT('Ctrl Pts',(3.38282967336676,-1.,2.30588783640389));
#49977=CARTESIAN_POINT('Ctrl Pts',(3.38695751492659,-1.,2.31243319489505));
#49978=CARTESIAN_POINT('Ctrl Pts',(3.39105869475112,-1.,2.31900513925627));
#49979=CARTESIAN_POINT('Ctrl Pts',(3.39513342020045,-1.,2.32560343902683));
#49980=CARTESIAN_POINT('Ctrl Pts',(3.39918194578115,-1.,2.33222789882601));
#49981=CARTESIAN_POINT('Ctrl Pts',(3.40320452776646,-1.,2.33887832342715));
#49982=CARTESIAN_POINT('Ctrl Pts',(3.40720137403888,-1.,2.34555447648901));
#49983=CARTESIAN_POINT('Ctrl Pts',(3.41117262313464,-1.,2.35225606823649));
#49984=CARTESIAN_POINT('Ctrl Pts',(3.4151183675076,-1.,2.35898278606449));
#49985=CARTESIAN_POINT('Ctrl Pts',(3.41903866635384,-1.,2.36573431470314));
#49986=CARTESIAN_POINT('Ctrl Pts',(3.42293356216595,-1.,2.37251035954351));
#49987=CARTESIAN_POINT('Ctrl Pts',(3.42680309755241,-1.,2.37931067029517));
#49988=CARTESIAN_POINT('Ctrl Pts',(3.43064732714472,-1.,2.38613505844641));
#49989=CARTESIAN_POINT('Ctrl Pts',(3.43446630680436,-1.,2.39298338805823));
#49990=CARTESIAN_POINT('Ctrl Pts',(3.43750133066036,-1.,2.39848113411429));
#49991=CARTESIAN_POINT('Ctrl Pts',(3.43976627485223,-1.,2.40261515590099));
#49992=CARTESIAN_POINT('Ctrl Pts',(3.44127120683402,-1.,2.40537592959345));
#49993=CARTESIAN_POINT('Ctrl Pts',(3.44202241512147,-1.,2.40675750623143));
#49994=CARTESIAN_POINT('',(3.35260583073571,-1.,2.52982887637028));
#49995=CARTESIAN_POINT('',(3.44202241512147,-1.,2.40675750623143));
#49996=CARTESIAN_POINT('',(2.90994629141676,-1.,2.36531447826074));
#49997=CARTESIAN_POINT('Ctrl Pts',(3.35260583073571,-1.,2.52982887637028));
#49998=CARTESIAN_POINT('Ctrl Pts',(3.35105973714071,-1.,2.5295413654909));
#49999=CARTESIAN_POINT('Ctrl Pts',(3.34796903576663,-1.,2.52896321610703));
#50000=CARTESIAN_POINT('Ctrl Pts',(3.34333744115511,-1.,2.52808660915689));
#50001=CARTESIAN_POINT('Ctrl Pts',(3.33717089999103,-1.,2.52689902690158));
#50002=CARTESIAN_POINT('Ctrl Pts',(3.32947762187533,-1.,2.52538321164634));
#50003=CARTESIAN_POINT('Ctrl Pts',(3.32179931078699,-1.,2.5238359839626));
#50004=CARTESIAN_POINT('Ctrl Pts',(3.31413607874645,-1.,2.52225724871313));
#50005=CARTESIAN_POINT('Ctrl Pts',(3.30648808815442,-1.,2.52064689568511));
#50006=CARTESIAN_POINT('Ctrl Pts',(3.29885556388352,-1.,2.51900480701069));
#50007=CARTESIAN_POINT('Ctrl Pts',(3.2912387729927,-1.,2.51733085123797));
#50008=CARTESIAN_POINT('Ctrl Pts',(3.28363799702982,-1.,2.51562487464514));
#50009=CARTESIAN_POINT('Ctrl Pts',(3.27605350473142,-1.,2.513886692704));
#50010=CARTESIAN_POINT('Ctrl Pts',(3.26848552888115,-1.,2.51211608411423));
#50011=CARTESIAN_POINT('Ctrl Pts',(3.26093423001434,-1.,2.51031277813486));
#50012=CARTESIAN_POINT('Ctrl Pts',(3.25339971460982,-1.,2.50847647070723));
#50013=CARTESIAN_POINT('Ctrl Pts',(3.24588208983849,-1.,2.506606859405));
#50014=CARTESIAN_POINT('Ctrl Pts',(3.23838151080319,-1.,2.5047036758003));
#50015=CARTESIAN_POINT('Ctrl Pts',(3.23089822320646,-1.,2.50276671338111));
#50016=CARTESIAN_POINT('Ctrl Pts',(3.22343262620503,-1.,2.50079587201958));
#50017=CARTESIAN_POINT('Ctrl Pts',(3.21598526261286,-1.,2.4987911459939));
#50018=CARTESIAN_POINT('Ctrl Pts',(3.20855669849836,-1.,2.4967525264737));
#50019=CARTESIAN_POINT('Ctrl Pts',(3.20114742397588,-1.,2.49467992057755));
#50020=CARTESIAN_POINT('Ctrl Pts',(3.19375775555798,-1.,2.49257307239848));
#50021=CARTESIAN_POINT('Ctrl Pts',(3.18638771282266,-1.,2.49043146334059));
#50022=CARTESIAN_POINT('Ctrl Pts',(3.17903698136622,-1.,2.48825428288201));
#50023=CARTESIAN_POINT('Ctrl Pts',(3.17170518863313,-1.,2.48604065348587));
#50024=CARTESIAN_POINT('Ctrl Pts',(3.16439213290161,-1.,2.48378981792725));
#50025=CARTESIAN_POINT('Ctrl Pts',(3.15709802322739,-1.,2.48150133566571));
#50026=CARTESIAN_POINT('Ctrl Pts',(3.14982373241352,-1.,2.47917529057029));
#50027=CARTESIAN_POINT('Ctrl Pts',(3.1425709954655,-1.,2.47681245356109));
#50028=CARTESIAN_POINT('Ctrl Pts',(3.13534181229295,-1.,2.47441378371932));
#50029=CARTESIAN_POINT('Ctrl Pts',(3.12813790805952,-1.,2.47197997765871));
#50030=CARTESIAN_POINT('Ctrl Pts',(3.12096015766983,-1.,2.46951098947469));
#50031=CARTESIAN_POINT('Ctrl Pts',(3.11380805536122,-1.,2.46700558843506));
#50032=CARTESIAN_POINT('Ctrl Pts',(3.1066790790198,-1.,2.46446082979646));
#50033=CARTESIAN_POINT('Ctrl Pts',(3.09956993697052,-1.,2.46187308501884));
#50034=CARTESIAN_POINT('Ctrl Pts',(3.09247787931887,-1.,2.4592391256388));
#50035=CARTESIAN_POINT('Ctrl Pts',(3.08540206545315,-1.,2.45655725437039));
#50036=CARTESIAN_POINT('Ctrl Pts',(3.07834472886139,-1.,2.4538282678779));
#50037=CARTESIAN_POINT('Ctrl Pts',(3.07131290521297,-1.,2.45105688854422));
#50038=CARTESIAN_POINT('Ctrl Pts',(3.06431596421405,-1.,2.44824970516544));
#50039=CARTESIAN_POINT('Ctrl Pts',(3.05736242671506,-1.,2.44541251892556));
#50040=CARTESIAN_POINT('Ctrl Pts',(3.05045678021504,-1.,2.44254768923105));
#50041=CARTESIAN_POINT('Ctrl Pts',(3.04359685040555,-1.,2.43965194061857));
#50042=CARTESIAN_POINT('Ctrl Pts',(3.03676949672821,-1.,2.43671278042414));
#50043=CARTESIAN_POINT('Ctrl Pts',(3.02995534946978,-1.,2.43371241361488));
#50044=CARTESIAN_POINT('Ctrl Pts',(3.02313656036004,-1.,2.43063415586637));
#50045=CARTESIAN_POINT('Ctrl Pts',(3.01630420830504,-1.,2.42746856264168));
#50046=CARTESIAN_POINT('Ctrl Pts',(3.00946442616658,-1.,2.42421849439613));
#50047=CARTESIAN_POINT('Ctrl Pts',(3.00264868585996,-1.,2.42090763946779));
#50048=CARTESIAN_POINT('Ctrl Pts',(2.99590509293503,-1.,2.41757324500514));
#50049=CARTESIAN_POINT('Ctrl Pts',(2.98927983005796,-1.,2.41425064199586));
#50050=CARTESIAN_POINT('Ctrl Pts',(2.98280015815107,-1.,2.41095909342571));
#50051=CARTESIAN_POINT('Ctrl Pts',(2.97646002822422,-1.,2.40768975073713));
#50052=CARTESIAN_POINT('Ctrl Pts',(2.9701964131236,-1.,2.40438604734919));
#50053=CARTESIAN_POINT('Ctrl Pts',(2.96390432240312,-1.,2.4009556571164));
#50054=CARTESIAN_POINT('Ctrl Pts',(2.95748006482942,-1.,2.39730553974517));
#50055=CARTESIAN_POINT('Ctrl Pts',(2.95085857128439,-1.,2.39337207631667));
#50056=CARTESIAN_POINT('Ctrl Pts',(2.94404820669076,-1.,2.38914929090759));
#50057=CARTESIAN_POINT('Ctrl Pts',(2.93717903280391,-1.,2.38472771516311));
#50058=CARTESIAN_POINT('Ctrl Pts',(2.93049643640206,-1.,2.38028989582073));
#50059=CARTESIAN_POINT('Ctrl Pts',(2.92430340582608,-1.,2.3760651052403));
#50060=CARTESIAN_POINT('Ctrl Pts',(2.91891503791411,-1.,2.37229381109821));
#50061=CARTESIAN_POINT('Ctrl Pts',(2.9146124988314,-1.,2.36919161373173));
#50062=CARTESIAN_POINT('Ctrl Pts',(2.91181344022548,-1.,2.36707658451664));
#50063=CARTESIAN_POINT('Ctrl Pts',(2.91051690822156,-1.,2.36599991765749));
#50064=CARTESIAN_POINT('Ctrl Pts',(2.91005770527719,-1.,2.36553202948613));
#50065=CARTESIAN_POINT('Ctrl Pts',(2.90995756655606,-1.,2.36536211188453));
#50066=CARTESIAN_POINT('Ctrl Pts',(2.90994629141676,-1.,2.36531447826074));
#50067=CARTESIAN_POINT('',(2.79140942341378,-1.,2.50410331873042));
#50068=CARTESIAN_POINT('Origin',(0.,-1.,0.));
#50069=CARTESIAN_POINT('',(3.02314558451372,-1.,2.91557726271063));
#50070=CARTESIAN_POINT('Ctrl Pts',(2.79140942341378,-1.,2.50410331873043));
#50071=CARTESIAN_POINT('Ctrl Pts',(2.79145823440899,-1.,2.50410700351427));
#50072=CARTESIAN_POINT('Ctrl Pts',(2.79164172519039,-1.,2.50417932839343));
#50073=CARTESIAN_POINT('Ctrl Pts',(2.79217568804874,-1.,2.50455968395235));
#50074=CARTESIAN_POINT('Ctrl Pts',(2.79344192164204,-1.,2.50567182569153));
#50075=CARTESIAN_POINT('Ctrl Pts',(2.7959687805717,-1.,2.50810555977564));
#50076=CARTESIAN_POINT('Ctrl Pts',(2.79970585014308,-1.,2.51186983687947));
#50077=CARTESIAN_POINT('Ctrl Pts',(2.80427363984939,-1.,2.51660190466067));
#50078=CARTESIAN_POINT('Ctrl Pts',(2.80941521967234,-1.,2.52205778589922));
#50079=CARTESIAN_POINT('Ctrl Pts',(2.8148437904867,-1.,2.52796388055457));
#50080=CARTESIAN_POINT('Ctrl Pts',(2.82028550483744,-1.,2.53405679667463));
#50081=CARTESIAN_POINT('Ctrl Pts',(2.82552167649157,-1.,2.54012272520141));
#50082=CARTESIAN_POINT('Ctrl Pts',(2.83044254225794,-1.,2.54604736792542));
#50083=CARTESIAN_POINT('Ctrl Pts',(2.83505269592412,-1.,2.55182152806964));
#50084=CARTESIAN_POINT('Ctrl Pts',(2.83942515220699,-1.,2.55749952145165));
#50085=CARTESIAN_POINT('Ctrl Pts',(2.84366802680211,-1.,2.56316920798489));
#50086=CARTESIAN_POINT('Ctrl Pts',(2.84788893329091,-1.,2.56891984251743));
#50087=CARTESIAN_POINT('Ctrl Pts',(2.85215360144482,-1.,2.57480482727128));
#50088=CARTESIAN_POINT('Ctrl Pts',(2.85647171715147,-1.,2.58082875254407));
#50089=CARTESIAN_POINT('Ctrl Pts',(2.86081999003668,-1.,2.5869677064356));
#50090=CARTESIAN_POINT('Ctrl Pts',(2.86515629953528,-1.,2.59318160184921));
#50091=CARTESIAN_POINT('Ctrl Pts',(2.86943633170712,-1.,2.59942875223202));
#50092=CARTESIAN_POINT('Ctrl Pts',(2.87363176656475,-1.,2.6056817788128));
#50093=CARTESIAN_POINT('Ctrl Pts',(2.87773881947885,-1.,2.61193507170928));
#50094=CARTESIAN_POINT('Ctrl Pts',(2.88176821427502,-1.,2.61819596473087));
#50095=CARTESIAN_POINT('Ctrl Pts',(2.88573922195049,-1.,2.62447947640253));
#50096=CARTESIAN_POINT('Ctrl Pts',(2.88967244854243,-1.,2.63080195420771));
#50097=CARTESIAN_POINT('Ctrl Pts',(2.89358228854557,-1.,2.63717442263944));
#50098=CARTESIAN_POINT('Ctrl Pts',(2.89747231723361,-1.,2.64359851684146));
#50099=CARTESIAN_POINT('Ctrl Pts',(2.90133950224879,-1.,2.65007017365576));
#50100=CARTESIAN_POINT('Ctrl Pts',(2.90517678087467,-1.,2.65658188464287));
#50101=CARTESIAN_POINT('Ctrl Pts',(2.90897617968921,-1.,2.66312542616809));
#50102=CARTESIAN_POINT('Ctrl Pts',(2.91273193382876,-1.,2.66969458792627));
#50103=CARTESIAN_POINT('Ctrl Pts',(2.91644290704281,-1.,2.67628728855309));
#50104=CARTESIAN_POINT('Ctrl Pts',(2.92011090722152,-1.,2.68290409279689));
#50105=CARTESIAN_POINT('Ctrl Pts',(2.92373955325876,-1.,2.68954721165342));
#50106=CARTESIAN_POINT('Ctrl Pts',(2.92733294395268,-1.,2.69621932864302));
#50107=CARTESIAN_POINT('Ctrl Pts',(2.93089438233746,-1.,2.70292247416881));
#50108=CARTESIAN_POINT('Ctrl Pts',(2.93442516311167,-1.,2.70965695523776));
#50109=CARTESIAN_POINT('Ctrl Pts',(2.93792519474955,-1.,2.71642190053575));
#50110=CARTESIAN_POINT('Ctrl Pts',(2.94139351933882,-1.,2.72321571511322));
#50111=CARTESIAN_POINT('Ctrl Pts',(2.94482887675139,-1.,2.73003657371613));
#50112=CARTESIAN_POINT('Ctrl Pts',(2.94823023414381,-1.,2.73688288329825));
#50113=CARTESIAN_POINT('Ctrl Pts',(2.95159737214304,-1.,2.7437537949221));
#50114=CARTESIAN_POINT('Ctrl Pts',(2.95493069316211,-1.,2.75064903318996));
#50115=CARTESIAN_POINT('Ctrl Pts',(2.9582309766594,-1.,2.75756867888393));
#50116=CARTESIAN_POINT('Ctrl Pts',(2.96149914764832,-1.,2.76451296269571));
#50117=CARTESIAN_POINT('Ctrl Pts',(2.96473605585548,-1.,2.77148206836464));
#50118=CARTESIAN_POINT('Ctrl Pts',(2.9679422104295,-1.,2.77847589542767));
#50119=CARTESIAN_POINT('Ctrl Pts',(2.97111781461349,-1.,2.78549409123657));
#50120=CARTESIAN_POINT('Ctrl Pts',(2.97426288347475,-1.,2.79253615718147));
#50121=CARTESIAN_POINT('Ctrl Pts',(2.97737733718242,-1.,2.79960153278186));
#50122=CARTESIAN_POINT('Ctrl Pts',(2.98046109647299,-1.,2.80668968101162));
#50123=CARTESIAN_POINT('Ctrl Pts',(2.9835141977994,-1.,2.81380019196454));
#50124=CARTESIAN_POINT('Ctrl Pts',(2.98653680669434,-1.,2.82093279065704));
#50125=CARTESIAN_POINT('Ctrl Pts',(2.98952916401699,-1.,2.82808728190402));
#50126=CARTESIAN_POINT('Ctrl Pts',(2.99249155170479,-1.,2.83526351254383));
#50127=CARTESIAN_POINT('Ctrl Pts',(2.995424253416,-1.,2.84246132984334));
#50128=CARTESIAN_POINT('Ctrl Pts',(2.99832751144566,-1.,2.84968053289104));
#50129=CARTESIAN_POINT('Ctrl Pts',(3.0012015079552,-1.,2.85692085715129));
#50130=CARTESIAN_POINT('Ctrl Pts',(3.00404638316245,-1.,2.86418200833065));
#50131=CARTESIAN_POINT('Ctrl Pts',(3.00686224485374,-1.,2.87146368430104));
#50132=CARTESIAN_POINT('Ctrl Pts',(3.0096491810855,-1.,2.87876560072799));
#50133=CARTESIAN_POINT('Ctrl Pts',(3.01240727309568,-1.,2.88608751706796));
#50134=CARTESIAN_POINT('Ctrl Pts',(3.01513660433291,-1.,2.8934292556764));
#50135=CARTESIAN_POINT('Ctrl Pts',(3.01783725123646,-1.,2.90079069102661));
#50136=CARTESIAN_POINT('Ctrl Pts',(3.01997487194926,-1.,2.90669553303902));
#50137=CARTESIAN_POINT('Ctrl Pts',(3.02156522743299,-1.,2.91113297349052));
#50138=CARTESIAN_POINT('Ctrl Pts',(3.02261975104912,-1.,2.91409518070707));
#50139=CARTESIAN_POINT('Ctrl Pts',(3.02314558451372,-1.,2.91557726271063));
#50140=CARTESIAN_POINT('',(2.91557726271063,-1.,3.02314558451372));
#50141=CARTESIAN_POINT('',(3.02314558451372,-1.,2.91557726271063));
#50142=CARTESIAN_POINT('',(2.50410331873176,-1.,2.79140942341258));
#50143=CARTESIAN_POINT('Ctrl Pts',(2.91557726271063,-1.,3.02314558451372));
#50144=CARTESIAN_POINT('Ctrl Pts',(2.91409518070399,-1.,3.02261975104593));
#50145=CARTESIAN_POINT('Ctrl Pts',(2.91113297348212,-1.,3.02156522742431));
#50146=CARTESIAN_POINT('Ctrl Pts',(2.90669553302526,-1.,3.01997487193503));
#50147=CARTESIAN_POINT('Ctrl Pts',(2.9007906910105,-1.,3.01783725121981));
#50148=CARTESIAN_POINT('Ctrl Pts',(2.89342925566321,-1.,3.01513660431928));
#50149=CARTESIAN_POINT('Ctrl Pts',(2.8860875170608,-1.,3.01240727308829));
#50150=CARTESIAN_POINT('Ctrl Pts',(2.87876560072727,-1.,3.00964918108476));
#50151=CARTESIAN_POINT('Ctrl Pts',(2.87146368430501,-1.,3.00686224485784));
#50152=CARTESIAN_POINT('Ctrl Pts',(2.86418200833667,-1.,3.00404638316867));
#50153=CARTESIAN_POINT('Ctrl Pts',(2.85692085715685,-1.,3.00120150796095));
#50154=CARTESIAN_POINT('Ctrl Pts',(2.84968053289451,-1.,2.99832751144925));
#50155=CARTESIAN_POINT('Ctrl Pts',(2.84246132984415,-1.,2.99542425341685));
#50156=CARTESIAN_POINT('Ctrl Pts',(2.83526351254248,-1.,2.9924915517034));
#50157=CARTESIAN_POINT('Ctrl Pts',(2.82808728190157,-1.,2.98952916401446));
#50158=CARTESIAN_POINT('Ctrl Pts',(2.82093279065457,-1.,2.9865368066918));
#50159=CARTESIAN_POINT('Ctrl Pts',(2.81380019196286,-1.,2.98351419779767));
#50160=CARTESIAN_POINT('Ctrl Pts',(2.80668968101106,-1.,2.98046109647241));
#50161=CARTESIAN_POINT('Ctrl Pts',(2.7996015327823,-1.,2.97737733718287));
#50162=CARTESIAN_POINT('Ctrl Pts',(2.79253615718248,-1.,2.9742628834758));
#50163=CARTESIAN_POINT('Ctrl Pts',(2.78549409123769,-1.,2.97111781461465));
#50164=CARTESIAN_POINT('Ctrl Pts',(2.7784758954285,-1.,2.96794221043036));
#50165=CARTESIAN_POINT('Ctrl Pts',(2.77148206836498,-1.,2.96473605585583));
#50166=CARTESIAN_POINT('Ctrl Pts',(2.76451296269557,-1.,2.96149914764818));
#50167=CARTESIAN_POINT('Ctrl Pts',(2.7575686788835,-1.,2.95823097665896));
#50168=CARTESIAN_POINT('Ctrl Pts',(2.75064903318947,-1.,2.95493069316161));
#50169=CARTESIAN_POINT('Ctrl Pts',(2.74375379492172,-1.,2.95159737214266));
#50170=CARTESIAN_POINT('Ctrl Pts',(2.73688288329808,-1.,2.94823023414364));
#50171=CARTESIAN_POINT('Ctrl Pts',(2.73003657371616,-1.,2.94482887675143));
#50172=CARTESIAN_POINT('Ctrl Pts',(2.72321571511337,-1.,2.94139351933897));
#50173=CARTESIAN_POINT('Ctrl Pts',(2.71642190053592,-1.,2.93792519474972));
#50174=CARTESIAN_POINT('Ctrl Pts',(2.70965695523787,-1.,2.93442516311179));
#50175=CARTESIAN_POINT('Ctrl Pts',(2.70292247416885,-1.,2.9308943823375));
#50176=CARTESIAN_POINT('Ctrl Pts',(2.69621932864301,-1.,2.92733294395267));
#50177=CARTESIAN_POINT('Ctrl Pts',(2.68954721165339,-1.,2.92373955325875));
#50178=CARTESIAN_POINT('Ctrl Pts',(2.68290409279688,-1.,2.92011090722152));
#50179=CARTESIAN_POINT('Ctrl Pts',(2.67628728855312,-1.,2.91644290704285));
#50180=CARTESIAN_POINT('Ctrl Pts',(2.66969458792631,-1.,2.91273193382882));
#50181=CARTESIAN_POINT('Ctrl Pts',(2.6631254261681,-1.,2.90897617968923));
#50182=CARTESIAN_POINT('Ctrl Pts',(2.65658188464282,-1.,2.90517678087461));
#50183=CARTESIAN_POINT('Ctrl Pts',(2.65007017365564,-1.,2.90133950224867));
#50184=CARTESIAN_POINT('Ctrl Pts',(2.64359851684131,-1.,2.89747231723345));
#50185=CARTESIAN_POINT('Ctrl Pts',(2.63717442263932,-1.,2.89358228854544));
#50186=CARTESIAN_POINT('Ctrl Pts',(2.63080195420767,-1.,2.88967244854239));
#50187=CARTESIAN_POINT('Ctrl Pts',(2.62447947640262,-1.,2.88573922195059));
#50188=CARTESIAN_POINT('Ctrl Pts',(2.61819596473108,-1.,2.88176821427525));
#50189=CARTESIAN_POINT('Ctrl Pts',(2.61193507170955,-1.,2.87773881947916));
#50190=CARTESIAN_POINT('Ctrl Pts',(2.60568177881303,-1.,2.87363176656501));
#50191=CARTESIAN_POINT('Ctrl Pts',(2.5994287522321,-1.,2.86943633170722));
#50192=CARTESIAN_POINT('Ctrl Pts',(2.59318160184908,-1.,2.86515629953513));
#50193=CARTESIAN_POINT('Ctrl Pts',(2.58696770643524,-1.,2.86081999003629));
#50194=CARTESIAN_POINT('Ctrl Pts',(2.58082875254357,-1.,2.85647171715092));
#50195=CARTESIAN_POINT('Ctrl Pts',(2.57480482727081,-1.,2.85215360144431));
#50196=CARTESIAN_POINT('Ctrl Pts',(2.56891984251721,-1.,2.84788893329067));
#50197=CARTESIAN_POINT('Ctrl Pts',(2.56316920798513,-1.,2.84366802680237));
#50198=CARTESIAN_POINT('Ctrl Pts',(2.55749952145241,-1.,2.83942515220782));
#50199=CARTESIAN_POINT('Ctrl Pts',(2.55182152807077,-1.,2.83505269592536));
#50200=CARTESIAN_POINT('Ctrl Pts',(2.54604736792655,-1.,2.83044254225917));
#50201=CARTESIAN_POINT('Ctrl Pts',(2.54012272520199,-1.,2.8255216764922));
#50202=CARTESIAN_POINT('Ctrl Pts',(2.53405679667412,-1.,2.82028550483689));
#50203=CARTESIAN_POINT('Ctrl Pts',(2.52796388055278,-1.,2.81484379048475));
#50204=CARTESIAN_POINT('Ctrl Pts',(2.52205778589653,-1.,2.80941521966941));
#50205=CARTESIAN_POINT('Ctrl Pts',(2.51660190465805,-1.,2.80427363984653));
#50206=CARTESIAN_POINT('Ctrl Pts',(2.51186983687818,-1.,2.79970585014168));
#50207=CARTESIAN_POINT('Ctrl Pts',(2.5081055597767,-1.,2.79596878057287));
#50208=CARTESIAN_POINT('Ctrl Pts',(2.50567182569081,-1.,2.79344192164147));
#50209=CARTESIAN_POINT('Ctrl Pts',(2.50455968395146,-1.,2.79217568804755));
#50210=CARTESIAN_POINT('Ctrl Pts',(2.50417932839313,-1.,2.79164172518905));
#50211=CARTESIAN_POINT('Ctrl Pts',(2.50410700351493,-1.,2.79145823440781));
#50212=CARTESIAN_POINT('Ctrl Pts',(2.50410331873176,-1.,2.79140942341258));
#50213=CARTESIAN_POINT('',(2.36531447826213,-1.,2.90994629141563));
#50214=CARTESIAN_POINT('Origin',(0.,-1.,0.));
#50215=CARTESIAN_POINT('',(2.52982887637028,-1.,3.35260583073571));
#50216=CARTESIAN_POINT('Ctrl Pts',(2.36531447826213,-1.,2.90994629141563));
#50217=CARTESIAN_POINT('Ctrl Pts',(2.3653621118858,-1.,2.90995756655559));
#50218=CARTESIAN_POINT('Ctrl Pts',(2.36553202948741,-1.,2.9100577052777));
#50219=CARTESIAN_POINT('Ctrl Pts',(2.36599991765853,-1.,2.91051690822262));
#50220=CARTESIAN_POINT('Ctrl Pts',(2.36707658451709,-1.,2.91181344022628));
#50221=CARTESIAN_POINT('Ctrl Pts',(2.36919161373074,-1.,2.91461249883016));
#50222=CARTESIAN_POINT('Ctrl Pts',(2.37229381109939,-1.,2.9189150379156));
#50223=CARTESIAN_POINT('Ctrl Pts',(2.37606510524271,-1.,2.92430340582912));
#50224=CARTESIAN_POINT('Ctrl Pts',(2.3802898958232,-1.,2.93049643640517));
#50225=CARTESIAN_POINT('Ctrl Pts',(2.38472771516476,-1.,2.93717903280599));
#50226=CARTESIAN_POINT('Ctrl Pts',(2.38914929090806,-1.,2.94404820669135));
#50227=CARTESIAN_POINT('Ctrl Pts',(2.39337207631613,-1.,2.95085857128372));
#50228=CARTESIAN_POINT('Ctrl Pts',(2.39730553974412,-1.,2.95748006482811));
#50229=CARTESIAN_POINT('Ctrl Pts',(2.40095565711535,-1.,2.96390432240181));
#50230=CARTESIAN_POINT('Ctrl Pts',(2.40438604734848,-1.,2.97019641312272));
#50231=CARTESIAN_POINT('Ctrl Pts',(2.40768975073691,-1.,2.97646002822395));
#50232=CARTESIAN_POINT('Ctrl Pts',(2.41095909342591,-1.,2.98280015815132));
#50233=CARTESIAN_POINT('Ctrl Pts',(2.4142506419963,-1.,2.98927983005851));
#50234=CARTESIAN_POINT('Ctrl Pts',(2.4175732450056,-1.,2.99590509293561));
#50235=CARTESIAN_POINT('Ctrl Pts',(2.42090763946812,-1.,3.00264868586038));
#50236=CARTESIAN_POINT('Ctrl Pts',(2.42421849439625,-1.,3.00946442616674));
#50237=CARTESIAN_POINT('Ctrl Pts',(2.4274685626416,-1.,3.01630420830494));
#50238=CARTESIAN_POINT('Ctrl Pts',(2.43063415586615,-1.,3.02313656035977));
#50239=CARTESIAN_POINT('Ctrl Pts',(2.43371241361462,-1.,3.02995534946946));
#50240=CARTESIAN_POINT('Ctrl Pts',(2.43671278042394,-1.,3.03676949672797));
#50241=CARTESIAN_POINT('Ctrl Pts',(2.43965194061849,-1.,3.04359685040545));
#50242=CARTESIAN_POINT('Ctrl Pts',(2.44254768923109,-1.,3.05045678021509));
#50243=CARTESIAN_POINT('Ctrl Pts',(2.44541251892568,-1.,3.05736242671521));
#50244=CARTESIAN_POINT('Ctrl Pts',(2.44824970516557,-1.,3.06431596421422));
#50245=CARTESIAN_POINT('Ctrl Pts',(2.45105688854432,-1.,3.0713129052131));
#50246=CARTESIAN_POINT('Ctrl Pts',(2.45382826787795,-1.,3.07834472886145));
#50247=CARTESIAN_POINT('Ctrl Pts',(2.45655725437037,-1.,3.08540206545313));
#50248=CARTESIAN_POINT('Ctrl Pts',(2.45923912563875,-1.,3.09247787931881));
#50249=CARTESIAN_POINT('Ctrl Pts',(2.4618730850188,-1.,3.09956993697048));
#50250=CARTESIAN_POINT('Ctrl Pts',(2.46446082979645,-1.,3.10667907901981));
#50251=CARTESIAN_POINT('Ctrl Pts',(2.46700558843507,-1.,3.11380805536124));
#50252=CARTESIAN_POINT('Ctrl Pts',(2.4695109894747,-1.,3.12096015766984));
#50253=CARTESIAN_POINT('Ctrl Pts',(2.47197997765868,-1.,3.12813790805948));
#50254=CARTESIAN_POINT('Ctrl Pts',(2.47441378371923,-1.,3.13534181229282));
#50255=CARTESIAN_POINT('Ctrl Pts',(2.47681245356095,-1.,3.14257099546531));
#50256=CARTESIAN_POINT('Ctrl Pts',(2.47917529057016,-1.,3.14982373241335));
#50257=CARTESIAN_POINT('Ctrl Pts',(2.48150133566568,-1.,3.15709802322735));
#50258=CARTESIAN_POINT('Ctrl Pts',(2.48378981792739,-1.,3.16439213290181));
#50259=CARTESIAN_POINT('Ctrl Pts',(2.48604065348619,-1.,3.17170518863357));
#50260=CARTESIAN_POINT('Ctrl Pts',(2.48825428288242,-1.,3.17903698136679));
#50261=CARTESIAN_POINT('Ctrl Pts',(2.49043146334095,-1.,3.18638771282315));
#50262=CARTESIAN_POINT('Ctrl Pts',(2.4925730723986,-1.,3.19375775555814));
#50263=CARTESIAN_POINT('Ctrl Pts',(2.49467992057726,-1.,3.20114742397549));
#50264=CARTESIAN_POINT('Ctrl Pts',(2.49675252647298,-1.,3.2085566984974));
#50265=CARTESIAN_POINT('Ctrl Pts',(2.49879114599293,-1.,3.21598526261157));
#50266=CARTESIAN_POINT('Ctrl Pts',(2.5007958720187,-1.,3.22343262620387));
#50267=CARTESIAN_POINT('Ctrl Pts',(2.50276671338074,-1.,3.23089822320596));
#50268=CARTESIAN_POINT('Ctrl Pts',(2.50470367580078,-1.,3.23838151080383));
#50269=CARTESIAN_POINT('Ctrl Pts',(2.50660685940645,-1.,3.24588208984042));
#50270=CARTESIAN_POINT('Ctrl Pts',(2.50847647070936,-1.,3.25339971461265));
#50271=CARTESIAN_POINT('Ctrl Pts',(2.51031277813697,-1.,3.26093423001716));
#50272=CARTESIAN_POINT('Ctrl Pts',(2.51211608411539,-1.,3.26848552888271));
#50273=CARTESIAN_POINT('Ctrl Pts',(2.51388669270329,-1.,3.27605350473048));
#50274=CARTESIAN_POINT('Ctrl Pts',(2.51562487464214,-1.,3.28363799702583));
#50275=CARTESIAN_POINT('Ctrl Pts',(2.51733085123316,-1.,3.2912387729863));
#50276=CARTESIAN_POINT('Ctrl Pts',(2.51900480700548,-1.,3.29885556387661));
#50277=CARTESIAN_POINT('Ctrl Pts',(2.52064689568167,-1.,3.30648808814986));
#50278=CARTESIAN_POINT('Ctrl Pts',(2.52225724871375,-1.,3.31413607874727));
#50279=CARTESIAN_POINT('Ctrl Pts',(2.52383598396878,-1.,3.32179931079521));
#50280=CARTESIAN_POINT('Ctrl Pts',(2.52538321165774,-1.,3.32947762189049));
#50281=CARTESIAN_POINT('Ctrl Pts',(2.52689902691551,-1.,3.33717090000955));
#50282=CARTESIAN_POINT('Ctrl Pts',(2.52808660916879,-1.,3.34333744117093));
#50283=CARTESIAN_POINT('Ctrl Pts',(2.5289632161143,-1.,3.34796903577628));
#50284=CARTESIAN_POINT('Ctrl Pts',(2.52954136549357,-1.,3.35105973714426));
#50285=CARTESIAN_POINT('Ctrl Pts',(2.52982887637028,-1.,3.35260583073571));
#50286=CARTESIAN_POINT('',(2.40675750623143,-1.,3.44202241512147));
#50287=CARTESIAN_POINT('',(2.52982887637028,-1.,3.35260583073571));
#50288=CARTESIAN_POINT('',(2.03660101169714,-1.,3.14877060440328));
#50289=CARTESIAN_POINT('Ctrl Pts',(2.40675750623143,-1.,3.44202241512147));
#50290=CARTESIAN_POINT('Ctrl Pts',(2.4053759295909,-1.,3.44127120683039));
#50291=CARTESIAN_POINT('Ctrl Pts',(2.40261515589405,-1.,3.43976627484234));
#50292=CARTESIAN_POINT('Ctrl Pts',(2.39848113410292,-1.,3.43750133064416));
#50293=CARTESIAN_POINT('Ctrl Pts',(2.39298338804493,-1.,3.4344663067854));
#50294=CARTESIAN_POINT('Ctrl Pts',(2.38613505843552,-1.,3.4306473271292));
#50295=CARTESIAN_POINT('Ctrl Pts',(2.37931067028926,-1.,3.42680309754399));
#50296=CARTESIAN_POINT('Ctrl Pts',(2.37251035954292,-1.,3.42293356216511));
#50297=CARTESIAN_POINT('Ctrl Pts',(2.36573431470642,-1.,3.41903866635852));
#50298=CARTESIAN_POINT('Ctrl Pts',(2.35898278606946,-1.,3.41511836751469));
#50299=CARTESIAN_POINT('Ctrl Pts',(2.35225606824109,-1.,3.41117262314119));
#50300=CARTESIAN_POINT('Ctrl Pts',(2.34555447649188,-1.,3.40720137404297));
#50301=CARTESIAN_POINT('Ctrl Pts',(2.33887832342782,-1.,3.40320452776743));
#50302=CARTESIAN_POINT('Ctrl Pts',(2.33222789882489,-1.,3.39918194577956));
#50303=CARTESIAN_POINT('Ctrl Pts',(2.3256034390248,-1.,3.39513342019756));
#50304=CARTESIAN_POINT('Ctrl Pts',(2.31900513925424,-1.,3.39105869474822));
#50305=CARTESIAN_POINT('Ctrl Pts',(2.31243319489367,-1.,3.38695751492462));
#50306=CARTESIAN_POINT('Ctrl Pts',(2.30588783640343,-1.,3.3828296733661));
#50307=CARTESIAN_POINT('Ctrl Pts',(2.29936936127624,-1.,3.37867504959433));
#50308=CARTESIAN_POINT('Ctrl Pts',(2.29287818007393,-1.,3.37449367172826));
#50309=CARTESIAN_POINT('Ctrl Pts',(2.28641481081137,-1.,3.37028570206488));
#50310=CARTESIAN_POINT('Ctrl Pts',(2.27997979458037,-1.,3.36605130713076));
#50311=CARTESIAN_POINT('Ctrl Pts',(2.2735736262093,-1.,3.36179055004409));
#50312=CARTESIAN_POINT('Ctrl Pts',(2.26719668579909,-1.,3.35750328523061));
#50313=CARTESIAN_POINT('Ctrl Pts',(2.26084915222449,-1.,3.35318902552626));
#50314=CARTESIAN_POINT('Ctrl Pts',(2.25453097693483,-1.,3.34884690292285));
#50315=CARTESIAN_POINT('Ctrl Pts',(2.24824207678256,-1.,3.34447596770723));
#50316=CARTESIAN_POINT('Ctrl Pts',(2.24198249391422,-1.,3.34007543738025));
#50317=CARTESIAN_POINT('Ctrl Pts',(2.23575256328812,-1.,3.33564495756482));
#50318=CARTESIAN_POINT('Ctrl Pts',(2.22955308907233,-1.,3.33118487773611));
#50319=CARTESIAN_POINT('Ctrl Pts',(2.22338548312772,-1.,3.3266964672289));
#50320=CARTESIAN_POINT('Ctrl Pts',(2.21725135110898,-1.,3.32218125618968));
#50321=CARTESIAN_POINT('Ctrl Pts',(2.21115211847875,-1.,3.31764044024235));
#50322=CARTESIAN_POINT('Ctrl Pts',(2.20508863150607,-1.,3.31307424608949));
#50323=CARTESIAN_POINT('Ctrl Pts',(2.19906078949922,-1.,3.30848134694595));
#50324=CARTESIAN_POINT('Ctrl Pts',(2.19306710376111,-1.,3.30385816281831));
#50325=CARTESIAN_POINT('Ctrl Pts',(2.18710556500327,-1.,3.29920022557639));
#50326=CARTESIAN_POINT('Ctrl Pts',(2.18117455557065,-1.,3.2945036150049));
#50327=CARTESIAN_POINT('Ctrl Pts',(2.17527380048423,-1.,3.28976645712568));
#50328=CARTESIAN_POINT('Ctrl Pts',(2.16940517773455,-1.,3.28499019979724));
#50329=CARTESIAN_POINT('Ctrl Pts',(2.16357391934425,-1.,3.280181508414));
#50330=CARTESIAN_POINT('Ctrl Pts',(2.15778690038347,-1.,3.27534954469187));
#50331=CARTESIAN_POINT('Ctrl Pts',(2.15205043199808,-1.,3.27050245897228));
#50332=CARTESIAN_POINT('Ctrl Pts',(2.1463680529566,-1.,3.26564388189759));
#50333=CARTESIAN_POINT('Ctrl Pts',(2.14073870754264,-1.,3.26077002641879));
#50334=CARTESIAN_POINT('Ctrl Pts',(2.13515375878803,-1.,3.25586495065054));
#50335=CARTESIAN_POINT('Ctrl Pts',(2.12960028396832,-1.,3.25090574494028));
#50336=CARTESIAN_POINT('Ctrl Pts',(2.12406646410962,-1.,3.24587102613376));
#50337=CARTESIAN_POINT('Ctrl Pts',(2.11854673326979,-1.,3.24074905517293));
#50338=CARTESIAN_POINT('Ctrl Pts',(2.11304604021773,-1.,3.23554444767099));
#50339=CARTESIAN_POINT('Ctrl Pts',(2.10758699642451,-1.,3.23028945793289));
#50340=CARTESIAN_POINT('Ctrl Pts',(2.10220384298492,-1.,3.22503437553434));
#50341=CARTESIAN_POINT('Ctrl Pts',(2.09692958434895,-1.,3.21982707347009));
#50342=CARTESIAN_POINT('Ctrl Pts',(2.09178419460443,-1.,3.21469429601654));
#50343=CARTESIAN_POINT('Ctrl Pts',(2.08676465517455,-1.,3.20962575845463));
#50344=CARTESIAN_POINT('Ctrl Pts',(2.08182850370878,-1.,3.2045481863073));
#50345=CARTESIAN_POINT('Ctrl Pts',(2.07690441870722,-1.,3.19934132836019));
#50346=CARTESIAN_POINT('Ctrl Pts',(2.07192253497857,-1.,3.19388465568252));
#50347=CARTESIAN_POINT('Ctrl Pts',(2.06684062744112,-1.,3.18809755562368));
#50348=CARTESIAN_POINT('Ctrl Pts',(2.06166849827101,-1.,3.18197692964614));
#50349=CARTESIAN_POINT('Ctrl Pts',(2.05650186773132,-1.,3.17564906975371));
#50350=CARTESIAN_POINT('Ctrl Pts',(2.05151770247233,-1.,3.16936341689527));
#50351=CARTESIAN_POINT('Ctrl Pts',(2.04693331247446,-1.,3.16343165058912));
#50352=CARTESIAN_POINT('Ctrl Pts',(2.04297406404027,-1.,3.15817983946367));
#50353=CARTESIAN_POINT('Ctrl Pts',(2.03984073791519,-1.,3.15389991674792));
#50354=CARTESIAN_POINT('Ctrl Pts',(2.03783225495961,-1.,3.15102344775328));
#50355=CARTESIAN_POINT('Ctrl Pts',(2.03693188810544,-1.,3.14959882629805));
#50356=CARTESIAN_POINT('Ctrl Pts',(2.03663974554932,-1.,3.1490119366901));
#50357=CARTESIAN_POINT('Ctrl Pts',(2.03659701539259,-1.,3.14881939088124));
#50358=CARTESIAN_POINT('Ctrl Pts',(2.03660101169714,-1.,3.14877060440328));
#50359=CARTESIAN_POINT('',(1.88097764062697,-1.,3.24413672884812));
#50360=CARTESIAN_POINT('Origin',(0.,-1.,0.));
#50361=CARTESIAN_POINT('',(1.97421938526992,-1.,3.70708211654725));
#50362=CARTESIAN_POINT('Ctrl Pts',(1.88097764062697,-1.,3.24413672884812));
#50363=CARTESIAN_POINT('Ctrl Pts',(1.8810229239812,-1.,3.24415531671284));
#50364=CARTESIAN_POINT('Ctrl Pts',(1.88117508446775,-1.,3.24428080353022));
#50365=CARTESIAN_POINT('Ctrl Pts',(1.88156537699203,-1.,3.24480754676064));
#50366=CARTESIAN_POINT('Ctrl Pts',(1.88242596600454,-1.,3.2462565441079));
#50367=CARTESIAN_POINT('Ctrl Pts',(1.88407708646357,-1.,3.24935200511918));
#50368=CARTESIAN_POINT('Ctrl Pts',(1.88646802523466,-1.,3.25408686339463));
#50369=CARTESIAN_POINT('Ctrl Pts',(1.88934996203698,-1.,3.25999885193947));
#50370=CARTESIAN_POINT('Ctrl Pts',(1.89255393500965,-1.,3.26677653888676));
#50371=CARTESIAN_POINT('Ctrl Pts',(1.89589172903793,-1.,3.27407108933139));
#50372=CARTESIAN_POINT('Ctrl Pts',(1.89918429230462,-1.,3.28154737912352));
#50373=CARTESIAN_POINT('Ctrl Pts',(1.90228971247527,-1.,3.2889344860029));
#50374=CARTESIAN_POINT('Ctrl Pts',(1.90513891864087,-1.,3.29608978722113));
#50375=CARTESIAN_POINT('Ctrl Pts',(1.90773912171341,-1.,3.30300595568195));
#50376=CARTESIAN_POINT('Ctrl Pts',(1.91014297830446,-1.,3.30975721158596));
#50377=CARTESIAN_POINT('Ctrl Pts',(1.91242616234442,-1.,3.31646052426364));
#50378=CARTESIAN_POINT('Ctrl Pts',(1.91466343916627,-1.,3.32323403454535));
#50379=CARTESIAN_POINT('Ctrl Pts',(1.91690081930331,-1.,3.33014884257873));
#50380=CARTESIAN_POINT('Ctrl Pts',(1.9191460961021,-1.,3.33721230710012));
#50381=CARTESIAN_POINT('Ctrl Pts',(1.92138450828404,-1.,3.34439448941961));
#50382=CARTESIAN_POINT('Ctrl Pts',(1.92358838440528,-1.,3.35164424847223));
#50383=CARTESIAN_POINT('Ctrl Pts',(1.92572846125756,-1.,3.35890824422965));
#50384=CARTESIAN_POINT('Ctrl Pts',(1.92778626543786,-1.,3.36615168657567));
#50385=CARTESIAN_POINT('Ctrl Pts',(1.92975993109877,-1.,3.37336807068043));
#50386=CARTESIAN_POINT('Ctrl Pts',(1.93165739093276,-1.,3.3805676852555));
#50387=CARTESIAN_POINT('Ctrl Pts',(1.93349233176788,-1.,3.38777076883256));
#50388=CARTESIAN_POINT('Ctrl Pts',(1.93527929945985,-1.,3.39499923640795));
#50389=CARTESIAN_POINT('Ctrl Pts',(1.93702857723098,-1.,3.40226802104109));
#50390=CARTESIAN_POINT('Ctrl Pts',(1.93874306008143,-1.,3.40957978266642));
#50391=CARTESIAN_POINT('Ctrl Pts',(1.94042111965246,-1.,3.41692971994096));
#50392=CARTESIAN_POINT('Ctrl Pts',(1.94205835913696,-1.,3.42430850941503));
#50393=CARTESIAN_POINT('Ctrl Pts',(1.94364973660284,-1.,3.43170586602434));
#50394=CARTESIAN_POINT('Ctrl Pts',(1.94519168842879,-1.,3.43911410197687));
#50395=CARTESIAN_POINT('Ctrl Pts',(1.94668377715329,-1.,3.44653088665681));
#50396=CARTESIAN_POINT('Ctrl Pts',(1.94812754766524,-1.,3.45395731584051));
#50397=CARTESIAN_POINT('Ctrl Pts',(1.94952575850197,-1.,3.46139661060962));
#50398=CARTESIAN_POINT('Ctrl Pts',(1.95088147859876,-1.,3.46885258974191));
#50399=CARTESIAN_POINT('Ctrl Pts',(1.95219722189876,-1.,3.47632820495921));
#50400=CARTESIAN_POINT('Ctrl Pts',(1.95347412486308,-1.,3.48382414832634));
#50401=CARTESIAN_POINT('Ctrl Pts',(1.95471236969643,-1.,3.49133956289133));
#50402=CARTESIAN_POINT('Ctrl Pts',(1.95591153823661,-1.,3.49887263575583));
#50403=CARTESIAN_POINT('Ctrl Pts',(1.95707099606511,-1.,3.50642124159909));
#50404=CARTESIAN_POINT('Ctrl Pts',(1.95819025316779,-1.,3.51398354617794));
#50405=CARTESIAN_POINT('Ctrl Pts',(1.95926936324461,-1.,3.52155867431486));
#50406=CARTESIAN_POINT('Ctrl Pts',(1.96030879411566,-1.,3.52914648844351));
#50407=CARTESIAN_POINT('Ctrl Pts',(1.96130926212689,-1.,3.53674730625813));
#50408=CARTESIAN_POINT('Ctrl Pts',(1.96227157573067,-1.,3.54436163300443));
#50409=CARTESIAN_POINT('Ctrl Pts',(1.96319648628644,-1.,3.55198990600886));
#50410=CARTESIAN_POINT('Ctrl Pts',(1.96408450906812,-1.,3.55963218706096));
#50411=CARTESIAN_POINT('Ctrl Pts',(1.96493594634567,-1.,3.56728820357791));
#50412=CARTESIAN_POINT('Ctrl Pts',(1.96575096652789,-1.,3.57495748600959));
#50413=CARTESIAN_POINT('Ctrl Pts',(1.96652966688911,-1.,3.58263947663829));
#50414=CARTESIAN_POINT('Ctrl Pts',(1.96727213799544,-1.,3.59033364022801));
#50415=CARTESIAN_POINT('Ctrl Pts',(1.96797854118369,-1.,3.59803959819938));
#50416=CARTESIAN_POINT('Ctrl Pts',(1.9686491188594,-1.,3.60575714017989));
#50417=CARTESIAN_POINT('Ctrl Pts',(1.96928416040877,-1.,3.61348615496704));
#50418=CARTESIAN_POINT('Ctrl Pts',(1.96988398129978,-1.,3.62122658401893));
#50419=CARTESIAN_POINT('Ctrl Pts',(1.97044889850463,-1.,3.62897836973293));
#50420=CARTESIAN_POINT('Ctrl Pts',(1.97097920454464,-1.,3.63674139590412));
#50421=CARTESIAN_POINT('Ctrl Pts',(1.97147515441164,-1.,3.64451546723514));
#50422=CARTESIAN_POINT('Ctrl Pts',(1.97193697240239,-1.,3.652300347166));
#50423=CARTESIAN_POINT('Ctrl Pts',(1.9723648543905,-1.,3.6600957816636));
#50424=CARTESIAN_POINT('Ctrl Pts',(1.97275897198678,-1.,3.66790152752075));
#50425=CARTESIAN_POINT('Ctrl Pts',(1.97311947678516,-1.,3.67571738107084));
#50426=CARTESIAN_POINT('Ctrl Pts',(1.97344650304519,-1.,3.68354319915092));
#50427=CARTESIAN_POINT('Ctrl Pts',(1.97374016225483,-1.,3.69137888599902));
#50428=CARTESIAN_POINT('Ctrl Pts',(1.97394846383216,-1.,3.6976552856004));
#50429=CARTESIAN_POINT('Ctrl Pts',(1.97408973726715,-1.,3.70236698912904));
#50430=CARTESIAN_POINT('Ctrl Pts',(1.97417727645308,-1.,3.70551008132332));
#50431=CARTESIAN_POINT('Ctrl Pts',(1.97421938526992,-1.,3.70708211654725));
#50432=CARTESIAN_POINT('',(1.8386753923786,-1.,3.77614523045147));
#50433=CARTESIAN_POINT('',(1.97421938526992,-1.,3.70708211654725));
#50434=CARTESIAN_POINT('',(1.5189508286633,-1.,3.42859860294306));
#50435=CARTESIAN_POINT('Ctrl Pts',(1.8386753923786,-1.,3.77614523045147));
#50436=CARTESIAN_POINT('Ctrl Pts',(1.83742834010626,-1.,3.77518714457833));
#50437=CARTESIAN_POINT('Ctrl Pts',(1.83493697934534,-1.,3.77326886064398));
#50438=CARTESIAN_POINT('Ctrl Pts',(1.83120816955645,-1.,3.77038509817999));
#50439=CARTESIAN_POINT('Ctrl Pts',(1.82625289220915,-1.,3.76652740353775));
#50440=CARTESIAN_POINT('Ctrl Pts',(1.82008629694091,-1.,3.76168412707948));
#50441=CARTESIAN_POINT('Ctrl Pts',(1.8139472983358,-1.,3.75681965683071));
#50442=CARTESIAN_POINT('Ctrl Pts',(1.80783603939617,-1.,3.75193395887977));
#50443=CARTESIAN_POINT('Ctrl Pts',(1.8017527148577,-1.,3.74702700875467));
#50444=CARTESIAN_POINT('Ctrl Pts',(1.79569757859422,-1.,3.74209880352445));
#50445=CARTESIAN_POINT('Ctrl Pts',(1.78967092823491,-1.,3.73714934730681));
#50446=CARTESIAN_POINT('Ctrl Pts',(1.78367308442901,-1.,3.7321786309547));
#50447=CARTESIAN_POINT('Ctrl Pts',(1.77770437039658,-1.,3.72718661205609));
#50448=CARTESIAN_POINT('Ctrl Pts',(1.77176509401761,-1.,3.72217319911254));
#50449=CARTESIAN_POINT('Ctrl Pts',(1.76585552124394,-1.,3.71713822377359));
#50450=CARTESIAN_POINT('Ctrl Pts',(1.75997588498865,-1.,3.71208146346136));
#50451=CARTESIAN_POINT('Ctrl Pts',(1.75412641804042,-1.,3.70700269736659));
#50452=CARTESIAN_POINT('Ctrl Pts',(1.74830738046057,-1.,3.7019017567335));
#50453=CARTESIAN_POINT('Ctrl Pts',(1.74251908492617,-1.,3.69677856910517));
#50454=CARTESIAN_POINT('Ctrl Pts',(1.73676193254557,-1.,3.69163322648036));
#50455=CARTESIAN_POINT('Ctrl Pts',(1.73103640956717,-1.,3.68646597019332));
#50456=CARTESIAN_POINT('Ctrl Pts',(1.72534302437056,-1.,3.68127704936579));
#50457=CARTESIAN_POINT('Ctrl Pts',(1.71968225581808,-1.,3.67606660374709));
#50458=CARTESIAN_POINT('Ctrl Pts',(1.71405450210383,-1.,3.67083454901611));
#50459=CARTESIAN_POINT('Ctrl Pts',(1.70846001610956,-1.,3.66558043198876));
#50460=CARTESIAN_POINT('Ctrl Pts',(1.70289888566873,-1.,3.66030338774847));
#50461=CARTESIAN_POINT('Ctrl Pts',(1.69737117722534,-1.,3.65500246526749));
#50462=CARTESIAN_POINT('Ctrl Pts',(1.69187705481689,-1.,3.64967689827371));
#50463=CARTESIAN_POINT('Ctrl Pts',(1.68641690471457,-1.,3.64432638915203));
#50464=CARTESIAN_POINT('Ctrl Pts',(1.68099146651586,-1.,3.63895140887462));
#50465=CARTESIAN_POINT('Ctrl Pts',(1.67560193613156,-1.,3.63355343201232));
#50466=CARTESIAN_POINT('Ctrl Pts',(1.67024966008044,-1.,3.62813422105271));
#50467=CARTESIAN_POINT('Ctrl Pts',(1.66493585923855,-1.,3.62269517989109));
#50468=CARTESIAN_POINT('Ctrl Pts',(1.65966133399186,-1.,3.61723666482456));
#50469=CARTESIAN_POINT('Ctrl Pts',(1.65442619244325,-1.,3.61175734965127));
#50470=CARTESIAN_POINT('Ctrl Pts',(1.64922952425832,-1.,3.60625346556992));
#50471=CARTESIAN_POINT('Ctrl Pts',(1.64407004385582,-1.,3.60072028513845));
#50472=CARTESIAN_POINT('Ctrl Pts',(1.63894676675352,-1.,3.59515368334893));
#50473=CARTESIAN_POINT('Ctrl Pts',(1.6338597145126,-1.,3.58955176627879));
#50474=CARTESIAN_POINT('Ctrl Pts',(1.62881051550745,-1.,3.58391625774343));
#50475=CARTESIAN_POINT('Ctrl Pts',(1.62380329464844,-1.,3.5782545595439));
#50476=CARTESIAN_POINT('Ctrl Pts',(1.61884340915404,-1.,3.57257679609806));
#50477=CARTESIAN_POINT('Ctrl Pts',(1.61393581747514,-1.,3.56689200468387));
#50478=CARTESIAN_POINT('Ctrl Pts',(1.60908344685457,-1.,3.5612043248298));
#50479=CARTESIAN_POINT('Ctrl Pts',(1.60428584699853,-1.,3.55550985096129));
#50480=CARTESIAN_POINT('Ctrl Pts',(1.59953698113457,-1.,3.54979148634454));
#50481=CARTESIAN_POINT('Ctrl Pts',(1.59482766949766,-1.,3.54402458182337));
#50482=CARTESIAN_POINT('Ctrl Pts',(1.59014958368739,-1.,3.53818616861077));
#50483=CARTESIAN_POINT('Ctrl Pts',(1.58549906268088,-1.,3.5322637814708));
#50484=CARTESIAN_POINT('Ctrl Pts',(1.58088027227848,-1.,3.52626275334881));
#50485=CARTESIAN_POINT('Ctrl Pts',(1.57631049988158,-1.,3.52021847865912));
#50486=CARTESIAN_POINT('Ctrl Pts',(1.57181569799743,-1.,3.51418598431665));
#50487=CARTESIAN_POINT('Ctrl Pts',(1.56742097575012,-1.,3.50821771695363));
#50488=CARTESIAN_POINT('Ctrl Pts',(1.56314187758675,-1.,3.50234321621578));
#50489=CARTESIAN_POINT('Ctrl Pts',(1.55897703097874,-1.,3.49655185179655));
#50490=CARTESIAN_POINT('Ctrl Pts',(1.55489595901116,-1.,3.4907646087742));
#50491=CARTESIAN_POINT('Ctrl Pts',(1.55084702970452,-1.,3.48485155928567));
#50492=CARTESIAN_POINT('Ctrl Pts',(1.54678009290276,-1.,3.47868272898751));
#50493=CARTESIAN_POINT('Ctrl Pts',(1.54266605398187,-1.,3.47217189224653));
#50494=CARTESIAN_POINT('Ctrl Pts',(1.53851507915502,-1.,3.46531752207153));
#50495=CARTESIAN_POINT('Ctrl Pts',(1.53440195378792,-1.,3.45825932955032));
#50496=CARTESIAN_POINT('Ctrl Pts',(1.53046244461635,-1.,3.45127136828305));
#50497=CARTESIAN_POINT('Ctrl Pts',(1.52686242875556,-1.,3.44469547526647));
#50498=CARTESIAN_POINT('Ctrl Pts',(1.5237734895035,-1.,3.4388889597401));
#50499=CARTESIAN_POINT('Ctrl Pts',(1.52134826724292,-1.,3.43417156977893));
#50500=CARTESIAN_POINT('Ctrl Pts',(1.5198144909338,-1.,3.43101631893414));
#50501=CARTESIAN_POINT('Ctrl Pts',(1.51914806898491,-1.,3.42946838852587));
#50502=CARTESIAN_POINT('Ctrl Pts',(1.5189513329503,-1.,3.42884302333841));
#50503=CARTESIAN_POINT('Ctrl Pts',(1.51893924967331,-1.,3.42864616361875));
#50504=CARTESIAN_POINT('Ctrl Pts',(1.5189508286633,-1.,3.42859860294306));
#50505=CARTESIAN_POINT('',(1.35032489087269,-1.,3.49844575334386));
#50506=CARTESIAN_POINT('Origin',(0.,-1.,0.));
#50507=CARTESIAN_POINT('',(1.36999806084572,-1.,3.97027773754922));
#50508=CARTESIAN_POINT('Ctrl Pts',(1.35032489087269,-1.,3.49844575334386));
#50509=CARTESIAN_POINT('Ctrl Pts',(1.35036670893102,-1.,3.49847119623841));
#50510=CARTESIAN_POINT('Ctrl Pts',(1.35049736560633,-1.,3.49861894124915));
#50511=CARTESIAN_POINT('Ctrl Pts',(1.35080045218652,-1.,3.49920025459856));
#50512=CARTESIAN_POINT('Ctrl Pts',(1.35142377279535,-1.,3.5007660381658));
#50513=CARTESIAN_POINT('Ctrl Pts',(1.3525703284343,-1.,3.50408168106113));
#50514=CARTESIAN_POINT('Ctrl Pts',(1.35419113576022,-1.,3.50913227060177));
#50515=CARTESIAN_POINT('Ctrl Pts',(1.35611275237288,-1.,3.51542230699919));
#50516=CARTESIAN_POINT('Ctrl Pts',(1.35821701528975,-1.,3.52261776117121));
#50517=CARTESIAN_POINT('Ctrl Pts',(1.36037259643827,-1.,3.53034464961849));
#50518=CARTESIAN_POINT('Ctrl Pts',(1.36245507339334,-1.,3.53824396425032));
#50519=CARTESIAN_POINT('Ctrl Pts',(1.36436666257567,-1.,3.54602591832893));
#50520=CARTESIAN_POINT('Ctrl Pts',(1.36606145456711,-1.,3.55353883995793));
#50521=CARTESIAN_POINT('Ctrl Pts',(1.36754771771174,-1.,3.56077662028492));
#50522=CARTESIAN_POINT('Ctrl Pts',(1.36886584973349,-1.,3.56782080304554));
#50523=CARTESIAN_POINT('Ctrl Pts',(1.37007229485646,-1.,3.57479875549453));
#50524=CARTESIAN_POINT('Ctrl Pts',(1.37122241663073,-1.,3.58183885982745));
#50525=CARTESIAN_POINT('Ctrl Pts',(1.37235053661,-1.,3.5890185384643));
#50526=CARTESIAN_POINT('Ctrl Pts',(1.37346320103184,-1.,3.59634627869117));
#50527=CARTESIAN_POINT('Ctrl Pts',(1.37455051379642,-1.,3.60379020124038));
#50528=CARTESIAN_POINT('Ctrl Pts',(1.37559314436641,-1.,3.61129546591082));
#50529=CARTESIAN_POINT('Ctrl Pts',(1.37657053403102,-1.,3.61880481160408));
#50530=CARTESIAN_POINT('Ctrl Pts',(1.37746987919868,-1.,3.62628098665112));
#50531=CARTESIAN_POINT('Ctrl Pts',(1.37829035457324,-1.,3.63371727442448));
#50532=CARTESIAN_POINT('Ctrl Pts',(1.37903818567347,-1.,3.64112507791112));
#50533=CARTESIAN_POINT('Ctrl Pts',(1.37972372481598,-1.,3.64852652756444));
#50534=CARTESIAN_POINT('Ctrl Pts',(1.38035791051215,-1.,3.65594554404396));
#50535=CARTESIAN_POINT('Ctrl Pts',(1.38094856333558,-1.,3.66339848520874));
#50536=CARTESIAN_POINT('Ctrl Pts',(1.38149812653876,-1.,3.67088843112282));
#50537=CARTESIAN_POINT('Ctrl Pts',(1.38200574290626,-1.,3.6784103848243));
#50538=CARTESIAN_POINT('Ctrl Pts',(1.38246852827185,-1.,3.68595444983844));
#50539=CARTESIAN_POINT('Ctrl Pts',(1.38288311171649,-1.,3.69350967899523));
#50540=CARTESIAN_POINT('Ctrl Pts',(1.38324717612862,-1.,3.70106792167894));
#50541=CARTESIAN_POINT('Ctrl Pts',(1.38356065402122,-1.,3.70862680753343));
#50542=CARTESIAN_POINT('Ctrl Pts',(1.38382489984585,-1.,3.7161876605181));
#50543=CARTESIAN_POINT('Ctrl Pts',(1.3840421342895,-1.,3.72375409358805));
#50544=CARTESIAN_POINT('Ctrl Pts',(1.38421479111531,-1.,3.73133035859283));
#50545=CARTESIAN_POINT('Ctrl Pts',(1.38434489156456,-1.,3.73891976418099));
#50546=CARTESIAN_POINT('Ctrl Pts',(1.38443344984389,-1.,3.7465231716786));
#50547=CARTESIAN_POINT('Ctrl Pts',(1.38448077997155,-1.,3.75413976318727));
#50548=CARTESIAN_POINT('Ctrl Pts',(1.38448675253343,-1.,3.76176768271347));
#50549=CARTESIAN_POINT('Ctrl Pts',(1.38445107339517,-1.,3.76940473185775));
#50550=CARTESIAN_POINT('Ctrl Pts',(1.38437354551435,-1.,3.77704902230441));
#50551=CARTESIAN_POINT('Ctrl Pts',(1.38425435883773,-1.,3.78469969805134));
#50552=CARTESIAN_POINT('Ctrl Pts',(1.38409399694588,-1.,3.79235669640907));
#50553=CARTESIAN_POINT('Ctrl Pts',(1.38389311766701,-1.,3.80002044322169));
#50554=CARTESIAN_POINT('Ctrl Pts',(1.38365244046226,-1.,3.80769156398429));
#50555=CARTESIAN_POINT('Ctrl Pts',(1.38337263902766,-1.,3.81537060817765));
#50556=CARTESIAN_POINT('Ctrl Pts',(1.38305421262724,-1.,3.82305771743715));
#50557=CARTESIAN_POINT('Ctrl Pts',(1.38269750245086,-1.,3.83075266982138));
#50558=CARTESIAN_POINT('Ctrl Pts',(1.38230274828774,-1.,3.83845502790609));
#50559=CARTESIAN_POINT('Ctrl Pts',(1.38187013346089,-1.,3.84616425605705));
#50560=CARTESIAN_POINT('Ctrl Pts',(1.38139983115075,-1.,3.85387983979557));
#50561=CARTESIAN_POINT('Ctrl Pts',(1.38089205993067,-1.,3.86160143044187));
#50562=CARTESIAN_POINT('Ctrl Pts',(1.38034709213129,-1.,3.86932885813403));
#50563=CARTESIAN_POINT('Ctrl Pts',(1.37976523097187,-1.,3.87706205830865));
#50564=CARTESIAN_POINT('Ctrl Pts',(1.37914679719446,-1.,3.88480102249461));
#50565=CARTESIAN_POINT('Ctrl Pts',(1.37849211287981,-1.,3.89254574338385));
#50566=CARTESIAN_POINT('Ctrl Pts',(1.3778014851263,-1.,3.90029615196255));
#50567=CARTESIAN_POINT('Ctrl Pts',(1.3770751963376,-1.,3.90805209522729));
#50568=CARTESIAN_POINT('Ctrl Pts',(1.37631350505516,-1.,3.91581337461825));
#50569=CARTESIAN_POINT('Ctrl Pts',(1.37551664448057,-1.,3.92357976987132));
#50570=CARTESIAN_POINT('Ctrl Pts',(1.37468482215784,-1.,3.93135106761941));
#50571=CARTESIAN_POINT('Ctrl Pts',(1.37381821967499,-1.,3.93912709041791));
#50572=CARTESIAN_POINT('Ctrl Pts',(1.37291699203423,-1.,3.94690771786926));
#50573=CARTESIAN_POINT('Ctrl Pts',(1.37198126433139,-1.,3.95469287283105));
#50574=CARTESIAN_POINT('Ctrl Pts',(1.37120515615663,-1.,3.96092458508407));
#50575=CARTESIAN_POINT('Ctrl Pts',(1.37060761746027,-1.,3.96560037975788));
#50576=CARTESIAN_POINT('Ctrl Pts',(1.37020239094758,-1.,3.9687184694173));
#50577=CARTESIAN_POINT('Ctrl Pts',(1.36999806084572,-1.,3.97027773754922));
#50578=CARTESIAN_POINT('',(1.22531898815164,-1.,4.01728681790024));
#50579=CARTESIAN_POINT('',(1.36999806084572,-1.,3.97027773754922));
#50580=CARTESIAN_POINT('',(0.963899035118985,-1.,3.62400312501199));
#50581=CARTESIAN_POINT('Ctrl Pts',(1.22531898815164,-1.,4.01728681790024));
#50582=CARTESIAN_POINT('Ctrl Pts',(1.22423716681317,-1.,4.01614544569895));
#50583=CARTESIAN_POINT('Ctrl Pts',(1.22207656455845,-1.,4.01386104433519));
#50584=CARTESIAN_POINT('Ctrl Pts',(1.21884478244403,-1.,4.01042947140789));
#50585=CARTESIAN_POINT('Ctrl Pts',(1.21455398918133,-1.,4.00584409522722));
#50586=CARTESIAN_POINT('Ctrl Pts',(1.20922097029551,-1.,4.00009577950721));
#50587=CARTESIAN_POINT('Ctrl Pts',(1.20391852375138,-1.,3.99433084799666));
#50588=CARTESIAN_POINT('Ctrl Pts',(1.19864679609566,-1.,3.98854928957189));
#50589=CARTESIAN_POINT('Ctrl Pts',(1.19340598349475,-1.,3.98275111052561));
#50590=CARTESIAN_POINT('Ctrl Pts',(1.18819633715539,-1.,3.97693634767754));
#50591=CARTESIAN_POINT('Ctrl Pts',(1.18301815039831,-1.,3.97110505165415));
#50592=CARTESIAN_POINT('Ctrl Pts',(1.17787174135592,-1.,3.96525726358159));
#50593=CARTESIAN_POINT('Ctrl Pts',(1.17275743590361,-1.,3.95939299213276));
#50594=CARTESIAN_POINT('Ctrl Pts',(1.16767555244438,-1.,3.95351219509876));
#50595=CARTESIAN_POINT('Ctrl Pts',(1.16262637999157,-1.,3.94761474780583));
#50596=CARTESIAN_POINT('Ctrl Pts',(1.15761018340956,-1.,3.94170046685203));
#50597=CARTESIAN_POINT('Ctrl Pts',(1.1526272271632,-1.,3.9357691705628));
#50598=CARTESIAN_POINT('Ctrl Pts',(1.14767779451123,-1.,3.92982073294257));
#50599=CARTESIAN_POINT('Ctrl Pts',(1.14276220561593,-1.,3.92385513133997));
#50600=CARTESIAN_POINT('Ctrl Pts',(1.13788084225554,-1.,3.91787251936827));
#50601=CARTESIAN_POINT('Ctrl Pts',(1.13303414693896,-1.,3.91187321145649));
#50602=CARTESIAN_POINT('Ctrl Pts',(1.12822258281553,-1.,3.90585753318737));
#50603=CARTESIAN_POINT('Ctrl Pts',(1.12344660099043,-1.,3.89982569750025));
#50604=CARTESIAN_POINT('Ctrl Pts',(1.11870660794603,-1.,3.89377768340344));
#50605=CARTESIAN_POINT('Ctrl Pts',(1.11400292434429,-1.,3.88771308285171));
#50606=CARTESIAN_POINT('Ctrl Pts',(1.10933577224008,-1.,3.88163105531724));
#50607=CARTESIAN_POINT('Ctrl Pts',(1.10470536603287,-1.,3.87553067187514));
#50608=CARTESIAN_POINT('Ctrl Pts',(1.10011198761195,-1.,3.86941120134849));
#50609=CARTESIAN_POINT('Ctrl Pts',(1.09555606505013,-1.,3.86327241021247));
#50610=CARTESIAN_POINT('Ctrl Pts',(1.09103825516294,-1.,3.85711487933931));
#50611=CARTESIAN_POINT('Ctrl Pts',(1.08655950846384,-1.,3.85094025222713));
#50612=CARTESIAN_POINT('Ctrl Pts',(1.08212087917991,-1.,3.8447504803063));
#50613=CARTESIAN_POINT('Ctrl Pts',(1.07772335353858,-1.,3.83854714117491));
#50614=CARTESIAN_POINT('Ctrl Pts',(1.07336766633459,-1.,3.83233071195144));
#50615=CARTESIAN_POINT('Ctrl Pts',(1.06905413180359,-1.,3.82609989967276));
#50616=CARTESIAN_POINT('Ctrl Pts',(1.0647824403893,-1.,3.81985083953012));
#50617=CARTESIAN_POINT('Ctrl Pts',(1.06055206187299,-1.,3.8135786611749));
#50618=CARTESIAN_POINT('Ctrl Pts',(1.05636266918644,-1.,3.80727913637791));
#50619=CARTESIAN_POINT('Ctrl Pts',(1.05221457990016,-1.,3.80095039790681));
#50620=CARTESIAN_POINT('Ctrl Pts',(1.04810913267639,-1.,3.79459440308786));
#50621=CARTESIAN_POINT('Ctrl Pts',(1.04404924374422,-1.,3.78821910787179));
#50622=CARTESIAN_POINT('Ctrl Pts',(1.04003862055798,-1.,3.7818353500817));
#50623=CARTESIAN_POINT('Ctrl Pts',(1.03608074678008,-1.,3.77545283140427));
#50624=CARTESIAN_POINT('Ctrl Pts',(1.03217786604919,-1.,3.76907609832516));
#50625=CARTESIAN_POINT('Ctrl Pts',(1.02833014458184,-1.,3.76270122291245));
#50626=CARTESIAN_POINT('Ctrl Pts',(1.02453429444668,-1.,3.75631037456224));
#50627=CARTESIAN_POINT('Ctrl Pts',(1.02078510487439,-1.,3.74987777155873));
#50628=CARTESIAN_POINT('Ctrl Pts',(1.01707794311088,-1.,3.74337942504993));
#50629=CARTESIAN_POINT('Ctrl Pts',(1.01341114319906,-1.,3.73680245055747));
#50630=CARTESIAN_POINT('Ctrl Pts',(1.00978798539491,-1.,3.73015276704407));
#50631=CARTESIAN_POINT('Ctrl Pts',(1.00622000735696,-1.,3.72346803750544));
#50632=CARTESIAN_POINT('Ctrl Pts',(1.00272423396802,-1.,3.71680667125047));
#50633=CARTESIAN_POINT('Ctrl Pts',(0.999317260756344,-1.,3.7102243971387));
#50634=CARTESIAN_POINT('Ctrl Pts',(0.996009819772431,-1.,3.70375282282107));
#50635=CARTESIAN_POINT('Ctrl Pts',(0.992802218332103,-1.,3.69738123415696));
#50636=CARTESIAN_POINT('Ctrl Pts',(0.989676715398858,-1.,3.69102682138955));
#50637=CARTESIAN_POINT('Ctrl Pts',(0.986602639864285,-1.,3.6845531792623));
#50638=CARTESIAN_POINT('Ctrl Pts',(0.983550791470864,-1.,3.67782408841876));
#50639=CARTESIAN_POINT('Ctrl Pts',(0.980505922458494,-1.,3.67074983340444));
#50640=CARTESIAN_POINT('Ctrl Pts',(0.977478312751416,-1.,3.66333049637403));
#50641=CARTESIAN_POINT('Ctrl Pts',(0.974519971354138,-1.,3.6557157673487));
#50642=CARTESIAN_POINT('Ctrl Pts',(0.971722122060277,-1.,3.64819756447072));
#50643=CARTESIAN_POINT('Ctrl Pts',(0.969195124674828,-1.,3.64113946505393));
#50644=CARTESIAN_POINT('Ctrl Pts',(0.967052554540877,-1.,3.6349212208096));
#50645=CARTESIAN_POINT('Ctrl Pts',(0.965395153165715,-1.,3.62988252139998));
#50646=CARTESIAN_POINT('Ctrl Pts',(0.964373850166081,-1.,3.62652618145252));
#50647=CARTESIAN_POINT('Ctrl Pts',(0.963957782642589,-1.,3.62489305727516));
#50648=CARTESIAN_POINT('Ctrl Pts',(0.963861297423578,-1.,3.62424461507455));
#50649=CARTESIAN_POINT('Ctrl Pts',(0.963880158556713,-1.,3.62404828878374));
#50650=CARTESIAN_POINT('Ctrl Pts',(0.963899035118985,-1.,3.62400312501199));
#50651=CARTESIAN_POINT('',(0.786422660833742,-1.,3.66661143271648));
#50652=CARTESIAN_POINT('Origin',(0.,-1.,0.));
#50653=CARTESIAN_POINT('',(0.732042837400619,-1.,4.13571194405636));
#50654=CARTESIAN_POINT('Ctrl Pts',(0.786422660833742,-1.,3.66661143271648));
#50655=CARTESIAN_POINT('Ctrl Pts',(0.786459983896781,-1.,3.66664310415236));
#50656=CARTESIAN_POINT('Ctrl Pts',(0.786565919559889,-1.,3.66680946938396));
#50657=CARTESIAN_POINT('Ctrl Pts',(0.786774337198499,-1.,3.66743103898844));
#50658=CARTESIAN_POINT('Ctrl Pts',(0.787145041181588,-1.,3.66907505398769));
#50659=CARTESIAN_POINT('Ctrl Pts',(0.787758799995426,-1.,3.672529236635));
#50660=CARTESIAN_POINT('Ctrl Pts',(0.788569566220662,-1.,3.67777119516438));
#50661=CARTESIAN_POINT('Ctrl Pts',(0.789483546065158,-1.,3.68428439784285));
#50662=CARTESIAN_POINT('Ctrl Pts',(0.790436284989579,-1.,3.69172044327754));
#50663=CARTESIAN_POINT('Ctrl Pts',(0.791356575696508,-1.,3.69968940808982));
#50664=CARTESIAN_POINT('Ctrl Pts',(0.792177688845967,-1.,3.70781724021879));
#50665=CARTESIAN_POINT('Ctrl Pts',(0.792848377370115,-1.,3.7158024239604));
#50666=CARTESIAN_POINT('Ctrl Pts',(0.79334702378387,-1.,3.7234879729357));
#50667=CARTESIAN_POINT('Ctrl Pts',(0.793682750269347,-1.,3.7308691469564));
#50668=CARTESIAN_POINT('Ctrl Pts',(0.79388270093679,-1.,3.73803280541576));
#50669=CARTESIAN_POINT('Ctrl Pts',(0.79398270045988,-1.,3.74511357728827));
#50670=CARTESIAN_POINT('Ctrl Pts',(0.79401734737144,-1.,3.75224692493895));
#50671=CARTESIAN_POINT('Ctrl Pts',(0.794008429135046,-1.,3.75951468666325));
#50672=CARTESIAN_POINT('Ctrl Pts',(0.793961083689141,-1.,3.76692626931184));
#50673=CARTESIAN_POINT('Ctrl Pts',(0.793870523787515,-1.,3.77444863801264));
#50674=CARTESIAN_POINT('Ctrl Pts',(0.793726235781339,-1.,3.78202460377617));
#50675=CARTESIAN_POINT('Ctrl Pts',(0.793516871680965,-1.,3.78959439439222));
#50676=CARTESIAN_POINT('Ctrl Pts',(0.7932356129732,-1.,3.79711921389862));
#50677=CARTESIAN_POINT('Ctrl Pts',(0.792882695234692,-1.,3.80459229925598));
#50678=CARTESIAN_POINT('Ctrl Pts',(0.792462483517568,-1.,3.81202588694726));
#50679=CARTESIAN_POINT('Ctrl Pts',(0.791981740718606,-1.,3.81944345442237));
#50680=CARTESIAN_POINT('Ctrl Pts',(0.791447528662381,-1.,3.82687033899799));
#50681=CARTESIAN_POINT('Ctrl Pts',(0.790865012705339,-1.,3.83432392054804));
#50682=CARTESIAN_POINT('Ctrl Pts',(0.790236124191289,-1.,3.84180762342476));
#50683=CARTESIAN_POINT('Ctrl Pts',(0.789560798155618,-1.,3.8493163780891));
#50684=CARTESIAN_POINT('Ctrl Pts',(0.788837734090688,-1.,3.85683995872536));
#50685=CARTESIAN_POINT('Ctrl Pts',(0.78806531509377,-1.,3.86436702561342));
#50686=CARTESIAN_POINT('Ctrl Pts',(0.78724252761798,-1.,3.87188916600905));
#50687=CARTESIAN_POINT('Ctrl Pts',(0.786369675812591,-1.,3.87940402818186));
#50688=CARTESIAN_POINT('Ctrl Pts',(0.785447890340723,-1.,3.88691313167399));
#50689=CARTESIAN_POINT('Ctrl Pts',(0.784478799358335,-1.,3.89442039235105));
#50690=CARTESIAN_POINT('Ctrl Pts',(0.783464141529082,-1.,3.90193039043971));
#50691=CARTESIAN_POINT('Ctrl Pts',(0.782405395622758,-1.,3.90944671004536));
#50692=CARTESIAN_POINT('Ctrl Pts',(0.781303428618343,-1.,3.9169703605466));
#50693=CARTESIAN_POINT('Ctrl Pts',(0.780158678615506,-1.,3.92450058323799));
#50694=CARTESIAN_POINT('Ctrl Pts',(0.778971308134786,-1.,3.93203552473153));
#50695=CARTESIAN_POINT('Ctrl Pts',(0.777741370568549,-1.,3.93957296768098));
#50696=CARTESIAN_POINT('Ctrl Pts',(0.776468966697959,-1.,3.94711101619471));
#50697=CARTESIAN_POINT('Ctrl Pts',(0.775154418039441,-1.,3.95464885452364));
#50698=CARTESIAN_POINT('Ctrl Pts',(0.773798212026682,-1.,3.96218649639876));
#50699=CARTESIAN_POINT('Ctrl Pts',(0.772400931772238,-1.,3.96972446532832));
#50700=CARTESIAN_POINT('Ctrl Pts',(0.770963190030503,-1.,3.97726349165507));
#50701=CARTESIAN_POINT('Ctrl Pts',(0.769485566245459,-1.,3.98480422348403));
#50702=CARTESIAN_POINT('Ctrl Pts',(0.767968531377707,-1.,3.99234687880892));
#50703=CARTESIAN_POINT('Ctrl Pts',(0.766412457135785,-1.,3.99989129179464));
#50704=CARTESIAN_POINT('Ctrl Pts',(0.764817648784946,-1.,4.00743706791366));
#50705=CARTESIAN_POINT('Ctrl Pts',(0.763184371182826,-1.,4.01498370680434));
#50706=CARTESIAN_POINT('Ctrl Pts',(0.761512875859941,-1.,4.02253072741347));
#50707=CARTESIAN_POINT('Ctrl Pts',(0.759803433244165,-1.,4.0300778195465));
#50708=CARTESIAN_POINT('Ctrl Pts',(0.758056338885553,-1.,4.03762485803468));
#50709=CARTESIAN_POINT('Ctrl Pts',(0.756271902370186,-1.,4.04517182654344));
#50710=CARTESIAN_POINT('Ctrl Pts',(0.754450441816411,-1.,4.05271876688106));
#50711=CARTESIAN_POINT('Ctrl Pts',(0.752592276482868,-1.,4.06026572221399));
#50712=CARTESIAN_POINT('Ctrl Pts',(0.750697720483175,-1.,4.06781267241886));
#50713=CARTESIAN_POINT('Ctrl Pts',(0.748767076679176,-1.,4.07535951055363));
#50714=CARTESIAN_POINT('Ctrl Pts',(0.746800631490821,-1.,4.08290608094789));
#50715=CARTESIAN_POINT('Ctrl Pts',(0.744798649705513,-1.,4.09045220253011));
#50716=CARTESIAN_POINT('Ctrl Pts',(0.742761369690017,-1.,4.09799769702712));
#50717=CARTESIAN_POINT('Ctrl Pts',(0.740688998555151,-1.,4.1055424175856));
#50718=CARTESIAN_POINT('Ctrl Pts',(0.738581708229118,-1.,4.11308626953795));
#50719=CARTESIAN_POINT('Ctrl Pts',(0.736439634335347,-1.,4.12062919626082));
#50720=CARTESIAN_POINT('Ctrl Pts',(0.734698226767512,-1.,4.12666277572794));
#50721=CARTESIAN_POINT('Ctrl Pts',(0.733376589325634,-1.,4.13118752796397));
#50722=CARTESIAN_POINT('Ctrl Pts',(0.732488575135925,-1.,4.13420383737278));
#50723=CARTESIAN_POINT('Ctrl Pts',(0.732042837400619,-1.,4.13571194405636));
#50724=CARTESIAN_POINT('',(0.581791163835814,-1.,4.15950947128175));
#50725=CARTESIAN_POINT('',(0.732042837400619,-1.,4.13571194405636));
#50726=CARTESIAN_POINT('',(0.385112848332549,-1.,3.73017266276632));
#50727=CARTESIAN_POINT('Ctrl Pts',(0.581791163835814,-1.,4.15950947128175));
#50728=CARTESIAN_POINT('Ctrl Pts',(0.580901211462913,-1.,4.15821291712391));
#50729=CARTESIAN_POINT('Ctrl Pts',(0.579124568912543,-1.,4.15561864787379));
#50730=CARTESIAN_POINT('Ctrl Pts',(0.576469391673916,-1.,4.1517237611974));
#50731=CARTESIAN_POINT('Ctrl Pts',(0.572948736066276,-1.,4.14652361065787));
#50732=CARTESIAN_POINT('Ctrl Pts',(0.568580610187115,-1.,4.14001179828669));
#50733=CARTESIAN_POINT('Ctrl Pts',(0.564245279535705,-1.,4.13348835726086));
#50734=CARTESIAN_POINT('Ctrl Pts',(0.559942890594628,-1.,4.12695329951859));
#50735=CARTESIAN_POINT('Ctrl Pts',(0.555673636130778,-1.,4.1204066619623));
#50736=CARTESIAN_POINT('Ctrl Pts',(0.551437758498246,-1.,4.11384852025578));
#50737=CARTESIAN_POINT('Ctrl Pts',(0.547235539486759,-1.,4.1072789702877));
#50738=CARTESIAN_POINT('Ctrl Pts',(0.543067286878457,-1.,4.10069810244473));
#50739=CARTESIAN_POINT('Ctrl Pts',(0.53893332117992,-1.,4.09410597627116));
#50740=CARTESIAN_POINT('Ctrl Pts',(0.534833963476999,-1.,4.08750259988693));
#50741=CARTESIAN_POINT('Ctrl Pts',(0.530769518728075,-1.,4.08088789536488));
#50742=CARTESIAN_POINT('Ctrl Pts',(0.526740277226999,-1.,4.07426172299496));
#50743=CARTESIAN_POINT('Ctrl Pts',(0.522746528602767,-1.,4.06762394471075));
#50744=CARTESIAN_POINT('Ctrl Pts',(0.518788572336809,-1.,4.06097448037934));
#50745=CARTESIAN_POINT('Ctrl Pts',(0.514866728193103,-1.,4.05431335771261));
#50746=CARTESIAN_POINT('Ctrl Pts',(0.510981349219173,-1.,4.04764078815591));
#50747=CARTESIAN_POINT('Ctrl Pts',(0.507132823288361,-1.,4.04095715149074));
#50748=CARTESIAN_POINT('Ctrl Pts',(0.503321556915513,-1.,4.0342628417439));
#50749=CARTESIAN_POINT('Ctrl Pts',(0.499547962340889,-1.,4.0275581398015));
#50750=CARTESIAN_POINT('Ctrl Pts',(0.495812444326222,-1.,4.02084308851813));
#50751=CARTESIAN_POINT('Ctrl Pts',(0.49211538341793,-1.,4.01411733503486));
#50752=CARTESIAN_POINT('Ctrl Pts',(0.48845713042453,-1.,4.0073800839092));
#50753=CARTESIAN_POINT('Ctrl Pts',(0.484838042421754,-1.,4.00063045119234));
#50754=CARTESIAN_POINT('Ctrl Pts',(0.481258512209637,-1.,3.99386775880655));
#50755=CARTESIAN_POINT('Ctrl Pts',(0.477718999122033,-1.,3.98709184306743));
#50756=CARTESIAN_POINT('Ctrl Pts',(0.474220061019542,-1.,3.9803033804443));
#50757=CARTESIAN_POINT('Ctrl Pts',(0.470762379613477,-1.,3.97350414289415));
#50758=CARTESIAN_POINT('Ctrl Pts',(0.467346690880671,-1.,3.96669622273946));
#50759=CARTESIAN_POINT('Ctrl Pts',(0.463973722115744,-1.,3.95988133243543));
#50760=CARTESIAN_POINT('Ctrl Pts',(0.460644124429119,-1.,3.95306005817363));
#50761=CARTESIAN_POINT('Ctrl Pts',(0.457358410451673,-1.,3.94623117206675));
#50762=CARTESIAN_POINT('Ctrl Pts',(0.454116879027575,-1.,3.93939080846298));
#50763=CARTESIAN_POINT('Ctrl Pts',(0.450919768356346,-1.,3.93253407403128));
#50764=CARTESIAN_POINT('Ctrl Pts',(0.447767416837296,-1.,3.92565674143424));
#50765=CARTESIAN_POINT('Ctrl Pts',(0.444660430230592,-1.,3.91875701610721));
#50766=CARTESIAN_POINT('Ctrl Pts',(0.441599824524047,-1.,3.91183704069146));
#50767=CARTESIAN_POINT('Ctrl Pts',(0.438587235458233,-1.,3.90490512938546));
#50768=CARTESIAN_POINT('Ctrl Pts',(0.435624629433505,-1.,3.8979725665544));
#50769=CARTESIAN_POINT('Ctrl Pts',(0.432713929544439,-1.,3.89104947940592));
#50770=CARTESIAN_POINT('Ctrl Pts',(0.429856640579733,-1.,3.88414070943334));
#50771=CARTESIAN_POINT('Ctrl Pts',(0.427053541173469,-1.,3.87724240306609));
#50772=CARTESIAN_POINT('Ctrl Pts',(0.424304173195142,-1.,3.87033643487882));
#50773=CARTESIAN_POINT('Ctrl Pts',(0.421607423177575,-1.,3.86339652542749));
#50774=CARTESIAN_POINT('Ctrl Pts',(0.418962468086809,-1.,3.85639825648031));
#50775=CARTESIAN_POINT('Ctrl Pts',(0.41636967805292,-1.,3.8493286415751));
#50776=CARTESIAN_POINT('Ctrl Pts',(0.413831367016726,-1.,3.84219403994742));
#50777=CARTESIAN_POINT('Ctrl Pts',(0.411353038798459,-1.,3.83503345578645));
#50778=CARTESIAN_POINT('Ctrl Pts',(0.408942371447376,-1.,3.82790724256397));
#50779=CARTESIAN_POINT('Ctrl Pts',(0.406607038258906,-1.,3.82087303913741));
#50780=CARTESIAN_POINT('Ctrl Pts',(0.404352694628236,-1.,3.81396374287762));
#50781=CARTESIAN_POINT('Ctrl Pts',(0.402181320148474,-1.,3.80716881962763));
#50782=CARTESIAN_POINT('Ctrl Pts',(0.400088346504726,-1.,3.80040370384659));
#50783=CARTESIAN_POINT('Ctrl Pts',(0.398064818684158,-1.,3.79352887163457));
#50784=CARTESIAN_POINT('Ctrl Pts',(0.396103205335028,-1.,3.78640521279479));
#50785=CARTESIAN_POINT('Ctrl Pts',(0.394202481011595,-1.,3.77894173114368));
#50786=CARTESIAN_POINT('Ctrl Pts',(0.392372786223346,-1.,3.77114011595892));
#50787=CARTESIAN_POINT('Ctrl Pts',(0.390642072979258,-1.,3.76315635032993));
#50788=CARTESIAN_POINT('Ctrl Pts',(0.38905477589825,-1.,3.75529302894757));
#50789=CARTESIAN_POINT('Ctrl Pts',(0.387663020050396,-1.,3.74792651696269));
#50790=CARTESIAN_POINT('Ctrl Pts',(0.386519576222035,-1.,3.74144965781088));
#50791=CARTESIAN_POINT('Ctrl Pts',(0.385670806454744,-1.,3.73621371845475));
#50792=CARTESIAN_POINT('Ctrl Pts',(0.385187124633964,-1.,3.73273893363318));
#50793=CARTESIAN_POINT('Ctrl Pts',(0.385031656499141,-1.,3.73106082862399));
#50794=CARTESIAN_POINT('Ctrl Pts',(0.385037797882046,-1.,3.73040527620929));
#50795=CARTESIAN_POINT('Ctrl Pts',(0.385087139001608,-1.,3.73021431755218));
#50796=CARTESIAN_POINT('Ctrl Pts',(0.385112848332549,-1.,3.73017266276632));
#50797=CARTESIAN_POINT('',(0.203156094897895,-1.,3.74449296982994));
#50798=CARTESIAN_POINT('Origin',(0.,-1.,0.));
#50799=CARTESIAN_POINT('',(0.0760622897878233,-1.,4.19931119685982));
#50800=CARTESIAN_POINT('Ctrl Pts',(0.203156094897895,-1.,3.74449296982994));
#50801=CARTESIAN_POINT('Ctrl Pts',(0.203188003947964,-1.,3.74453008995129));
#50802=CARTESIAN_POINT('Ctrl Pts',(0.203266610111263,-1.,3.74471097893961));
#50803=CARTESIAN_POINT('Ctrl Pts',(0.203375226874331,-1.,3.74535749969262));
#50804=CARTESIAN_POINT('Ctrl Pts',(0.203484186269314,-1.,3.74703926501843));
#50805=CARTESIAN_POINT('Ctrl Pts',(0.203550035479096,-1.,3.75054693397716));
#50806=CARTESIAN_POINT('Ctrl Pts',(0.203530796848403,-1.,3.75585118707924));
#50807=CARTESIAN_POINT('Ctrl Pts',(0.203414634707646,-1.,3.76242717937273));
#50808=CARTESIAN_POINT('Ctrl Pts',(0.203192390045337,-1.,3.76992071595267));
#50809=CARTESIAN_POINT('Ctrl Pts',(0.202854729699196,-1.,3.77793553476879));
#50810=CARTESIAN_POINT('Ctrl Pts',(0.202394260512192,-1.,3.78609175019317));
#50811=CARTESIAN_POINT('Ctrl Pts',(0.201807533800798,-1.,3.79408354187274));
#50812=CARTESIAN_POINT('Ctrl Pts',(0.201097756307251,-1.,3.80175247447171));
#50813=CARTESIAN_POINT('Ctrl Pts',(0.200274679433289,-1.,3.80909529318501));
#50814=CARTESIAN_POINT('Ctrl Pts',(0.199351525297396,-1.,3.81620203429702));
#50815=CARTESIAN_POINT('Ctrl Pts',(0.198342616900469,-1.,3.82321127348981));
#50816=CARTESIAN_POINT('Ctrl Pts',(0.197260935827375,-1.,3.83026221776488));
#50817=CARTESIAN_POINT('Ctrl Pts',(0.196115198971889,-1.,3.83743910616265));
#50818=CARTESIAN_POINT('Ctrl Pts',(0.194909009460254,-1.,3.84475203347052));
#50819=CARTESIAN_POINT('Ctrl Pts',(0.193642806777747,-1.,3.85216762264019));
#50820=CARTESIAN_POINT('Ctrl Pts',(0.192315153044979,-1.,3.85962774407652));
#50821=CARTESIAN_POINT('Ctrl Pts',(0.190924190418612,-1.,3.8670715862477));
#50822=CARTESIAN_POINT('Ctrl Pts',(0.189469253358254,-1.,3.87445976418377));
#50823=CARTESIAN_POINT('Ctrl Pts',(0.187951632512663,-1.,3.88178563496187));
#50824=CARTESIAN_POINT('Ctrl Pts',(0.186373724985263,-1.,3.88906196725817));
#50825=CARTESIAN_POINT('Ctrl Pts',(0.184738537728034,-1.,3.89631300742633));
#50826=CARTESIAN_POINT('Ctrl Pts',(0.183049081993193,-1.,3.90356488555138));
#50827=CARTESIAN_POINT('Ctrl Pts',(0.181307740731795,-1.,3.91083557557193));
#50828=CARTESIAN_POINT('Ctrl Pts',(0.179515885822894,-1.,3.91812876180948));
#50829=CARTESIAN_POINT('Ctrl Pts',(0.177674246152328,-1.,3.92543942697672));
#50830=CARTESIAN_POINT('Ctrl Pts',(0.175783136893872,-1.,3.93275726771049));
#50831=CARTESIAN_POINT('Ctrl Pts',(0.173842734974607,-1.,3.94007083096214));
#50832=CARTESIAN_POINT('Ctrl Pts',(0.171853355369232,-1.,3.94737164900861));
#50833=CARTESIAN_POINT('Ctrl Pts',(0.16981566637413,-1.,3.95465744665263));
#50834=CARTESIAN_POINT('Ctrl Pts',(0.167730547023312,-1.,3.96192990160296));
#50835=CARTESIAN_POINT('Ctrl Pts',(0.165598992851097,-1.,3.9691931362141));
#50836=CARTESIAN_POINT('Ctrl Pts',(0.163422004609998,-1.,3.97645194630944));
#50837=CARTESIAN_POINT('Ctrl Pts',(0.161200482186087,-1.,3.98371010319866));
#50838=CARTESIAN_POINT('Ctrl Pts',(0.158935123982796,-1.,3.99096873945862));
#50839=CARTESIAN_POINT('Ctrl Pts',(0.156626481393735,-1.,3.99822717425869));
#50840=CARTESIAN_POINT('Ctrl Pts',(0.154275004872309,-1.,4.00548360245297));
#50841=CARTESIAN_POINT('Ctrl Pts',(0.151881094022909,-1.,4.01273584234684));
#50842=CARTESIAN_POINT('Ctrl Pts',(0.149445144968707,-1.,4.01998203715588));
#50843=CARTESIAN_POINT('Ctrl Pts',(0.146967602878998,-1.,4.02722143147048));
#50844=CARTESIAN_POINT('Ctrl Pts',(0.144448947038352,-1.,4.03445411510403));
#50845=CARTESIAN_POINT('Ctrl Pts',(0.141889671485507,-1.,4.04168069633842));
#50846=CARTESIAN_POINT('Ctrl Pts',(0.139290267180059,-1.,4.04890199238056));
#50847=CARTESIAN_POINT('Ctrl Pts',(0.136651205046111,-1.,4.05611873400122));
#50848=CARTESIAN_POINT('Ctrl Pts',(0.133972916144225,-1.,4.06333121018476));
#50849=CARTESIAN_POINT('Ctrl Pts',(0.131255793548914,-1.,4.07053931528579));
#50850=CARTESIAN_POINT('Ctrl Pts',(0.128500200484813,-1.,4.07774270738809));
#50851=CARTESIAN_POINT('Ctrl Pts',(0.125706476822529,-1.,4.08494093372315));
#50852=CARTESIAN_POINT('Ctrl Pts',(0.122874946249119,-1.,4.09213355850836));
#50853=CARTESIAN_POINT('Ctrl Pts',(0.120005924388162,-1.,4.09932031767243));
#50854=CARTESIAN_POINT('Ctrl Pts',(0.117099722731704,-1.,4.10650113382187));
#50855=CARTESIAN_POINT('Ctrl Pts',(0.114156649609601,-1.,4.11367603925313));
#50856=CARTESIAN_POINT('Ctrl Pts',(0.111177012683377,-1.,4.12084512502444));
#50857=CARTESIAN_POINT('Ctrl Pts',(0.10816112052835,-1.,4.12800848371386));
#50858=CARTESIAN_POINT('Ctrl Pts',(0.105109286538864,-1.,4.13516614458396));
#50859=CARTESIAN_POINT('Ctrl Pts',(0.102021826577453,-1.,4.14231804938737));
#50860=CARTESIAN_POINT('Ctrl Pts',(0.0988990478899809,-1.,4.1494640891762));
#50861=CARTESIAN_POINT('Ctrl Pts',(0.0957412403297065,-1.,4.15660412653006));
#50862=CARTESIAN_POINT('Ctrl Pts',(0.0925486672167687,-1.,4.16373802265942));
#50863=CARTESIAN_POINT('Ctrl Pts',(0.0893215560850325,-1.,4.17086566491823));
#50864=CARTESIAN_POINT('Ctrl Pts',(0.0860600915552512,-1.,4.17798698669991));
#50865=CARTESIAN_POINT('Ctrl Pts',(0.0827644164389507,-1.,4.1851019532944));
#50866=CARTESIAN_POINT('Ctrl Pts',(0.08010058871176,-1.,4.19078883322483));
#50867=CARTESIAN_POINT('Ctrl Pts',(0.0780873956244399,-1.,4.19505112860624));
#50868=CARTESIAN_POINT('Ctrl Pts',(0.0767384596142192,-1.,4.19789138621624));
#50869=CARTESIAN_POINT('Ctrl Pts',(0.0760622897878233,-1.,4.19931119685982));
#50870=CARTESIAN_POINT('',(-0.0760622897878249,-1.,4.19931119685982));
#50871=CARTESIAN_POINT('',(0.0760622897878233,-1.,4.19931119685982));
#50872=CARTESIAN_POINT('',(-0.203156094896101,-1.,3.74449296983004));
#50873=CARTESIAN_POINT('Ctrl Pts',(-0.0760622897878249,-1.,4.19931119685982));
#50874=CARTESIAN_POINT('Ctrl Pts',(-0.0767384596141467,-1.,4.1978913862118));
#50875=CARTESIAN_POINT('Ctrl Pts',(-0.07808739562424,-1.,4.19505112859416));
#50876=CARTESIAN_POINT('Ctrl Pts',(-0.0801005887114322,-1.,4.19078883320504));
#50877=CARTESIAN_POINT('Ctrl Pts',(-0.0827644164385681,-1.,4.18510195327123));
#50878=CARTESIAN_POINT('Ctrl Pts',(-0.0860600915549399,-1.,4.17798698668094));
#50879=CARTESIAN_POINT('Ctrl Pts',(-0.0893215560848652,-1.,4.17086566490794));
#50880=CARTESIAN_POINT('Ctrl Pts',(-0.0925486672167534,-1.,4.16373802265839));
#50881=CARTESIAN_POINT('Ctrl Pts',(-0.0957412403298009,-1.,4.15660412653577));
#50882=CARTESIAN_POINT('Ctrl Pts',(-0.0988990478901228,-1.,4.14946408918485));
#50883=CARTESIAN_POINT('Ctrl Pts',(-0.102021826577584,-1.,4.14231804939538));
#50884=CARTESIAN_POINT('Ctrl Pts',(-0.105109286538945,-1.,4.13516614458895));
#50885=CARTESIAN_POINT('Ctrl Pts',(-0.10816112052837,-1.,4.12800848371504));
#50886=CARTESIAN_POINT('Ctrl Pts',(-0.111177012683347,-1.,4.1208451250225));
#50887=CARTESIAN_POINT('Ctrl Pts',(-0.114156649609546,-1.,4.11367603924961));
#50888=CARTESIAN_POINT('Ctrl Pts',(-0.117099722731648,-1.,4.10650113381833));
#50889=CARTESIAN_POINT('Ctrl Pts',(-0.120005924388124,-1.,4.09932031767002));
#50890=CARTESIAN_POINT('Ctrl Pts',(-0.122874946249107,-1.,4.09213355850756));
#50891=CARTESIAN_POINT('Ctrl Pts',(-0.12570647682254,-1.,4.08494093372377));
#50892=CARTESIAN_POINT('Ctrl Pts',(-0.128500200484838,-1.,4.07774270738954));
#50893=CARTESIAN_POINT('Ctrl Pts',(-0.131255793548941,-1.,4.0705393152874));
#50894=CARTESIAN_POINT('Ctrl Pts',(-0.133972916144245,-1.,4.06333121018596));
#50895=CARTESIAN_POINT('Ctrl Pts',(-0.136651205046119,-1.,4.05611873400172));
#50896=CARTESIAN_POINT('Ctrl Pts',(-0.139290267180057,-1.,4.04890199238036));
#50897=CARTESIAN_POINT('Ctrl Pts',(-0.1418896714855,-1.,4.04168069633781));
#50898=CARTESIAN_POINT('Ctrl Pts',(-0.144448947038345,-1.,4.03445411510333));
#50899=CARTESIAN_POINT('Ctrl Pts',(-0.146967602878994,-1.,4.02722143146994));
#50900=CARTESIAN_POINT('Ctrl Pts',(-0.149445144968707,-1.,4.01998203715564));
#50901=CARTESIAN_POINT('Ctrl Pts',(-0.151881094022911,-1.,4.01273584234689));
#50902=CARTESIAN_POINT('Ctrl Pts',(-0.154275004872311,-1.,4.00548360245319));
#50903=CARTESIAN_POINT('Ctrl Pts',(-0.156626481393734,-1.,3.99822717425893));
#50904=CARTESIAN_POINT('Ctrl Pts',(-0.158935123982793,-1.,3.99096873945878));
#50905=CARTESIAN_POINT('Ctrl Pts',(-0.161200482186085,-1.,3.98371010319872));
#50906=CARTESIAN_POINT('Ctrl Pts',(-0.163422004609999,-1.,3.97645194630943));
#50907=CARTESIAN_POINT('Ctrl Pts',(-0.165598992851102,-1.,3.96919313621407));
#50908=CARTESIAN_POINT('Ctrl Pts',(-0.16773054702332,-1.,3.96192990160296));
#50909=CARTESIAN_POINT('Ctrl Pts',(-0.169815666374139,-1.,3.95465744665268));
#50910=CARTESIAN_POINT('Ctrl Pts',(-0.17185335536924,-1.,3.94737164900868));
#50911=CARTESIAN_POINT('Ctrl Pts',(-0.17384273497461,-1.,3.94007083096217));
#50912=CARTESIAN_POINT('Ctrl Pts',(-0.175783136893868,-1.,3.93275726771042));
#50913=CARTESIAN_POINT('Ctrl Pts',(-0.177674246152318,-1.,3.92543942697655));
#50914=CARTESIAN_POINT('Ctrl Pts',(-0.179515885822882,-1.,3.91812876180926));
#50915=CARTESIAN_POINT('Ctrl Pts',(-0.181307740731786,-1.,3.91083557557175));
#50916=CARTESIAN_POINT('Ctrl Pts',(-0.183049081993191,-1.,3.90356488555132));
#50917=CARTESIAN_POINT('Ctrl Pts',(-0.184738537728043,-1.,3.89631300742646));
#50918=CARTESIAN_POINT('Ctrl Pts',(-0.186373724985281,-1.,3.88906196725848));
#50919=CARTESIAN_POINT('Ctrl Pts',(-0.187951632512685,-1.,3.88178563496228));
#50920=CARTESIAN_POINT('Ctrl Pts',(-0.189469253358273,-1.,3.87445976418412));
#50921=CARTESIAN_POINT('Ctrl Pts',(-0.19092419041862,-1.,3.86707158624783));
#50922=CARTESIAN_POINT('Ctrl Pts',(-0.192315153044971,-1.,3.85962774407633));
#50923=CARTESIAN_POINT('Ctrl Pts',(-0.193642806777723,-1.,3.85216762263966));
#50924=CARTESIAN_POINT('Ctrl Pts',(-0.194909009460221,-1.,3.84475203346977));
#50925=CARTESIAN_POINT('Ctrl Pts',(-0.196115198971859,-1.,3.83743910616195));
#50926=CARTESIAN_POINT('Ctrl Pts',(-0.197260935827362,-1.,3.83026221776456));
#50927=CARTESIAN_POINT('Ctrl Pts',(-0.198342616900487,-1.,3.82321127349016));
#50928=CARTESIAN_POINT('Ctrl Pts',(-0.199351525297447,-1.,3.81620203429815));
#50929=CARTESIAN_POINT('Ctrl Pts',(-0.200274679433365,-1.,3.80909529318669));
#50930=CARTESIAN_POINT('Ctrl Pts',(-0.201097756307326,-1.,3.80175247447337));
#50931=CARTESIAN_POINT('Ctrl Pts',(-0.201807533800837,-1.,3.7940835418736));
#50932=CARTESIAN_POINT('Ctrl Pts',(-0.20239426051216,-1.,3.78609175019242));
#50933=CARTESIAN_POINT('Ctrl Pts',(-0.202854729699081,-1.,3.77793553476614));
#50934=CARTESIAN_POINT('Ctrl Pts',(-0.203192390045165,-1.,3.7699207159487));
#50935=CARTESIAN_POINT('Ctrl Pts',(-0.203414634707479,-1.,3.76242717936885));
#50936=CARTESIAN_POINT('Ctrl Pts',(-0.203530796848322,-1.,3.75585118707734));
#50937=CARTESIAN_POINT('Ctrl Pts',(-0.203550035479166,-1.,3.75054693397875));
#50938=CARTESIAN_POINT('Ctrl Pts',(-0.203484186269415,-1.,3.74703926501752));
#50939=CARTESIAN_POINT('Ctrl Pts',(-0.203375226874122,-1.,3.74535749969115));
#50940=CARTESIAN_POINT('Ctrl Pts',(-0.203266610110531,-1.,3.74471097893845));
#50941=CARTESIAN_POINT('Ctrl Pts',(-0.203188003946657,-1.,3.74453008995092));
#50942=CARTESIAN_POINT('Ctrl Pts',(-0.203156094896101,-1.,3.74449296983004));
#50943=CARTESIAN_POINT('',(-0.385112848330762,-1.,3.73017266276651));
#50944=CARTESIAN_POINT('Origin',(0.,-1.,0.));
#50945=CARTESIAN_POINT('',(-0.581791163835815,-1.,4.15950947128175));
#50946=CARTESIAN_POINT('Ctrl Pts',(-0.385112848330762,-1.,3.73017266276651));
#50947=CARTESIAN_POINT('Ctrl Pts',(-0.385087139000375,-1.,3.73021431755274));
#50948=CARTESIAN_POINT('Ctrl Pts',(-0.385037797881504,-1.,3.73040527621055));
#50949=CARTESIAN_POINT('Ctrl Pts',(-0.385031656499164,-1.,3.73106082862548));
#50950=CARTESIAN_POINT('Ctrl Pts',(-0.385187124634206,-1.,3.73273893363406));
#50951=CARTESIAN_POINT('Ctrl Pts',(-0.385670806454566,-1.,3.73621371845318));
#50952=CARTESIAN_POINT('Ctrl Pts',(-0.386519576222251,-1.,3.74144965781276));
#50953=CARTESIAN_POINT('Ctrl Pts',(-0.387663020050836,-1.,3.74792651696654));
#50954=CARTESIAN_POINT('Ctrl Pts',(-0.389054775898702,-1.,3.75529302895152));
#50955=CARTESIAN_POINT('Ctrl Pts',(-0.39064207297956,-1.,3.76315635033257));
#50956=CARTESIAN_POINT('Ctrl Pts',(-0.392372786223433,-1.,3.77114011595967));
#50957=CARTESIAN_POINT('Ctrl Pts',(-0.394202481011499,-1.,3.77894173114283));
#50958=CARTESIAN_POINT('Ctrl Pts',(-0.396103205334841,-1.,3.78640521279313));
#50959=CARTESIAN_POINT('Ctrl Pts',(-0.39806481868397,-1.,3.7935288716329));
#50960=CARTESIAN_POINT('Ctrl Pts',(-0.4000883465046,-1.,3.80040370384546));
#50961=CARTESIAN_POINT('Ctrl Pts',(-0.402181320148436,-1.,3.80716881962728));
#50962=CARTESIAN_POINT('Ctrl Pts',(-0.404352694628273,-1.,3.81396374287793));
#50963=CARTESIAN_POINT('Ctrl Pts',(-0.406607038258985,-1.,3.8208730391381));
#50964=CARTESIAN_POINT('Ctrl Pts',(-0.40894237144746,-1.,3.82790724256471));
#50965=CARTESIAN_POINT('Ctrl Pts',(-0.411353038798519,-1.,3.83503345578698));
#50966=CARTESIAN_POINT('Ctrl Pts',(-0.413831367016748,-1.,3.84219403994762));
#50967=CARTESIAN_POINT('Ctrl Pts',(-0.416369678052907,-1.,3.84932864157497));
#50968=CARTESIAN_POINT('Ctrl Pts',(-0.418962468086773,-1.,3.85639825647996));
#50969=CARTESIAN_POINT('Ctrl Pts',(-0.421607423177534,-1.,3.86339652542709));
#50970=CARTESIAN_POINT('Ctrl Pts',(-0.424304173195111,-1.,3.87033643487851));
#50971=CARTESIAN_POINT('Ctrl Pts',(-0.427053541173457,-1.,3.87724240306597));
#50972=CARTESIAN_POINT('Ctrl Pts',(-0.429856640579741,-1.,3.88414070943341));
#50973=CARTESIAN_POINT('Ctrl Pts',(-0.432713929544458,-1.,3.89104947940611));
#50974=CARTESIAN_POINT('Ctrl Pts',(-0.435624629433528,-1.,3.89797256655462));
#50975=CARTESIAN_POINT('Ctrl Pts',(-0.43858723545825,-1.,3.90490512938563));
#50976=CARTESIAN_POINT('Ctrl Pts',(-0.441599824524054,-1.,3.91183704069153));
#50977=CARTESIAN_POINT('Ctrl Pts',(-0.444660430230591,-1.,3.91875701610719));
#50978=CARTESIAN_POINT('Ctrl Pts',(-0.447767416837293,-1.,3.92565674143416));
#50979=CARTESIAN_POINT('Ctrl Pts',(-0.450919768356348,-1.,3.93253407403123));
#50980=CARTESIAN_POINT('Ctrl Pts',(-0.454116879027584,-1.,3.93939080846298));
#50981=CARTESIAN_POINT('Ctrl Pts',(-0.457358410451683,-1.,3.94623117206678));
#50982=CARTESIAN_POINT('Ctrl Pts',(-0.460644124429121,-1.,3.95306005817364));
#50983=CARTESIAN_POINT('Ctrl Pts',(-0.463973722115733,-1.,3.95988133243538));
#50984=CARTESIAN_POINT('Ctrl Pts',(-0.467346690880643,-1.,3.9666962227393));
#50985=CARTESIAN_POINT('Ctrl Pts',(-0.470762379613439,-1.,3.97350414289392));
#50986=CARTESIAN_POINT('Ctrl Pts',(-0.47422006101951,-1.,3.98030338044409));
#50987=CARTESIAN_POINT('Ctrl Pts',(-0.477718999122027,-1.,3.98709184306738));
#50988=CARTESIAN_POINT('Ctrl Pts',(-0.481258512209675,-1.,3.99386775880679));
#50989=CARTESIAN_POINT('Ctrl Pts',(-0.484838042421835,-1.,4.00063045119288));
#50990=CARTESIAN_POINT('Ctrl Pts',(-0.488457130424633,-1.,4.0073800839099));
#50991=CARTESIAN_POINT('Ctrl Pts',(-0.492115383418018,-1.,4.01411733503546));
#50992=CARTESIAN_POINT('Ctrl Pts',(-0.495812444326251,-1.,4.02084308851832));
#50993=CARTESIAN_POINT('Ctrl Pts',(-0.499547962340821,-1.,4.02755813980101));
#50994=CARTESIAN_POINT('Ctrl Pts',(-0.503321556915346,-1.,4.03426284174272));
#50995=CARTESIAN_POINT('Ctrl Pts',(-0.507132823288136,-1.,4.04095715148915));
#50996=CARTESIAN_POINT('Ctrl Pts',(-0.51098134921897,-1.,4.04764078815447));
#50997=CARTESIAN_POINT('Ctrl Pts',(-0.514866728193017,-1.,4.05431335771199));
#50998=CARTESIAN_POINT('Ctrl Pts',(-0.518788572336924,-1.,4.06097448038013));
#50999=CARTESIAN_POINT('Ctrl Pts',(-0.522746528603107,-1.,4.06762394471314));
#51000=CARTESIAN_POINT('Ctrl Pts',(-0.526740277227498,-1.,4.07426172299847));
#51001=CARTESIAN_POINT('Ctrl Pts',(-0.530769518728571,-1.,4.08088789536836));
#51002=CARTESIAN_POINT('Ctrl Pts',(-0.534833963477273,-1.,4.08750259988885));
#51003=CARTESIAN_POINT('Ctrl Pts',(-0.538933321179756,-1.,4.09410597627));
#51004=CARTESIAN_POINT('Ctrl Pts',(-0.543067286877757,-1.,4.10069810243979));
#51005=CARTESIAN_POINT('Ctrl Pts',(-0.547235539485637,-1.,4.10727897027977));
#51006=CARTESIAN_POINT('Ctrl Pts',(-0.551437758497033,-1.,4.11384852024721));
#51007=CARTESIAN_POINT('Ctrl Pts',(-0.555673636129977,-1.,4.12040666195664));
#51008=CARTESIAN_POINT('Ctrl Pts',(-0.559942890594774,-1.,4.12695329951961));
#51009=CARTESIAN_POINT('Ctrl Pts',(-0.564245279537149,-1.,4.13348835727104));
#51010=CARTESIAN_POINT('Ctrl Pts',(-0.568580610189775,-1.,4.14001179830547));
#51011=CARTESIAN_POINT('Ctrl Pts',(-0.572948736069522,-1.,4.14652361068081));
#51012=CARTESIAN_POINT('Ctrl Pts',(-0.576469391676688,-1.,4.151723761217));
#51013=CARTESIAN_POINT('Ctrl Pts',(-0.579124568914235,-1.,4.15561864788576));
#51014=CARTESIAN_POINT('Ctrl Pts',(-0.580901211463535,-1.,4.1582129171283));
#51015=CARTESIAN_POINT('Ctrl Pts',(-0.581791163835815,-1.,4.15950947128175));
#51016=CARTESIAN_POINT('',(-0.73204283740062,-1.,4.13571194405636));
#51017=CARTESIAN_POINT('',(-0.581791163835815,-1.,4.15950947128175));
#51018=CARTESIAN_POINT('',(-0.786422660831985,-1.,3.66661143271685));
#51019=CARTESIAN_POINT('Ctrl Pts',(-0.73204283740062,-1.,4.13571194405636));
#51020=CARTESIAN_POINT('Ctrl Pts',(-0.73248857513516,-1.,4.1342038373684));
#51021=CARTESIAN_POINT('Ctrl Pts',(-0.733376589323546,-1.,4.13118752795207));
#51022=CARTESIAN_POINT('Ctrl Pts',(-0.734698226764092,-1.,4.12666277570844));
#51023=CARTESIAN_POINT('Ctrl Pts',(-0.736439634331345,-1.,4.120629196238));
#51024=CARTESIAN_POINT('Ctrl Pts',(-0.738581708225844,-1.,4.11308626951927));
#51025=CARTESIAN_POINT('Ctrl Pts',(-0.740688998553377,-1.,4.10554241757547));
#51026=CARTESIAN_POINT('Ctrl Pts',(-0.742761369689841,-1.,4.09799769702611));
#51027=CARTESIAN_POINT('Ctrl Pts',(-0.7447986497065,-1.,4.09045220253573));
#51028=CARTESIAN_POINT('Ctrl Pts',(-0.746800631492315,-1.,4.08290608095642));
#51029=CARTESIAN_POINT('Ctrl Pts',(-0.748767076680557,-1.,4.07535951056152));
#51030=CARTESIAN_POINT('Ctrl Pts',(-0.750697720484036,-1.,4.06781267242378));
#51031=CARTESIAN_POINT('Ctrl Pts',(-0.752592276483072,-1.,4.06026572221515));
#51032=CARTESIAN_POINT('Ctrl Pts',(-0.754450441816078,-1.,4.05271876687915));
#51033=CARTESIAN_POINT('Ctrl Pts',(-0.756271902369581,-1.,4.04517182653997));
#51034=CARTESIAN_POINT('Ctrl Pts',(-0.758056338884944,-1.,4.03762485803119));
#51035=CARTESIAN_POINT('Ctrl Pts',(-0.759803433243752,-1.,4.03007781954412));
#51036=CARTESIAN_POINT('Ctrl Pts',(-0.761512875859804,-1.,4.02253072741268));
#51037=CARTESIAN_POINT('Ctrl Pts',(-0.763184371182935,-1.,4.01498370680496));
#51038=CARTESIAN_POINT('Ctrl Pts',(-0.764817648785198,-1.,4.00743706791509));
#51039=CARTESIAN_POINT('Ctrl Pts',(-0.766412457136064,-1.,3.99989129179622));
#51040=CARTESIAN_POINT('Ctrl Pts',(-0.767968531377915,-1.,3.9923468788101));
#51041=CARTESIAN_POINT('Ctrl Pts',(-0.769485566245544,-1.,3.98480422348451));
#51042=CARTESIAN_POINT('Ctrl Pts',(-0.770963190030471,-1.,3.97726349165488));
#51043=CARTESIAN_POINT('Ctrl Pts',(-0.772400931772136,-1.,3.96972446532772));
#51044=CARTESIAN_POINT('Ctrl Pts',(-0.773798212026566,-1.,3.96218649639807));
#51045=CARTESIAN_POINT('Ctrl Pts',(-0.775154418039352,-1.,3.9546488545231));
#51046=CARTESIAN_POINT('Ctrl Pts',(-0.776468966697921,-1.,3.94711101619447));
#51047=CARTESIAN_POINT('Ctrl Pts',(-0.777741370568559,-1.,3.93957296768103));
#51048=CARTESIAN_POINT('Ctrl Pts',(-0.778971308134821,-1.,3.93203552473174));
#51049=CARTESIAN_POINT('Ctrl Pts',(-0.780158678615543,-1.,3.92450058323823));
#51050=CARTESIAN_POINT('Ctrl Pts',(-0.781303428618367,-1.,3.91697036054676));
#51051=CARTESIAN_POINT('Ctrl Pts',(-0.782405395622764,-1.,3.90944671004542));
#51052=CARTESIAN_POINT('Ctrl Pts',(-0.783464141529081,-1.,3.9019303904397));
#51053=CARTESIAN_POINT('Ctrl Pts',(-0.784478799358336,-1.,3.89442039235103));
#51054=CARTESIAN_POINT('Ctrl Pts',(-0.78544789034073,-1.,3.88691313167398));
#51055=CARTESIAN_POINT('Ctrl Pts',(-0.786369675812609,-1.,3.8794040281819));
#51056=CARTESIAN_POINT('Ctrl Pts',(-0.787242527617999,-1.,3.87188916600912));
#51057=CARTESIAN_POINT('Ctrl Pts',(-0.788065315093778,-1.,3.86436702561345));
#51058=CARTESIAN_POINT('Ctrl Pts',(-0.788837734090672,-1.,3.85683995872529));
#51059=CARTESIAN_POINT('Ctrl Pts',(-0.789560798155582,-1.,3.84931637808894));
#51060=CARTESIAN_POINT('Ctrl Pts',(-0.790236124191242,-1.,3.84180762342454));
#51061=CARTESIAN_POINT('Ctrl Pts',(-0.790865012705301,-1.,3.83432392054786));
#51062=CARTESIAN_POINT('Ctrl Pts',(-0.791447528662369,-1.,3.82687033899792));
#51063=CARTESIAN_POINT('Ctrl Pts',(-0.791981740718635,-1.,3.81944345442249));
#51064=CARTESIAN_POINT('Ctrl Pts',(-0.792462483517634,-1.,3.81202588694756));
#51065=CARTESIAN_POINT('Ctrl Pts',(-0.792882695234778,-1.,3.80459229925637));
#51066=CARTESIAN_POINT('Ctrl Pts',(-0.793235612973273,-1.,3.79711921389897));
#51067=CARTESIAN_POINT('Ctrl Pts',(-0.793516871680993,-1.,3.78959439439235));
#51068=CARTESIAN_POINT('Ctrl Pts',(-0.7937262357813,-1.,3.78202460377598));
#51069=CARTESIAN_POINT('Ctrl Pts',(-0.793870523787408,-1.,3.77444863801212));
#51070=CARTESIAN_POINT('Ctrl Pts',(-0.793961083688992,-1.,3.76692626931111));
#51071=CARTESIAN_POINT('Ctrl Pts',(-0.794008429134907,-1.,3.75951468666257));
#51072=CARTESIAN_POINT('Ctrl Pts',(-0.794017347371377,-1.,3.75224692493864));
#51073=CARTESIAN_POINT('Ctrl Pts',(-0.793982700459952,-1.,3.74511357728861));
#51074=CARTESIAN_POINT('Ctrl Pts',(-0.793882700937017,-1.,3.73803280541687));
#51075=CARTESIAN_POINT('Ctrl Pts',(-0.793682750269684,-1.,3.73086914695805));
#51076=CARTESIAN_POINT('Ctrl Pts',(-0.793347023784205,-1.,3.72348797293734));
#51077=CARTESIAN_POINT('Ctrl Pts',(-0.792848377370287,-1.,3.71580242396124));
#51078=CARTESIAN_POINT('Ctrl Pts',(-0.792177688845818,-1.,3.70781724021806));
#51079=CARTESIAN_POINT('Ctrl Pts',(-0.79135657569598,-1.,3.69968940808721));
#51080=CARTESIAN_POINT('Ctrl Pts',(-0.790436284988788,-1.,3.69172044327364));
#51081=CARTESIAN_POINT('Ctrl Pts',(-0.789483546064387,-1.,3.68428439783905));
#51082=CARTESIAN_POINT('Ctrl Pts',(-0.788569566220285,-1.,3.67777119516252));
#51083=CARTESIAN_POINT('Ctrl Pts',(-0.787758799995743,-1.,3.67252923663655));
#51084=CARTESIAN_POINT('Ctrl Pts',(-0.787145041181546,-1.,3.66907505398677));
#51085=CARTESIAN_POINT('Ctrl Pts',(-0.786774337198062,-1.,3.66743103898702));
#51086=CARTESIAN_POINT('Ctrl Pts',(-0.786565919558984,-1.,3.66680946938292));
#51087=CARTESIAN_POINT('Ctrl Pts',(-0.786459983895432,-1.,3.6666431041522));
#51088=CARTESIAN_POINT('Ctrl Pts',(-0.786422660831985,-1.,3.66661143271685));
#51089=CARTESIAN_POINT('',(-0.963899035117249,-1.,3.62400312501245));
#51090=CARTESIAN_POINT('Origin',(0.,-1.,0.));
#51091=CARTESIAN_POINT('',(-1.22531898815164,-1.,4.01728681790024));
#51092=CARTESIAN_POINT('Ctrl Pts',(-0.963899035117249,-1.,3.62400312501245));
#51093=CARTESIAN_POINT('Ctrl Pts',(-0.963880158555582,-1.,3.6240482887845));
#51094=CARTESIAN_POINT('Ctrl Pts',(-0.963861297423241,-1.,3.62424461507588));
#51095=CARTESIAN_POINT('Ctrl Pts',(-0.963957782642843,-1.,3.62489305727662));
#51096=CARTESIAN_POINT('Ctrl Pts',(-0.964373850166458,-1.,3.62652618145335));
#51097=CARTESIAN_POINT('Ctrl Pts',(-0.965395153165293,-1.,3.62988252139846));
#51098=CARTESIAN_POINT('Ctrl Pts',(-0.967052554541386,-1.,3.63492122081143));
#51099=CARTESIAN_POINT('Ctrl Pts',(-0.969195124675866,-1.,3.64113946505766));
#51100=CARTESIAN_POINT('Ctrl Pts',(-0.971722122061341,-1.,3.64819756447455));
#51101=CARTESIAN_POINT('Ctrl Pts',(-0.974519971354848,-1.,3.65571576735126));
#51102=CARTESIAN_POINT('Ctrl Pts',(-0.977478312751618,-1.,3.66333049637475));
#51103=CARTESIAN_POINT('Ctrl Pts',(-0.980505922458267,-1.,3.67074983340361));
#51104=CARTESIAN_POINT('Ctrl Pts',(-0.983550791470419,-1.,3.67782408841715));
#51105=CARTESIAN_POINT('Ctrl Pts',(-0.986602639863838,-1.,3.68455317926068));
#51106=CARTESIAN_POINT('Ctrl Pts',(-0.989676715398558,-1.,3.69102682138846));
#51107=CARTESIAN_POINT('Ctrl Pts',(-0.99280221833201,-1.,3.69738123415662));
#51108=CARTESIAN_POINT('Ctrl Pts',(-0.996009819772518,-1.,3.70375282282138));
#51109=CARTESIAN_POINT('Ctrl Pts',(-0.999317260756531,-1.,3.71022439713938));
#51110=CARTESIAN_POINT('Ctrl Pts',(-1.00272423396822,-1.,3.71680667125118));
#51111=CARTESIAN_POINT('Ctrl Pts',(-1.0062200073571,-1.,3.72346803750595));
#51112=CARTESIAN_POINT('Ctrl Pts',(-1.00978798539496,-1.,3.73015276704426));
#51113=CARTESIAN_POINT('Ctrl Pts',(-1.01341114319903,-1.,3.73680245055734));
#51114=CARTESIAN_POINT('Ctrl Pts',(-1.01707794311079,-1.,3.74337942504959));
#51115=CARTESIAN_POINT('Ctrl Pts',(-1.02078510487428,-1.,3.74987777155834));
#51116=CARTESIAN_POINT('Ctrl Pts',(-1.0245342944466,-1.,3.75631037456194));
#51117=CARTESIAN_POINT('Ctrl Pts',(-1.02833014458181,-1.,3.76270122291232));
#51118=CARTESIAN_POINT('Ctrl Pts',(-1.0321778660492,-1.,3.76907609832522));
#51119=CARTESIAN_POINT('Ctrl Pts',(-1.03608074678013,-1.,3.77545283140445));
#51120=CARTESIAN_POINT('Ctrl Pts',(-1.04003862055804,-1.,3.78183535008192));
#51121=CARTESIAN_POINT('Ctrl Pts',(-1.04404924374426,-1.,3.78821910787195));
#51122=CARTESIAN_POINT('Ctrl Pts',(-1.04810913267641,-1.,3.79459440308793));
#51123=CARTESIAN_POINT('Ctrl Pts',(-1.05221457990015,-1.,3.80095039790678));
#51124=CARTESIAN_POINT('Ctrl Pts',(-1.05636266918643,-1.,3.80727913637784));
#51125=CARTESIAN_POINT('Ctrl Pts',(-1.06055206187298,-1.,3.81357866117485));
#51126=CARTESIAN_POINT('Ctrl Pts',(-1.06478244038931,-1.,3.81985083953012));
#51127=CARTESIAN_POINT('Ctrl Pts',(-1.0690541318036,-1.,3.82609989967278));
#51128=CARTESIAN_POINT('Ctrl Pts',(-1.0733676663346,-1.,3.83233071195145));
#51129=CARTESIAN_POINT('Ctrl Pts',(-1.07772335353856,-1.,3.83854714117486));
#51130=CARTESIAN_POINT('Ctrl Pts',(-1.08212087917986,-1.,3.84475048030615));
#51131=CARTESIAN_POINT('Ctrl Pts',(-1.08655950846377,-1.,3.8509402522269));
#51132=CARTESIAN_POINT('Ctrl Pts',(-1.09103825516288,-1.,3.85711487933911));
#51133=CARTESIAN_POINT('Ctrl Pts',(-1.09555606505012,-1.,3.86327241021242));
#51134=CARTESIAN_POINT('Ctrl Pts',(-1.10011198761202,-1.,3.86941120134872));
#51135=CARTESIAN_POINT('Ctrl Pts',(-1.10470536603303,-1.,3.87553067187566));
#51136=CARTESIAN_POINT('Ctrl Pts',(-1.10933577224029,-1.,3.88163105531791));
#51137=CARTESIAN_POINT('Ctrl Pts',(-1.11400292434447,-1.,3.88771308285229));
#51138=CARTESIAN_POINT('Ctrl Pts',(-1.11870660794609,-1.,3.89377768340362));
#51139=CARTESIAN_POINT('Ctrl Pts',(-1.12344660099029,-1.,3.89982569749978));
#51140=CARTESIAN_POINT('Ctrl Pts',(-1.12822258281518,-1.,3.90585753318622));
#51141=CARTESIAN_POINT('Ctrl Pts',(-1.13303414693849,-1.,3.91187321145495));
#51142=CARTESIAN_POINT('Ctrl Pts',(-1.13788084225511,-1.,3.91787251936688));
#51143=CARTESIAN_POINT('Ctrl Pts',(-1.14276220561575,-1.,3.92385513133937));
#51144=CARTESIAN_POINT('Ctrl Pts',(-1.14767779451147,-1.,3.92982073294334));
#51145=CARTESIAN_POINT('Ctrl Pts',(-1.15262722716391,-1.,3.9357691705651));
#51146=CARTESIAN_POINT('Ctrl Pts',(-1.1576101834106,-1.,3.94170046685542));
#51147=CARTESIAN_POINT('Ctrl Pts',(-1.16262637999261,-1.,3.9476147478092));
#51148=CARTESIAN_POINT('Ctrl Pts',(-1.16767555244495,-1.,3.95351219510062));
#51149=CARTESIAN_POINT('Ctrl Pts',(-1.17275743590327,-1.,3.95939299213164));
#51150=CARTESIAN_POINT('Ctrl Pts',(-1.17787174135445,-1.,3.96525726357682));
#51151=CARTESIAN_POINT('Ctrl Pts',(-1.18301815039596,-1.,3.9711050516465));
#51152=CARTESIAN_POINT('Ctrl Pts',(-1.18819633715285,-1.,3.97693634766926));
#51153=CARTESIAN_POINT('Ctrl Pts',(-1.19340598349307,-1.,3.98275111052015));
#51154=CARTESIAN_POINT('Ctrl Pts',(-1.19864679609596,-1.,3.98854928957287));
#51155=CARTESIAN_POINT('Ctrl Pts',(-1.2039185237544,-1.,3.99433084800649));
#51156=CARTESIAN_POINT('Ctrl Pts',(-1.20922097030107,-1.,4.00009577952534));
#51157=CARTESIAN_POINT('Ctrl Pts',(-1.21455398918813,-1.,4.00584409524937));
#51158=CARTESIAN_POINT('Ctrl Pts',(-1.21884478244983,-1.,4.01042947142681));
#51159=CARTESIAN_POINT('Ctrl Pts',(-1.22207656456199,-1.,4.01386104434674));
#51160=CARTESIAN_POINT('Ctrl Pts',(-1.22423716681447,-1.,4.0161454457032));
#51161=CARTESIAN_POINT('Ctrl Pts',(-1.22531898815164,-1.,4.01728681790024));
#51162=CARTESIAN_POINT('',(-1.36999806084572,-1.,3.97027773754922));
#51163=CARTESIAN_POINT('',(-1.22531898815164,-1.,4.01728681790024));
#51164=CARTESIAN_POINT('',(-1.35032489087101,-1.,3.4984457533445));
#51165=CARTESIAN_POINT('Ctrl Pts',(-1.36999806084572,-1.,3.97027773754922));
#51166=CARTESIAN_POINT('Ctrl Pts',(-1.37020239094614,-1.,3.9687184694131));
#51167=CARTESIAN_POINT('Ctrl Pts',(-1.37060761745635,-1.,3.96560037974645));
#51168=CARTESIAN_POINT('Ctrl Pts',(-1.3712051561502,-1.,3.96092458506535));
#51169=CARTESIAN_POINT('Ctrl Pts',(-1.37198126432386,-1.,3.95469287280914));
#51170=CARTESIAN_POINT('Ctrl Pts',(-1.37291699202807,-1.,3.94690771785133));
#51171=CARTESIAN_POINT('Ctrl Pts',(-1.37381821967165,-1.,3.93912709040818));
#51172=CARTESIAN_POINT('Ctrl Pts',(-1.37468482215751,-1.,3.93135106761844));
#51173=CARTESIAN_POINT('Ctrl Pts',(-1.37551664448242,-1.,3.92357976987672));
#51174=CARTESIAN_POINT('Ctrl Pts',(-1.37631350505797,-1.,3.91581337462644));
#51175=CARTESIAN_POINT('Ctrl Pts',(-1.3770751963402,-1.,3.90805209523486));
#51176=CARTESIAN_POINT('Ctrl Pts',(-1.37780148512792,-1.,3.90029615196727));
#51177=CARTESIAN_POINT('Ctrl Pts',(-1.3784921128802,-1.,3.89254574338496));
#51178=CARTESIAN_POINT('Ctrl Pts',(-1.37914679719383,-1.,3.88480102249277));
#51179=CARTESIAN_POINT('Ctrl Pts',(-1.37976523097073,-1.,3.87706205830532));
#51180=CARTESIAN_POINT('Ctrl Pts',(-1.38034709213014,-1.,3.86932885813068));
#51181=CARTESIAN_POINT('Ctrl Pts',(-1.38089205992989,-1.,3.86160143043959));
#51182=CARTESIAN_POINT('Ctrl Pts',(-1.38139983115049,-1.,3.85387983979481));
#51183=CARTESIAN_POINT('Ctrl Pts',(-1.38187013346109,-1.,3.84616425605764));
#51184=CARTESIAN_POINT('Ctrl Pts',(-1.38230274828822,-1.,3.83845502790746));
#51185=CARTESIAN_POINT('Ctrl Pts',(-1.38269750245138,-1.,3.8307526698229));
#51186=CARTESIAN_POINT('Ctrl Pts',(-1.38305421262763,-1.,3.82305771743829));
#51187=CARTESIAN_POINT('Ctrl Pts',(-1.38337263902782,-1.,3.81537060817811));
#51188=CARTESIAN_POINT('Ctrl Pts',(-1.3836524404622,-1.,3.80769156398411));
#51189=CARTESIAN_POINT('Ctrl Pts',(-1.38389311766682,-1.,3.80002044322111));
#51190=CARTESIAN_POINT('Ctrl Pts',(-1.38409399694566,-1.,3.79235669640841));
#51191=CARTESIAN_POINT('Ctrl Pts',(-1.38425435883756,-1.,3.78469969805082));
#51192=CARTESIAN_POINT('Ctrl Pts',(-1.38437354551428,-1.,3.77704902230418));
#51193=CARTESIAN_POINT('Ctrl Pts',(-1.38445107339518,-1.,3.76940473185779));
#51194=CARTESIAN_POINT('Ctrl Pts',(-1.3844867525335,-1.,3.76176768271367));
#51195=CARTESIAN_POINT('Ctrl Pts',(-1.38448077997163,-1.,3.7541397631875));
#51196=CARTESIAN_POINT('Ctrl Pts',(-1.38443344984394,-1.,3.74652317167876));
#51197=CARTESIAN_POINT('Ctrl Pts',(-1.38434489156458,-1.,3.73891976418104));
#51198=CARTESIAN_POINT('Ctrl Pts',(-1.38421479111531,-1.,3.73133035859282));
#51199=CARTESIAN_POINT('Ctrl Pts',(-1.3840421342895,-1.,3.72375409358803));
#51200=CARTESIAN_POINT('Ctrl Pts',(-1.38382489984586,-1.,3.7161876605181));
#51201=CARTESIAN_POINT('Ctrl Pts',(-1.38356065402124,-1.,3.70862680753347));
#51202=CARTESIAN_POINT('Ctrl Pts',(-1.38324717612865,-1.,3.701067921679));
#51203=CARTESIAN_POINT('Ctrl Pts',(-1.38288311171651,-1.,3.69350967899526));
#51204=CARTESIAN_POINT('Ctrl Pts',(-1.38246852827182,-1.,3.68595444983837));
#51205=CARTESIAN_POINT('Ctrl Pts',(-1.3820057429062,-1.,3.67841038482414));
#51206=CARTESIAN_POINT('Ctrl Pts',(-1.38149812653868,-1.,3.67088843112262));
#51207=CARTESIAN_POINT('Ctrl Pts',(-1.38094856333552,-1.,3.66339848520857));
#51208=CARTESIAN_POINT('Ctrl Pts',(-1.38035791051213,-1.,3.6559455440439));
#51209=CARTESIAN_POINT('Ctrl Pts',(-1.37972372481603,-1.,3.64852652756456));
#51210=CARTESIAN_POINT('Ctrl Pts',(-1.37903818567359,-1.,3.64112507791141));
#51211=CARTESIAN_POINT('Ctrl Pts',(-1.37829035457339,-1.,3.63371727442486));
#51212=CARTESIAN_POINT('Ctrl Pts',(-1.37746987919881,-1.,3.62628098665145));
#51213=CARTESIAN_POINT('Ctrl Pts',(-1.37657053403107,-1.,3.6188048116042));
#51214=CARTESIAN_POINT('Ctrl Pts',(-1.37559314436634,-1.,3.61129546591064));
#51215=CARTESIAN_POINT('Ctrl Pts',(-1.37455051379623,-1.,3.60379020123988));
#51216=CARTESIAN_POINT('Ctrl Pts',(-1.37346320103157,-1.,3.59634627869048));
#51217=CARTESIAN_POINT('Ctrl Pts',(-1.37235053660976,-1.,3.58901853846365));
#51218=CARTESIAN_POINT('Ctrl Pts',(-1.37122241663062,-1.,3.58183885982715));
#51219=CARTESIAN_POINT('Ctrl Pts',(-1.37007229485659,-1.,3.57479875549486));
#51220=CARTESIAN_POINT('Ctrl Pts',(-1.36886584973389,-1.,3.5678208030466));
#51221=CARTESIAN_POINT('Ctrl Pts',(-1.36754771771233,-1.,3.56077662028649));
#51222=CARTESIAN_POINT('Ctrl Pts',(-1.3660614545677,-1.,3.55353883995949));
#51223=CARTESIAN_POINT('Ctrl Pts',(-1.36436666257598,-1.,3.54602591832973));
#51224=CARTESIAN_POINT('Ctrl Pts',(-1.36245507339307,-1.,3.53824396424961));
#51225=CARTESIAN_POINT('Ctrl Pts',(-1.36037259643734,-1.,3.530344649616));
#51226=CARTESIAN_POINT('Ctrl Pts',(-1.35821701528836,-1.,3.52261776116748));
#51227=CARTESIAN_POINT('Ctrl Pts',(-1.35611275237152,-1.,3.51542230699556));
#51228=CARTESIAN_POINT('Ctrl Pts',(-1.35419113575956,-1.,3.50913227059999));
#51229=CARTESIAN_POINT('Ctrl Pts',(-1.35257032843486,-1.,3.50408168106261));
#51230=CARTESIAN_POINT('Ctrl Pts',(-1.35142377279517,-1.,3.5007660381649));
#51231=CARTESIAN_POINT('Ctrl Pts',(-1.35080045218587,-1.,3.49920025459723));
#51232=CARTESIAN_POINT('Ctrl Pts',(-1.35049736560527,-1.,3.49861894124827));
#51233=CARTESIAN_POINT('Ctrl Pts',(-1.35036670892966,-1.,3.49847119623846));
#51234=CARTESIAN_POINT('Ctrl Pts',(-1.35032489087101,-1.,3.4984457533445));
#51235=CARTESIAN_POINT('',(-1.51895082866166,-1.,3.42859860294378));
#51236=CARTESIAN_POINT('Origin',(0.,-1.,0.));
#51237=CARTESIAN_POINT('',(-1.83867539237861,-1.,3.77614523045147));
#51238=CARTESIAN_POINT('Ctrl Pts',(-1.51895082866166,-1.,3.42859860294378));
#51239=CARTESIAN_POINT('Ctrl Pts',(-1.51893924967231,-1.,3.42864616361967));
#51240=CARTESIAN_POINT('Ctrl Pts',(-1.51895133295017,-1.,3.42884302333978));
#51241=CARTESIAN_POINT('Ctrl Pts',(-1.51914806898539,-1.,3.42946838852728));
#51242=CARTESIAN_POINT('Ctrl Pts',(-1.5198144909343,-1.,3.4310163189349));
#51243=CARTESIAN_POINT('Ctrl Pts',(-1.52134826724227,-1.,3.43417156977749));
#51244=CARTESIAN_POINT('Ctrl Pts',(-1.52377348950429,-1.,3.43888895974182));
#51245=CARTESIAN_POINT('Ctrl Pts',(-1.52686242875717,-1.,3.44469547527));
#51246=CARTESIAN_POINT('Ctrl Pts',(-1.530462444618,-1.,3.45127136828667));
#51247=CARTESIAN_POINT('Ctrl Pts',(-1.53440195378902,-1.,3.45825932955273));
#51248=CARTESIAN_POINT('Ctrl Pts',(-1.53851507915533,-1.,3.46531752207222));
#51249=CARTESIAN_POINT('Ctrl Pts',(-1.54266605398152,-1.,3.47217189224576));
#51250=CARTESIAN_POINT('Ctrl Pts',(-1.54678009290207,-1.,3.47868272898599));
#51251=CARTESIAN_POINT('Ctrl Pts',(-1.55084702970382,-1.,3.48485155928414));
#51252=CARTESIAN_POINT('Ctrl Pts',(-1.5548959590107,-1.,3.49076460877317));
#51253=CARTESIAN_POINT('Ctrl Pts',(-1.55897703097859,-1.,3.49655185179623));
#51254=CARTESIAN_POINT('Ctrl Pts',(-1.56314187758689,-1.,3.50234321621607));
#51255=CARTESIAN_POINT('Ctrl Pts',(-1.56742097575041,-1.,3.50821771695427));
#51256=CARTESIAN_POINT('Ctrl Pts',(-1.57181569799774,-1.,3.51418598431733));
#51257=CARTESIAN_POINT('Ctrl Pts',(-1.5763104998818,-1.,3.52021847865961));
#51258=CARTESIAN_POINT('Ctrl Pts',(-1.58088027227856,-1.,3.52626275334899));
#51259=CARTESIAN_POINT('Ctrl Pts',(-1.58549906268083,-1.,3.53226378147068));
#51260=CARTESIAN_POINT('Ctrl Pts',(-1.59014958368725,-1.,3.53818616861045));
#51261=CARTESIAN_POINT('Ctrl Pts',(-1.5948276694975,-1.,3.544024581823));
#51262=CARTESIAN_POINT('Ctrl Pts',(-1.59953698113444,-1.,3.54979148634426));
#51263=CARTESIAN_POINT('Ctrl Pts',(-1.60428584699848,-1.,3.55550985096117));
#51264=CARTESIAN_POINT('Ctrl Pts',(-1.60908344685459,-1.,3.56120432482986));
#51265=CARTESIAN_POINT('Ctrl Pts',(-1.61393581747522,-1.,3.56689200468404));
#51266=CARTESIAN_POINT('Ctrl Pts',(-1.61884340915412,-1.,3.57257679609826));
#51267=CARTESIAN_POINT('Ctrl Pts',(-1.62380329464851,-1.,3.57825455954405));
#51268=CARTESIAN_POINT('Ctrl Pts',(-1.62881051550748,-1.,3.5839162577435));
#51269=CARTESIAN_POINT('Ctrl Pts',(-1.63385971451259,-1.,3.58955176627876));
#51270=CARTESIAN_POINT('Ctrl Pts',(-1.63894676675349,-1.,3.59515368334887));
#51271=CARTESIAN_POINT('Ctrl Pts',(-1.6440700438558,-1.,3.6007202851384));
#51272=CARTESIAN_POINT('Ctrl Pts',(-1.64922952425833,-1.,3.60625346556992));
#51273=CARTESIAN_POINT('Ctrl Pts',(-1.65442619244327,-1.,3.61175734965129));
#51274=CARTESIAN_POINT('Ctrl Pts',(-1.65966133399186,-1.,3.61723666482457));
#51275=CARTESIAN_POINT('Ctrl Pts',(-1.66493585923853,-1.,3.62269517989104));
#51276=CARTESIAN_POINT('Ctrl Pts',(-1.67024966008037,-1.,3.62813422105257));
#51277=CARTESIAN_POINT('Ctrl Pts',(-1.67560193613145,-1.,3.63355343201211));
#51278=CARTESIAN_POINT('Ctrl Pts',(-1.68099146651577,-1.,3.63895140887443));
#51279=CARTESIAN_POINT('Ctrl Pts',(-1.68641690471455,-1.,3.64432638915199));
#51280=CARTESIAN_POINT('Ctrl Pts',(-1.691877054817,-1.,3.64967689827393));
#51281=CARTESIAN_POINT('Ctrl Pts',(-1.69737117722559,-1.,3.65500246526798));
#51282=CARTESIAN_POINT('Ctrl Pts',(-1.70289888566904,-1.,3.6603033877491));
#51283=CARTESIAN_POINT('Ctrl Pts',(-1.70846001610983,-1.,3.6655804319893));
#51284=CARTESIAN_POINT('Ctrl Pts',(-1.71405450210392,-1.,3.67083454901629));
#51285=CARTESIAN_POINT('Ctrl Pts',(-1.71968225581787,-1.,3.67606660374665));
#51286=CARTESIAN_POINT('Ctrl Pts',(-1.72534302437003,-1.,3.68127704936472));
#51287=CARTESIAN_POINT('Ctrl Pts',(-1.73103640956647,-1.,3.68646597019188));
#51288=CARTESIAN_POINT('Ctrl Pts',(-1.73676193254493,-1.,3.69163322647906));
#51289=CARTESIAN_POINT('Ctrl Pts',(-1.74251908492589,-1.,3.6967785691046));
#51290=CARTESIAN_POINT('Ctrl Pts',(-1.74830738046092,-1.,3.70190175673422));
#51291=CARTESIAN_POINT('Ctrl Pts',(-1.75412641804148,-1.,3.70700269736876));
#51292=CARTESIAN_POINT('Ctrl Pts',(-1.75997588499021,-1.,3.71208146346454));
#51293=CARTESIAN_POINT('Ctrl Pts',(-1.76585552124549,-1.,3.71713822377675));
#51294=CARTESIAN_POINT('Ctrl Pts',(-1.77176509401846,-1.,3.72217319911429));
#51295=CARTESIAN_POINT('Ctrl Pts',(-1.77770437039606,-1.,3.72718661205504));
#51296=CARTESIAN_POINT('Ctrl Pts',(-1.78367308442682,-1.,3.73217863095022));
#51297=CARTESIAN_POINT('Ctrl Pts',(-1.78967092823139,-1.,3.73714934729962));
#51298=CARTESIAN_POINT('Ctrl Pts',(-1.79569757859041,-1.,3.74209880351667));
#51299=CARTESIAN_POINT('Ctrl Pts',(-1.80175271485519,-1.,3.74702700874954));
#51300=CARTESIAN_POINT('Ctrl Pts',(-1.80783603939662,-1.,3.75193395888069));
#51301=CARTESIAN_POINT('Ctrl Pts',(-1.81394729834032,-1.,3.75681965683995));
#51302=CARTESIAN_POINT('Ctrl Pts',(-1.82008629694924,-1.,3.76168412709652));
#51303=CARTESIAN_POINT('Ctrl Pts',(-1.82625289221933,-1.,3.76652740355856));
#51304=CARTESIAN_POINT('Ctrl Pts',(-1.83120816956515,-1.,3.77038509819777));
#51305=CARTESIAN_POINT('Ctrl Pts',(-1.83493697935064,-1.,3.77326886065484));
#51306=CARTESIAN_POINT('Ctrl Pts',(-1.83742834010821,-1.,3.77518714458232));
#51307=CARTESIAN_POINT('Ctrl Pts',(-1.83867539237861,-1.,3.77614523045147));
#51308=CARTESIAN_POINT('',(-1.97421938526992,-1.,3.70708211654725));
#51309=CARTESIAN_POINT('',(-1.83867539237861,-1.,3.77614523045147));
#51310=CARTESIAN_POINT('',(-1.88097764062542,-1.,3.24413672884902));
#51311=CARTESIAN_POINT('Ctrl Pts',(-1.97421938526992,-1.,3.70708211654725));
#51312=CARTESIAN_POINT('Ctrl Pts',(-1.974177276451,-1.,3.7055100813194));
#51313=CARTESIAN_POINT('Ctrl Pts',(-1.97408973726149,-1.,3.70236698911837));
#51314=CARTESIAN_POINT('Ctrl Pts',(-1.97394846382289,-1.,3.69765528558292));
#51315=CARTESIAN_POINT('Ctrl Pts',(-1.97374016224397,-1.,3.69137888597855));
#51316=CARTESIAN_POINT('Ctrl Pts',(-1.97344650303631,-1.,3.68354319913416));
#51317=CARTESIAN_POINT('Ctrl Pts',(-1.97311947678035,-1.,3.67571738106175));
#51318=CARTESIAN_POINT('Ctrl Pts',(-1.9727589719863,-1.,3.66790152751984));
#51319=CARTESIAN_POINT('Ctrl Pts',(-1.97236485439317,-1.,3.66009578166865));
#51320=CARTESIAN_POINT('Ctrl Pts',(-1.97193697240645,-1.,3.65230034717364));
#51321=CARTESIAN_POINT('Ctrl Pts',(-1.97147515441539,-1.,3.64451546724221));
#51322=CARTESIAN_POINT('Ctrl Pts',(-1.97097920454698,-1.,3.63674139590853));
#51323=CARTESIAN_POINT('Ctrl Pts',(-1.97044889850518,-1.,3.62897836973397));
#51324=CARTESIAN_POINT('Ctrl Pts',(-1.96988398129888,-1.,3.62122658401722));
#51325=CARTESIAN_POINT('Ctrl Pts',(-1.96928416040712,-1.,3.61348615496393));
#51326=CARTESIAN_POINT('Ctrl Pts',(-1.96864911885775,-1.,3.60575714017676));
#51327=CARTESIAN_POINT('Ctrl Pts',(-1.96797854118257,-1.,3.59803959819725));
#51328=CARTESIAN_POINT('Ctrl Pts',(-1.96727213799507,-1.,3.5903336402273));
#51329=CARTESIAN_POINT('Ctrl Pts',(-1.9665296668894,-1.,3.58263947663884));
#51330=CARTESIAN_POINT('Ctrl Pts',(-1.96575096652857,-1.,3.57495748601088));
#51331=CARTESIAN_POINT('Ctrl Pts',(-1.96493594634643,-1.,3.56728820357933));
#51332=CARTESIAN_POINT('Ctrl Pts',(-1.96408450906868,-1.,3.55963218706201));
#51333=CARTESIAN_POINT('Ctrl Pts',(-1.96319648628667,-1.,3.55198990600929));
#51334=CARTESIAN_POINT('Ctrl Pts',(-1.96227157573058,-1.,3.54436163300425));
#51335=CARTESIAN_POINT('Ctrl Pts',(-1.96130926212661,-1.,3.53674730625759));
#51336=CARTESIAN_POINT('Ctrl Pts',(-1.96030879411534,-1.,3.52914648844289));
#51337=CARTESIAN_POINT('Ctrl Pts',(-1.95926936324436,-1.,3.52155867431438));
#51338=CARTESIAN_POINT('Ctrl Pts',(-1.95819025316768,-1.,3.51398354617772));
#51339=CARTESIAN_POINT('Ctrl Pts',(-1.95707099606514,-1.,3.50642124159913));
#51340=CARTESIAN_POINT('Ctrl Pts',(-1.9559115382367,-1.,3.49887263575602));
#51341=CARTESIAN_POINT('Ctrl Pts',(-1.95471236969653,-1.,3.49133956289154));
#51342=CARTESIAN_POINT('Ctrl Pts',(-1.95347412486316,-1.,3.48382414832648));
#51343=CARTESIAN_POINT('Ctrl Pts',(-1.95219722189878,-1.,3.47632820495926));
#51344=CARTESIAN_POINT('Ctrl Pts',(-1.95088147859876,-1.,3.4688525897419));
#51345=CARTESIAN_POINT('Ctrl Pts',(-1.94952575850196,-1.,3.46139661060959));
#51346=CARTESIAN_POINT('Ctrl Pts',(-1.94812754766524,-1.,3.45395731584051));
#51347=CARTESIAN_POINT('Ctrl Pts',(-1.94668377715332,-1.,3.44653088665685));
#51348=CARTESIAN_POINT('Ctrl Pts',(-1.94519168842883,-1.,3.43911410197693));
#51349=CARTESIAN_POINT('Ctrl Pts',(-1.94364973660285,-1.,3.43170586602436));
#51350=CARTESIAN_POINT('Ctrl Pts',(-1.94205835913692,-1.,3.42430850941497));
#51351=CARTESIAN_POINT('Ctrl Pts',(-1.94042111965237,-1.,3.41692971994082));
#51352=CARTESIAN_POINT('Ctrl Pts',(-1.93874306008132,-1.,3.40957978266622));
#51353=CARTESIAN_POINT('Ctrl Pts',(-1.93702857723089,-1.,3.40226802104093));
#51354=CARTESIAN_POINT('Ctrl Pts',(-1.93527929945982,-1.,3.39499923640789));
#51355=CARTESIAN_POINT('Ctrl Pts',(-1.93349233176794,-1.,3.38777076883267));
#51356=CARTESIAN_POINT('Ctrl Pts',(-1.93165739093292,-1.,3.38056768525577));
#51357=CARTESIAN_POINT('Ctrl Pts',(-1.92975993109897,-1.,3.37336807068078));
#51358=CARTESIAN_POINT('Ctrl Pts',(-1.92778626543803,-1.,3.36615168657597));
#51359=CARTESIAN_POINT('Ctrl Pts',(-1.92572846125763,-1.,3.35890824422976));
#51360=CARTESIAN_POINT('Ctrl Pts',(-1.92358838440518,-1.,3.35164424847206));
#51361=CARTESIAN_POINT('Ctrl Pts',(-1.92138450828378,-1.,3.34439448941915));
#51362=CARTESIAN_POINT('Ctrl Pts',(-1.91914609610173,-1.,3.33721230709948));
#51363=CARTESIAN_POINT('Ctrl Pts',(-1.91690081930297,-1.,3.33014884257812));
#51364=CARTESIAN_POINT('Ctrl Pts',(-1.91466343916612,-1.,3.32323403454507));
#51365=CARTESIAN_POINT('Ctrl Pts',(-1.91242616234459,-1.,3.31646052426395));
#51366=CARTESIAN_POINT('Ctrl Pts',(-1.91014297830502,-1.,3.30975721158694));
#51367=CARTESIAN_POINT('Ctrl Pts',(-1.90773912171424,-1.,3.30300595568341));
#51368=CARTESIAN_POINT('Ctrl Pts',(-1.9051389186417,-1.,3.29608978722258));
#51369=CARTESIAN_POINT('Ctrl Pts',(-1.9022897124757,-1.,3.28893448600364));
#51370=CARTESIAN_POINT('Ctrl Pts',(-1.89918429230425,-1.,3.28154737912287));
#51371=CARTESIAN_POINT('Ctrl Pts',(-1.89589172903662,-1.,3.27407108932908));
#51372=CARTESIAN_POINT('Ctrl Pts',(-1.89255393500769,-1.,3.2667765388833));
#51373=CARTESIAN_POINT('Ctrl Pts',(-1.88934996203508,-1.,3.2599988519361));
#51374=CARTESIAN_POINT('Ctrl Pts',(-1.88646802523372,-1.,3.25408686339298));
#51375=CARTESIAN_POINT('Ctrl Pts',(-1.88407708646435,-1.,3.24935200512055));
#51376=CARTESIAN_POINT('Ctrl Pts',(-1.88242596600422,-1.,3.24625654410705));
#51377=CARTESIAN_POINT('Ctrl Pts',(-1.88156537699118,-1.,3.24480754675942));
#51378=CARTESIAN_POINT('Ctrl Pts',(-1.88117508446657,-1.,3.24428080352952));
#51379=CARTESIAN_POINT('Ctrl Pts',(-1.88102292397987,-1.,3.2441553167131));
#51380=CARTESIAN_POINT('Ctrl Pts',(-1.88097764062542,-1.,3.24413672884902));
#51381=CARTESIAN_POINT('',(-2.03660101169564,-1.,3.14877060440425));
#51382=CARTESIAN_POINT('Origin',(0.,-1.,0.));
#51383=CARTESIAN_POINT('',(-2.40675750623143,-1.,3.44202241512147));
#51384=CARTESIAN_POINT('Ctrl Pts',(-2.03660101169564,-1.,3.14877060440425));
#51385=CARTESIAN_POINT('Ctrl Pts',(-2.03659701539175,-1.,3.1488193908823));
#51386=CARTESIAN_POINT('Ctrl Pts',(-2.03663974554941,-1.,3.14901193669147));
#51387=CARTESIAN_POINT('Ctrl Pts',(-2.03693188810614,-1.,3.14959882629936));
#51388=CARTESIAN_POINT('Ctrl Pts',(-2.03783225496023,-1.,3.15102344775396));
#51389=CARTESIAN_POINT('Ctrl Pts',(-2.03984073791432,-1.,3.1538999167466));
#51390=CARTESIAN_POINT('Ctrl Pts',(-2.04297406404132,-1.,3.15817983946525));
#51391=CARTESIAN_POINT('Ctrl Pts',(-2.0469333124766,-1.,3.16343165059235));
#51392=CARTESIAN_POINT('Ctrl Pts',(-2.05151770247452,-1.,3.16936341689859));
#51393=CARTESIAN_POINT('Ctrl Pts',(-2.05650186773279,-1.,3.17564906975592));
#51394=CARTESIAN_POINT('Ctrl Pts',(-2.06166849827143,-1.,3.18197692964677));
#51395=CARTESIAN_POINT('Ctrl Pts',(-2.06684062744065,-1.,3.18809755562297));
#51396=CARTESIAN_POINT('Ctrl Pts',(-2.07192253497765,-1.,3.19388465568113));
#51397=CARTESIAN_POINT('Ctrl Pts',(-2.0769044187063,-1.,3.19934132835879));
#51398=CARTESIAN_POINT('Ctrl Pts',(-2.08182850370816,-1.,3.20454818630635));
#51399=CARTESIAN_POINT('Ctrl Pts',(-2.08676465517435,-1.,3.20962575845433));
#51400=CARTESIAN_POINT('Ctrl Pts',(-2.0917841946046,-1.,3.2146942960168));
#51401=CARTESIAN_POINT('Ctrl Pts',(-2.09692958434933,-1.,3.21982707347067));
#51402=CARTESIAN_POINT('Ctrl Pts',(-2.10220384298533,-1.,3.22503437553496));
#51403=CARTESIAN_POINT('Ctrl Pts',(-2.1075869964248,-1.,3.23028945793334));
#51404=CARTESIAN_POINT('Ctrl Pts',(-2.11304604021784,-1.,3.23554444767115));
#51405=CARTESIAN_POINT('Ctrl Pts',(-2.11854673326972,-1.,3.24074905517282));
#51406=CARTESIAN_POINT('Ctrl Pts',(-2.12406646410943,-1.,3.24587102613347));
#51407=CARTESIAN_POINT('Ctrl Pts',(-2.1296002839681,-1.,3.25090574493994));
#51408=CARTESIAN_POINT('Ctrl Pts',(-2.13515375878786,-1.,3.25586495065027));
#51409=CARTESIAN_POINT('Ctrl Pts',(-2.14073870754257,-1.,3.26077002641868));
#51410=CARTESIAN_POINT('Ctrl Pts',(-2.14636805295663,-1.,3.26564388189764));
#51411=CARTESIAN_POINT('Ctrl Pts',(-2.15205043199818,-1.,3.27050245897244));
#51412=CARTESIAN_POINT('Ctrl Pts',(-2.15778690038359,-1.,3.27534954469206));
#51413=CARTESIAN_POINT('Ctrl Pts',(-2.16357391934434,-1.,3.28018150841414));
#51414=CARTESIAN_POINT('Ctrl Pts',(-2.16940517773459,-1.,3.2849901997973));
#51415=CARTESIAN_POINT('Ctrl Pts',(-2.17527380048422,-1.,3.28976645712566));
#51416=CARTESIAN_POINT('Ctrl Pts',(-2.18117455557062,-1.,3.29450361500484));
#51417=CARTESIAN_POINT('Ctrl Pts',(-2.18710556500325,-1.,3.29920022557635));
#51418=CARTESIAN_POINT('Ctrl Pts',(-2.19306710376112,-1.,3.30385816281831));
#51419=CARTESIAN_POINT('Ctrl Pts',(-2.19906078949924,-1.,3.30848134694596));
#51420=CARTESIAN_POINT('Ctrl Pts',(-2.20508863150608,-1.,3.3130742460895));
#51421=CARTESIAN_POINT('Ctrl Pts',(-2.21115211847872,-1.,3.31764044024231));
#51422=CARTESIAN_POINT('Ctrl Pts',(-2.21725135110889,-1.,3.32218125618955));
#51423=CARTESIAN_POINT('Ctrl Pts',(-2.22338548312758,-1.,3.32669646722871));
#51424=CARTESIAN_POINT('Ctrl Pts',(-2.22955308907221,-1.,3.33118487773593));
#51425=CARTESIAN_POINT('Ctrl Pts',(-2.2357525632881,-1.,3.33564495756478));
#51426=CARTESIAN_POINT('Ctrl Pts',(-2.24198249391437,-1.,3.34007543738044));
#51427=CARTESIAN_POINT('Ctrl Pts',(-2.24824207678288,-1.,3.34447596770768));
#51428=CARTESIAN_POINT('Ctrl Pts',(-2.25453097693524,-1.,3.34884690292342));
#51429=CARTESIAN_POINT('Ctrl Pts',(-2.26084915222484,-1.,3.35318902552676));
#51430=CARTESIAN_POINT('Ctrl Pts',(-2.26719668579921,-1.,3.35750328523077));
#51431=CARTESIAN_POINT('Ctrl Pts',(-2.27357362620902,-1.,3.36179055004369));
#51432=CARTESIAN_POINT('Ctrl Pts',(-2.27997979457968,-1.,3.36605130712978));
#51433=CARTESIAN_POINT('Ctrl Pts',(-2.28641481081045,-1.,3.37028570206357));
#51434=CARTESIAN_POINT('Ctrl Pts',(-2.2928781800731,-1.,3.37449367172707));
#51435=CARTESIAN_POINT('Ctrl Pts',(-2.29936936127588,-1.,3.37867504959382));
#51436=CARTESIAN_POINT('Ctrl Pts',(-2.30588783640389,-1.,3.38282967336676));
#51437=CARTESIAN_POINT('Ctrl Pts',(-2.31243319489505,-1.,3.38695751492659));
#51438=CARTESIAN_POINT('Ctrl Pts',(-2.31900513925627,-1.,3.39105869475112));
#51439=CARTESIAN_POINT('Ctrl Pts',(-2.32560343902683,-1.,3.39513342020045));
#51440=CARTESIAN_POINT('Ctrl Pts',(-2.33222789882601,-1.,3.39918194578115));
#51441=CARTESIAN_POINT('Ctrl Pts',(-2.33887832342715,-1.,3.40320452776646));
#51442=CARTESIAN_POINT('Ctrl Pts',(-2.34555447648901,-1.,3.40720137403888));
#51443=CARTESIAN_POINT('Ctrl Pts',(-2.35225606823649,-1.,3.41117262313464));
#51444=CARTESIAN_POINT('Ctrl Pts',(-2.35898278606449,-1.,3.4151183675076));
#51445=CARTESIAN_POINT('Ctrl Pts',(-2.36573431470314,-1.,3.41903866635384));
#51446=CARTESIAN_POINT('Ctrl Pts',(-2.37251035954351,-1.,3.42293356216595));
#51447=CARTESIAN_POINT('Ctrl Pts',(-2.37931067029517,-1.,3.42680309755241));
#51448=CARTESIAN_POINT('Ctrl Pts',(-2.38613505844641,-1.,3.43064732714472));
#51449=CARTESIAN_POINT('Ctrl Pts',(-2.39298338805823,-1.,3.43446630680436));
#51450=CARTESIAN_POINT('Ctrl Pts',(-2.39848113411429,-1.,3.43750133066036));
#51451=CARTESIAN_POINT('Ctrl Pts',(-2.40261515590099,-1.,3.43976627485223));
#51452=CARTESIAN_POINT('Ctrl Pts',(-2.40537592959345,-1.,3.44127120683402));
#51453=CARTESIAN_POINT('Ctrl Pts',(-2.40675750623143,-1.,3.44202241512147));
#51454=CARTESIAN_POINT('',(-2.52982887637028,-1.,3.35260583073571));
#51455=CARTESIAN_POINT('',(-2.40675750623143,-1.,3.44202241512147));
#51456=CARTESIAN_POINT('',(-2.36531447826073,-1.,2.90994629141676));
#51457=CARTESIAN_POINT('Ctrl Pts',(-2.52982887637028,-1.,3.35260583073571));
#51458=CARTESIAN_POINT('Ctrl Pts',(-2.5295413654909,-1.,3.35105973714071));
#51459=CARTESIAN_POINT('Ctrl Pts',(-2.52896321610703,-1.,3.34796903576663));
#51460=CARTESIAN_POINT('Ctrl Pts',(-2.52808660915689,-1.,3.34333744115511));
#51461=CARTESIAN_POINT('Ctrl Pts',(-2.52689902690158,-1.,3.33717089999103));
#51462=CARTESIAN_POINT('Ctrl Pts',(-2.52538321164634,-1.,3.32947762187533));
#51463=CARTESIAN_POINT('Ctrl Pts',(-2.5238359839626,-1.,3.32179931078699));
#51464=CARTESIAN_POINT('Ctrl Pts',(-2.52225724871313,-1.,3.31413607874645));
#51465=CARTESIAN_POINT('Ctrl Pts',(-2.52064689568511,-1.,3.30648808815442));
#51466=CARTESIAN_POINT('Ctrl Pts',(-2.51900480701069,-1.,3.29885556388352));
#51467=CARTESIAN_POINT('Ctrl Pts',(-2.51733085123797,-1.,3.2912387729927));
#51468=CARTESIAN_POINT('Ctrl Pts',(-2.51562487464514,-1.,3.28363799702982));
#51469=CARTESIAN_POINT('Ctrl Pts',(-2.513886692704,-1.,3.27605350473142));
#51470=CARTESIAN_POINT('Ctrl Pts',(-2.51211608411423,-1.,3.26848552888115));
#51471=CARTESIAN_POINT('Ctrl Pts',(-2.51031277813486,-1.,3.26093423001434));
#51472=CARTESIAN_POINT('Ctrl Pts',(-2.50847647070723,-1.,3.25339971460982));
#51473=CARTESIAN_POINT('Ctrl Pts',(-2.506606859405,-1.,3.24588208983849));
#51474=CARTESIAN_POINT('Ctrl Pts',(-2.5047036758003,-1.,3.23838151080319));
#51475=CARTESIAN_POINT('Ctrl Pts',(-2.50276671338111,-1.,3.23089822320646));
#51476=CARTESIAN_POINT('Ctrl Pts',(-2.50079587201957,-1.,3.22343262620503));
#51477=CARTESIAN_POINT('Ctrl Pts',(-2.4987911459939,-1.,3.21598526261286));
#51478=CARTESIAN_POINT('Ctrl Pts',(-2.4967525264737,-1.,3.20855669849836));
#51479=CARTESIAN_POINT('Ctrl Pts',(-2.49467992057755,-1.,3.20114742397588));
#51480=CARTESIAN_POINT('Ctrl Pts',(-2.49257307239848,-1.,3.19375775555798));
#51481=CARTESIAN_POINT('Ctrl Pts',(-2.49043146334059,-1.,3.18638771282266));
#51482=CARTESIAN_POINT('Ctrl Pts',(-2.48825428288201,-1.,3.17903698136622));
#51483=CARTESIAN_POINT('Ctrl Pts',(-2.48604065348587,-1.,3.17170518863313));
#51484=CARTESIAN_POINT('Ctrl Pts',(-2.48378981792725,-1.,3.16439213290161));
#51485=CARTESIAN_POINT('Ctrl Pts',(-2.48150133566571,-1.,3.15709802322739));
#51486=CARTESIAN_POINT('Ctrl Pts',(-2.47917529057029,-1.,3.14982373241352));
#51487=CARTESIAN_POINT('Ctrl Pts',(-2.47681245356109,-1.,3.1425709954655));
#51488=CARTESIAN_POINT('Ctrl Pts',(-2.47441378371932,-1.,3.13534181229295));
#51489=CARTESIAN_POINT('Ctrl Pts',(-2.47197997765871,-1.,3.12813790805952));
#51490=CARTESIAN_POINT('Ctrl Pts',(-2.46951098947469,-1.,3.12096015766983));
#51491=CARTESIAN_POINT('Ctrl Pts',(-2.46700558843506,-1.,3.11380805536122));
#51492=CARTESIAN_POINT('Ctrl Pts',(-2.46446082979646,-1.,3.1066790790198));
#51493=CARTESIAN_POINT('Ctrl Pts',(-2.46187308501884,-1.,3.09956993697052));
#51494=CARTESIAN_POINT('Ctrl Pts',(-2.4592391256388,-1.,3.09247787931887));
#51495=CARTESIAN_POINT('Ctrl Pts',(-2.45655725437039,-1.,3.08540206545315));
#51496=CARTESIAN_POINT('Ctrl Pts',(-2.4538282678779,-1.,3.07834472886139));
#51497=CARTESIAN_POINT('Ctrl Pts',(-2.45105688854422,-1.,3.07131290521297));
#51498=CARTESIAN_POINT('Ctrl Pts',(-2.44824970516544,-1.,3.06431596421405));
#51499=CARTESIAN_POINT('Ctrl Pts',(-2.44541251892556,-1.,3.05736242671506));
#51500=CARTESIAN_POINT('Ctrl Pts',(-2.44254768923105,-1.,3.05045678021504));
#51501=CARTESIAN_POINT('Ctrl Pts',(-2.43965194061857,-1.,3.04359685040555));
#51502=CARTESIAN_POINT('Ctrl Pts',(-2.43671278042414,-1.,3.03676949672821));
#51503=CARTESIAN_POINT('Ctrl Pts',(-2.43371241361488,-1.,3.02995534946978));
#51504=CARTESIAN_POINT('Ctrl Pts',(-2.43063415586637,-1.,3.02313656036004));
#51505=CARTESIAN_POINT('Ctrl Pts',(-2.42746856264168,-1.,3.01630420830504));
#51506=CARTESIAN_POINT('Ctrl Pts',(-2.42421849439613,-1.,3.00946442616658));
#51507=CARTESIAN_POINT('Ctrl Pts',(-2.42090763946779,-1.,3.00264868585996));
#51508=CARTESIAN_POINT('Ctrl Pts',(-2.41757324500514,-1.,2.99590509293503));
#51509=CARTESIAN_POINT('Ctrl Pts',(-2.41425064199586,-1.,2.98927983005796));
#51510=CARTESIAN_POINT('Ctrl Pts',(-2.41095909342571,-1.,2.98280015815107));
#51511=CARTESIAN_POINT('Ctrl Pts',(-2.40768975073713,-1.,2.97646002822422));
#51512=CARTESIAN_POINT('Ctrl Pts',(-2.40438604734919,-1.,2.9701964131236));
#51513=CARTESIAN_POINT('Ctrl Pts',(-2.4009556571164,-1.,2.96390432240312));
#51514=CARTESIAN_POINT('Ctrl Pts',(-2.39730553974517,-1.,2.95748006482942));
#51515=CARTESIAN_POINT('Ctrl Pts',(-2.39337207631667,-1.,2.95085857128439));
#51516=CARTESIAN_POINT('Ctrl Pts',(-2.38914929090759,-1.,2.94404820669076));
#51517=CARTESIAN_POINT('Ctrl Pts',(-2.38472771516311,-1.,2.93717903280391));
#51518=CARTESIAN_POINT('Ctrl Pts',(-2.38028989582073,-1.,2.93049643640206));
#51519=CARTESIAN_POINT('Ctrl Pts',(-2.3760651052403,-1.,2.92430340582608));
#51520=CARTESIAN_POINT('Ctrl Pts',(-2.37229381109821,-1.,2.91891503791411));
#51521=CARTESIAN_POINT('Ctrl Pts',(-2.36919161373173,-1.,2.9146124988314));
#51522=CARTESIAN_POINT('Ctrl Pts',(-2.36707658451664,-1.,2.91181344022549));
#51523=CARTESIAN_POINT('Ctrl Pts',(-2.36599991765749,-1.,2.91051690822156));
#51524=CARTESIAN_POINT('Ctrl Pts',(-2.36553202948613,-1.,2.91005770527719));
#51525=CARTESIAN_POINT('Ctrl Pts',(-2.36536211188453,-1.,2.90995756655606));
#51526=CARTESIAN_POINT('Ctrl Pts',(-2.36531447826074,-1.,2.90994629141676));
#51527=CARTESIAN_POINT('',(-2.50410331873042,-1.,2.79140942341378));
#51528=CARTESIAN_POINT('Origin',(0.,-1.,0.));
#51529=CARTESIAN_POINT('',(-2.91557726271063,-1.,3.02314558451372));
#51530=CARTESIAN_POINT('Ctrl Pts',(-2.50410331873042,-1.,2.79140942341378));
#51531=CARTESIAN_POINT('Ctrl Pts',(-2.50410700351426,-1.,2.79145823440899));
#51532=CARTESIAN_POINT('Ctrl Pts',(-2.50417932839343,-1.,2.79164172519039));
#51533=CARTESIAN_POINT('Ctrl Pts',(-2.50455968395235,-1.,2.79217568804874));
#51534=CARTESIAN_POINT('Ctrl Pts',(-2.50567182569153,-1.,2.79344192164204));
#51535=CARTESIAN_POINT('Ctrl Pts',(-2.50810555977564,-1.,2.7959687805717));
#51536=CARTESIAN_POINT('Ctrl Pts',(-2.51186983687947,-1.,2.79970585014308));
#51537=CARTESIAN_POINT('Ctrl Pts',(-2.51660190466067,-1.,2.80427363984939));
#51538=CARTESIAN_POINT('Ctrl Pts',(-2.52205778589922,-1.,2.80941521967234));
#51539=CARTESIAN_POINT('Ctrl Pts',(-2.52796388055457,-1.,2.8148437904867));
#51540=CARTESIAN_POINT('Ctrl Pts',(-2.53405679667463,-1.,2.82028550483744));
#51541=CARTESIAN_POINT('Ctrl Pts',(-2.54012272520141,-1.,2.82552167649157));
#51542=CARTESIAN_POINT('Ctrl Pts',(-2.54604736792542,-1.,2.83044254225794));
#51543=CARTESIAN_POINT('Ctrl Pts',(-2.55182152806964,-1.,2.83505269592412));
#51544=CARTESIAN_POINT('Ctrl Pts',(-2.55749952145165,-1.,2.83942515220699));
#51545=CARTESIAN_POINT('Ctrl Pts',(-2.56316920798489,-1.,2.84366802680211));
#51546=CARTESIAN_POINT('Ctrl Pts',(-2.56891984251743,-1.,2.84788893329091));
#51547=CARTESIAN_POINT('Ctrl Pts',(-2.57480482727128,-1.,2.85215360144483));
#51548=CARTESIAN_POINT('Ctrl Pts',(-2.58082875254407,-1.,2.85647171715147));
#51549=CARTESIAN_POINT('Ctrl Pts',(-2.5869677064356,-1.,2.86081999003668));
#51550=CARTESIAN_POINT('Ctrl Pts',(-2.59318160184921,-1.,2.86515629953528));
#51551=CARTESIAN_POINT('Ctrl Pts',(-2.59942875223202,-1.,2.86943633170712));
#51552=CARTESIAN_POINT('Ctrl Pts',(-2.6056817788128,-1.,2.87363176656475));
#51553=CARTESIAN_POINT('Ctrl Pts',(-2.61193507170928,-1.,2.87773881947885));
#51554=CARTESIAN_POINT('Ctrl Pts',(-2.61819596473087,-1.,2.88176821427502));
#51555=CARTESIAN_POINT('Ctrl Pts',(-2.62447947640253,-1.,2.88573922195049));
#51556=CARTESIAN_POINT('Ctrl Pts',(-2.63080195420771,-1.,2.88967244854243));
#51557=CARTESIAN_POINT('Ctrl Pts',(-2.63717442263944,-1.,2.89358228854557));
#51558=CARTESIAN_POINT('Ctrl Pts',(-2.64359851684146,-1.,2.89747231723361));
#51559=CARTESIAN_POINT('Ctrl Pts',(-2.65007017365576,-1.,2.90133950224879));
#51560=CARTESIAN_POINT('Ctrl Pts',(-2.65658188464287,-1.,2.90517678087467));
#51561=CARTESIAN_POINT('Ctrl Pts',(-2.66312542616809,-1.,2.90897617968921));
#51562=CARTESIAN_POINT('Ctrl Pts',(-2.66969458792627,-1.,2.91273193382876));
#51563=CARTESIAN_POINT('Ctrl Pts',(-2.67628728855309,-1.,2.91644290704281));
#51564=CARTESIAN_POINT('Ctrl Pts',(-2.68290409279689,-1.,2.92011090722152));
#51565=CARTESIAN_POINT('Ctrl Pts',(-2.68954721165342,-1.,2.92373955325876));
#51566=CARTESIAN_POINT('Ctrl Pts',(-2.69621932864302,-1.,2.92733294395268));
#51567=CARTESIAN_POINT('Ctrl Pts',(-2.70292247416881,-1.,2.93089438233746));
#51568=CARTESIAN_POINT('Ctrl Pts',(-2.70965695523776,-1.,2.93442516311168));
#51569=CARTESIAN_POINT('Ctrl Pts',(-2.71642190053575,-1.,2.93792519474955));
#51570=CARTESIAN_POINT('Ctrl Pts',(-2.72321571511322,-1.,2.94139351933882));
#51571=CARTESIAN_POINT('Ctrl Pts',(-2.73003657371613,-1.,2.94482887675139));
#51572=CARTESIAN_POINT('Ctrl Pts',(-2.73688288329825,-1.,2.94823023414381));
#51573=CARTESIAN_POINT('Ctrl Pts',(-2.7437537949221,-1.,2.95159737214305));
#51574=CARTESIAN_POINT('Ctrl Pts',(-2.75064903318996,-1.,2.95493069316211));
#51575=CARTESIAN_POINT('Ctrl Pts',(-2.75756867888393,-1.,2.9582309766594));
#51576=CARTESIAN_POINT('Ctrl Pts',(-2.76451296269571,-1.,2.96149914764832));
#51577=CARTESIAN_POINT('Ctrl Pts',(-2.77148206836464,-1.,2.96473605585548));
#51578=CARTESIAN_POINT('Ctrl Pts',(-2.77847589542767,-1.,2.9679422104295));
#51579=CARTESIAN_POINT('Ctrl Pts',(-2.78549409123657,-1.,2.97111781461349));
#51580=CARTESIAN_POINT('Ctrl Pts',(-2.79253615718147,-1.,2.97426288347475));
#51581=CARTESIAN_POINT('Ctrl Pts',(-2.79960153278186,-1.,2.97737733718242));
#51582=CARTESIAN_POINT('Ctrl Pts',(-2.80668968101162,-1.,2.98046109647299));
#51583=CARTESIAN_POINT('Ctrl Pts',(-2.81380019196454,-1.,2.9835141977994));
#51584=CARTESIAN_POINT('Ctrl Pts',(-2.82093279065704,-1.,2.98653680669434));
#51585=CARTESIAN_POINT('Ctrl Pts',(-2.82808728190402,-1.,2.98952916401699));
#51586=CARTESIAN_POINT('Ctrl Pts',(-2.83526351254383,-1.,2.99249155170479));
#51587=CARTESIAN_POINT('Ctrl Pts',(-2.84246132984334,-1.,2.995424253416));
#51588=CARTESIAN_POINT('Ctrl Pts',(-2.84968053289104,-1.,2.99832751144566));
#51589=CARTESIAN_POINT('Ctrl Pts',(-2.85692085715129,-1.,3.0012015079552));
#51590=CARTESIAN_POINT('Ctrl Pts',(-2.86418200833065,-1.,3.00404638316245));
#51591=CARTESIAN_POINT('Ctrl Pts',(-2.87146368430104,-1.,3.00686224485374));
#51592=CARTESIAN_POINT('Ctrl Pts',(-2.87876560072799,-1.,3.0096491810855));
#51593=CARTESIAN_POINT('Ctrl Pts',(-2.88608751706796,-1.,3.01240727309568));
#51594=CARTESIAN_POINT('Ctrl Pts',(-2.8934292556764,-1.,3.01513660433291));
#51595=CARTESIAN_POINT('Ctrl Pts',(-2.90079069102661,-1.,3.01783725123646));
#51596=CARTESIAN_POINT('Ctrl Pts',(-2.90669553303902,-1.,3.01997487194926));
#51597=CARTESIAN_POINT('Ctrl Pts',(-2.91113297349052,-1.,3.02156522743299));
#51598=CARTESIAN_POINT('Ctrl Pts',(-2.91409518070707,-1.,3.02261975104912));
#51599=CARTESIAN_POINT('Ctrl Pts',(-2.91557726271063,-1.,3.02314558451372));
#51600=CARTESIAN_POINT('',(-3.02314558451372,-1.,2.91557726271063));
#51601=CARTESIAN_POINT('',(-2.91557726271063,-1.,3.02314558451372));
#51602=CARTESIAN_POINT('',(-2.79140942341258,-1.,2.50410331873176));
#51603=CARTESIAN_POINT('Ctrl Pts',(-3.02314558451372,-1.,2.91557726271063));
#51604=CARTESIAN_POINT('Ctrl Pts',(-3.02261975104593,-1.,2.91409518070399));
#51605=CARTESIAN_POINT('Ctrl Pts',(-3.02156522742431,-1.,2.91113297348212));
#51606=CARTESIAN_POINT('Ctrl Pts',(-3.01997487193503,-1.,2.90669553302526));
#51607=CARTESIAN_POINT('Ctrl Pts',(-3.01783725121981,-1.,2.9007906910105));
#51608=CARTESIAN_POINT('Ctrl Pts',(-3.01513660431928,-1.,2.89342925566321));
#51609=CARTESIAN_POINT('Ctrl Pts',(-3.01240727308829,-1.,2.8860875170608));
#51610=CARTESIAN_POINT('Ctrl Pts',(-3.00964918108476,-1.,2.87876560072727));
#51611=CARTESIAN_POINT('Ctrl Pts',(-3.00686224485784,-1.,2.87146368430502));
#51612=CARTESIAN_POINT('Ctrl Pts',(-3.00404638316867,-1.,2.86418200833667));
#51613=CARTESIAN_POINT('Ctrl Pts',(-3.00120150796095,-1.,2.85692085715686));
#51614=CARTESIAN_POINT('Ctrl Pts',(-2.99832751144925,-1.,2.84968053289451));
#51615=CARTESIAN_POINT('Ctrl Pts',(-2.99542425341685,-1.,2.84246132984415));
#51616=CARTESIAN_POINT('Ctrl Pts',(-2.9924915517034,-1.,2.83526351254248));
#51617=CARTESIAN_POINT('Ctrl Pts',(-2.98952916401446,-1.,2.82808728190157));
#51618=CARTESIAN_POINT('Ctrl Pts',(-2.9865368066918,-1.,2.82093279065457));
#51619=CARTESIAN_POINT('Ctrl Pts',(-2.98351419779767,-1.,2.81380019196286));
#51620=CARTESIAN_POINT('Ctrl Pts',(-2.98046109647241,-1.,2.80668968101106));
#51621=CARTESIAN_POINT('Ctrl Pts',(-2.97737733718287,-1.,2.7996015327823));
#51622=CARTESIAN_POINT('Ctrl Pts',(-2.9742628834758,-1.,2.79253615718248));
#51623=CARTESIAN_POINT('Ctrl Pts',(-2.97111781461465,-1.,2.78549409123769));
#51624=CARTESIAN_POINT('Ctrl Pts',(-2.96794221043036,-1.,2.7784758954285));
#51625=CARTESIAN_POINT('Ctrl Pts',(-2.96473605585583,-1.,2.77148206836498));
#51626=CARTESIAN_POINT('Ctrl Pts',(-2.96149914764818,-1.,2.76451296269557));
#51627=CARTESIAN_POINT('Ctrl Pts',(-2.95823097665896,-1.,2.7575686788835));
#51628=CARTESIAN_POINT('Ctrl Pts',(-2.95493069316161,-1.,2.75064903318947));
#51629=CARTESIAN_POINT('Ctrl Pts',(-2.95159737214266,-1.,2.74375379492172));
#51630=CARTESIAN_POINT('Ctrl Pts',(-2.94823023414364,-1.,2.73688288329808));
#51631=CARTESIAN_POINT('Ctrl Pts',(-2.94482887675143,-1.,2.73003657371617));
#51632=CARTESIAN_POINT('Ctrl Pts',(-2.94139351933897,-1.,2.72321571511337));
#51633=CARTESIAN_POINT('Ctrl Pts',(-2.93792519474972,-1.,2.71642190053592));
#51634=CARTESIAN_POINT('Ctrl Pts',(-2.93442516311179,-1.,2.70965695523787));
#51635=CARTESIAN_POINT('Ctrl Pts',(-2.9308943823375,-1.,2.70292247416885));
#51636=CARTESIAN_POINT('Ctrl Pts',(-2.92733294395267,-1.,2.69621932864301));
#51637=CARTESIAN_POINT('Ctrl Pts',(-2.92373955325875,-1.,2.68954721165339));
#51638=CARTESIAN_POINT('Ctrl Pts',(-2.92011090722152,-1.,2.68290409279688));
#51639=CARTESIAN_POINT('Ctrl Pts',(-2.91644290704285,-1.,2.67628728855312));
#51640=CARTESIAN_POINT('Ctrl Pts',(-2.91273193382882,-1.,2.66969458792631));
#51641=CARTESIAN_POINT('Ctrl Pts',(-2.90897617968923,-1.,2.6631254261681));
#51642=CARTESIAN_POINT('Ctrl Pts',(-2.90517678087461,-1.,2.65658188464282));
#51643=CARTESIAN_POINT('Ctrl Pts',(-2.90133950224867,-1.,2.65007017365564));
#51644=CARTESIAN_POINT('Ctrl Pts',(-2.89747231723345,-1.,2.64359851684131));
#51645=CARTESIAN_POINT('Ctrl Pts',(-2.89358228854544,-1.,2.63717442263932));
#51646=CARTESIAN_POINT('Ctrl Pts',(-2.88967244854239,-1.,2.63080195420767));
#51647=CARTESIAN_POINT('Ctrl Pts',(-2.88573922195059,-1.,2.62447947640262));
#51648=CARTESIAN_POINT('Ctrl Pts',(-2.88176821427525,-1.,2.61819596473108));
#51649=CARTESIAN_POINT('Ctrl Pts',(-2.87773881947916,-1.,2.61193507170955));
#51650=CARTESIAN_POINT('Ctrl Pts',(-2.87363176656501,-1.,2.60568177881303));
#51651=CARTESIAN_POINT('Ctrl Pts',(-2.86943633170722,-1.,2.5994287522321));
#51652=CARTESIAN_POINT('Ctrl Pts',(-2.86515629953513,-1.,2.59318160184908));
#51653=CARTESIAN_POINT('Ctrl Pts',(-2.86081999003629,-1.,2.58696770643524));
#51654=CARTESIAN_POINT('Ctrl Pts',(-2.85647171715092,-1.,2.58082875254357));
#51655=CARTESIAN_POINT('Ctrl Pts',(-2.85215360144431,-1.,2.57480482727081));
#51656=CARTESIAN_POINT('Ctrl Pts',(-2.84788893329067,-1.,2.56891984251721));
#51657=CARTESIAN_POINT('Ctrl Pts',(-2.84366802680237,-1.,2.56316920798513));
#51658=CARTESIAN_POINT('Ctrl Pts',(-2.83942515220782,-1.,2.55749952145241));
#51659=CARTESIAN_POINT('Ctrl Pts',(-2.83505269592536,-1.,2.55182152807077));
#51660=CARTESIAN_POINT('Ctrl Pts',(-2.83044254225917,-1.,2.54604736792655));
#51661=CARTESIAN_POINT('Ctrl Pts',(-2.8255216764922,-1.,2.54012272520199));
#51662=CARTESIAN_POINT('Ctrl Pts',(-2.82028550483689,-1.,2.53405679667412));
#51663=CARTESIAN_POINT('Ctrl Pts',(-2.81484379048475,-1.,2.52796388055278));
#51664=CARTESIAN_POINT('Ctrl Pts',(-2.80941521966941,-1.,2.52205778589653));
#51665=CARTESIAN_POINT('Ctrl Pts',(-2.80427363984653,-1.,2.51660190465805));
#51666=CARTESIAN_POINT('Ctrl Pts',(-2.79970585014168,-1.,2.51186983687818));
#51667=CARTESIAN_POINT('Ctrl Pts',(-2.79596878057287,-1.,2.50810555977671));
#51668=CARTESIAN_POINT('Ctrl Pts',(-2.79344192164147,-1.,2.50567182569081));
#51669=CARTESIAN_POINT('Ctrl Pts',(-2.79217568804755,-1.,2.50455968395146));
#51670=CARTESIAN_POINT('Ctrl Pts',(-2.79164172518905,-1.,2.50417932839313));
#51671=CARTESIAN_POINT('Ctrl Pts',(-2.79145823440781,-1.,2.50410700351493));
#51672=CARTESIAN_POINT('Ctrl Pts',(-2.79140942341258,-1.,2.50410331873176));
#51673=CARTESIAN_POINT('',(-2.90994629141562,-1.,2.36531447826213));
#51674=CARTESIAN_POINT('Origin',(0.,-1.,0.));
#51675=CARTESIAN_POINT('',(-3.35260583073571,-1.,2.52982887637028));
#51676=CARTESIAN_POINT('Ctrl Pts',(-2.90994629141562,-1.,2.36531447826213));
#51677=CARTESIAN_POINT('Ctrl Pts',(-2.90995756655558,-1.,2.3653621118858));
#51678=CARTESIAN_POINT('Ctrl Pts',(-2.9100577052777,-1.,2.36553202948741));
#51679=CARTESIAN_POINT('Ctrl Pts',(-2.91051690822262,-1.,2.36599991765853));
#51680=CARTESIAN_POINT('Ctrl Pts',(-2.91181344022628,-1.,2.36707658451709));
#51681=CARTESIAN_POINT('Ctrl Pts',(-2.91461249883016,-1.,2.36919161373074));
#51682=CARTESIAN_POINT('Ctrl Pts',(-2.9189150379156,-1.,2.37229381109939));
#51683=CARTESIAN_POINT('Ctrl Pts',(-2.92430340582912,-1.,2.37606510524271));
#51684=CARTESIAN_POINT('Ctrl Pts',(-2.93049643640517,-1.,2.3802898958232));
#51685=CARTESIAN_POINT('Ctrl Pts',(-2.93717903280599,-1.,2.38472771516476));
#51686=CARTESIAN_POINT('Ctrl Pts',(-2.94404820669135,-1.,2.38914929090806));
#51687=CARTESIAN_POINT('Ctrl Pts',(-2.95085857128372,-1.,2.39337207631613));
#51688=CARTESIAN_POINT('Ctrl Pts',(-2.95748006482811,-1.,2.39730553974412));
#51689=CARTESIAN_POINT('Ctrl Pts',(-2.96390432240181,-1.,2.40095565711535));
#51690=CARTESIAN_POINT('Ctrl Pts',(-2.97019641312272,-1.,2.40438604734848));
#51691=CARTESIAN_POINT('Ctrl Pts',(-2.97646002822395,-1.,2.40768975073691));
#51692=CARTESIAN_POINT('Ctrl Pts',(-2.98280015815132,-1.,2.41095909342591));
#51693=CARTESIAN_POINT('Ctrl Pts',(-2.98927983005851,-1.,2.4142506419963));
#51694=CARTESIAN_POINT('Ctrl Pts',(-2.99590509293561,-1.,2.4175732450056));
#51695=CARTESIAN_POINT('Ctrl Pts',(-3.00264868586038,-1.,2.42090763946812));
#51696=CARTESIAN_POINT('Ctrl Pts',(-3.00946442616674,-1.,2.42421849439625));
#51697=CARTESIAN_POINT('Ctrl Pts',(-3.01630420830494,-1.,2.4274685626416));
#51698=CARTESIAN_POINT('Ctrl Pts',(-3.02313656035977,-1.,2.43063415586615));
#51699=CARTESIAN_POINT('Ctrl Pts',(-3.02995534946946,-1.,2.43371241361462));
#51700=CARTESIAN_POINT('Ctrl Pts',(-3.03676949672797,-1.,2.43671278042394));
#51701=CARTESIAN_POINT('Ctrl Pts',(-3.04359685040545,-1.,2.43965194061849));
#51702=CARTESIAN_POINT('Ctrl Pts',(-3.05045678021509,-1.,2.44254768923109));
#51703=CARTESIAN_POINT('Ctrl Pts',(-3.05736242671521,-1.,2.44541251892568));
#51704=CARTESIAN_POINT('Ctrl Pts',(-3.06431596421422,-1.,2.44824970516558));
#51705=CARTESIAN_POINT('Ctrl Pts',(-3.0713129052131,-1.,2.45105688854432));
#51706=CARTESIAN_POINT('Ctrl Pts',(-3.07834472886145,-1.,2.45382826787795));
#51707=CARTESIAN_POINT('Ctrl Pts',(-3.08540206545313,-1.,2.45655725437037));
#51708=CARTESIAN_POINT('Ctrl Pts',(-3.09247787931881,-1.,2.45923912563875));
#51709=CARTESIAN_POINT('Ctrl Pts',(-3.09956993697048,-1.,2.4618730850188));
#51710=CARTESIAN_POINT('Ctrl Pts',(-3.10667907901981,-1.,2.46446082979645));
#51711=CARTESIAN_POINT('Ctrl Pts',(-3.11380805536124,-1.,2.46700558843507));
#51712=CARTESIAN_POINT('Ctrl Pts',(-3.12096015766984,-1.,2.4695109894747));
#51713=CARTESIAN_POINT('Ctrl Pts',(-3.12813790805948,-1.,2.47197997765868));
#51714=CARTESIAN_POINT('Ctrl Pts',(-3.13534181229282,-1.,2.47441378371923));
#51715=CARTESIAN_POINT('Ctrl Pts',(-3.14257099546531,-1.,2.47681245356095));
#51716=CARTESIAN_POINT('Ctrl Pts',(-3.14982373241335,-1.,2.47917529057016));
#51717=CARTESIAN_POINT('Ctrl Pts',(-3.15709802322735,-1.,2.48150133566568));
#51718=CARTESIAN_POINT('Ctrl Pts',(-3.16439213290181,-1.,2.48378981792739));
#51719=CARTESIAN_POINT('Ctrl Pts',(-3.17170518863357,-1.,2.48604065348619));
#51720=CARTESIAN_POINT('Ctrl Pts',(-3.17903698136679,-1.,2.48825428288243));
#51721=CARTESIAN_POINT('Ctrl Pts',(-3.18638771282315,-1.,2.49043146334095));
#51722=CARTESIAN_POINT('Ctrl Pts',(-3.19375775555814,-1.,2.4925730723986));
#51723=CARTESIAN_POINT('Ctrl Pts',(-3.20114742397549,-1.,2.49467992057726));
#51724=CARTESIAN_POINT('Ctrl Pts',(-3.2085566984974,-1.,2.49675252647298));
#51725=CARTESIAN_POINT('Ctrl Pts',(-3.21598526261157,-1.,2.49879114599293));
#51726=CARTESIAN_POINT('Ctrl Pts',(-3.22343262620387,-1.,2.5007958720187));
#51727=CARTESIAN_POINT('Ctrl Pts',(-3.23089822320596,-1.,2.50276671338074));
#51728=CARTESIAN_POINT('Ctrl Pts',(-3.23838151080383,-1.,2.50470367580078));
#51729=CARTESIAN_POINT('Ctrl Pts',(-3.24588208984042,-1.,2.50660685940645));
#51730=CARTESIAN_POINT('Ctrl Pts',(-3.25339971461265,-1.,2.50847647070936));
#51731=CARTESIAN_POINT('Ctrl Pts',(-3.26093423001716,-1.,2.51031277813697));
#51732=CARTESIAN_POINT('Ctrl Pts',(-3.26848552888271,-1.,2.51211608411539));
#51733=CARTESIAN_POINT('Ctrl Pts',(-3.27605350473048,-1.,2.51388669270329));
#51734=CARTESIAN_POINT('Ctrl Pts',(-3.28363799702583,-1.,2.51562487464215));
#51735=CARTESIAN_POINT('Ctrl Pts',(-3.2912387729863,-1.,2.51733085123316));
#51736=CARTESIAN_POINT('Ctrl Pts',(-3.29885556387661,-1.,2.51900480700548));
#51737=CARTESIAN_POINT('Ctrl Pts',(-3.30648808814986,-1.,2.52064689568167));
#51738=CARTESIAN_POINT('Ctrl Pts',(-3.31413607874727,-1.,2.52225724871375));
#51739=CARTESIAN_POINT('Ctrl Pts',(-3.32179931079521,-1.,2.52383598396878));
#51740=CARTESIAN_POINT('Ctrl Pts',(-3.32947762189049,-1.,2.52538321165774));
#51741=CARTESIAN_POINT('Ctrl Pts',(-3.33717090000955,-1.,2.52689902691551));
#51742=CARTESIAN_POINT('Ctrl Pts',(-3.34333744117093,-1.,2.52808660916879));
#51743=CARTESIAN_POINT('Ctrl Pts',(-3.34796903577628,-1.,2.5289632161143));
#51744=CARTESIAN_POINT('Ctrl Pts',(-3.35105973714426,-1.,2.52954136549357));
#51745=CARTESIAN_POINT('Ctrl Pts',(-3.35260583073571,-1.,2.52982887637028));
#51746=CARTESIAN_POINT('',(-3.44202241512147,-1.,2.40675750623143));
#51747=CARTESIAN_POINT('',(-3.35260583073571,-1.,2.52982887637028));
#51748=CARTESIAN_POINT('',(-3.14877060440327,-1.,2.03660101169715));
#51749=CARTESIAN_POINT('Ctrl Pts',(-3.44202241512147,-1.,2.40675750623143));
#51750=CARTESIAN_POINT('Ctrl Pts',(-3.44127120683039,-1.,2.4053759295909));
#51751=CARTESIAN_POINT('Ctrl Pts',(-3.43976627484234,-1.,2.40261515589405));
#51752=CARTESIAN_POINT('Ctrl Pts',(-3.43750133064416,-1.,2.39848113410292));
#51753=CARTESIAN_POINT('Ctrl Pts',(-3.4344663067854,-1.,2.39298338804493));
#51754=CARTESIAN_POINT('Ctrl Pts',(-3.4306473271292,-1.,2.38613505843552));
#51755=CARTESIAN_POINT('Ctrl Pts',(-3.42680309754399,-1.,2.37931067028926));
#51756=CARTESIAN_POINT('Ctrl Pts',(-3.42293356216511,-1.,2.37251035954292));
#51757=CARTESIAN_POINT('Ctrl Pts',(-3.41903866635852,-1.,2.36573431470642));
#51758=CARTESIAN_POINT('Ctrl Pts',(-3.41511836751469,-1.,2.35898278606946));
#51759=CARTESIAN_POINT('Ctrl Pts',(-3.41117262314119,-1.,2.35225606824109));
#51760=CARTESIAN_POINT('Ctrl Pts',(-3.40720137404297,-1.,2.34555447649188));
#51761=CARTESIAN_POINT('Ctrl Pts',(-3.40320452776743,-1.,2.33887832342782));
#51762=CARTESIAN_POINT('Ctrl Pts',(-3.39918194577956,-1.,2.33222789882489));
#51763=CARTESIAN_POINT('Ctrl Pts',(-3.39513342019756,-1.,2.3256034390248));
#51764=CARTESIAN_POINT('Ctrl Pts',(-3.39105869474822,-1.,2.31900513925424));
#51765=CARTESIAN_POINT('Ctrl Pts',(-3.38695751492462,-1.,2.31243319489367));
#51766=CARTESIAN_POINT('Ctrl Pts',(-3.3828296733661,-1.,2.30588783640343));
#51767=CARTESIAN_POINT('Ctrl Pts',(-3.37867504959433,-1.,2.29936936127624));
#51768=CARTESIAN_POINT('Ctrl Pts',(-3.37449367172826,-1.,2.29287818007393));
#51769=CARTESIAN_POINT('Ctrl Pts',(-3.37028570206488,-1.,2.28641481081137));
#51770=CARTESIAN_POINT('Ctrl Pts',(-3.36605130713076,-1.,2.27997979458037));
#51771=CARTESIAN_POINT('Ctrl Pts',(-3.36179055004409,-1.,2.2735736262093));
#51772=CARTESIAN_POINT('Ctrl Pts',(-3.35750328523061,-1.,2.2671966857991));
#51773=CARTESIAN_POINT('Ctrl Pts',(-3.35318902552626,-1.,2.26084915222449));
#51774=CARTESIAN_POINT('Ctrl Pts',(-3.34884690292285,-1.,2.25453097693483));
#51775=CARTESIAN_POINT('Ctrl Pts',(-3.34447596770723,-1.,2.24824207678256));
#51776=CARTESIAN_POINT('Ctrl Pts',(-3.34007543738025,-1.,2.24198249391422));
#51777=CARTESIAN_POINT('Ctrl Pts',(-3.33564495756482,-1.,2.23575256328812));
#51778=CARTESIAN_POINT('Ctrl Pts',(-3.33118487773611,-1.,2.22955308907233));
#51779=CARTESIAN_POINT('Ctrl Pts',(-3.3266964672289,-1.,2.22338548312772));
#51780=CARTESIAN_POINT('Ctrl Pts',(-3.32218125618968,-1.,2.21725135110898));
#51781=CARTESIAN_POINT('Ctrl Pts',(-3.31764044024235,-1.,2.21115211847875));
#51782=CARTESIAN_POINT('Ctrl Pts',(-3.31307424608949,-1.,2.20508863150607));
#51783=CARTESIAN_POINT('Ctrl Pts',(-3.30848134694595,-1.,2.19906078949923));
#51784=CARTESIAN_POINT('Ctrl Pts',(-3.30385816281831,-1.,2.19306710376111));
#51785=CARTESIAN_POINT('Ctrl Pts',(-3.29920022557639,-1.,2.18710556500327));
#51786=CARTESIAN_POINT('Ctrl Pts',(-3.2945036150049,-1.,2.18117455557065));
#51787=CARTESIAN_POINT('Ctrl Pts',(-3.28976645712568,-1.,2.17527380048423));
#51788=CARTESIAN_POINT('Ctrl Pts',(-3.28499019979724,-1.,2.16940517773455));
#51789=CARTESIAN_POINT('Ctrl Pts',(-3.280181508414,-1.,2.16357391934425));
#51790=CARTESIAN_POINT('Ctrl Pts',(-3.27534954469187,-1.,2.15778690038347));
#51791=CARTESIAN_POINT('Ctrl Pts',(-3.27050245897228,-1.,2.15205043199808));
#51792=CARTESIAN_POINT('Ctrl Pts',(-3.26564388189759,-1.,2.1463680529566));
#51793=CARTESIAN_POINT('Ctrl Pts',(-3.26077002641879,-1.,2.14073870754264));
#51794=CARTESIAN_POINT('Ctrl Pts',(-3.25586495065054,-1.,2.13515375878803));
#51795=CARTESIAN_POINT('Ctrl Pts',(-3.25090574494028,-1.,2.12960028396832));
#51796=CARTESIAN_POINT('Ctrl Pts',(-3.24587102613376,-1.,2.12406646410962));
#51797=CARTESIAN_POINT('Ctrl Pts',(-3.24074905517293,-1.,2.11854673326979));
#51798=CARTESIAN_POINT('Ctrl Pts',(-3.23554444767099,-1.,2.11304604021773));
#51799=CARTESIAN_POINT('Ctrl Pts',(-3.23028945793289,-1.,2.10758699642451));
#51800=CARTESIAN_POINT('Ctrl Pts',(-3.22503437553434,-1.,2.10220384298492));
#51801=CARTESIAN_POINT('Ctrl Pts',(-3.21982707347009,-1.,2.09692958434895));
#51802=CARTESIAN_POINT('Ctrl Pts',(-3.21469429601654,-1.,2.09178419460443));
#51803=CARTESIAN_POINT('Ctrl Pts',(-3.20962575845463,-1.,2.08676465517455));
#51804=CARTESIAN_POINT('Ctrl Pts',(-3.2045481863073,-1.,2.08182850370878));
#51805=CARTESIAN_POINT('Ctrl Pts',(-3.19934132836019,-1.,2.07690441870722));
#51806=CARTESIAN_POINT('Ctrl Pts',(-3.19388465568252,-1.,2.07192253497857));
#51807=CARTESIAN_POINT('Ctrl Pts',(-3.18809755562368,-1.,2.06684062744112));
#51808=CARTESIAN_POINT('Ctrl Pts',(-3.18197692964614,-1.,2.06166849827101));
#51809=CARTESIAN_POINT('Ctrl Pts',(-3.17564906975371,-1.,2.05650186773132));
#51810=CARTESIAN_POINT('Ctrl Pts',(-3.16936341689527,-1.,2.05151770247233));
#51811=CARTESIAN_POINT('Ctrl Pts',(-3.16343165058912,-1.,2.04693331247446));
#51812=CARTESIAN_POINT('Ctrl Pts',(-3.15817983946367,-1.,2.04297406404027));
#51813=CARTESIAN_POINT('Ctrl Pts',(-3.15389991674792,-1.,2.03984073791519));
#51814=CARTESIAN_POINT('Ctrl Pts',(-3.15102344775328,-1.,2.03783225495961));
#51815=CARTESIAN_POINT('Ctrl Pts',(-3.14959882629805,-1.,2.03693188810544));
#51816=CARTESIAN_POINT('Ctrl Pts',(-3.1490119366901,-1.,2.03663974554932));
#51817=CARTESIAN_POINT('Ctrl Pts',(-3.14881939088124,-1.,2.03659701539259));
#51818=CARTESIAN_POINT('Ctrl Pts',(-3.14877060440328,-1.,2.03660101169715));
#51819=CARTESIAN_POINT('',(-3.24413672884812,-1.,1.88097764062697));
#51820=CARTESIAN_POINT('Origin',(0.,-1.,0.));
#51821=CARTESIAN_POINT('',(-3.70708211654725,-1.,1.97421938526992));
#51822=CARTESIAN_POINT('Ctrl Pts',(-3.24413672884812,-1.,1.88097764062697));
#51823=CARTESIAN_POINT('Ctrl Pts',(-3.24415531671284,-1.,1.8810229239812));
#51824=CARTESIAN_POINT('Ctrl Pts',(-3.24428080353022,-1.,1.88117508446775));
#51825=CARTESIAN_POINT('Ctrl Pts',(-3.24480754676064,-1.,1.88156537699203));
#51826=CARTESIAN_POINT('Ctrl Pts',(-3.2462565441079,-1.,1.88242596600454));
#51827=CARTESIAN_POINT('Ctrl Pts',(-3.24935200511918,-1.,1.88407708646357));
#51828=CARTESIAN_POINT('Ctrl Pts',(-3.25408686339463,-1.,1.88646802523466));
#51829=CARTESIAN_POINT('Ctrl Pts',(-3.25999885193947,-1.,1.88934996203698));
#51830=CARTESIAN_POINT('Ctrl Pts',(-3.26677653888676,-1.,1.89255393500965));
#51831=CARTESIAN_POINT('Ctrl Pts',(-3.27407108933139,-1.,1.89589172903793));
#51832=CARTESIAN_POINT('Ctrl Pts',(-3.28154737912352,-1.,1.89918429230462));
#51833=CARTESIAN_POINT('Ctrl Pts',(-3.2889344860029,-1.,1.90228971247527));
#51834=CARTESIAN_POINT('Ctrl Pts',(-3.29608978722113,-1.,1.90513891864087));
#51835=CARTESIAN_POINT('Ctrl Pts',(-3.30300595568195,-1.,1.90773912171341));
#51836=CARTESIAN_POINT('Ctrl Pts',(-3.30975721158596,-1.,1.91014297830446));
#51837=CARTESIAN_POINT('Ctrl Pts',(-3.31646052426364,-1.,1.91242616234442));
#51838=CARTESIAN_POINT('Ctrl Pts',(-3.32323403454535,-1.,1.91466343916628));
#51839=CARTESIAN_POINT('Ctrl Pts',(-3.33014884257873,-1.,1.91690081930331));
#51840=CARTESIAN_POINT('Ctrl Pts',(-3.33721230710012,-1.,1.9191460961021));
#51841=CARTESIAN_POINT('Ctrl Pts',(-3.34439448941961,-1.,1.92138450828404));
#51842=CARTESIAN_POINT('Ctrl Pts',(-3.35164424847223,-1.,1.92358838440528));
#51843=CARTESIAN_POINT('Ctrl Pts',(-3.35890824422965,-1.,1.92572846125756));
#51844=CARTESIAN_POINT('Ctrl Pts',(-3.36615168657567,-1.,1.92778626543786));
#51845=CARTESIAN_POINT('Ctrl Pts',(-3.37336807068043,-1.,1.92975993109877));
#51846=CARTESIAN_POINT('Ctrl Pts',(-3.3805676852555,-1.,1.93165739093276));
#51847=CARTESIAN_POINT('Ctrl Pts',(-3.38777076883256,-1.,1.93349233176788));
#51848=CARTESIAN_POINT('Ctrl Pts',(-3.39499923640795,-1.,1.93527929945985));
#51849=CARTESIAN_POINT('Ctrl Pts',(-3.40226802104109,-1.,1.93702857723098));
#51850=CARTESIAN_POINT('Ctrl Pts',(-3.40957978266642,-1.,1.93874306008143));
#51851=CARTESIAN_POINT('Ctrl Pts',(-3.41692971994096,-1.,1.94042111965246));
#51852=CARTESIAN_POINT('Ctrl Pts',(-3.42430850941503,-1.,1.94205835913696));
#51853=CARTESIAN_POINT('Ctrl Pts',(-3.43170586602434,-1.,1.94364973660284));
#51854=CARTESIAN_POINT('Ctrl Pts',(-3.43911410197687,-1.,1.94519168842879));
#51855=CARTESIAN_POINT('Ctrl Pts',(-3.44653088665681,-1.,1.94668377715329));
#51856=CARTESIAN_POINT('Ctrl Pts',(-3.45395731584051,-1.,1.94812754766524));
#51857=CARTESIAN_POINT('Ctrl Pts',(-3.46139661060962,-1.,1.94952575850197));
#51858=CARTESIAN_POINT('Ctrl Pts',(-3.46885258974191,-1.,1.95088147859876));
#51859=CARTESIAN_POINT('Ctrl Pts',(-3.47632820495921,-1.,1.95219722189876));
#51860=CARTESIAN_POINT('Ctrl Pts',(-3.48382414832634,-1.,1.95347412486308));
#51861=CARTESIAN_POINT('Ctrl Pts',(-3.49133956289133,-1.,1.95471236969643));
#51862=CARTESIAN_POINT('Ctrl Pts',(-3.49887263575583,-1.,1.95591153823661));
#51863=CARTESIAN_POINT('Ctrl Pts',(-3.50642124159909,-1.,1.95707099606511));
#51864=CARTESIAN_POINT('Ctrl Pts',(-3.51398354617794,-1.,1.95819025316779));
#51865=CARTESIAN_POINT('Ctrl Pts',(-3.52155867431486,-1.,1.95926936324461));
#51866=CARTESIAN_POINT('Ctrl Pts',(-3.52914648844351,-1.,1.96030879411566));
#51867=CARTESIAN_POINT('Ctrl Pts',(-3.53674730625813,-1.,1.96130926212689));
#51868=CARTESIAN_POINT('Ctrl Pts',(-3.54436163300443,-1.,1.96227157573067));
#51869=CARTESIAN_POINT('Ctrl Pts',(-3.55198990600886,-1.,1.96319648628644));
#51870=CARTESIAN_POINT('Ctrl Pts',(-3.55963218706096,-1.,1.96408450906812));
#51871=CARTESIAN_POINT('Ctrl Pts',(-3.56728820357791,-1.,1.96493594634567));
#51872=CARTESIAN_POINT('Ctrl Pts',(-3.57495748600959,-1.,1.96575096652789));
#51873=CARTESIAN_POINT('Ctrl Pts',(-3.58263947663829,-1.,1.96652966688911));
#51874=CARTESIAN_POINT('Ctrl Pts',(-3.59033364022801,-1.,1.96727213799544));
#51875=CARTESIAN_POINT('Ctrl Pts',(-3.59803959819938,-1.,1.96797854118369));
#51876=CARTESIAN_POINT('Ctrl Pts',(-3.60575714017989,-1.,1.9686491188594));
#51877=CARTESIAN_POINT('Ctrl Pts',(-3.61348615496704,-1.,1.96928416040877));
#51878=CARTESIAN_POINT('Ctrl Pts',(-3.62122658401893,-1.,1.96988398129978));
#51879=CARTESIAN_POINT('Ctrl Pts',(-3.62897836973293,-1.,1.97044889850463));
#51880=CARTESIAN_POINT('Ctrl Pts',(-3.63674139590412,-1.,1.97097920454464));
#51881=CARTESIAN_POINT('Ctrl Pts',(-3.64451546723514,-1.,1.97147515441164));
#51882=CARTESIAN_POINT('Ctrl Pts',(-3.652300347166,-1.,1.9719369724024));
#51883=CARTESIAN_POINT('Ctrl Pts',(-3.6600957816636,-1.,1.9723648543905));
#51884=CARTESIAN_POINT('Ctrl Pts',(-3.66790152752075,-1.,1.97275897198678));
#51885=CARTESIAN_POINT('Ctrl Pts',(-3.67571738107084,-1.,1.97311947678516));
#51886=CARTESIAN_POINT('Ctrl Pts',(-3.68354319915092,-1.,1.97344650304519));
#51887=CARTESIAN_POINT('Ctrl Pts',(-3.69137888599902,-1.,1.97374016225483));
#51888=CARTESIAN_POINT('Ctrl Pts',(-3.6976552856004,-1.,1.97394846383216));
#51889=CARTESIAN_POINT('Ctrl Pts',(-3.70236698912904,-1.,1.97408973726715));
#51890=CARTESIAN_POINT('Ctrl Pts',(-3.70551008132332,-1.,1.97417727645308));
#51891=CARTESIAN_POINT('Ctrl Pts',(-3.70708211654725,-1.,1.97421938526992));
#51892=CARTESIAN_POINT('',(-3.77614523045147,-1.,1.8386753923786));
#51893=CARTESIAN_POINT('',(-3.70708211654725,-1.,1.97421938526992));
#51894=CARTESIAN_POINT('',(-3.42859860294306,-1.,1.5189508286633));
#51895=CARTESIAN_POINT('Ctrl Pts',(-3.77614523045147,-1.,1.8386753923786));
#51896=CARTESIAN_POINT('Ctrl Pts',(-3.77518714457833,-1.,1.83742834010626));
#51897=CARTESIAN_POINT('Ctrl Pts',(-3.77326886064398,-1.,1.83493697934534));
#51898=CARTESIAN_POINT('Ctrl Pts',(-3.77038509817999,-1.,1.83120816955645));
#51899=CARTESIAN_POINT('Ctrl Pts',(-3.76652740353775,-1.,1.82625289220915));
#51900=CARTESIAN_POINT('Ctrl Pts',(-3.76168412707948,-1.,1.82008629694091));
#51901=CARTESIAN_POINT('Ctrl Pts',(-3.75681965683071,-1.,1.8139472983358));
#51902=CARTESIAN_POINT('Ctrl Pts',(-3.75193395887977,-1.,1.80783603939617));
#51903=CARTESIAN_POINT('Ctrl Pts',(-3.74702700875467,-1.,1.8017527148577));
#51904=CARTESIAN_POINT('Ctrl Pts',(-3.74209880352445,-1.,1.79569757859422));
#51905=CARTESIAN_POINT('Ctrl Pts',(-3.73714934730681,-1.,1.78967092823491));
#51906=CARTESIAN_POINT('Ctrl Pts',(-3.7321786309547,-1.,1.78367308442901));
#51907=CARTESIAN_POINT('Ctrl Pts',(-3.72718661205609,-1.,1.77770437039658));
#51908=CARTESIAN_POINT('Ctrl Pts',(-3.72217319911254,-1.,1.77176509401761));
#51909=CARTESIAN_POINT('Ctrl Pts',(-3.71713822377359,-1.,1.76585552124394));
#51910=CARTESIAN_POINT('Ctrl Pts',(-3.71208146346136,-1.,1.75997588498865));
#51911=CARTESIAN_POINT('Ctrl Pts',(-3.70700269736659,-1.,1.75412641804042));
#51912=CARTESIAN_POINT('Ctrl Pts',(-3.7019017567335,-1.,1.74830738046057));
#51913=CARTESIAN_POINT('Ctrl Pts',(-3.69677856910517,-1.,1.74251908492617));
#51914=CARTESIAN_POINT('Ctrl Pts',(-3.69163322648036,-1.,1.73676193254557));
#51915=CARTESIAN_POINT('Ctrl Pts',(-3.68646597019332,-1.,1.73103640956717));
#51916=CARTESIAN_POINT('Ctrl Pts',(-3.68127704936579,-1.,1.72534302437056));
#51917=CARTESIAN_POINT('Ctrl Pts',(-3.67606660374709,-1.,1.71968225581808));
#51918=CARTESIAN_POINT('Ctrl Pts',(-3.67083454901611,-1.,1.71405450210383));
#51919=CARTESIAN_POINT('Ctrl Pts',(-3.66558043198876,-1.,1.70846001610956));
#51920=CARTESIAN_POINT('Ctrl Pts',(-3.66030338774847,-1.,1.70289888566873));
#51921=CARTESIAN_POINT('Ctrl Pts',(-3.65500246526749,-1.,1.69737117722534));
#51922=CARTESIAN_POINT('Ctrl Pts',(-3.64967689827371,-1.,1.69187705481689));
#51923=CARTESIAN_POINT('Ctrl Pts',(-3.64432638915203,-1.,1.68641690471457));
#51924=CARTESIAN_POINT('Ctrl Pts',(-3.63895140887462,-1.,1.68099146651586));
#51925=CARTESIAN_POINT('Ctrl Pts',(-3.63355343201232,-1.,1.67560193613156));
#51926=CARTESIAN_POINT('Ctrl Pts',(-3.62813422105271,-1.,1.67024966008045));
#51927=CARTESIAN_POINT('Ctrl Pts',(-3.62269517989109,-1.,1.66493585923855));
#51928=CARTESIAN_POINT('Ctrl Pts',(-3.61723666482456,-1.,1.65966133399186));
#51929=CARTESIAN_POINT('Ctrl Pts',(-3.61175734965127,-1.,1.65442619244325));
#51930=CARTESIAN_POINT('Ctrl Pts',(-3.60625346556992,-1.,1.64922952425832));
#51931=CARTESIAN_POINT('Ctrl Pts',(-3.60072028513845,-1.,1.64407004385582));
#51932=CARTESIAN_POINT('Ctrl Pts',(-3.59515368334893,-1.,1.63894676675352));
#51933=CARTESIAN_POINT('Ctrl Pts',(-3.58955176627879,-1.,1.6338597145126));
#51934=CARTESIAN_POINT('Ctrl Pts',(-3.58391625774343,-1.,1.62881051550745));
#51935=CARTESIAN_POINT('Ctrl Pts',(-3.5782545595439,-1.,1.62380329464844));
#51936=CARTESIAN_POINT('Ctrl Pts',(-3.57257679609806,-1.,1.61884340915404));
#51937=CARTESIAN_POINT('Ctrl Pts',(-3.56689200468387,-1.,1.61393581747514));
#51938=CARTESIAN_POINT('Ctrl Pts',(-3.5612043248298,-1.,1.60908344685457));
#51939=CARTESIAN_POINT('Ctrl Pts',(-3.55550985096129,-1.,1.60428584699853));
#51940=CARTESIAN_POINT('Ctrl Pts',(-3.54979148634454,-1.,1.59953698113457));
#51941=CARTESIAN_POINT('Ctrl Pts',(-3.54402458182337,-1.,1.59482766949766));
#51942=CARTESIAN_POINT('Ctrl Pts',(-3.53818616861077,-1.,1.59014958368739));
#51943=CARTESIAN_POINT('Ctrl Pts',(-3.5322637814708,-1.,1.58549906268088));
#51944=CARTESIAN_POINT('Ctrl Pts',(-3.52626275334881,-1.,1.58088027227848));
#51945=CARTESIAN_POINT('Ctrl Pts',(-3.52021847865912,-1.,1.57631049988158));
#51946=CARTESIAN_POINT('Ctrl Pts',(-3.51418598431665,-1.,1.57181569799743));
#51947=CARTESIAN_POINT('Ctrl Pts',(-3.50821771695363,-1.,1.56742097575012));
#51948=CARTESIAN_POINT('Ctrl Pts',(-3.50234321621578,-1.,1.56314187758675));
#51949=CARTESIAN_POINT('Ctrl Pts',(-3.49655185179655,-1.,1.55897703097874));
#51950=CARTESIAN_POINT('Ctrl Pts',(-3.4907646087742,-1.,1.55489595901116));
#51951=CARTESIAN_POINT('Ctrl Pts',(-3.48485155928567,-1.,1.55084702970452));
#51952=CARTESIAN_POINT('Ctrl Pts',(-3.47868272898751,-1.,1.54678009290276));
#51953=CARTESIAN_POINT('Ctrl Pts',(-3.47217189224653,-1.,1.54266605398187));
#51954=CARTESIAN_POINT('Ctrl Pts',(-3.46531752207153,-1.,1.53851507915502));
#51955=CARTESIAN_POINT('Ctrl Pts',(-3.45825932955032,-1.,1.53440195378792));
#51956=CARTESIAN_POINT('Ctrl Pts',(-3.45127136828305,-1.,1.53046244461635));
#51957=CARTESIAN_POINT('Ctrl Pts',(-3.44469547526647,-1.,1.52686242875556));
#51958=CARTESIAN_POINT('Ctrl Pts',(-3.4388889597401,-1.,1.5237734895035));
#51959=CARTESIAN_POINT('Ctrl Pts',(-3.43417156977893,-1.,1.52134826724292));
#51960=CARTESIAN_POINT('Ctrl Pts',(-3.43101631893414,-1.,1.5198144909338));
#51961=CARTESIAN_POINT('Ctrl Pts',(-3.42946838852587,-1.,1.51914806898491));
#51962=CARTESIAN_POINT('Ctrl Pts',(-3.42884302333841,-1.,1.5189513329503));
#51963=CARTESIAN_POINT('Ctrl Pts',(-3.42864616361875,-1.,1.51893924967331));
#51964=CARTESIAN_POINT('Ctrl Pts',(-3.42859860294306,-1.,1.5189508286633));
#51965=CARTESIAN_POINT('',(-3.49844575334386,-1.,1.35032489087269));
#51966=CARTESIAN_POINT('Origin',(0.,-1.,0.));
#51967=CARTESIAN_POINT('',(-3.97027773754922,-1.,1.36999806084572));
#51968=CARTESIAN_POINT('Ctrl Pts',(-3.49844575334386,-1.,1.35032489087269));
#51969=CARTESIAN_POINT('Ctrl Pts',(-3.49847119623841,-1.,1.35036670893102));
#51970=CARTESIAN_POINT('Ctrl Pts',(-3.49861894124915,-1.,1.35049736560633));
#51971=CARTESIAN_POINT('Ctrl Pts',(-3.49920025459856,-1.,1.35080045218652));
#51972=CARTESIAN_POINT('Ctrl Pts',(-3.5007660381658,-1.,1.35142377279535));
#51973=CARTESIAN_POINT('Ctrl Pts',(-3.50408168106113,-1.,1.3525703284343));
#51974=CARTESIAN_POINT('Ctrl Pts',(-3.50913227060177,-1.,1.35419113576022));
#51975=CARTESIAN_POINT('Ctrl Pts',(-3.51542230699919,-1.,1.35611275237288));
#51976=CARTESIAN_POINT('Ctrl Pts',(-3.52261776117121,-1.,1.35821701528975));
#51977=CARTESIAN_POINT('Ctrl Pts',(-3.53034464961849,-1.,1.36037259643827));
#51978=CARTESIAN_POINT('Ctrl Pts',(-3.53824396425032,-1.,1.36245507339334));
#51979=CARTESIAN_POINT('Ctrl Pts',(-3.54602591832893,-1.,1.36436666257567));
#51980=CARTESIAN_POINT('Ctrl Pts',(-3.55353883995793,-1.,1.36606145456711));
#51981=CARTESIAN_POINT('Ctrl Pts',(-3.56077662028492,-1.,1.36754771771174));
#51982=CARTESIAN_POINT('Ctrl Pts',(-3.56782080304554,-1.,1.36886584973349));
#51983=CARTESIAN_POINT('Ctrl Pts',(-3.57479875549453,-1.,1.37007229485646));
#51984=CARTESIAN_POINT('Ctrl Pts',(-3.58183885982745,-1.,1.37122241663073));
#51985=CARTESIAN_POINT('Ctrl Pts',(-3.5890185384643,-1.,1.37235053661));
#51986=CARTESIAN_POINT('Ctrl Pts',(-3.59634627869117,-1.,1.37346320103184));
#51987=CARTESIAN_POINT('Ctrl Pts',(-3.60379020124038,-1.,1.37455051379642));
#51988=CARTESIAN_POINT('Ctrl Pts',(-3.61129546591082,-1.,1.37559314436641));
#51989=CARTESIAN_POINT('Ctrl Pts',(-3.61880481160408,-1.,1.37657053403102));
#51990=CARTESIAN_POINT('Ctrl Pts',(-3.62628098665112,-1.,1.37746987919868));
#51991=CARTESIAN_POINT('Ctrl Pts',(-3.63371727442448,-1.,1.37829035457324));
#51992=CARTESIAN_POINT('Ctrl Pts',(-3.64112507791112,-1.,1.37903818567347));
#51993=CARTESIAN_POINT('Ctrl Pts',(-3.64852652756444,-1.,1.37972372481598));
#51994=CARTESIAN_POINT('Ctrl Pts',(-3.65594554404396,-1.,1.38035791051215));
#51995=CARTESIAN_POINT('Ctrl Pts',(-3.66339848520874,-1.,1.38094856333558));
#51996=CARTESIAN_POINT('Ctrl Pts',(-3.67088843112282,-1.,1.38149812653876));
#51997=CARTESIAN_POINT('Ctrl Pts',(-3.6784103848243,-1.,1.38200574290626));
#51998=CARTESIAN_POINT('Ctrl Pts',(-3.68595444983844,-1.,1.38246852827185));
#51999=CARTESIAN_POINT('Ctrl Pts',(-3.69350967899523,-1.,1.38288311171649));
#52000=CARTESIAN_POINT('Ctrl Pts',(-3.70106792167894,-1.,1.38324717612862));
#52001=CARTESIAN_POINT('Ctrl Pts',(-3.70862680753343,-1.,1.38356065402122));
#52002=CARTESIAN_POINT('Ctrl Pts',(-3.7161876605181,-1.,1.38382489984585));
#52003=CARTESIAN_POINT('Ctrl Pts',(-3.72375409358805,-1.,1.3840421342895));
#52004=CARTESIAN_POINT('Ctrl Pts',(-3.73133035859283,-1.,1.38421479111531));
#52005=CARTESIAN_POINT('Ctrl Pts',(-3.73891976418099,-1.,1.38434489156456));
#52006=CARTESIAN_POINT('Ctrl Pts',(-3.7465231716786,-1.,1.38443344984389));
#52007=CARTESIAN_POINT('Ctrl Pts',(-3.75413976318727,-1.,1.38448077997155));
#52008=CARTESIAN_POINT('Ctrl Pts',(-3.76176768271347,-1.,1.38448675253343));
#52009=CARTESIAN_POINT('Ctrl Pts',(-3.76940473185775,-1.,1.38445107339517));
#52010=CARTESIAN_POINT('Ctrl Pts',(-3.77704902230441,-1.,1.38437354551435));
#52011=CARTESIAN_POINT('Ctrl Pts',(-3.78469969805134,-1.,1.38425435883773));
#52012=CARTESIAN_POINT('Ctrl Pts',(-3.79235669640907,-1.,1.38409399694588));
#52013=CARTESIAN_POINT('Ctrl Pts',(-3.80002044322169,-1.,1.38389311766701));
#52014=CARTESIAN_POINT('Ctrl Pts',(-3.80769156398429,-1.,1.38365244046226));
#52015=CARTESIAN_POINT('Ctrl Pts',(-3.81537060817765,-1.,1.38337263902766));
#52016=CARTESIAN_POINT('Ctrl Pts',(-3.82305771743715,-1.,1.38305421262724));
#52017=CARTESIAN_POINT('Ctrl Pts',(-3.83075266982138,-1.,1.38269750245086));
#52018=CARTESIAN_POINT('Ctrl Pts',(-3.83845502790609,-1.,1.38230274828774));
#52019=CARTESIAN_POINT('Ctrl Pts',(-3.84616425605705,-1.,1.38187013346089));
#52020=CARTESIAN_POINT('Ctrl Pts',(-3.85387983979557,-1.,1.38139983115075));
#52021=CARTESIAN_POINT('Ctrl Pts',(-3.86160143044187,-1.,1.38089205993067));
#52022=CARTESIAN_POINT('Ctrl Pts',(-3.86932885813403,-1.,1.38034709213129));
#52023=CARTESIAN_POINT('Ctrl Pts',(-3.87706205830865,-1.,1.37976523097187));
#52024=CARTESIAN_POINT('Ctrl Pts',(-3.88480102249461,-1.,1.37914679719446));
#52025=CARTESIAN_POINT('Ctrl Pts',(-3.89254574338385,-1.,1.37849211287981));
#52026=CARTESIAN_POINT('Ctrl Pts',(-3.90029615196255,-1.,1.3778014851263));
#52027=CARTESIAN_POINT('Ctrl Pts',(-3.90805209522729,-1.,1.3770751963376));
#52028=CARTESIAN_POINT('Ctrl Pts',(-3.91581337461825,-1.,1.37631350505516));
#52029=CARTESIAN_POINT('Ctrl Pts',(-3.92357976987132,-1.,1.37551664448057));
#52030=CARTESIAN_POINT('Ctrl Pts',(-3.93135106761941,-1.,1.37468482215784));
#52031=CARTESIAN_POINT('Ctrl Pts',(-3.93912709041791,-1.,1.37381821967499));
#52032=CARTESIAN_POINT('Ctrl Pts',(-3.94690771786926,-1.,1.37291699203423));
#52033=CARTESIAN_POINT('Ctrl Pts',(-3.95469287283105,-1.,1.37198126433139));
#52034=CARTESIAN_POINT('Ctrl Pts',(-3.96092458508407,-1.,1.37120515615663));
#52035=CARTESIAN_POINT('Ctrl Pts',(-3.96560037975788,-1.,1.37060761746027));
#52036=CARTESIAN_POINT('Ctrl Pts',(-3.9687184694173,-1.,1.37020239094758));
#52037=CARTESIAN_POINT('Ctrl Pts',(-3.97027773754922,-1.,1.36999806084572));
#52038=CARTESIAN_POINT('',(-4.01728681790024,-1.,1.22531898815164));
#52039=CARTESIAN_POINT('',(-3.97027773754922,-1.,1.36999806084572));
#52040=CARTESIAN_POINT('',(-3.62400312501199,-1.,0.963899035118985));
#52041=CARTESIAN_POINT('Ctrl Pts',(-4.01728681790024,-1.,1.22531898815164));
#52042=CARTESIAN_POINT('Ctrl Pts',(-4.01614544569895,-1.,1.22423716681317));
#52043=CARTESIAN_POINT('Ctrl Pts',(-4.01386104433519,-1.,1.22207656455845));
#52044=CARTESIAN_POINT('Ctrl Pts',(-4.01042947140789,-1.,1.21884478244403));
#52045=CARTESIAN_POINT('Ctrl Pts',(-4.00584409522722,-1.,1.21455398918133));
#52046=CARTESIAN_POINT('Ctrl Pts',(-4.00009577950721,-1.,1.20922097029551));
#52047=CARTESIAN_POINT('Ctrl Pts',(-3.99433084799666,-1.,1.20391852375139));
#52048=CARTESIAN_POINT('Ctrl Pts',(-3.98854928957189,-1.,1.19864679609566));
#52049=CARTESIAN_POINT('Ctrl Pts',(-3.98275111052561,-1.,1.19340598349475));
#52050=CARTESIAN_POINT('Ctrl Pts',(-3.97693634767754,-1.,1.18819633715539));
#52051=CARTESIAN_POINT('Ctrl Pts',(-3.97110505165415,-1.,1.18301815039831));
#52052=CARTESIAN_POINT('Ctrl Pts',(-3.96525726358159,-1.,1.17787174135592));
#52053=CARTESIAN_POINT('Ctrl Pts',(-3.95939299213276,-1.,1.17275743590361));
#52054=CARTESIAN_POINT('Ctrl Pts',(-3.95351219509876,-1.,1.16767555244438));
#52055=CARTESIAN_POINT('Ctrl Pts',(-3.94761474780583,-1.,1.16262637999157));
#52056=CARTESIAN_POINT('Ctrl Pts',(-3.94170046685203,-1.,1.15761018340956));
#52057=CARTESIAN_POINT('Ctrl Pts',(-3.9357691705628,-1.,1.1526272271632));
#52058=CARTESIAN_POINT('Ctrl Pts',(-3.92982073294257,-1.,1.14767779451123));
#52059=CARTESIAN_POINT('Ctrl Pts',(-3.92385513133997,-1.,1.14276220561593));
#52060=CARTESIAN_POINT('Ctrl Pts',(-3.91787251936827,-1.,1.13788084225554));
#52061=CARTESIAN_POINT('Ctrl Pts',(-3.91187321145649,-1.,1.13303414693896));
#52062=CARTESIAN_POINT('Ctrl Pts',(-3.90585753318737,-1.,1.12822258281553));
#52063=CARTESIAN_POINT('Ctrl Pts',(-3.89982569750025,-1.,1.12344660099043));
#52064=CARTESIAN_POINT('Ctrl Pts',(-3.89377768340344,-1.,1.11870660794603));
#52065=CARTESIAN_POINT('Ctrl Pts',(-3.88771308285171,-1.,1.11400292434429));
#52066=CARTESIAN_POINT('Ctrl Pts',(-3.88163105531724,-1.,1.10933577224008));
#52067=CARTESIAN_POINT('Ctrl Pts',(-3.87553067187514,-1.,1.10470536603287));
#52068=CARTESIAN_POINT('Ctrl Pts',(-3.86941120134849,-1.,1.10011198761195));
#52069=CARTESIAN_POINT('Ctrl Pts',(-3.86327241021247,-1.,1.09555606505013));
#52070=CARTESIAN_POINT('Ctrl Pts',(-3.85711487933931,-1.,1.09103825516294));
#52071=CARTESIAN_POINT('Ctrl Pts',(-3.85094025222713,-1.,1.08655950846384));
#52072=CARTESIAN_POINT('Ctrl Pts',(-3.8447504803063,-1.,1.08212087917991));
#52073=CARTESIAN_POINT('Ctrl Pts',(-3.83854714117491,-1.,1.07772335353858));
#52074=CARTESIAN_POINT('Ctrl Pts',(-3.83233071195144,-1.,1.07336766633459));
#52075=CARTESIAN_POINT('Ctrl Pts',(-3.82609989967276,-1.,1.06905413180359));
#52076=CARTESIAN_POINT('Ctrl Pts',(-3.81985083953012,-1.,1.0647824403893));
#52077=CARTESIAN_POINT('Ctrl Pts',(-3.8135786611749,-1.,1.06055206187299));
#52078=CARTESIAN_POINT('Ctrl Pts',(-3.80727913637791,-1.,1.05636266918644));
#52079=CARTESIAN_POINT('Ctrl Pts',(-3.80095039790681,-1.,1.05221457990016));
#52080=CARTESIAN_POINT('Ctrl Pts',(-3.79459440308786,-1.,1.04810913267639));
#52081=CARTESIAN_POINT('Ctrl Pts',(-3.78821910787179,-1.,1.04404924374422));
#52082=CARTESIAN_POINT('Ctrl Pts',(-3.7818353500817,-1.,1.04003862055798));
#52083=CARTESIAN_POINT('Ctrl Pts',(-3.77545283140427,-1.,1.03608074678008));
#52084=CARTESIAN_POINT('Ctrl Pts',(-3.76907609832516,-1.,1.03217786604919));
#52085=CARTESIAN_POINT('Ctrl Pts',(-3.76270122291245,-1.,1.02833014458184));
#52086=CARTESIAN_POINT('Ctrl Pts',(-3.75631037456224,-1.,1.02453429444668));
#52087=CARTESIAN_POINT('Ctrl Pts',(-3.74987777155873,-1.,1.02078510487439));
#52088=CARTESIAN_POINT('Ctrl Pts',(-3.74337942504993,-1.,1.01707794311088));
#52089=CARTESIAN_POINT('Ctrl Pts',(-3.73680245055747,-1.,1.01341114319906));
#52090=CARTESIAN_POINT('Ctrl Pts',(-3.73015276704407,-1.,1.00978798539491));
#52091=CARTESIAN_POINT('Ctrl Pts',(-3.72346803750544,-1.,1.00622000735696));
#52092=CARTESIAN_POINT('Ctrl Pts',(-3.71680667125047,-1.,1.00272423396802));
#52093=CARTESIAN_POINT('Ctrl Pts',(-3.7102243971387,-1.,0.999317260756344));
#52094=CARTESIAN_POINT('Ctrl Pts',(-3.70375282282107,-1.,0.996009819772431));
#52095=CARTESIAN_POINT('Ctrl Pts',(-3.69738123415696,-1.,0.992802218332103));
#52096=CARTESIAN_POINT('Ctrl Pts',(-3.69102682138955,-1.,0.989676715398858));
#52097=CARTESIAN_POINT('Ctrl Pts',(-3.6845531792623,-1.,0.986602639864285));
#52098=CARTESIAN_POINT('Ctrl Pts',(-3.67782408841876,-1.,0.983550791470864));
#52099=CARTESIAN_POINT('Ctrl Pts',(-3.67074983340444,-1.,0.980505922458494));
#52100=CARTESIAN_POINT('Ctrl Pts',(-3.66333049637403,-1.,0.977478312751416));
#52101=CARTESIAN_POINT('Ctrl Pts',(-3.6557157673487,-1.,0.974519971354138));
#52102=CARTESIAN_POINT('Ctrl Pts',(-3.64819756447072,-1.,0.971722122060277));
#52103=CARTESIAN_POINT('Ctrl Pts',(-3.64113946505393,-1.,0.969195124674829));
#52104=CARTESIAN_POINT('Ctrl Pts',(-3.6349212208096,-1.,0.967052554540877));
#52105=CARTESIAN_POINT('Ctrl Pts',(-3.62988252139998,-1.,0.965395153165716));
#52106=CARTESIAN_POINT('Ctrl Pts',(-3.62652618145252,-1.,0.964373850166081));
#52107=CARTESIAN_POINT('Ctrl Pts',(-3.62489305727516,-1.,0.963957782642589));
#52108=CARTESIAN_POINT('Ctrl Pts',(-3.62424461507455,-1.,0.963861297423579));
#52109=CARTESIAN_POINT('Ctrl Pts',(-3.62404828878375,-1.,0.963880158556713));
#52110=CARTESIAN_POINT('Ctrl Pts',(-3.62400312501199,-1.,0.963899035118985));
#52111=CARTESIAN_POINT('',(-3.66661143271648,-1.,0.786422660833743));
#52112=CARTESIAN_POINT('Origin',(0.,-1.,0.));
#52113=CARTESIAN_POINT('',(-4.13571194405636,-1.,0.732042837400619));
#52114=CARTESIAN_POINT('Ctrl Pts',(-3.66661143271648,-1.,0.786422660833743));
#52115=CARTESIAN_POINT('Ctrl Pts',(-3.66664310415236,-1.,0.786459983896781));
#52116=CARTESIAN_POINT('Ctrl Pts',(-3.66680946938396,-1.,0.78656591955989));
#52117=CARTESIAN_POINT('Ctrl Pts',(-3.66743103898844,-1.,0.786774337198499));
#52118=CARTESIAN_POINT('Ctrl Pts',(-3.66907505398769,-1.,0.787145041181588));
#52119=CARTESIAN_POINT('Ctrl Pts',(-3.672529236635,-1.,0.787758799995426));
#52120=CARTESIAN_POINT('Ctrl Pts',(-3.67777119516438,-1.,0.788569566220662));
#52121=CARTESIAN_POINT('Ctrl Pts',(-3.68428439784285,-1.,0.789483546065158));
#52122=CARTESIAN_POINT('Ctrl Pts',(-3.69172044327754,-1.,0.79043628498958));
#52123=CARTESIAN_POINT('Ctrl Pts',(-3.69968940808982,-1.,0.791356575696509));
#52124=CARTESIAN_POINT('Ctrl Pts',(-3.70781724021879,-1.,0.792177688845967));
#52125=CARTESIAN_POINT('Ctrl Pts',(-3.7158024239604,-1.,0.792848377370115));
#52126=CARTESIAN_POINT('Ctrl Pts',(-3.7234879729357,-1.,0.79334702378387));
#52127=CARTESIAN_POINT('Ctrl Pts',(-3.7308691469564,-1.,0.793682750269347));
#52128=CARTESIAN_POINT('Ctrl Pts',(-3.73803280541576,-1.,0.79388270093679));
#52129=CARTESIAN_POINT('Ctrl Pts',(-3.74511357728827,-1.,0.79398270045988));
#52130=CARTESIAN_POINT('Ctrl Pts',(-3.75224692493895,-1.,0.79401734737144));
#52131=CARTESIAN_POINT('Ctrl Pts',(-3.75951468666325,-1.,0.794008429135047));
#52132=CARTESIAN_POINT('Ctrl Pts',(-3.76692626931184,-1.,0.793961083689141));
#52133=CARTESIAN_POINT('Ctrl Pts',(-3.77444863801264,-1.,0.793870523787515));
#52134=CARTESIAN_POINT('Ctrl Pts',(-3.78202460377617,-1.,0.793726235781339));
#52135=CARTESIAN_POINT('Ctrl Pts',(-3.78959439439222,-1.,0.793516871680966));
#52136=CARTESIAN_POINT('Ctrl Pts',(-3.79711921389862,-1.,0.7932356129732));
#52137=CARTESIAN_POINT('Ctrl Pts',(-3.80459229925598,-1.,0.792882695234693));
#52138=CARTESIAN_POINT('Ctrl Pts',(-3.81202588694726,-1.,0.792462483517568));
#52139=CARTESIAN_POINT('Ctrl Pts',(-3.81944345442237,-1.,0.791981740718606));
#52140=CARTESIAN_POINT('Ctrl Pts',(-3.82687033899799,-1.,0.791447528662381));
#52141=CARTESIAN_POINT('Ctrl Pts',(-3.83432392054804,-1.,0.79086501270534));
#52142=CARTESIAN_POINT('Ctrl Pts',(-3.84180762342476,-1.,0.790236124191289));
#52143=CARTESIAN_POINT('Ctrl Pts',(-3.8493163780891,-1.,0.789560798155618));
#52144=CARTESIAN_POINT('Ctrl Pts',(-3.85683995872536,-1.,0.788837734090688));
#52145=CARTESIAN_POINT('Ctrl Pts',(-3.86436702561342,-1.,0.788065315093771));
#52146=CARTESIAN_POINT('Ctrl Pts',(-3.87188916600905,-1.,0.78724252761798));
#52147=CARTESIAN_POINT('Ctrl Pts',(-3.87940402818186,-1.,0.786369675812592));
#52148=CARTESIAN_POINT('Ctrl Pts',(-3.88691313167399,-1.,0.785447890340723));
#52149=CARTESIAN_POINT('Ctrl Pts',(-3.89442039235105,-1.,0.784478799358335));
#52150=CARTESIAN_POINT('Ctrl Pts',(-3.90193039043971,-1.,0.783464141529082));
#52151=CARTESIAN_POINT('Ctrl Pts',(-3.90944671004536,-1.,0.782405395622758));
#52152=CARTESIAN_POINT('Ctrl Pts',(-3.9169703605466,-1.,0.781303428618343));
#52153=CARTESIAN_POINT('Ctrl Pts',(-3.92450058323799,-1.,0.780158678615506));
#52154=CARTESIAN_POINT('Ctrl Pts',(-3.93203552473153,-1.,0.778971308134786));
#52155=CARTESIAN_POINT('Ctrl Pts',(-3.93957296768098,-1.,0.777741370568549));
#52156=CARTESIAN_POINT('Ctrl Pts',(-3.94711101619471,-1.,0.77646896669796));
#52157=CARTESIAN_POINT('Ctrl Pts',(-3.95464885452364,-1.,0.775154418039441));
#52158=CARTESIAN_POINT('Ctrl Pts',(-3.96218649639876,-1.,0.773798212026682));
#52159=CARTESIAN_POINT('Ctrl Pts',(-3.96972446532832,-1.,0.772400931772238));
#52160=CARTESIAN_POINT('Ctrl Pts',(-3.97726349165507,-1.,0.770963190030503));
#52161=CARTESIAN_POINT('Ctrl Pts',(-3.98480422348403,-1.,0.769485566245459));
#52162=CARTESIAN_POINT('Ctrl Pts',(-3.99234687880892,-1.,0.767968531377708));
#52163=CARTESIAN_POINT('Ctrl Pts',(-3.99989129179464,-1.,0.766412457135785));
#52164=CARTESIAN_POINT('Ctrl Pts',(-4.00743706791366,-1.,0.764817648784946));
#52165=CARTESIAN_POINT('Ctrl Pts',(-4.01498370680434,-1.,0.763184371182826));
#52166=CARTESIAN_POINT('Ctrl Pts',(-4.02253072741347,-1.,0.761512875859941));
#52167=CARTESIAN_POINT('Ctrl Pts',(-4.0300778195465,-1.,0.759803433244166));
#52168=CARTESIAN_POINT('Ctrl Pts',(-4.03762485803468,-1.,0.758056338885553));
#52169=CARTESIAN_POINT('Ctrl Pts',(-4.04517182654344,-1.,0.756271902370186));
#52170=CARTESIAN_POINT('Ctrl Pts',(-4.05271876688106,-1.,0.754450441816411));
#52171=CARTESIAN_POINT('Ctrl Pts',(-4.06026572221399,-1.,0.752592276482869));
#52172=CARTESIAN_POINT('Ctrl Pts',(-4.06781267241886,-1.,0.750697720483175));
#52173=CARTESIAN_POINT('Ctrl Pts',(-4.07535951055363,-1.,0.748767076679177));
#52174=CARTESIAN_POINT('Ctrl Pts',(-4.08290608094789,-1.,0.746800631490821));
#52175=CARTESIAN_POINT('Ctrl Pts',(-4.09045220253011,-1.,0.744798649705514));
#52176=CARTESIAN_POINT('Ctrl Pts',(-4.09799769702712,-1.,0.742761369690017));
#52177=CARTESIAN_POINT('Ctrl Pts',(-4.1055424175856,-1.,0.740688998555151));
#52178=CARTESIAN_POINT('Ctrl Pts',(-4.11308626953795,-1.,0.738581708229118));
#52179=CARTESIAN_POINT('Ctrl Pts',(-4.12062919626082,-1.,0.736439634335347));
#52180=CARTESIAN_POINT('Ctrl Pts',(-4.12666277572794,-1.,0.734698226767512));
#52181=CARTESIAN_POINT('Ctrl Pts',(-4.13118752796397,-1.,0.733376589325634));
#52182=CARTESIAN_POINT('Ctrl Pts',(-4.13420383737278,-1.,0.732488575135926));
#52183=CARTESIAN_POINT('Ctrl Pts',(-4.13571194405636,-1.,0.732042837400619));
#52184=CARTESIAN_POINT('',(-4.15950947128175,-1.,0.581791163835814));
#52185=CARTESIAN_POINT('',(-4.13571194405636,-1.,0.732042837400619));
#52186=CARTESIAN_POINT('',(-3.73017266276632,-1.,0.385112848332549));
#52187=CARTESIAN_POINT('Ctrl Pts',(-4.15950947128175,-1.,0.581791163835814));
#52188=CARTESIAN_POINT('Ctrl Pts',(-4.15821291712391,-1.,0.580901211462913));
#52189=CARTESIAN_POINT('Ctrl Pts',(-4.15561864787379,-1.,0.579124568912543));
#52190=CARTESIAN_POINT('Ctrl Pts',(-4.1517237611974,-1.,0.576469391673916));
#52191=CARTESIAN_POINT('Ctrl Pts',(-4.14652361065787,-1.,0.572948736066276));
#52192=CARTESIAN_POINT('Ctrl Pts',(-4.14001179828669,-1.,0.568580610187116));
#52193=CARTESIAN_POINT('Ctrl Pts',(-4.13348835726086,-1.,0.564245279535705));
#52194=CARTESIAN_POINT('Ctrl Pts',(-4.12695329951859,-1.,0.559942890594628));
#52195=CARTESIAN_POINT('Ctrl Pts',(-4.1204066619623,-1.,0.555673636130778));
#52196=CARTESIAN_POINT('Ctrl Pts',(-4.11384852025578,-1.,0.551437758498246));
#52197=CARTESIAN_POINT('Ctrl Pts',(-4.1072789702877,-1.,0.547235539486759));
#52198=CARTESIAN_POINT('Ctrl Pts',(-4.10069810244473,-1.,0.543067286878457));
#52199=CARTESIAN_POINT('Ctrl Pts',(-4.09410597627116,-1.,0.53893332117992));
#52200=CARTESIAN_POINT('Ctrl Pts',(-4.08750259988693,-1.,0.534833963476999));
#52201=CARTESIAN_POINT('Ctrl Pts',(-4.08088789536488,-1.,0.530769518728075));
#52202=CARTESIAN_POINT('Ctrl Pts',(-4.07426172299496,-1.,0.526740277226999));
#52203=CARTESIAN_POINT('Ctrl Pts',(-4.06762394471075,-1.,0.522746528602767));
#52204=CARTESIAN_POINT('Ctrl Pts',(-4.06097448037934,-1.,0.518788572336809));
#52205=CARTESIAN_POINT('Ctrl Pts',(-4.05431335771261,-1.,0.514866728193104));
#52206=CARTESIAN_POINT('Ctrl Pts',(-4.04764078815591,-1.,0.510981349219173));
#52207=CARTESIAN_POINT('Ctrl Pts',(-4.04095715149074,-1.,0.507132823288361));
#52208=CARTESIAN_POINT('Ctrl Pts',(-4.0342628417439,-1.,0.503321556915513));
#52209=CARTESIAN_POINT('Ctrl Pts',(-4.0275581398015,-1.,0.499547962340889));
#52210=CARTESIAN_POINT('Ctrl Pts',(-4.02084308851813,-1.,0.495812444326223));
#52211=CARTESIAN_POINT('Ctrl Pts',(-4.01411733503486,-1.,0.49211538341793));
#52212=CARTESIAN_POINT('Ctrl Pts',(-4.0073800839092,-1.,0.48845713042453));
#52213=CARTESIAN_POINT('Ctrl Pts',(-4.00063045119234,-1.,0.484838042421754));
#52214=CARTESIAN_POINT('Ctrl Pts',(-3.99386775880655,-1.,0.481258512209638));
#52215=CARTESIAN_POINT('Ctrl Pts',(-3.98709184306743,-1.,0.477718999122033));
#52216=CARTESIAN_POINT('Ctrl Pts',(-3.9803033804443,-1.,0.474220061019542));
#52217=CARTESIAN_POINT('Ctrl Pts',(-3.97350414289415,-1.,0.470762379613477));
#52218=CARTESIAN_POINT('Ctrl Pts',(-3.96669622273946,-1.,0.467346690880671));
#52219=CARTESIAN_POINT('Ctrl Pts',(-3.95988133243543,-1.,0.463973722115744));
#52220=CARTESIAN_POINT('Ctrl Pts',(-3.95306005817363,-1.,0.460644124429119));
#52221=CARTESIAN_POINT('Ctrl Pts',(-3.94623117206675,-1.,0.457358410451674));
#52222=CARTESIAN_POINT('Ctrl Pts',(-3.93939080846298,-1.,0.454116879027576));
#52223=CARTESIAN_POINT('Ctrl Pts',(-3.93253407403128,-1.,0.450919768356347));
#52224=CARTESIAN_POINT('Ctrl Pts',(-3.92565674143424,-1.,0.447767416837296));
#52225=CARTESIAN_POINT('Ctrl Pts',(-3.91875701610721,-1.,0.444660430230592));
#52226=CARTESIAN_POINT('Ctrl Pts',(-3.91183704069146,-1.,0.441599824524047));
#52227=CARTESIAN_POINT('Ctrl Pts',(-3.90490512938546,-1.,0.438587235458233));
#52228=CARTESIAN_POINT('Ctrl Pts',(-3.8979725665544,-1.,0.435624629433505));
#52229=CARTESIAN_POINT('Ctrl Pts',(-3.89104947940592,-1.,0.432713929544439));
#52230=CARTESIAN_POINT('Ctrl Pts',(-3.88414070943334,-1.,0.429856640579733));
#52231=CARTESIAN_POINT('Ctrl Pts',(-3.87724240306609,-1.,0.427053541173469));
#52232=CARTESIAN_POINT('Ctrl Pts',(-3.87033643487882,-1.,0.424304173195142));
#52233=CARTESIAN_POINT('Ctrl Pts',(-3.86339652542749,-1.,0.421607423177575));
#52234=CARTESIAN_POINT('Ctrl Pts',(-3.85639825648031,-1.,0.418962468086809));
#52235=CARTESIAN_POINT('Ctrl Pts',(-3.8493286415751,-1.,0.41636967805292));
#52236=CARTESIAN_POINT('Ctrl Pts',(-3.84219403994742,-1.,0.413831367016726));
#52237=CARTESIAN_POINT('Ctrl Pts',(-3.83503345578645,-1.,0.411353038798459));
#52238=CARTESIAN_POINT('Ctrl Pts',(-3.82790724256397,-1.,0.408942371447377));
#52239=CARTESIAN_POINT('Ctrl Pts',(-3.82087303913741,-1.,0.406607038258906));
#52240=CARTESIAN_POINT('Ctrl Pts',(-3.81396374287762,-1.,0.404352694628236));
#52241=CARTESIAN_POINT('Ctrl Pts',(-3.80716881962763,-1.,0.402181320148474));
#52242=CARTESIAN_POINT('Ctrl Pts',(-3.80040370384659,-1.,0.400088346504726));
#52243=CARTESIAN_POINT('Ctrl Pts',(-3.79352887163457,-1.,0.398064818684158));
#52244=CARTESIAN_POINT('Ctrl Pts',(-3.78640521279479,-1.,0.396103205335028));
#52245=CARTESIAN_POINT('Ctrl Pts',(-3.77894173114368,-1.,0.394202481011595));
#52246=CARTESIAN_POINT('Ctrl Pts',(-3.77114011595892,-1.,0.392372786223346));
#52247=CARTESIAN_POINT('Ctrl Pts',(-3.76315635032993,-1.,0.390642072979259));
#52248=CARTESIAN_POINT('Ctrl Pts',(-3.75529302894757,-1.,0.389054775898251));
#52249=CARTESIAN_POINT('Ctrl Pts',(-3.74792651696269,-1.,0.387663020050396));
#52250=CARTESIAN_POINT('Ctrl Pts',(-3.74144965781088,-1.,0.386519576222035));
#52251=CARTESIAN_POINT('Ctrl Pts',(-3.73621371845475,-1.,0.385670806454744));
#52252=CARTESIAN_POINT('Ctrl Pts',(-3.73273893363318,-1.,0.385187124633964));
#52253=CARTESIAN_POINT('Ctrl Pts',(-3.73106082862399,-1.,0.385031656499141));
#52254=CARTESIAN_POINT('Ctrl Pts',(-3.73040527620929,-1.,0.385037797882046));
#52255=CARTESIAN_POINT('Ctrl Pts',(-3.73021431755218,-1.,0.385087139001609));
#52256=CARTESIAN_POINT('Ctrl Pts',(-3.73017266276632,-1.,0.385112848332549));
#52257=CARTESIAN_POINT('',(-3.74449296982994,-1.,0.203156094897895));
#52258=CARTESIAN_POINT('Origin',(0.,-1.,0.));
#52259=CARTESIAN_POINT('',(-4.19931119685982,-1.,0.0760622897878236));
#52260=CARTESIAN_POINT('Ctrl Pts',(-3.74449296982994,-1.,0.203156094897895));
#52261=CARTESIAN_POINT('Ctrl Pts',(-3.74453008995129,-1.,0.203188003947965));
#52262=CARTESIAN_POINT('Ctrl Pts',(-3.74471097893961,-1.,0.203266610111264));
#52263=CARTESIAN_POINT('Ctrl Pts',(-3.74535749969262,-1.,0.203375226874331));
#52264=CARTESIAN_POINT('Ctrl Pts',(-3.74703926501843,-1.,0.203484186269314));
#52265=CARTESIAN_POINT('Ctrl Pts',(-3.75054693397716,-1.,0.203550035479097));
#52266=CARTESIAN_POINT('Ctrl Pts',(-3.75585118707924,-1.,0.203530796848403));
#52267=CARTESIAN_POINT('Ctrl Pts',(-3.76242717937273,-1.,0.203414634707646));
#52268=CARTESIAN_POINT('Ctrl Pts',(-3.76992071595267,-1.,0.203192390045337));
#52269=CARTESIAN_POINT('Ctrl Pts',(-3.77793553476879,-1.,0.202854729699196));
#52270=CARTESIAN_POINT('Ctrl Pts',(-3.78609175019317,-1.,0.202394260512193));
#52271=CARTESIAN_POINT('Ctrl Pts',(-3.79408354187274,-1.,0.201807533800799));
#52272=CARTESIAN_POINT('Ctrl Pts',(-3.80175247447171,-1.,0.201097756307252));
#52273=CARTESIAN_POINT('Ctrl Pts',(-3.80909529318501,-1.,0.20027467943329));
#52274=CARTESIAN_POINT('Ctrl Pts',(-3.81620203429702,-1.,0.199351525297396));
#52275=CARTESIAN_POINT('Ctrl Pts',(-3.82321127348981,-1.,0.19834261690047));
#52276=CARTESIAN_POINT('Ctrl Pts',(-3.83026221776488,-1.,0.197260935827375));
#52277=CARTESIAN_POINT('Ctrl Pts',(-3.83743910616265,-1.,0.196115198971889));
#52278=CARTESIAN_POINT('Ctrl Pts',(-3.84475203347052,-1.,0.194909009460254));
#52279=CARTESIAN_POINT('Ctrl Pts',(-3.85216762264019,-1.,0.193642806777747));
#52280=CARTESIAN_POINT('Ctrl Pts',(-3.85962774407652,-1.,0.192315153044979));
#52281=CARTESIAN_POINT('Ctrl Pts',(-3.8670715862477,-1.,0.190924190418613));
#52282=CARTESIAN_POINT('Ctrl Pts',(-3.87445976418377,-1.,0.189469253358254));
#52283=CARTESIAN_POINT('Ctrl Pts',(-3.88178563496187,-1.,0.187951632512663));
#52284=CARTESIAN_POINT('Ctrl Pts',(-3.88906196725817,-1.,0.186373724985263));
#52285=CARTESIAN_POINT('Ctrl Pts',(-3.89631300742633,-1.,0.184738537728035));
#52286=CARTESIAN_POINT('Ctrl Pts',(-3.90356488555138,-1.,0.183049081993193));
#52287=CARTESIAN_POINT('Ctrl Pts',(-3.91083557557193,-1.,0.181307740731796));
#52288=CARTESIAN_POINT('Ctrl Pts',(-3.91812876180948,-1.,0.179515885822894));
#52289=CARTESIAN_POINT('Ctrl Pts',(-3.92543942697672,-1.,0.177674246152328));
#52290=CARTESIAN_POINT('Ctrl Pts',(-3.93275726771049,-1.,0.175783136893872));
#52291=CARTESIAN_POINT('Ctrl Pts',(-3.94007083096214,-1.,0.173842734974607));
#52292=CARTESIAN_POINT('Ctrl Pts',(-3.94737164900861,-1.,0.171853355369233));
#52293=CARTESIAN_POINT('Ctrl Pts',(-3.95465744665263,-1.,0.16981566637413));
#52294=CARTESIAN_POINT('Ctrl Pts',(-3.96192990160296,-1.,0.167730547023312));
#52295=CARTESIAN_POINT('Ctrl Pts',(-3.9691931362141,-1.,0.165598992851097));
#52296=CARTESIAN_POINT('Ctrl Pts',(-3.97645194630944,-1.,0.163422004609999));
#52297=CARTESIAN_POINT('Ctrl Pts',(-3.98371010319866,-1.,0.161200482186087));
#52298=CARTESIAN_POINT('Ctrl Pts',(-3.99096873945862,-1.,0.158935123982796));
#52299=CARTESIAN_POINT('Ctrl Pts',(-3.99822717425869,-1.,0.156626481393735));
#52300=CARTESIAN_POINT('Ctrl Pts',(-4.00548360245297,-1.,0.15427500487231));
#52301=CARTESIAN_POINT('Ctrl Pts',(-4.01273584234684,-1.,0.151881094022909));
#52302=CARTESIAN_POINT('Ctrl Pts',(-4.01998203715588,-1.,0.149445144968707));
#52303=CARTESIAN_POINT('Ctrl Pts',(-4.02722143147048,-1.,0.146967602878998));
#52304=CARTESIAN_POINT('Ctrl Pts',(-4.03445411510403,-1.,0.144448947038352));
#52305=CARTESIAN_POINT('Ctrl Pts',(-4.04168069633842,-1.,0.141889671485508));
#52306=CARTESIAN_POINT('Ctrl Pts',(-4.04890199238056,-1.,0.139290267180059));
#52307=CARTESIAN_POINT('Ctrl Pts',(-4.05611873400122,-1.,0.136651205046111));
#52308=CARTESIAN_POINT('Ctrl Pts',(-4.06333121018476,-1.,0.133972916144225));
#52309=CARTESIAN_POINT('Ctrl Pts',(-4.07053931528579,-1.,0.131255793548914));
#52310=CARTESIAN_POINT('Ctrl Pts',(-4.07774270738809,-1.,0.128500200484814));
#52311=CARTESIAN_POINT('Ctrl Pts',(-4.08494093372315,-1.,0.125706476822529));
#52312=CARTESIAN_POINT('Ctrl Pts',(-4.09213355850836,-1.,0.122874946249119));
#52313=CARTESIAN_POINT('Ctrl Pts',(-4.09932031767243,-1.,0.120005924388162));
#52314=CARTESIAN_POINT('Ctrl Pts',(-4.10650113382187,-1.,0.117099722731704));
#52315=CARTESIAN_POINT('Ctrl Pts',(-4.11367603925313,-1.,0.114156649609601));
#52316=CARTESIAN_POINT('Ctrl Pts',(-4.12084512502444,-1.,0.111177012683377));
#52317=CARTESIAN_POINT('Ctrl Pts',(-4.12800848371386,-1.,0.10816112052835));
#52318=CARTESIAN_POINT('Ctrl Pts',(-4.13516614458396,-1.,0.105109286538864));
#52319=CARTESIAN_POINT('Ctrl Pts',(-4.14231804938737,-1.,0.102021826577454));
#52320=CARTESIAN_POINT('Ctrl Pts',(-4.1494640891762,-1.,0.0988990478899811));
#52321=CARTESIAN_POINT('Ctrl Pts',(-4.15660412653006,-1.,0.0957412403297067));
#52322=CARTESIAN_POINT('Ctrl Pts',(-4.16373802265942,-1.,0.092548667216769));
#52323=CARTESIAN_POINT('Ctrl Pts',(-4.17086566491823,-1.,0.0893215560850327));
#52324=CARTESIAN_POINT('Ctrl Pts',(-4.17798698669991,-1.,0.0860600915552515));
#52325=CARTESIAN_POINT('Ctrl Pts',(-4.1851019532944,-1.,0.082764416438951));
#52326=CARTESIAN_POINT('Ctrl Pts',(-4.19078883322483,-1.,0.0801005887117603));
#52327=CARTESIAN_POINT('Ctrl Pts',(-4.19505112860624,-1.,0.0780873956244402));
#52328=CARTESIAN_POINT('Ctrl Pts',(-4.19789138621624,-1.,0.0767384596142195));
#52329=CARTESIAN_POINT('Ctrl Pts',(-4.19931119685982,-1.,0.0760622897878236));
#52330=CARTESIAN_POINT('',(-4.19931119685982,-1.,-0.0760622897878246));
#52331=CARTESIAN_POINT('',(-4.19931119685982,-1.,0.0760622897878236));
#52332=CARTESIAN_POINT('',(-3.74449296983004,-1.,-0.203156094896101));
#52333=CARTESIAN_POINT('Ctrl Pts',(-4.19931119685982,-1.,-0.0760622897878246));
#52334=CARTESIAN_POINT('Ctrl Pts',(-4.1978913862118,-1.,-0.0767384596141464));
#52335=CARTESIAN_POINT('Ctrl Pts',(-4.19505112859416,-1.,-0.0780873956242397));
#52336=CARTESIAN_POINT('Ctrl Pts',(-4.19078883320504,-1.,-0.080100588711432));
#52337=CARTESIAN_POINT('Ctrl Pts',(-4.18510195327123,-1.,-0.0827644164385679));
#52338=CARTESIAN_POINT('Ctrl Pts',(-4.17798698668094,-1.,-0.0860600915549397));
#52339=CARTESIAN_POINT('Ctrl Pts',(-4.17086566490794,-1.,-0.0893215560848649));
#52340=CARTESIAN_POINT('Ctrl Pts',(-4.16373802265839,-1.,-0.0925486672167531));
#52341=CARTESIAN_POINT('Ctrl Pts',(-4.15660412653577,-1.,-0.0957412403298007));
#52342=CARTESIAN_POINT('Ctrl Pts',(-4.14946408918485,-1.,-0.0988990478901226));
#52343=CARTESIAN_POINT('Ctrl Pts',(-4.14231804939538,-1.,-0.102021826577584));
#52344=CARTESIAN_POINT('Ctrl Pts',(-4.13516614458895,-1.,-0.105109286538945));
#52345=CARTESIAN_POINT('Ctrl Pts',(-4.12800848371504,-1.,-0.108161120528369));
#52346=CARTESIAN_POINT('Ctrl Pts',(-4.1208451250225,-1.,-0.111177012683347));
#52347=CARTESIAN_POINT('Ctrl Pts',(-4.11367603924961,-1.,-0.114156649609546));
#52348=CARTESIAN_POINT('Ctrl Pts',(-4.10650113381833,-1.,-0.117099722731648));
#52349=CARTESIAN_POINT('Ctrl Pts',(-4.09932031767002,-1.,-0.120005924388124));
#52350=CARTESIAN_POINT('Ctrl Pts',(-4.09213355850756,-1.,-0.122874946249107));
#52351=CARTESIAN_POINT('Ctrl Pts',(-4.08494093372377,-1.,-0.12570647682254));
#52352=CARTESIAN_POINT('Ctrl Pts',(-4.07774270738954,-1.,-0.128500200484838));
#52353=CARTESIAN_POINT('Ctrl Pts',(-4.0705393152874,-1.,-0.13125579354894));
#52354=CARTESIAN_POINT('Ctrl Pts',(-4.06333121018596,-1.,-0.133972916144245));
#52355=CARTESIAN_POINT('Ctrl Pts',(-4.05611873400172,-1.,-0.136651205046119));
#52356=CARTESIAN_POINT('Ctrl Pts',(-4.04890199238036,-1.,-0.139290267180057));
#52357=CARTESIAN_POINT('Ctrl Pts',(-4.04168069633781,-1.,-0.1418896714855));
#52358=CARTESIAN_POINT('Ctrl Pts',(-4.03445411510333,-1.,-0.144448947038345));
#52359=CARTESIAN_POINT('Ctrl Pts',(-4.02722143146994,-1.,-0.146967602878994));
#52360=CARTESIAN_POINT('Ctrl Pts',(-4.01998203715564,-1.,-0.149445144968707));
#52361=CARTESIAN_POINT('Ctrl Pts',(-4.01273584234689,-1.,-0.151881094022911));
#52362=CARTESIAN_POINT('Ctrl Pts',(-4.00548360245319,-1.,-0.154275004872311));
#52363=CARTESIAN_POINT('Ctrl Pts',(-3.99822717425893,-1.,-0.156626481393734));
#52364=CARTESIAN_POINT('Ctrl Pts',(-3.99096873945878,-1.,-0.158935123982793));
#52365=CARTESIAN_POINT('Ctrl Pts',(-3.98371010319872,-1.,-0.161200482186085));
#52366=CARTESIAN_POINT('Ctrl Pts',(-3.97645194630943,-1.,-0.163422004609999));
#52367=CARTESIAN_POINT('Ctrl Pts',(-3.96919313621407,-1.,-0.165598992851102));
#52368=CARTESIAN_POINT('Ctrl Pts',(-3.96192990160296,-1.,-0.167730547023319));
#52369=CARTESIAN_POINT('Ctrl Pts',(-3.95465744665268,-1.,-0.169815666374139));
#52370=CARTESIAN_POINT('Ctrl Pts',(-3.94737164900868,-1.,-0.17185335536924));
#52371=CARTESIAN_POINT('Ctrl Pts',(-3.94007083096217,-1.,-0.17384273497461));
#52372=CARTESIAN_POINT('Ctrl Pts',(-3.93275726771042,-1.,-0.175783136893868));
#52373=CARTESIAN_POINT('Ctrl Pts',(-3.92543942697655,-1.,-0.177674246152317));
#52374=CARTESIAN_POINT('Ctrl Pts',(-3.91812876180926,-1.,-0.179515885822882));
#52375=CARTESIAN_POINT('Ctrl Pts',(-3.91083557557175,-1.,-0.181307740731786));
#52376=CARTESIAN_POINT('Ctrl Pts',(-3.90356488555132,-1.,-0.183049081993191));
#52377=CARTESIAN_POINT('Ctrl Pts',(-3.89631300742646,-1.,-0.184738537728043));
#52378=CARTESIAN_POINT('Ctrl Pts',(-3.88906196725848,-1.,-0.18637372498528));
#52379=CARTESIAN_POINT('Ctrl Pts',(-3.88178563496228,-1.,-0.187951632512685));
#52380=CARTESIAN_POINT('Ctrl Pts',(-3.87445976418412,-1.,-0.189469253358272));
#52381=CARTESIAN_POINT('Ctrl Pts',(-3.86707158624783,-1.,-0.19092419041862));
#52382=CARTESIAN_POINT('Ctrl Pts',(-3.85962774407633,-1.,-0.192315153044971));
#52383=CARTESIAN_POINT('Ctrl Pts',(-3.85216762263966,-1.,-0.193642806777723));
#52384=CARTESIAN_POINT('Ctrl Pts',(-3.84475203346977,-1.,-0.194909009460221));
#52385=CARTESIAN_POINT('Ctrl Pts',(-3.83743910616195,-1.,-0.196115198971859));
#52386=CARTESIAN_POINT('Ctrl Pts',(-3.83026221776456,-1.,-0.197260935827361));
#52387=CARTESIAN_POINT('Ctrl Pts',(-3.82321127349016,-1.,-0.198342616900486));
#52388=CARTESIAN_POINT('Ctrl Pts',(-3.81620203429815,-1.,-0.199351525297447));
#52389=CARTESIAN_POINT('Ctrl Pts',(-3.80909529318669,-1.,-0.200274679433364));
#52390=CARTESIAN_POINT('Ctrl Pts',(-3.80175247447337,-1.,-0.201097756307326));
#52391=CARTESIAN_POINT('Ctrl Pts',(-3.7940835418736,-1.,-0.201807533800837));
#52392=CARTESIAN_POINT('Ctrl Pts',(-3.78609175019242,-1.,-0.20239426051216));
#52393=CARTESIAN_POINT('Ctrl Pts',(-3.77793553476614,-1.,-0.202854729699081));
#52394=CARTESIAN_POINT('Ctrl Pts',(-3.7699207159487,-1.,-0.203192390045164));
#52395=CARTESIAN_POINT('Ctrl Pts',(-3.76242717936885,-1.,-0.203414634707478));
#52396=CARTESIAN_POINT('Ctrl Pts',(-3.75585118707734,-1.,-0.203530796848322));
#52397=CARTESIAN_POINT('Ctrl Pts',(-3.75054693397875,-1.,-0.203550035479166));
#52398=CARTESIAN_POINT('Ctrl Pts',(-3.74703926501752,-1.,-0.203484186269415));
#52399=CARTESIAN_POINT('Ctrl Pts',(-3.74535749969115,-1.,-0.203375226874121));
#52400=CARTESIAN_POINT('Ctrl Pts',(-3.74471097893845,-1.,-0.203266610110531));
#52401=CARTESIAN_POINT('Ctrl Pts',(-3.74453008995092,-1.,-0.203188003946657));
#52402=CARTESIAN_POINT('Ctrl Pts',(-3.74449296983004,-1.,-0.203156094896101));
#52403=CARTESIAN_POINT('',(-3.73017266276651,-1.,-0.385112848330762));
#52404=CARTESIAN_POINT('Origin',(0.,-1.,0.));
#52405=CARTESIAN_POINT('',(-4.15950947128175,-1.,-0.581791163835815));
#52406=CARTESIAN_POINT('Ctrl Pts',(-3.73017266276651,-1.,-0.385112848330762));
#52407=CARTESIAN_POINT('Ctrl Pts',(-3.73021431755274,-1.,-0.385087139000374));
#52408=CARTESIAN_POINT('Ctrl Pts',(-3.73040527621055,-1.,-0.385037797881504));
#52409=CARTESIAN_POINT('Ctrl Pts',(-3.73106082862548,-1.,-0.385031656499164));
#52410=CARTESIAN_POINT('Ctrl Pts',(-3.73273893363406,-1.,-0.385187124634206));
#52411=CARTESIAN_POINT('Ctrl Pts',(-3.73621371845318,-1.,-0.385670806454566));
#52412=CARTESIAN_POINT('Ctrl Pts',(-3.74144965781276,-1.,-0.386519576222251));
#52413=CARTESIAN_POINT('Ctrl Pts',(-3.74792651696654,-1.,-0.387663020050836));
#52414=CARTESIAN_POINT('Ctrl Pts',(-3.75529302895152,-1.,-0.389054775898702));
#52415=CARTESIAN_POINT('Ctrl Pts',(-3.76315635033257,-1.,-0.39064207297956));
#52416=CARTESIAN_POINT('Ctrl Pts',(-3.77114011595967,-1.,-0.392372786223432));
#52417=CARTESIAN_POINT('Ctrl Pts',(-3.77894173114283,-1.,-0.394202481011499));
#52418=CARTESIAN_POINT('Ctrl Pts',(-3.78640521279313,-1.,-0.396103205334841));
#52419=CARTESIAN_POINT('Ctrl Pts',(-3.7935288716329,-1.,-0.398064818683969));
#52420=CARTESIAN_POINT('Ctrl Pts',(-3.80040370384546,-1.,-0.4000883465046));
#52421=CARTESIAN_POINT('Ctrl Pts',(-3.80716881962728,-1.,-0.402181320148436));
#52422=CARTESIAN_POINT('Ctrl Pts',(-3.81396374287793,-1.,-0.404352694628273));
#52423=CARTESIAN_POINT('Ctrl Pts',(-3.8208730391381,-1.,-0.406607038258985));
#52424=CARTESIAN_POINT('Ctrl Pts',(-3.82790724256471,-1.,-0.40894237144746));
#52425=CARTESIAN_POINT('Ctrl Pts',(-3.83503345578698,-1.,-0.411353038798518));
#52426=CARTESIAN_POINT('Ctrl Pts',(-3.84219403994762,-1.,-0.413831367016748));
#52427=CARTESIAN_POINT('Ctrl Pts',(-3.84932864157497,-1.,-0.416369678052907));
#52428=CARTESIAN_POINT('Ctrl Pts',(-3.85639825647996,-1.,-0.418962468086773));
#52429=CARTESIAN_POINT('Ctrl Pts',(-3.86339652542709,-1.,-0.421607423177534));
#52430=CARTESIAN_POINT('Ctrl Pts',(-3.87033643487851,-1.,-0.424304173195111));
#52431=CARTESIAN_POINT('Ctrl Pts',(-3.87724240306597,-1.,-0.427053541173457));
#52432=CARTESIAN_POINT('Ctrl Pts',(-3.88414070943341,-1.,-0.429856640579741));
#52433=CARTESIAN_POINT('Ctrl Pts',(-3.89104947940611,-1.,-0.432713929544458));
#52434=CARTESIAN_POINT('Ctrl Pts',(-3.89797256655462,-1.,-0.435624629433527));
#52435=CARTESIAN_POINT('Ctrl Pts',(-3.90490512938563,-1.,-0.438587235458249));
#52436=CARTESIAN_POINT('Ctrl Pts',(-3.91183704069153,-1.,-0.441599824524054));
#52437=CARTESIAN_POINT('Ctrl Pts',(-3.91875701610719,-1.,-0.444660430230591));
#52438=CARTESIAN_POINT('Ctrl Pts',(-3.92565674143416,-1.,-0.447767416837292));
#52439=CARTESIAN_POINT('Ctrl Pts',(-3.93253407403123,-1.,-0.450919768356348));
#52440=CARTESIAN_POINT('Ctrl Pts',(-3.93939080846298,-1.,-0.454116879027584));
#52441=CARTESIAN_POINT('Ctrl Pts',(-3.94623117206678,-1.,-0.457358410451683));
#52442=CARTESIAN_POINT('Ctrl Pts',(-3.95306005817364,-1.,-0.460644124429121));
#52443=CARTESIAN_POINT('Ctrl Pts',(-3.95988133243538,-1.,-0.463973722115733));
#52444=CARTESIAN_POINT('Ctrl Pts',(-3.9666962227393,-1.,-0.467346690880643));
#52445=CARTESIAN_POINT('Ctrl Pts',(-3.97350414289392,-1.,-0.470762379613439));
#52446=CARTESIAN_POINT('Ctrl Pts',(-3.98030338044409,-1.,-0.47422006101951));
#52447=CARTESIAN_POINT('Ctrl Pts',(-3.98709184306738,-1.,-0.477718999122027));
#52448=CARTESIAN_POINT('Ctrl Pts',(-3.99386775880679,-1.,-0.481258512209675));
#52449=CARTESIAN_POINT('Ctrl Pts',(-4.00063045119288,-1.,-0.484838042421835));
#52450=CARTESIAN_POINT('Ctrl Pts',(-4.0073800839099,-1.,-0.488457130424633));
#52451=CARTESIAN_POINT('Ctrl Pts',(-4.01411733503546,-1.,-0.492115383418018));
#52452=CARTESIAN_POINT('Ctrl Pts',(-4.02084308851832,-1.,-0.495812444326251));
#52453=CARTESIAN_POINT('Ctrl Pts',(-4.02755813980101,-1.,-0.499547962340821));
#52454=CARTESIAN_POINT('Ctrl Pts',(-4.03426284174272,-1.,-0.503321556915346));
#52455=CARTESIAN_POINT('Ctrl Pts',(-4.04095715148915,-1.,-0.507132823288136));
#52456=CARTESIAN_POINT('Ctrl Pts',(-4.04764078815447,-1.,-0.51098134921897));
#52457=CARTESIAN_POINT('Ctrl Pts',(-4.05431335771199,-1.,-0.514866728193017));
#52458=CARTESIAN_POINT('Ctrl Pts',(-4.06097448038013,-1.,-0.518788572336923));
#52459=CARTESIAN_POINT('Ctrl Pts',(-4.06762394471314,-1.,-0.522746528603107));
#52460=CARTESIAN_POINT('Ctrl Pts',(-4.07426172299847,-1.,-0.526740277227498));
#52461=CARTESIAN_POINT('Ctrl Pts',(-4.08088789536836,-1.,-0.530769518728571));
#52462=CARTESIAN_POINT('Ctrl Pts',(-4.08750259988885,-1.,-0.534833963477273));
#52463=CARTESIAN_POINT('Ctrl Pts',(-4.09410597627,-1.,-0.538933321179756));
#52464=CARTESIAN_POINT('Ctrl Pts',(-4.10069810243979,-1.,-0.543067286877757));
#52465=CARTESIAN_POINT('Ctrl Pts',(-4.10727897027977,-1.,-0.547235539485637));
#52466=CARTESIAN_POINT('Ctrl Pts',(-4.11384852024721,-1.,-0.551437758497032));
#52467=CARTESIAN_POINT('Ctrl Pts',(-4.12040666195664,-1.,-0.555673636129977));
#52468=CARTESIAN_POINT('Ctrl Pts',(-4.12695329951961,-1.,-0.559942890594773));
#52469=CARTESIAN_POINT('Ctrl Pts',(-4.13348835727104,-1.,-0.564245279537148));
#52470=CARTESIAN_POINT('Ctrl Pts',(-4.14001179830547,-1.,-0.568580610189774));
#52471=CARTESIAN_POINT('Ctrl Pts',(-4.14652361068081,-1.,-0.572948736069522));
#52472=CARTESIAN_POINT('Ctrl Pts',(-4.151723761217,-1.,-0.576469391676688));
#52473=CARTESIAN_POINT('Ctrl Pts',(-4.15561864788576,-1.,-0.579124568914235));
#52474=CARTESIAN_POINT('Ctrl Pts',(-4.1582129171283,-1.,-0.580901211463535));
#52475=CARTESIAN_POINT('Ctrl Pts',(-4.15950947128175,-1.,-0.581791163835815));
#52476=CARTESIAN_POINT('',(-4.13571194405636,-1.,-0.73204283740062));
#52477=CARTESIAN_POINT('',(-4.15950947128175,-1.,-0.581791163835815));
#52478=CARTESIAN_POINT('',(-3.66661143271685,-1.,-0.786422660831985));
#52479=CARTESIAN_POINT('Ctrl Pts',(-4.13571194405636,-1.,-0.73204283740062));
#52480=CARTESIAN_POINT('Ctrl Pts',(-4.1342038373684,-1.,-0.732488575135159));
#52481=CARTESIAN_POINT('Ctrl Pts',(-4.13118752795207,-1.,-0.733376589323546));
#52482=CARTESIAN_POINT('Ctrl Pts',(-4.12666277570844,-1.,-0.734698226764092));
#52483=CARTESIAN_POINT('Ctrl Pts',(-4.120629196238,-1.,-0.736439634331345));
#52484=CARTESIAN_POINT('Ctrl Pts',(-4.11308626951927,-1.,-0.738581708225844));
#52485=CARTESIAN_POINT('Ctrl Pts',(-4.10554241757547,-1.,-0.740688998553377));
#52486=CARTESIAN_POINT('Ctrl Pts',(-4.09799769702611,-1.,-0.742761369689841));
#52487=CARTESIAN_POINT('Ctrl Pts',(-4.09045220253573,-1.,-0.7447986497065));
#52488=CARTESIAN_POINT('Ctrl Pts',(-4.08290608095642,-1.,-0.746800631492315));
#52489=CARTESIAN_POINT('Ctrl Pts',(-4.07535951056152,-1.,-0.748767076680557));
#52490=CARTESIAN_POINT('Ctrl Pts',(-4.06781267242378,-1.,-0.750697720484036));
#52491=CARTESIAN_POINT('Ctrl Pts',(-4.06026572221515,-1.,-0.752592276483072));
#52492=CARTESIAN_POINT('Ctrl Pts',(-4.05271876687915,-1.,-0.754450441816078));
#52493=CARTESIAN_POINT('Ctrl Pts',(-4.04517182653997,-1.,-0.756271902369581));
#52494=CARTESIAN_POINT('Ctrl Pts',(-4.03762485803119,-1.,-0.758056338884944));
#52495=CARTESIAN_POINT('Ctrl Pts',(-4.03007781954412,-1.,-0.759803433243752));
#52496=CARTESIAN_POINT('Ctrl Pts',(-4.02253072741268,-1.,-0.761512875859804));
#52497=CARTESIAN_POINT('Ctrl Pts',(-4.01498370680496,-1.,-0.763184371182935));
#52498=CARTESIAN_POINT('Ctrl Pts',(-4.00743706791509,-1.,-0.764817648785197));
#52499=CARTESIAN_POINT('Ctrl Pts',(-3.99989129179622,-1.,-0.766412457136064));
#52500=CARTESIAN_POINT('Ctrl Pts',(-3.9923468788101,-1.,-0.767968531377915));
#52501=CARTESIAN_POINT('Ctrl Pts',(-3.98480422348451,-1.,-0.769485566245544));
#52502=CARTESIAN_POINT('Ctrl Pts',(-3.97726349165488,-1.,-0.770963190030471));
#52503=CARTESIAN_POINT('Ctrl Pts',(-3.96972446532772,-1.,-0.772400931772136));
#52504=CARTESIAN_POINT('Ctrl Pts',(-3.96218649639807,-1.,-0.773798212026565));
#52505=CARTESIAN_POINT('Ctrl Pts',(-3.9546488545231,-1.,-0.775154418039351));
#52506=CARTESIAN_POINT('Ctrl Pts',(-3.94711101619447,-1.,-0.776468966697921));
#52507=CARTESIAN_POINT('Ctrl Pts',(-3.93957296768103,-1.,-0.777741370568558));
#52508=CARTESIAN_POINT('Ctrl Pts',(-3.93203552473174,-1.,-0.778971308134821));
#52509=CARTESIAN_POINT('Ctrl Pts',(-3.92450058323823,-1.,-0.780158678615542));
#52510=CARTESIAN_POINT('Ctrl Pts',(-3.91697036054676,-1.,-0.781303428618366));
#52511=CARTESIAN_POINT('Ctrl Pts',(-3.90944671004542,-1.,-0.782405395622764));
#52512=CARTESIAN_POINT('Ctrl Pts',(-3.9019303904397,-1.,-0.783464141529081));
#52513=CARTESIAN_POINT('Ctrl Pts',(-3.89442039235103,-1.,-0.784478799358336));
#52514=CARTESIAN_POINT('Ctrl Pts',(-3.88691313167398,-1.,-0.78544789034073));
#52515=CARTESIAN_POINT('Ctrl Pts',(-3.8794040281819,-1.,-0.786369675812608));
#52516=CARTESIAN_POINT('Ctrl Pts',(-3.87188916600912,-1.,-0.787242527617999));
#52517=CARTESIAN_POINT('Ctrl Pts',(-3.86436702561345,-1.,-0.788065315093777));
#52518=CARTESIAN_POINT('Ctrl Pts',(-3.85683995872529,-1.,-0.788837734090672));
#52519=CARTESIAN_POINT('Ctrl Pts',(-3.84931637808894,-1.,-0.789560798155582));
#52520=CARTESIAN_POINT('Ctrl Pts',(-3.84180762342454,-1.,-0.790236124191242));
#52521=CARTESIAN_POINT('Ctrl Pts',(-3.83432392054786,-1.,-0.790865012705301));
#52522=CARTESIAN_POINT('Ctrl Pts',(-3.82687033899792,-1.,-0.791447528662369));
#52523=CARTESIAN_POINT('Ctrl Pts',(-3.81944345442249,-1.,-0.791981740718635));
#52524=CARTESIAN_POINT('Ctrl Pts',(-3.81202588694756,-1.,-0.792462483517634));
#52525=CARTESIAN_POINT('Ctrl Pts',(-3.80459229925637,-1.,-0.792882695234778));
#52526=CARTESIAN_POINT('Ctrl Pts',(-3.79711921389897,-1.,-0.793235612973273));
#52527=CARTESIAN_POINT('Ctrl Pts',(-3.78959439439235,-1.,-0.793516871680993));
#52528=CARTESIAN_POINT('Ctrl Pts',(-3.78202460377598,-1.,-0.7937262357813));
#52529=CARTESIAN_POINT('Ctrl Pts',(-3.77444863801212,-1.,-0.793870523787408));
#52530=CARTESIAN_POINT('Ctrl Pts',(-3.76692626931111,-1.,-0.793961083688991));
#52531=CARTESIAN_POINT('Ctrl Pts',(-3.75951468666257,-1.,-0.794008429134907));
#52532=CARTESIAN_POINT('Ctrl Pts',(-3.75224692493864,-1.,-0.794017347371377));
#52533=CARTESIAN_POINT('Ctrl Pts',(-3.74511357728861,-1.,-0.793982700459952));
#52534=CARTESIAN_POINT('Ctrl Pts',(-3.73803280541687,-1.,-0.793882700937017));
#52535=CARTESIAN_POINT('Ctrl Pts',(-3.73086914695805,-1.,-0.793682750269684));
#52536=CARTESIAN_POINT('Ctrl Pts',(-3.72348797293734,-1.,-0.793347023784205));
#52537=CARTESIAN_POINT('Ctrl Pts',(-3.71580242396124,-1.,-0.792848377370287));
#52538=CARTESIAN_POINT('Ctrl Pts',(-3.70781724021806,-1.,-0.792177688845818));
#52539=CARTESIAN_POINT('Ctrl Pts',(-3.69968940808721,-1.,-0.79135657569598));
#52540=CARTESIAN_POINT('Ctrl Pts',(-3.69172044327364,-1.,-0.790436284988787));
#52541=CARTESIAN_POINT('Ctrl Pts',(-3.68428439783905,-1.,-0.789483546064387));
#52542=CARTESIAN_POINT('Ctrl Pts',(-3.67777119516252,-1.,-0.788569566220285));
#52543=CARTESIAN_POINT('Ctrl Pts',(-3.67252923663655,-1.,-0.787758799995742));
#52544=CARTESIAN_POINT('Ctrl Pts',(-3.66907505398677,-1.,-0.787145041181545));
#52545=CARTESIAN_POINT('Ctrl Pts',(-3.66743103898702,-1.,-0.786774337198062));
#52546=CARTESIAN_POINT('Ctrl Pts',(-3.66680946938292,-1.,-0.786565919558984));
#52547=CARTESIAN_POINT('Ctrl Pts',(-3.6666431041522,-1.,-0.786459983895432));
#52548=CARTESIAN_POINT('Ctrl Pts',(-3.66661143271685,-1.,-0.786422660831985));
#52549=CARTESIAN_POINT('',(-3.62400312501245,-1.,-0.963899035117249));
#52550=CARTESIAN_POINT('Origin',(0.,-1.,0.));
#52551=CARTESIAN_POINT('',(-4.01728681790024,-1.,-1.22531898815164));
#52552=CARTESIAN_POINT('Ctrl Pts',(-3.62400312501245,-1.,-0.963899035117249));
#52553=CARTESIAN_POINT('Ctrl Pts',(-3.6240482887845,-1.,-0.963880158555582));
#52554=CARTESIAN_POINT('Ctrl Pts',(-3.62424461507588,-1.,-0.963861297423241));
#52555=CARTESIAN_POINT('Ctrl Pts',(-3.62489305727662,-1.,-0.963957782642843));
#52556=CARTESIAN_POINT('Ctrl Pts',(-3.62652618145335,-1.,-0.964373850166457));
#52557=CARTESIAN_POINT('Ctrl Pts',(-3.62988252139846,-1.,-0.965395153165293));
#52558=CARTESIAN_POINT('Ctrl Pts',(-3.63492122081143,-1.,-0.967052554541385));
#52559=CARTESIAN_POINT('Ctrl Pts',(-3.64113946505766,-1.,-0.969195124675865));
#52560=CARTESIAN_POINT('Ctrl Pts',(-3.64819756447455,-1.,-0.971722122061341));
#52561=CARTESIAN_POINT('Ctrl Pts',(-3.65571576735126,-1.,-0.974519971354848));
#52562=CARTESIAN_POINT('Ctrl Pts',(-3.66333049637475,-1.,-0.977478312751618));
#52563=CARTESIAN_POINT('Ctrl Pts',(-3.67074983340361,-1.,-0.980505922458267));
#52564=CARTESIAN_POINT('Ctrl Pts',(-3.67782408841715,-1.,-0.983550791470419));
#52565=CARTESIAN_POINT('Ctrl Pts',(-3.68455317926068,-1.,-0.986602639863837));
#52566=CARTESIAN_POINT('Ctrl Pts',(-3.69102682138846,-1.,-0.989676715398558));
#52567=CARTESIAN_POINT('Ctrl Pts',(-3.69738123415662,-1.,-0.99280221833201));
#52568=CARTESIAN_POINT('Ctrl Pts',(-3.70375282282138,-1.,-0.996009819772518));
#52569=CARTESIAN_POINT('Ctrl Pts',(-3.71022439713938,-1.,-0.99931726075653));
#52570=CARTESIAN_POINT('Ctrl Pts',(-3.71680667125118,-1.,-1.00272423396822));
#52571=CARTESIAN_POINT('Ctrl Pts',(-3.72346803750595,-1.,-1.0062200073571));
#52572=CARTESIAN_POINT('Ctrl Pts',(-3.73015276704426,-1.,-1.00978798539496));
#52573=CARTESIAN_POINT('Ctrl Pts',(-3.73680245055734,-1.,-1.01341114319903));
#52574=CARTESIAN_POINT('Ctrl Pts',(-3.74337942504959,-1.,-1.01707794311079));
#52575=CARTESIAN_POINT('Ctrl Pts',(-3.74987777155834,-1.,-1.02078510487428));
#52576=CARTESIAN_POINT('Ctrl Pts',(-3.75631037456194,-1.,-1.0245342944466));
#52577=CARTESIAN_POINT('Ctrl Pts',(-3.76270122291232,-1.,-1.02833014458181));
#52578=CARTESIAN_POINT('Ctrl Pts',(-3.76907609832522,-1.,-1.0321778660492));
#52579=CARTESIAN_POINT('Ctrl Pts',(-3.77545283140445,-1.,-1.03608074678013));
#52580=CARTESIAN_POINT('Ctrl Pts',(-3.78183535008192,-1.,-1.04003862055804));
#52581=CARTESIAN_POINT('Ctrl Pts',(-3.78821910787195,-1.,-1.04404924374426));
#52582=CARTESIAN_POINT('Ctrl Pts',(-3.79459440308793,-1.,-1.04810913267641));
#52583=CARTESIAN_POINT('Ctrl Pts',(-3.80095039790678,-1.,-1.05221457990015));
#52584=CARTESIAN_POINT('Ctrl Pts',(-3.80727913637784,-1.,-1.05636266918643));
#52585=CARTESIAN_POINT('Ctrl Pts',(-3.81357866117485,-1.,-1.06055206187298));
#52586=CARTESIAN_POINT('Ctrl Pts',(-3.81985083953012,-1.,-1.06478244038931));
#52587=CARTESIAN_POINT('Ctrl Pts',(-3.82609989967278,-1.,-1.0690541318036));
#52588=CARTESIAN_POINT('Ctrl Pts',(-3.83233071195145,-1.,-1.0733676663346));
#52589=CARTESIAN_POINT('Ctrl Pts',(-3.83854714117486,-1.,-1.07772335353856));
#52590=CARTESIAN_POINT('Ctrl Pts',(-3.84475048030615,-1.,-1.08212087917986));
#52591=CARTESIAN_POINT('Ctrl Pts',(-3.8509402522269,-1.,-1.08655950846377));
#52592=CARTESIAN_POINT('Ctrl Pts',(-3.85711487933911,-1.,-1.09103825516288));
#52593=CARTESIAN_POINT('Ctrl Pts',(-3.86327241021242,-1.,-1.09555606505012));
#52594=CARTESIAN_POINT('Ctrl Pts',(-3.86941120134872,-1.,-1.10011198761202));
#52595=CARTESIAN_POINT('Ctrl Pts',(-3.87553067187566,-1.,-1.10470536603303));
#52596=CARTESIAN_POINT('Ctrl Pts',(-3.88163105531791,-1.,-1.10933577224029));
#52597=CARTESIAN_POINT('Ctrl Pts',(-3.88771308285229,-1.,-1.11400292434447));
#52598=CARTESIAN_POINT('Ctrl Pts',(-3.89377768340362,-1.,-1.11870660794609));
#52599=CARTESIAN_POINT('Ctrl Pts',(-3.89982569749978,-1.,-1.12344660099029));
#52600=CARTESIAN_POINT('Ctrl Pts',(-3.90585753318622,-1.,-1.12822258281518));
#52601=CARTESIAN_POINT('Ctrl Pts',(-3.91187321145495,-1.,-1.13303414693849));
#52602=CARTESIAN_POINT('Ctrl Pts',(-3.91787251936688,-1.,-1.13788084225511));
#52603=CARTESIAN_POINT('Ctrl Pts',(-3.92385513133937,-1.,-1.14276220561575));
#52604=CARTESIAN_POINT('Ctrl Pts',(-3.92982073294334,-1.,-1.14767779451147));
#52605=CARTESIAN_POINT('Ctrl Pts',(-3.9357691705651,-1.,-1.1526272271639));
#52606=CARTESIAN_POINT('Ctrl Pts',(-3.94170046685542,-1.,-1.1576101834106));
#52607=CARTESIAN_POINT('Ctrl Pts',(-3.9476147478092,-1.,-1.16262637999261));
#52608=CARTESIAN_POINT('Ctrl Pts',(-3.95351219510062,-1.,-1.16767555244495));
#52609=CARTESIAN_POINT('Ctrl Pts',(-3.95939299213164,-1.,-1.17275743590327));
#52610=CARTESIAN_POINT('Ctrl Pts',(-3.96525726357682,-1.,-1.17787174135445));
#52611=CARTESIAN_POINT('Ctrl Pts',(-3.9711050516465,-1.,-1.18301815039596));
#52612=CARTESIAN_POINT('Ctrl Pts',(-3.97693634766926,-1.,-1.18819633715285));
#52613=CARTESIAN_POINT('Ctrl Pts',(-3.98275111052015,-1.,-1.19340598349307));
#52614=CARTESIAN_POINT('Ctrl Pts',(-3.98854928957287,-1.,-1.19864679609596));
#52615=CARTESIAN_POINT('Ctrl Pts',(-3.99433084800649,-1.,-1.2039185237544));
#52616=CARTESIAN_POINT('Ctrl Pts',(-4.00009577952534,-1.,-1.20922097030107));
#52617=CARTESIAN_POINT('Ctrl Pts',(-4.00584409524937,-1.,-1.21455398918813));
#52618=CARTESIAN_POINT('Ctrl Pts',(-4.01042947142681,-1.,-1.21884478244983));
#52619=CARTESIAN_POINT('Ctrl Pts',(-4.01386104434674,-1.,-1.22207656456199));
#52620=CARTESIAN_POINT('Ctrl Pts',(-4.0161454457032,-1.,-1.22423716681447));
#52621=CARTESIAN_POINT('Ctrl Pts',(-4.01728681790024,-1.,-1.22531898815164));
#52622=CARTESIAN_POINT('',(-3.97027773754922,-1.,-1.36999806084572));
#52623=CARTESIAN_POINT('',(-4.01728681790024,-1.,-1.22531898815164));
#52624=CARTESIAN_POINT('',(-3.4984457533445,-1.,-1.35032489087101));
#52625=CARTESIAN_POINT('Ctrl Pts',(-3.97027773754922,-1.,-1.36999806084572));
#52626=CARTESIAN_POINT('Ctrl Pts',(-3.9687184694131,-1.,-1.37020239094614));
#52627=CARTESIAN_POINT('Ctrl Pts',(-3.96560037974645,-1.,-1.37060761745635));
#52628=CARTESIAN_POINT('Ctrl Pts',(-3.96092458506535,-1.,-1.3712051561502));
#52629=CARTESIAN_POINT('Ctrl Pts',(-3.95469287280914,-1.,-1.37198126432386));
#52630=CARTESIAN_POINT('Ctrl Pts',(-3.94690771785133,-1.,-1.37291699202807));
#52631=CARTESIAN_POINT('Ctrl Pts',(-3.93912709040818,-1.,-1.37381821967165));
#52632=CARTESIAN_POINT('Ctrl Pts',(-3.93135106761844,-1.,-1.37468482215751));
#52633=CARTESIAN_POINT('Ctrl Pts',(-3.92357976987672,-1.,-1.37551664448242));
#52634=CARTESIAN_POINT('Ctrl Pts',(-3.91581337462644,-1.,-1.37631350505797));
#52635=CARTESIAN_POINT('Ctrl Pts',(-3.90805209523486,-1.,-1.3770751963402));
#52636=CARTESIAN_POINT('Ctrl Pts',(-3.90029615196727,-1.,-1.37780148512792));
#52637=CARTESIAN_POINT('Ctrl Pts',(-3.89254574338496,-1.,-1.3784921128802));
#52638=CARTESIAN_POINT('Ctrl Pts',(-3.88480102249277,-1.,-1.37914679719383));
#52639=CARTESIAN_POINT('Ctrl Pts',(-3.87706205830532,-1.,-1.37976523097073));
#52640=CARTESIAN_POINT('Ctrl Pts',(-3.86932885813068,-1.,-1.38034709213014));
#52641=CARTESIAN_POINT('Ctrl Pts',(-3.86160143043959,-1.,-1.38089205992989));
#52642=CARTESIAN_POINT('Ctrl Pts',(-3.85387983979481,-1.,-1.38139983115049));
#52643=CARTESIAN_POINT('Ctrl Pts',(-3.84616425605764,-1.,-1.38187013346109));
#52644=CARTESIAN_POINT('Ctrl Pts',(-3.83845502790746,-1.,-1.38230274828821));
#52645=CARTESIAN_POINT('Ctrl Pts',(-3.8307526698229,-1.,-1.38269750245138));
#52646=CARTESIAN_POINT('Ctrl Pts',(-3.82305771743829,-1.,-1.38305421262763));
#52647=CARTESIAN_POINT('Ctrl Pts',(-3.81537060817811,-1.,-1.38337263902782));
#52648=CARTESIAN_POINT('Ctrl Pts',(-3.80769156398411,-1.,-1.3836524404622));
#52649=CARTESIAN_POINT('Ctrl Pts',(-3.80002044322111,-1.,-1.38389311766682));
#52650=CARTESIAN_POINT('Ctrl Pts',(-3.79235669640841,-1.,-1.38409399694566));
#52651=CARTESIAN_POINT('Ctrl Pts',(-3.78469969805082,-1.,-1.38425435883756));
#52652=CARTESIAN_POINT('Ctrl Pts',(-3.77704902230418,-1.,-1.38437354551428));
#52653=CARTESIAN_POINT('Ctrl Pts',(-3.76940473185779,-1.,-1.38445107339518));
#52654=CARTESIAN_POINT('Ctrl Pts',(-3.76176768271367,-1.,-1.3844867525335));
#52655=CARTESIAN_POINT('Ctrl Pts',(-3.7541397631875,-1.,-1.38448077997163));
#52656=CARTESIAN_POINT('Ctrl Pts',(-3.74652317167876,-1.,-1.38443344984394));
#52657=CARTESIAN_POINT('Ctrl Pts',(-3.73891976418104,-1.,-1.38434489156458));
#52658=CARTESIAN_POINT('Ctrl Pts',(-3.73133035859282,-1.,-1.38421479111531));
#52659=CARTESIAN_POINT('Ctrl Pts',(-3.72375409358803,-1.,-1.3840421342895));
#52660=CARTESIAN_POINT('Ctrl Pts',(-3.7161876605181,-1.,-1.38382489984586));
#52661=CARTESIAN_POINT('Ctrl Pts',(-3.70862680753347,-1.,-1.38356065402124));
#52662=CARTESIAN_POINT('Ctrl Pts',(-3.701067921679,-1.,-1.38324717612865));
#52663=CARTESIAN_POINT('Ctrl Pts',(-3.69350967899526,-1.,-1.3828831117165));
#52664=CARTESIAN_POINT('Ctrl Pts',(-3.68595444983837,-1.,-1.38246852827182));
#52665=CARTESIAN_POINT('Ctrl Pts',(-3.67841038482414,-1.,-1.3820057429062));
#52666=CARTESIAN_POINT('Ctrl Pts',(-3.67088843112262,-1.,-1.38149812653868));
#52667=CARTESIAN_POINT('Ctrl Pts',(-3.66339848520857,-1.,-1.38094856333552));
#52668=CARTESIAN_POINT('Ctrl Pts',(-3.6559455440439,-1.,-1.38035791051212));
#52669=CARTESIAN_POINT('Ctrl Pts',(-3.64852652756456,-1.,-1.37972372481603));
#52670=CARTESIAN_POINT('Ctrl Pts',(-3.64112507791141,-1.,-1.37903818567359));
#52671=CARTESIAN_POINT('Ctrl Pts',(-3.63371727442486,-1.,-1.37829035457339));
#52672=CARTESIAN_POINT('Ctrl Pts',(-3.62628098665145,-1.,-1.37746987919881));
#52673=CARTESIAN_POINT('Ctrl Pts',(-3.6188048116042,-1.,-1.37657053403107));
#52674=CARTESIAN_POINT('Ctrl Pts',(-3.61129546591064,-1.,-1.37559314436634));
#52675=CARTESIAN_POINT('Ctrl Pts',(-3.60379020123988,-1.,-1.37455051379623));
#52676=CARTESIAN_POINT('Ctrl Pts',(-3.59634627869048,-1.,-1.37346320103157));
#52677=CARTESIAN_POINT('Ctrl Pts',(-3.58901853846365,-1.,-1.37235053660976));
#52678=CARTESIAN_POINT('Ctrl Pts',(-3.58183885982715,-1.,-1.37122241663062));
#52679=CARTESIAN_POINT('Ctrl Pts',(-3.57479875549486,-1.,-1.37007229485659));
#52680=CARTESIAN_POINT('Ctrl Pts',(-3.5678208030466,-1.,-1.36886584973389));
#52681=CARTESIAN_POINT('Ctrl Pts',(-3.56077662028649,-1.,-1.36754771771233));
#52682=CARTESIAN_POINT('Ctrl Pts',(-3.55353883995949,-1.,-1.3660614545677));
#52683=CARTESIAN_POINT('Ctrl Pts',(-3.54602591832973,-1.,-1.36436666257597));
#52684=CARTESIAN_POINT('Ctrl Pts',(-3.53824396424961,-1.,-1.36245507339307));
#52685=CARTESIAN_POINT('Ctrl Pts',(-3.530344649616,-1.,-1.36037259643734));
#52686=CARTESIAN_POINT('Ctrl Pts',(-3.52261776116748,-1.,-1.35821701528836));
#52687=CARTESIAN_POINT('Ctrl Pts',(-3.51542230699556,-1.,-1.35611275237152));
#52688=CARTESIAN_POINT('Ctrl Pts',(-3.50913227059999,-1.,-1.35419113575956));
#52689=CARTESIAN_POINT('Ctrl Pts',(-3.50408168106261,-1.,-1.35257032843486));
#52690=CARTESIAN_POINT('Ctrl Pts',(-3.5007660381649,-1.,-1.35142377279517));
#52691=CARTESIAN_POINT('Ctrl Pts',(-3.49920025459723,-1.,-1.35080045218587));
#52692=CARTESIAN_POINT('Ctrl Pts',(-3.49861894124827,-1.,-1.35049736560527));
#52693=CARTESIAN_POINT('Ctrl Pts',(-3.49847119623846,-1.,-1.35036670892966));
#52694=CARTESIAN_POINT('Ctrl Pts',(-3.4984457533445,-1.,-1.35032489087101));
#52695=CARTESIAN_POINT('',(-3.42859860294378,-1.,-1.51895082866166));
#52696=CARTESIAN_POINT('Origin',(0.,-1.,0.));
#52697=CARTESIAN_POINT('',(-3.77614523045147,-1.,-1.83867539237861));
#52698=CARTESIAN_POINT('Ctrl Pts',(-3.42859860294378,-1.,-1.51895082866166));
#52699=CARTESIAN_POINT('Ctrl Pts',(-3.42864616361967,-1.,-1.51893924967231));
#52700=CARTESIAN_POINT('Ctrl Pts',(-3.42884302333978,-1.,-1.51895133295017));
#52701=CARTESIAN_POINT('Ctrl Pts',(-3.42946838852728,-1.,-1.51914806898539));
#52702=CARTESIAN_POINT('Ctrl Pts',(-3.43101631893491,-1.,-1.5198144909343));
#52703=CARTESIAN_POINT('Ctrl Pts',(-3.43417156977749,-1.,-1.52134826724227));
#52704=CARTESIAN_POINT('Ctrl Pts',(-3.43888895974182,-1.,-1.52377348950429));
#52705=CARTESIAN_POINT('Ctrl Pts',(-3.44469547527,-1.,-1.52686242875717));
#52706=CARTESIAN_POINT('Ctrl Pts',(-3.45127136828667,-1.,-1.530462444618));
#52707=CARTESIAN_POINT('Ctrl Pts',(-3.45825932955273,-1.,-1.53440195378902));
#52708=CARTESIAN_POINT('Ctrl Pts',(-3.46531752207222,-1.,-1.53851507915533));
#52709=CARTESIAN_POINT('Ctrl Pts',(-3.47217189224576,-1.,-1.54266605398152));
#52710=CARTESIAN_POINT('Ctrl Pts',(-3.47868272898599,-1.,-1.54678009290206));
#52711=CARTESIAN_POINT('Ctrl Pts',(-3.48485155928414,-1.,-1.55084702970382));
#52712=CARTESIAN_POINT('Ctrl Pts',(-3.49076460877317,-1.,-1.5548959590107));
#52713=CARTESIAN_POINT('Ctrl Pts',(-3.49655185179623,-1.,-1.55897703097859));
#52714=CARTESIAN_POINT('Ctrl Pts',(-3.50234321621607,-1.,-1.56314187758689));
#52715=CARTESIAN_POINT('Ctrl Pts',(-3.50821771695427,-1.,-1.56742097575041));
#52716=CARTESIAN_POINT('Ctrl Pts',(-3.51418598431733,-1.,-1.57181569799774));
#52717=CARTESIAN_POINT('Ctrl Pts',(-3.52021847865961,-1.,-1.5763104998818));
#52718=CARTESIAN_POINT('Ctrl Pts',(-3.52626275334899,-1.,-1.58088027227856));
#52719=CARTESIAN_POINT('Ctrl Pts',(-3.53226378147068,-1.,-1.58549906268083));
#52720=CARTESIAN_POINT('Ctrl Pts',(-3.53818616861045,-1.,-1.59014958368725));
#52721=CARTESIAN_POINT('Ctrl Pts',(-3.544024581823,-1.,-1.5948276694975));
#52722=CARTESIAN_POINT('Ctrl Pts',(-3.54979148634426,-1.,-1.59953698113444));
#52723=CARTESIAN_POINT('Ctrl Pts',(-3.55550985096117,-1.,-1.60428584699848));
#52724=CARTESIAN_POINT('Ctrl Pts',(-3.56120432482986,-1.,-1.60908344685459));
#52725=CARTESIAN_POINT('Ctrl Pts',(-3.56689200468404,-1.,-1.61393581747522));
#52726=CARTESIAN_POINT('Ctrl Pts',(-3.57257679609826,-1.,-1.61884340915412));
#52727=CARTESIAN_POINT('Ctrl Pts',(-3.57825455954405,-1.,-1.62380329464851));
#52728=CARTESIAN_POINT('Ctrl Pts',(-3.5839162577435,-1.,-1.62881051550748));
#52729=CARTESIAN_POINT('Ctrl Pts',(-3.58955176627876,-1.,-1.63385971451259));
#52730=CARTESIAN_POINT('Ctrl Pts',(-3.59515368334887,-1.,-1.63894676675349));
#52731=CARTESIAN_POINT('Ctrl Pts',(-3.6007202851384,-1.,-1.6440700438558));
#52732=CARTESIAN_POINT('Ctrl Pts',(-3.60625346556992,-1.,-1.64922952425833));
#52733=CARTESIAN_POINT('Ctrl Pts',(-3.61175734965129,-1.,-1.65442619244327));
#52734=CARTESIAN_POINT('Ctrl Pts',(-3.61723666482457,-1.,-1.65966133399186));
#52735=CARTESIAN_POINT('Ctrl Pts',(-3.62269517989104,-1.,-1.66493585923853));
#52736=CARTESIAN_POINT('Ctrl Pts',(-3.62813422105257,-1.,-1.67024966008037));
#52737=CARTESIAN_POINT('Ctrl Pts',(-3.63355343201211,-1.,-1.67560193613145));
#52738=CARTESIAN_POINT('Ctrl Pts',(-3.63895140887443,-1.,-1.68099146651577));
#52739=CARTESIAN_POINT('Ctrl Pts',(-3.64432638915199,-1.,-1.68641690471455));
#52740=CARTESIAN_POINT('Ctrl Pts',(-3.64967689827393,-1.,-1.691877054817));
#52741=CARTESIAN_POINT('Ctrl Pts',(-3.65500246526798,-1.,-1.69737117722558));
#52742=CARTESIAN_POINT('Ctrl Pts',(-3.6603033877491,-1.,-1.70289888566904));
#52743=CARTESIAN_POINT('Ctrl Pts',(-3.6655804319893,-1.,-1.70846001610983));
#52744=CARTESIAN_POINT('Ctrl Pts',(-3.67083454901629,-1.,-1.71405450210392));
#52745=CARTESIAN_POINT('Ctrl Pts',(-3.67606660374665,-1.,-1.71968225581787));
#52746=CARTESIAN_POINT('Ctrl Pts',(-3.68127704936472,-1.,-1.72534302437003));
#52747=CARTESIAN_POINT('Ctrl Pts',(-3.68646597019188,-1.,-1.73103640956647));
#52748=CARTESIAN_POINT('Ctrl Pts',(-3.69163322647906,-1.,-1.73676193254493));
#52749=CARTESIAN_POINT('Ctrl Pts',(-3.6967785691046,-1.,-1.74251908492589));
#52750=CARTESIAN_POINT('Ctrl Pts',(-3.70190175673422,-1.,-1.74830738046092));
#52751=CARTESIAN_POINT('Ctrl Pts',(-3.70700269736876,-1.,-1.75412641804148));
#52752=CARTESIAN_POINT('Ctrl Pts',(-3.71208146346454,-1.,-1.75997588499021));
#52753=CARTESIAN_POINT('Ctrl Pts',(-3.71713822377675,-1.,-1.76585552124549));
#52754=CARTESIAN_POINT('Ctrl Pts',(-3.72217319911429,-1.,-1.77176509401846));
#52755=CARTESIAN_POINT('Ctrl Pts',(-3.72718661205504,-1.,-1.77770437039606));
#52756=CARTESIAN_POINT('Ctrl Pts',(-3.73217863095022,-1.,-1.78367308442682));
#52757=CARTESIAN_POINT('Ctrl Pts',(-3.73714934729962,-1.,-1.78967092823139));
#52758=CARTESIAN_POINT('Ctrl Pts',(-3.74209880351667,-1.,-1.79569757859041));
#52759=CARTESIAN_POINT('Ctrl Pts',(-3.74702700874954,-1.,-1.80175271485519));
#52760=CARTESIAN_POINT('Ctrl Pts',(-3.75193395888069,-1.,-1.80783603939662));
#52761=CARTESIAN_POINT('Ctrl Pts',(-3.75681965683995,-1.,-1.81394729834032));
#52762=CARTESIAN_POINT('Ctrl Pts',(-3.76168412709652,-1.,-1.82008629694924));
#52763=CARTESIAN_POINT('Ctrl Pts',(-3.76652740355856,-1.,-1.82625289221933));
#52764=CARTESIAN_POINT('Ctrl Pts',(-3.77038509819777,-1.,-1.83120816956515));
#52765=CARTESIAN_POINT('Ctrl Pts',(-3.77326886065484,-1.,-1.83493697935064));
#52766=CARTESIAN_POINT('Ctrl Pts',(-3.77518714458232,-1.,-1.83742834010821));
#52767=CARTESIAN_POINT('Ctrl Pts',(-3.77614523045147,-1.,-1.83867539237861));
#52768=CARTESIAN_POINT('',(-3.70708211654725,-1.,-1.97421938526992));
#52769=CARTESIAN_POINT('',(-3.77614523045147,-1.,-1.83867539237861));
#52770=CARTESIAN_POINT('',(-3.24413672884902,-1.,-1.88097764062542));
#52771=CARTESIAN_POINT('Ctrl Pts',(-3.70708211654725,-1.,-1.97421938526992));
#52772=CARTESIAN_POINT('Ctrl Pts',(-3.7055100813194,-1.,-1.974177276451));
#52773=CARTESIAN_POINT('Ctrl Pts',(-3.70236698911837,-1.,-1.97408973726149));
#52774=CARTESIAN_POINT('Ctrl Pts',(-3.69765528558292,-1.,-1.97394846382288));
#52775=CARTESIAN_POINT('Ctrl Pts',(-3.69137888597855,-1.,-1.97374016224397));
#52776=CARTESIAN_POINT('Ctrl Pts',(-3.68354319913416,-1.,-1.9734465030363));
#52777=CARTESIAN_POINT('Ctrl Pts',(-3.67571738106175,-1.,-1.97311947678035));
#52778=CARTESIAN_POINT('Ctrl Pts',(-3.66790152751984,-1.,-1.9727589719863));
#52779=CARTESIAN_POINT('Ctrl Pts',(-3.66009578166865,-1.,-1.97236485439317));
#52780=CARTESIAN_POINT('Ctrl Pts',(-3.65230034717364,-1.,-1.97193697240645));
#52781=CARTESIAN_POINT('Ctrl Pts',(-3.64451546724221,-1.,-1.97147515441539));
#52782=CARTESIAN_POINT('Ctrl Pts',(-3.63674139590853,-1.,-1.97097920454698));
#52783=CARTESIAN_POINT('Ctrl Pts',(-3.62897836973397,-1.,-1.97044889850518));
#52784=CARTESIAN_POINT('Ctrl Pts',(-3.62122658401722,-1.,-1.96988398129888));
#52785=CARTESIAN_POINT('Ctrl Pts',(-3.61348615496393,-1.,-1.96928416040712));
#52786=CARTESIAN_POINT('Ctrl Pts',(-3.60575714017676,-1.,-1.96864911885775));
#52787=CARTESIAN_POINT('Ctrl Pts',(-3.59803959819725,-1.,-1.96797854118257));
#52788=CARTESIAN_POINT('Ctrl Pts',(-3.5903336402273,-1.,-1.96727213799507));
#52789=CARTESIAN_POINT('Ctrl Pts',(-3.58263947663884,-1.,-1.9665296668894));
#52790=CARTESIAN_POINT('Ctrl Pts',(-3.57495748601088,-1.,-1.96575096652857));
#52791=CARTESIAN_POINT('Ctrl Pts',(-3.56728820357933,-1.,-1.96493594634643));
#52792=CARTESIAN_POINT('Ctrl Pts',(-3.55963218706201,-1.,-1.96408450906868));
#52793=CARTESIAN_POINT('Ctrl Pts',(-3.55198990600929,-1.,-1.96319648628667));
#52794=CARTESIAN_POINT('Ctrl Pts',(-3.54436163300425,-1.,-1.96227157573058));
#52795=CARTESIAN_POINT('Ctrl Pts',(-3.53674730625759,-1.,-1.96130926212661));
#52796=CARTESIAN_POINT('Ctrl Pts',(-3.52914648844289,-1.,-1.96030879411534));
#52797=CARTESIAN_POINT('Ctrl Pts',(-3.52155867431438,-1.,-1.95926936324436));
#52798=CARTESIAN_POINT('Ctrl Pts',(-3.51398354617772,-1.,-1.95819025316768));
#52799=CARTESIAN_POINT('Ctrl Pts',(-3.50642124159913,-1.,-1.95707099606513));
#52800=CARTESIAN_POINT('Ctrl Pts',(-3.49887263575602,-1.,-1.9559115382367));
#52801=CARTESIAN_POINT('Ctrl Pts',(-3.49133956289154,-1.,-1.95471236969653));
#52802=CARTESIAN_POINT('Ctrl Pts',(-3.48382414832648,-1.,-1.95347412486316));
#52803=CARTESIAN_POINT('Ctrl Pts',(-3.47632820495926,-1.,-1.95219722189878));
#52804=CARTESIAN_POINT('Ctrl Pts',(-3.4688525897419,-1.,-1.95088147859876));
#52805=CARTESIAN_POINT('Ctrl Pts',(-3.46139661060959,-1.,-1.94952575850196));
#52806=CARTESIAN_POINT('Ctrl Pts',(-3.45395731584051,-1.,-1.94812754766524));
#52807=CARTESIAN_POINT('Ctrl Pts',(-3.44653088665685,-1.,-1.94668377715332));
#52808=CARTESIAN_POINT('Ctrl Pts',(-3.43911410197693,-1.,-1.94519168842883));
#52809=CARTESIAN_POINT('Ctrl Pts',(-3.43170586602436,-1.,-1.94364973660285));
#52810=CARTESIAN_POINT('Ctrl Pts',(-3.42430850941497,-1.,-1.94205835913692));
#52811=CARTESIAN_POINT('Ctrl Pts',(-3.41692971994082,-1.,-1.94042111965237));
#52812=CARTESIAN_POINT('Ctrl Pts',(-3.40957978266622,-1.,-1.93874306008132));
#52813=CARTESIAN_POINT('Ctrl Pts',(-3.40226802104093,-1.,-1.93702857723089));
#52814=CARTESIAN_POINT('Ctrl Pts',(-3.39499923640789,-1.,-1.93527929945982));
#52815=CARTESIAN_POINT('Ctrl Pts',(-3.38777076883267,-1.,-1.93349233176794));
#52816=CARTESIAN_POINT('Ctrl Pts',(-3.38056768525577,-1.,-1.93165739093292));
#52817=CARTESIAN_POINT('Ctrl Pts',(-3.37336807068078,-1.,-1.92975993109897));
#52818=CARTESIAN_POINT('Ctrl Pts',(-3.36615168657597,-1.,-1.92778626543803));
#52819=CARTESIAN_POINT('Ctrl Pts',(-3.35890824422976,-1.,-1.92572846125763));
#52820=CARTESIAN_POINT('Ctrl Pts',(-3.35164424847206,-1.,-1.92358838440518));
#52821=CARTESIAN_POINT('Ctrl Pts',(-3.34439448941915,-1.,-1.92138450828378));
#52822=CARTESIAN_POINT('Ctrl Pts',(-3.33721230709948,-1.,-1.91914609610173));
#52823=CARTESIAN_POINT('Ctrl Pts',(-3.33014884257812,-1.,-1.91690081930297));
#52824=CARTESIAN_POINT('Ctrl Pts',(-3.32323403454507,-1.,-1.91466343916612));
#52825=CARTESIAN_POINT('Ctrl Pts',(-3.31646052426395,-1.,-1.91242616234459));
#52826=CARTESIAN_POINT('Ctrl Pts',(-3.30975721158694,-1.,-1.91014297830502));
#52827=CARTESIAN_POINT('Ctrl Pts',(-3.30300595568341,-1.,-1.90773912171424));
#52828=CARTESIAN_POINT('Ctrl Pts',(-3.29608978722258,-1.,-1.9051389186417));
#52829=CARTESIAN_POINT('Ctrl Pts',(-3.28893448600364,-1.,-1.9022897124757));
#52830=CARTESIAN_POINT('Ctrl Pts',(-3.28154737912287,-1.,-1.89918429230424));
#52831=CARTESIAN_POINT('Ctrl Pts',(-3.27407108932908,-1.,-1.89589172903662));
#52832=CARTESIAN_POINT('Ctrl Pts',(-3.2667765388833,-1.,-1.89255393500769));
#52833=CARTESIAN_POINT('Ctrl Pts',(-3.2599988519361,-1.,-1.88934996203508));
#52834=CARTESIAN_POINT('Ctrl Pts',(-3.25408686339298,-1.,-1.88646802523372));
#52835=CARTESIAN_POINT('Ctrl Pts',(-3.24935200512055,-1.,-1.88407708646435));
#52836=CARTESIAN_POINT('Ctrl Pts',(-3.24625654410705,-1.,-1.88242596600422));
#52837=CARTESIAN_POINT('Ctrl Pts',(-3.24480754675942,-1.,-1.88156537699118));
#52838=CARTESIAN_POINT('Ctrl Pts',(-3.24428080352952,-1.,-1.88117508446657));
#52839=CARTESIAN_POINT('Ctrl Pts',(-3.24415531671311,-1.,-1.88102292397987));
#52840=CARTESIAN_POINT('Ctrl Pts',(-3.24413672884902,-1.,-1.88097764062542));
#52841=CARTESIAN_POINT('',(-3.14877060440425,-1.,-2.03660101169564));
#52842=CARTESIAN_POINT('Origin',(0.,-1.,0.));
#52843=CARTESIAN_POINT('',(-3.44202241512147,-1.,-2.40675750623143));
#52844=CARTESIAN_POINT('Ctrl Pts',(-3.14877060440425,-1.,-2.03660101169564));
#52845=CARTESIAN_POINT('Ctrl Pts',(-3.1488193908823,-1.,-2.03659701539175));
#52846=CARTESIAN_POINT('Ctrl Pts',(-3.14901193669147,-1.,-2.03663974554941));
#52847=CARTESIAN_POINT('Ctrl Pts',(-3.14959882629936,-1.,-2.03693188810614));
#52848=CARTESIAN_POINT('Ctrl Pts',(-3.15102344775396,-1.,-2.03783225496023));
#52849=CARTESIAN_POINT('Ctrl Pts',(-3.1538999167466,-1.,-2.03984073791432));
#52850=CARTESIAN_POINT('Ctrl Pts',(-3.15817983946525,-1.,-2.04297406404132));
#52851=CARTESIAN_POINT('Ctrl Pts',(-3.16343165059235,-1.,-2.0469333124766));
#52852=CARTESIAN_POINT('Ctrl Pts',(-3.16936341689859,-1.,-2.05151770247452));
#52853=CARTESIAN_POINT('Ctrl Pts',(-3.17564906975592,-1.,-2.05650186773279));
#52854=CARTESIAN_POINT('Ctrl Pts',(-3.18197692964677,-1.,-2.06166849827143));
#52855=CARTESIAN_POINT('Ctrl Pts',(-3.18809755562297,-1.,-2.06684062744065));
#52856=CARTESIAN_POINT('Ctrl Pts',(-3.19388465568113,-1.,-2.07192253497765));
#52857=CARTESIAN_POINT('Ctrl Pts',(-3.19934132835879,-1.,-2.0769044187063));
#52858=CARTESIAN_POINT('Ctrl Pts',(-3.20454818630635,-1.,-2.08182850370816));
#52859=CARTESIAN_POINT('Ctrl Pts',(-3.20962575845433,-1.,-2.08676465517435));
#52860=CARTESIAN_POINT('Ctrl Pts',(-3.2146942960168,-1.,-2.0917841946046));
#52861=CARTESIAN_POINT('Ctrl Pts',(-3.21982707347067,-1.,-2.09692958434933));
#52862=CARTESIAN_POINT('Ctrl Pts',(-3.22503437553496,-1.,-2.10220384298533));
#52863=CARTESIAN_POINT('Ctrl Pts',(-3.23028945793334,-1.,-2.1075869964248));
#52864=CARTESIAN_POINT('Ctrl Pts',(-3.23554444767115,-1.,-2.11304604021784));
#52865=CARTESIAN_POINT('Ctrl Pts',(-3.24074905517282,-1.,-2.11854673326972));
#52866=CARTESIAN_POINT('Ctrl Pts',(-3.24587102613347,-1.,-2.12406646410943));
#52867=CARTESIAN_POINT('Ctrl Pts',(-3.25090574493994,-1.,-2.1296002839681));
#52868=CARTESIAN_POINT('Ctrl Pts',(-3.25586495065027,-1.,-2.13515375878786));
#52869=CARTESIAN_POINT('Ctrl Pts',(-3.26077002641868,-1.,-2.14073870754257));
#52870=CARTESIAN_POINT('Ctrl Pts',(-3.26564388189764,-1.,-2.14636805295663));
#52871=CARTESIAN_POINT('Ctrl Pts',(-3.27050245897244,-1.,-2.15205043199818));
#52872=CARTESIAN_POINT('Ctrl Pts',(-3.27534954469206,-1.,-2.15778690038359));
#52873=CARTESIAN_POINT('Ctrl Pts',(-3.28018150841414,-1.,-2.16357391934434));
#52874=CARTESIAN_POINT('Ctrl Pts',(-3.2849901997973,-1.,-2.16940517773459));
#52875=CARTESIAN_POINT('Ctrl Pts',(-3.28976645712566,-1.,-2.17527380048422));
#52876=CARTESIAN_POINT('Ctrl Pts',(-3.29450361500484,-1.,-2.18117455557062));
#52877=CARTESIAN_POINT('Ctrl Pts',(-3.29920022557635,-1.,-2.18710556500325));
#52878=CARTESIAN_POINT('Ctrl Pts',(-3.30385816281831,-1.,-2.19306710376112));
#52879=CARTESIAN_POINT('Ctrl Pts',(-3.30848134694596,-1.,-2.19906078949924));
#52880=CARTESIAN_POINT('Ctrl Pts',(-3.3130742460895,-1.,-2.20508863150608));
#52881=CARTESIAN_POINT('Ctrl Pts',(-3.31764044024231,-1.,-2.21115211847872));
#52882=CARTESIAN_POINT('Ctrl Pts',(-3.32218125618955,-1.,-2.21725135110889));
#52883=CARTESIAN_POINT('Ctrl Pts',(-3.32669646722871,-1.,-2.22338548312758));
#52884=CARTESIAN_POINT('Ctrl Pts',(-3.33118487773593,-1.,-2.22955308907221));
#52885=CARTESIAN_POINT('Ctrl Pts',(-3.33564495756478,-1.,-2.2357525632881));
#52886=CARTESIAN_POINT('Ctrl Pts',(-3.34007543738044,-1.,-2.24198249391437));
#52887=CARTESIAN_POINT('Ctrl Pts',(-3.34447596770768,-1.,-2.24824207678288));
#52888=CARTESIAN_POINT('Ctrl Pts',(-3.34884690292342,-1.,-2.25453097693524));
#52889=CARTESIAN_POINT('Ctrl Pts',(-3.35318902552676,-1.,-2.26084915222484));
#52890=CARTESIAN_POINT('Ctrl Pts',(-3.35750328523077,-1.,-2.26719668579921));
#52891=CARTESIAN_POINT('Ctrl Pts',(-3.36179055004369,-1.,-2.27357362620902));
#52892=CARTESIAN_POINT('Ctrl Pts',(-3.36605130712978,-1.,-2.27997979457968));
#52893=CARTESIAN_POINT('Ctrl Pts',(-3.37028570206357,-1.,-2.28641481081045));
#52894=CARTESIAN_POINT('Ctrl Pts',(-3.37449367172707,-1.,-2.2928781800731));
#52895=CARTESIAN_POINT('Ctrl Pts',(-3.37867504959382,-1.,-2.29936936127588));
#52896=CARTESIAN_POINT('Ctrl Pts',(-3.38282967336676,-1.,-2.30588783640389));
#52897=CARTESIAN_POINT('Ctrl Pts',(-3.38695751492659,-1.,-2.31243319489505));
#52898=CARTESIAN_POINT('Ctrl Pts',(-3.39105869475112,-1.,-2.31900513925627));
#52899=CARTESIAN_POINT('Ctrl Pts',(-3.39513342020045,-1.,-2.32560343902683));
#52900=CARTESIAN_POINT('Ctrl Pts',(-3.39918194578115,-1.,-2.33222789882601));
#52901=CARTESIAN_POINT('Ctrl Pts',(-3.40320452776646,-1.,-2.33887832342715));
#52902=CARTESIAN_POINT('Ctrl Pts',(-3.40720137403888,-1.,-2.34555447648901));
#52903=CARTESIAN_POINT('Ctrl Pts',(-3.41117262313464,-1.,-2.35225606823649));
#52904=CARTESIAN_POINT('Ctrl Pts',(-3.4151183675076,-1.,-2.35898278606449));
#52905=CARTESIAN_POINT('Ctrl Pts',(-3.41903866635384,-1.,-2.36573431470314));
#52906=CARTESIAN_POINT('Ctrl Pts',(-3.42293356216595,-1.,-2.37251035954351));
#52907=CARTESIAN_POINT('Ctrl Pts',(-3.42680309755241,-1.,-2.37931067029517));
#52908=CARTESIAN_POINT('Ctrl Pts',(-3.43064732714472,-1.,-2.38613505844641));
#52909=CARTESIAN_POINT('Ctrl Pts',(-3.43446630680436,-1.,-2.39298338805823));
#52910=CARTESIAN_POINT('Ctrl Pts',(-3.43750133066036,-1.,-2.39848113411429));
#52911=CARTESIAN_POINT('Ctrl Pts',(-3.43976627485223,-1.,-2.40261515590099));
#52912=CARTESIAN_POINT('Ctrl Pts',(-3.44127120683402,-1.,-2.40537592959345));
#52913=CARTESIAN_POINT('Ctrl Pts',(-3.44202241512147,-1.,-2.40675750623143));
#52914=CARTESIAN_POINT('',(-3.35260583073571,-1.,-2.52982887637028));
#52915=CARTESIAN_POINT('',(-3.44202241512147,-1.,-2.40675750623143));
#52916=CARTESIAN_POINT('',(-2.90994629141676,-1.,-2.36531447826073));
#52917=CARTESIAN_POINT('Ctrl Pts',(-3.35260583073571,-1.,-2.52982887637028));
#52918=CARTESIAN_POINT('Ctrl Pts',(-3.35105973714071,-1.,-2.5295413654909));
#52919=CARTESIAN_POINT('Ctrl Pts',(-3.34796903576663,-1.,-2.52896321610703));
#52920=CARTESIAN_POINT('Ctrl Pts',(-3.34333744115511,-1.,-2.52808660915689));
#52921=CARTESIAN_POINT('Ctrl Pts',(-3.33717089999103,-1.,-2.52689902690158));
#52922=CARTESIAN_POINT('Ctrl Pts',(-3.32947762187533,-1.,-2.52538321164634));
#52923=CARTESIAN_POINT('Ctrl Pts',(-3.32179931078699,-1.,-2.5238359839626));
#52924=CARTESIAN_POINT('Ctrl Pts',(-3.31413607874645,-1.,-2.52225724871313));
#52925=CARTESIAN_POINT('Ctrl Pts',(-3.30648808815442,-1.,-2.52064689568511));
#52926=CARTESIAN_POINT('Ctrl Pts',(-3.29885556388352,-1.,-2.51900480701069));
#52927=CARTESIAN_POINT('Ctrl Pts',(-3.2912387729927,-1.,-2.51733085123797));
#52928=CARTESIAN_POINT('Ctrl Pts',(-3.28363799702982,-1.,-2.51562487464514));
#52929=CARTESIAN_POINT('Ctrl Pts',(-3.27605350473142,-1.,-2.513886692704));
#52930=CARTESIAN_POINT('Ctrl Pts',(-3.26848552888115,-1.,-2.51211608411423));
#52931=CARTESIAN_POINT('Ctrl Pts',(-3.26093423001434,-1.,-2.51031277813486));
#52932=CARTESIAN_POINT('Ctrl Pts',(-3.25339971460982,-1.,-2.50847647070723));
#52933=CARTESIAN_POINT('Ctrl Pts',(-3.24588208983849,-1.,-2.506606859405));
#52934=CARTESIAN_POINT('Ctrl Pts',(-3.23838151080319,-1.,-2.5047036758003));
#52935=CARTESIAN_POINT('Ctrl Pts',(-3.23089822320646,-1.,-2.50276671338111));
#52936=CARTESIAN_POINT('Ctrl Pts',(-3.22343262620503,-1.,-2.50079587201957));
#52937=CARTESIAN_POINT('Ctrl Pts',(-3.21598526261286,-1.,-2.4987911459939));
#52938=CARTESIAN_POINT('Ctrl Pts',(-3.20855669849836,-1.,-2.4967525264737));
#52939=CARTESIAN_POINT('Ctrl Pts',(-3.20114742397588,-1.,-2.49467992057755));
#52940=CARTESIAN_POINT('Ctrl Pts',(-3.19375775555798,-1.,-2.49257307239848));
#52941=CARTESIAN_POINT('Ctrl Pts',(-3.18638771282266,-1.,-2.49043146334059));
#52942=CARTESIAN_POINT('Ctrl Pts',(-3.17903698136622,-1.,-2.48825428288201));
#52943=CARTESIAN_POINT('Ctrl Pts',(-3.17170518863313,-1.,-2.48604065348587));
#52944=CARTESIAN_POINT('Ctrl Pts',(-3.16439213290161,-1.,-2.48378981792725));
#52945=CARTESIAN_POINT('Ctrl Pts',(-3.15709802322739,-1.,-2.48150133566571));
#52946=CARTESIAN_POINT('Ctrl Pts',(-3.14982373241352,-1.,-2.47917529057029));
#52947=CARTESIAN_POINT('Ctrl Pts',(-3.1425709954655,-1.,-2.47681245356109));
#52948=CARTESIAN_POINT('Ctrl Pts',(-3.13534181229295,-1.,-2.47441378371932));
#52949=CARTESIAN_POINT('Ctrl Pts',(-3.12813790805952,-1.,-2.47197997765871));
#52950=CARTESIAN_POINT('Ctrl Pts',(-3.12096015766983,-1.,-2.46951098947469));
#52951=CARTESIAN_POINT('Ctrl Pts',(-3.11380805536122,-1.,-2.46700558843506));
#52952=CARTESIAN_POINT('Ctrl Pts',(-3.1066790790198,-1.,-2.46446082979646));
#52953=CARTESIAN_POINT('Ctrl Pts',(-3.09956993697052,-1.,-2.46187308501884));
#52954=CARTESIAN_POINT('Ctrl Pts',(-3.09247787931887,-1.,-2.4592391256388));
#52955=CARTESIAN_POINT('Ctrl Pts',(-3.08540206545315,-1.,-2.45655725437039));
#52956=CARTESIAN_POINT('Ctrl Pts',(-3.07834472886139,-1.,-2.4538282678779));
#52957=CARTESIAN_POINT('Ctrl Pts',(-3.07131290521297,-1.,-2.45105688854422));
#52958=CARTESIAN_POINT('Ctrl Pts',(-3.06431596421405,-1.,-2.44824970516544));
#52959=CARTESIAN_POINT('Ctrl Pts',(-3.05736242671506,-1.,-2.44541251892556));
#52960=CARTESIAN_POINT('Ctrl Pts',(-3.05045678021504,-1.,-2.44254768923105));
#52961=CARTESIAN_POINT('Ctrl Pts',(-3.04359685040555,-1.,-2.43965194061857));
#52962=CARTESIAN_POINT('Ctrl Pts',(-3.03676949672821,-1.,-2.43671278042414));
#52963=CARTESIAN_POINT('Ctrl Pts',(-3.02995534946978,-1.,-2.43371241361488));
#52964=CARTESIAN_POINT('Ctrl Pts',(-3.02313656036004,-1.,-2.43063415586637));
#52965=CARTESIAN_POINT('Ctrl Pts',(-3.01630420830504,-1.,-2.42746856264168));
#52966=CARTESIAN_POINT('Ctrl Pts',(-3.00946442616658,-1.,-2.42421849439613));
#52967=CARTESIAN_POINT('Ctrl Pts',(-3.00264868585996,-1.,-2.42090763946779));
#52968=CARTESIAN_POINT('Ctrl Pts',(-2.99590509293503,-1.,-2.41757324500514));
#52969=CARTESIAN_POINT('Ctrl Pts',(-2.98927983005796,-1.,-2.41425064199586));
#52970=CARTESIAN_POINT('Ctrl Pts',(-2.98280015815107,-1.,-2.41095909342571));
#52971=CARTESIAN_POINT('Ctrl Pts',(-2.97646002822422,-1.,-2.40768975073713));
#52972=CARTESIAN_POINT('Ctrl Pts',(-2.9701964131236,-1.,-2.40438604734919));
#52973=CARTESIAN_POINT('Ctrl Pts',(-2.96390432240312,-1.,-2.4009556571164));
#52974=CARTESIAN_POINT('Ctrl Pts',(-2.95748006482942,-1.,-2.39730553974517));
#52975=CARTESIAN_POINT('Ctrl Pts',(-2.95085857128439,-1.,-2.39337207631667));
#52976=CARTESIAN_POINT('Ctrl Pts',(-2.94404820669076,-1.,-2.38914929090759));
#52977=CARTESIAN_POINT('Ctrl Pts',(-2.93717903280391,-1.,-2.38472771516311));
#52978=CARTESIAN_POINT('Ctrl Pts',(-2.93049643640206,-1.,-2.38028989582073));
#52979=CARTESIAN_POINT('Ctrl Pts',(-2.92430340582608,-1.,-2.3760651052403));
#52980=CARTESIAN_POINT('Ctrl Pts',(-2.91891503791411,-1.,-2.37229381109821));
#52981=CARTESIAN_POINT('Ctrl Pts',(-2.9146124988314,-1.,-2.36919161373173));
#52982=CARTESIAN_POINT('Ctrl Pts',(-2.91181344022549,-1.,-2.36707658451664));
#52983=CARTESIAN_POINT('Ctrl Pts',(-2.91051690822156,-1.,-2.36599991765749));
#52984=CARTESIAN_POINT('Ctrl Pts',(-2.91005770527719,-1.,-2.36553202948613));
#52985=CARTESIAN_POINT('Ctrl Pts',(-2.90995756655606,-1.,-2.36536211188453));
#52986=CARTESIAN_POINT('Ctrl Pts',(-2.90994629141676,-1.,-2.36531447826074));
#52987=CARTESIAN_POINT('',(-2.79140942341378,-1.,-2.50410331873042));
#52988=CARTESIAN_POINT('Origin',(0.,-1.,0.));
#52989=CARTESIAN_POINT('',(-3.02314558451372,-1.,-2.91557726271063));
#52990=CARTESIAN_POINT('Ctrl Pts',(-2.79140942341378,-1.,-2.50410331873042));
#52991=CARTESIAN_POINT('Ctrl Pts',(-2.79145823440899,-1.,-2.50410700351426));
#52992=CARTESIAN_POINT('Ctrl Pts',(-2.79164172519039,-1.,-2.50417932839343));
#52993=CARTESIAN_POINT('Ctrl Pts',(-2.79217568804874,-1.,-2.50455968395235));
#52994=CARTESIAN_POINT('Ctrl Pts',(-2.79344192164204,-1.,-2.50567182569153));
#52995=CARTESIAN_POINT('Ctrl Pts',(-2.7959687805717,-1.,-2.50810555977564));
#52996=CARTESIAN_POINT('Ctrl Pts',(-2.79970585014308,-1.,-2.51186983687947));
#52997=CARTESIAN_POINT('Ctrl Pts',(-2.80427363984939,-1.,-2.51660190466067));
#52998=CARTESIAN_POINT('Ctrl Pts',(-2.80941521967234,-1.,-2.52205778589922));
#52999=CARTESIAN_POINT('Ctrl Pts',(-2.8148437904867,-1.,-2.52796388055457));
#53000=CARTESIAN_POINT('Ctrl Pts',(-2.82028550483744,-1.,-2.53405679667463));
#53001=CARTESIAN_POINT('Ctrl Pts',(-2.82552167649157,-1.,-2.54012272520141));
#53002=CARTESIAN_POINT('Ctrl Pts',(-2.83044254225794,-1.,-2.54604736792542));
#53003=CARTESIAN_POINT('Ctrl Pts',(-2.83505269592412,-1.,-2.55182152806964));
#53004=CARTESIAN_POINT('Ctrl Pts',(-2.83942515220699,-1.,-2.55749952145165));
#53005=CARTESIAN_POINT('Ctrl Pts',(-2.84366802680211,-1.,-2.56316920798489));
#53006=CARTESIAN_POINT('Ctrl Pts',(-2.84788893329091,-1.,-2.56891984251743));
#53007=CARTESIAN_POINT('Ctrl Pts',(-2.85215360144483,-1.,-2.57480482727128));
#53008=CARTESIAN_POINT('Ctrl Pts',(-2.85647171715147,-1.,-2.58082875254407));
#53009=CARTESIAN_POINT('Ctrl Pts',(-2.86081999003668,-1.,-2.5869677064356));
#53010=CARTESIAN_POINT('Ctrl Pts',(-2.86515629953528,-1.,-2.59318160184921));
#53011=CARTESIAN_POINT('Ctrl Pts',(-2.86943633170712,-1.,-2.59942875223202));
#53012=CARTESIAN_POINT('Ctrl Pts',(-2.87363176656475,-1.,-2.6056817788128));
#53013=CARTESIAN_POINT('Ctrl Pts',(-2.87773881947885,-1.,-2.61193507170928));
#53014=CARTESIAN_POINT('Ctrl Pts',(-2.88176821427502,-1.,-2.61819596473087));
#53015=CARTESIAN_POINT('Ctrl Pts',(-2.88573922195049,-1.,-2.62447947640253));
#53016=CARTESIAN_POINT('Ctrl Pts',(-2.88967244854243,-1.,-2.63080195420771));
#53017=CARTESIAN_POINT('Ctrl Pts',(-2.89358228854557,-1.,-2.63717442263944));
#53018=CARTESIAN_POINT('Ctrl Pts',(-2.89747231723361,-1.,-2.64359851684146));
#53019=CARTESIAN_POINT('Ctrl Pts',(-2.90133950224879,-1.,-2.65007017365576));
#53020=CARTESIAN_POINT('Ctrl Pts',(-2.90517678087467,-1.,-2.65658188464287));
#53021=CARTESIAN_POINT('Ctrl Pts',(-2.90897617968921,-1.,-2.66312542616808));
#53022=CARTESIAN_POINT('Ctrl Pts',(-2.91273193382876,-1.,-2.66969458792627));
#53023=CARTESIAN_POINT('Ctrl Pts',(-2.91644290704281,-1.,-2.67628728855309));
#53024=CARTESIAN_POINT('Ctrl Pts',(-2.92011090722152,-1.,-2.68290409279689));
#53025=CARTESIAN_POINT('Ctrl Pts',(-2.92373955325876,-1.,-2.68954721165342));
#53026=CARTESIAN_POINT('Ctrl Pts',(-2.92733294395268,-1.,-2.69621932864302));
#53027=CARTESIAN_POINT('Ctrl Pts',(-2.93089438233746,-1.,-2.70292247416881));
#53028=CARTESIAN_POINT('Ctrl Pts',(-2.93442516311168,-1.,-2.70965695523776));
#53029=CARTESIAN_POINT('Ctrl Pts',(-2.93792519474955,-1.,-2.71642190053575));
#53030=CARTESIAN_POINT('Ctrl Pts',(-2.94139351933882,-1.,-2.72321571511322));
#53031=CARTESIAN_POINT('Ctrl Pts',(-2.94482887675139,-1.,-2.73003657371613));
#53032=CARTESIAN_POINT('Ctrl Pts',(-2.94823023414381,-1.,-2.73688288329825));
#53033=CARTESIAN_POINT('Ctrl Pts',(-2.95159737214305,-1.,-2.7437537949221));
#53034=CARTESIAN_POINT('Ctrl Pts',(-2.95493069316211,-1.,-2.75064903318996));
#53035=CARTESIAN_POINT('Ctrl Pts',(-2.9582309766594,-1.,-2.75756867888393));
#53036=CARTESIAN_POINT('Ctrl Pts',(-2.96149914764832,-1.,-2.76451296269571));
#53037=CARTESIAN_POINT('Ctrl Pts',(-2.96473605585548,-1.,-2.77148206836464));
#53038=CARTESIAN_POINT('Ctrl Pts',(-2.9679422104295,-1.,-2.77847589542767));
#53039=CARTESIAN_POINT('Ctrl Pts',(-2.97111781461349,-1.,-2.78549409123657));
#53040=CARTESIAN_POINT('Ctrl Pts',(-2.97426288347475,-1.,-2.79253615718147));
#53041=CARTESIAN_POINT('Ctrl Pts',(-2.97737733718242,-1.,-2.79960153278186));
#53042=CARTESIAN_POINT('Ctrl Pts',(-2.98046109647299,-1.,-2.80668968101162));
#53043=CARTESIAN_POINT('Ctrl Pts',(-2.9835141977994,-1.,-2.81380019196454));
#53044=CARTESIAN_POINT('Ctrl Pts',(-2.98653680669434,-1.,-2.82093279065704));
#53045=CARTESIAN_POINT('Ctrl Pts',(-2.98952916401699,-1.,-2.82808728190402));
#53046=CARTESIAN_POINT('Ctrl Pts',(-2.99249155170479,-1.,-2.83526351254383));
#53047=CARTESIAN_POINT('Ctrl Pts',(-2.995424253416,-1.,-2.84246132984334));
#53048=CARTESIAN_POINT('Ctrl Pts',(-2.99832751144566,-1.,-2.84968053289104));
#53049=CARTESIAN_POINT('Ctrl Pts',(-3.0012015079552,-1.,-2.85692085715129));
#53050=CARTESIAN_POINT('Ctrl Pts',(-3.00404638316245,-1.,-2.86418200833065));
#53051=CARTESIAN_POINT('Ctrl Pts',(-3.00686224485374,-1.,-2.87146368430104));
#53052=CARTESIAN_POINT('Ctrl Pts',(-3.0096491810855,-1.,-2.87876560072799));
#53053=CARTESIAN_POINT('Ctrl Pts',(-3.01240727309568,-1.,-2.88608751706796));
#53054=CARTESIAN_POINT('Ctrl Pts',(-3.01513660433291,-1.,-2.8934292556764));
#53055=CARTESIAN_POINT('Ctrl Pts',(-3.01783725123646,-1.,-2.90079069102661));
#53056=CARTESIAN_POINT('Ctrl Pts',(-3.01997487194926,-1.,-2.90669553303902));
#53057=CARTESIAN_POINT('Ctrl Pts',(-3.02156522743299,-1.,-2.91113297349052));
#53058=CARTESIAN_POINT('Ctrl Pts',(-3.02261975104912,-1.,-2.91409518070707));
#53059=CARTESIAN_POINT('Ctrl Pts',(-3.02314558451372,-1.,-2.91557726271063));
#53060=CARTESIAN_POINT('',(-2.91557726271063,-1.,-3.02314558451372));
#53061=CARTESIAN_POINT('',(-3.02314558451372,-1.,-2.91557726271063));
#53062=CARTESIAN_POINT('',(-2.50410331873176,-1.,-2.79140942341258));
#53063=CARTESIAN_POINT('Ctrl Pts',(-2.91557726271063,-1.,-3.02314558451372));
#53064=CARTESIAN_POINT('Ctrl Pts',(-2.91409518070399,-1.,-3.02261975104593));
#53065=CARTESIAN_POINT('Ctrl Pts',(-2.91113297348212,-1.,-3.02156522742431));
#53066=CARTESIAN_POINT('Ctrl Pts',(-2.90669553302526,-1.,-3.01997487193503));
#53067=CARTESIAN_POINT('Ctrl Pts',(-2.9007906910105,-1.,-3.01783725121981));
#53068=CARTESIAN_POINT('Ctrl Pts',(-2.89342925566321,-1.,-3.01513660431928));
#53069=CARTESIAN_POINT('Ctrl Pts',(-2.8860875170608,-1.,-3.01240727308829));
#53070=CARTESIAN_POINT('Ctrl Pts',(-2.87876560072727,-1.,-3.00964918108476));
#53071=CARTESIAN_POINT('Ctrl Pts',(-2.87146368430502,-1.,-3.00686224485784));
#53072=CARTESIAN_POINT('Ctrl Pts',(-2.86418200833667,-1.,-3.00404638316867));
#53073=CARTESIAN_POINT('Ctrl Pts',(-2.85692085715686,-1.,-3.00120150796095));
#53074=CARTESIAN_POINT('Ctrl Pts',(-2.84968053289451,-1.,-2.99832751144925));
#53075=CARTESIAN_POINT('Ctrl Pts',(-2.84246132984415,-1.,-2.99542425341685));
#53076=CARTESIAN_POINT('Ctrl Pts',(-2.83526351254248,-1.,-2.99249155170339));
#53077=CARTESIAN_POINT('Ctrl Pts',(-2.82808728190157,-1.,-2.98952916401446));
#53078=CARTESIAN_POINT('Ctrl Pts',(-2.82093279065457,-1.,-2.9865368066918));
#53079=CARTESIAN_POINT('Ctrl Pts',(-2.81380019196286,-1.,-2.98351419779767));
#53080=CARTESIAN_POINT('Ctrl Pts',(-2.80668968101106,-1.,-2.98046109647241));
#53081=CARTESIAN_POINT('Ctrl Pts',(-2.7996015327823,-1.,-2.97737733718287));
#53082=CARTESIAN_POINT('Ctrl Pts',(-2.79253615718248,-1.,-2.9742628834758));
#53083=CARTESIAN_POINT('Ctrl Pts',(-2.78549409123769,-1.,-2.97111781461465));
#53084=CARTESIAN_POINT('Ctrl Pts',(-2.7784758954285,-1.,-2.96794221043036));
#53085=CARTESIAN_POINT('Ctrl Pts',(-2.77148206836498,-1.,-2.96473605585583));
#53086=CARTESIAN_POINT('Ctrl Pts',(-2.76451296269557,-1.,-2.96149914764818));
#53087=CARTESIAN_POINT('Ctrl Pts',(-2.7575686788835,-1.,-2.95823097665896));
#53088=CARTESIAN_POINT('Ctrl Pts',(-2.75064903318947,-1.,-2.95493069316161));
#53089=CARTESIAN_POINT('Ctrl Pts',(-2.74375379492172,-1.,-2.95159737214266));
#53090=CARTESIAN_POINT('Ctrl Pts',(-2.73688288329808,-1.,-2.94823023414364));
#53091=CARTESIAN_POINT('Ctrl Pts',(-2.73003657371617,-1.,-2.94482887675143));
#53092=CARTESIAN_POINT('Ctrl Pts',(-2.72321571511337,-1.,-2.94139351933897));
#53093=CARTESIAN_POINT('Ctrl Pts',(-2.71642190053592,-1.,-2.93792519474972));
#53094=CARTESIAN_POINT('Ctrl Pts',(-2.70965695523787,-1.,-2.93442516311179));
#53095=CARTESIAN_POINT('Ctrl Pts',(-2.70292247416885,-1.,-2.93089438233749));
#53096=CARTESIAN_POINT('Ctrl Pts',(-2.69621932864301,-1.,-2.92733294395267));
#53097=CARTESIAN_POINT('Ctrl Pts',(-2.68954721165339,-1.,-2.92373955325875));
#53098=CARTESIAN_POINT('Ctrl Pts',(-2.68290409279688,-1.,-2.92011090722152));
#53099=CARTESIAN_POINT('Ctrl Pts',(-2.67628728855312,-1.,-2.91644290704285));
#53100=CARTESIAN_POINT('Ctrl Pts',(-2.66969458792631,-1.,-2.91273193382882));
#53101=CARTESIAN_POINT('Ctrl Pts',(-2.6631254261681,-1.,-2.90897617968923));
#53102=CARTESIAN_POINT('Ctrl Pts',(-2.65658188464282,-1.,-2.90517678087461));
#53103=CARTESIAN_POINT('Ctrl Pts',(-2.65007017365564,-1.,-2.90133950224867));
#53104=CARTESIAN_POINT('Ctrl Pts',(-2.64359851684131,-1.,-2.89747231723345));
#53105=CARTESIAN_POINT('Ctrl Pts',(-2.63717442263932,-1.,-2.89358228854544));
#53106=CARTESIAN_POINT('Ctrl Pts',(-2.63080195420767,-1.,-2.88967244854239));
#53107=CARTESIAN_POINT('Ctrl Pts',(-2.62447947640262,-1.,-2.88573922195059));
#53108=CARTESIAN_POINT('Ctrl Pts',(-2.61819596473108,-1.,-2.88176821427525));
#53109=CARTESIAN_POINT('Ctrl Pts',(-2.61193507170955,-1.,-2.87773881947915));
#53110=CARTESIAN_POINT('Ctrl Pts',(-2.60568177881303,-1.,-2.87363176656501));
#53111=CARTESIAN_POINT('Ctrl Pts',(-2.5994287522321,-1.,-2.86943633170722));
#53112=CARTESIAN_POINT('Ctrl Pts',(-2.59318160184908,-1.,-2.86515629953513));
#53113=CARTESIAN_POINT('Ctrl Pts',(-2.58696770643524,-1.,-2.86081999003629));
#53114=CARTESIAN_POINT('Ctrl Pts',(-2.58082875254357,-1.,-2.85647171715092));
#53115=CARTESIAN_POINT('Ctrl Pts',(-2.57480482727081,-1.,-2.85215360144431));
#53116=CARTESIAN_POINT('Ctrl Pts',(-2.56891984251721,-1.,-2.84788893329067));
#53117=CARTESIAN_POINT('Ctrl Pts',(-2.56316920798513,-1.,-2.84366802680237));
#53118=CARTESIAN_POINT('Ctrl Pts',(-2.55749952145241,-1.,-2.83942515220782));
#53119=CARTESIAN_POINT('Ctrl Pts',(-2.55182152807077,-1.,-2.83505269592536));
#53120=CARTESIAN_POINT('Ctrl Pts',(-2.54604736792655,-1.,-2.83044254225917));
#53121=CARTESIAN_POINT('Ctrl Pts',(-2.54012272520199,-1.,-2.8255216764922));
#53122=CARTESIAN_POINT('Ctrl Pts',(-2.53405679667412,-1.,-2.82028550483689));
#53123=CARTESIAN_POINT('Ctrl Pts',(-2.52796388055278,-1.,-2.81484379048475));
#53124=CARTESIAN_POINT('Ctrl Pts',(-2.52205778589653,-1.,-2.80941521966941));
#53125=CARTESIAN_POINT('Ctrl Pts',(-2.51660190465805,-1.,-2.80427363984653));
#53126=CARTESIAN_POINT('Ctrl Pts',(-2.51186983687818,-1.,-2.79970585014168));
#53127=CARTESIAN_POINT('Ctrl Pts',(-2.50810555977671,-1.,-2.79596878057287));
#53128=CARTESIAN_POINT('Ctrl Pts',(-2.50567182569081,-1.,-2.79344192164147));
#53129=CARTESIAN_POINT('Ctrl Pts',(-2.50455968395146,-1.,-2.79217568804755));
#53130=CARTESIAN_POINT('Ctrl Pts',(-2.50417932839313,-1.,-2.79164172518905));
#53131=CARTESIAN_POINT('Ctrl Pts',(-2.50410700351493,-1.,-2.79145823440781));
#53132=CARTESIAN_POINT('Ctrl Pts',(-2.50410331873176,-1.,-2.79140942341258));
#53133=CARTESIAN_POINT('',(-2.36531447826213,-1.,-2.90994629141562));
#53134=CARTESIAN_POINT('Origin',(0.,-1.,0.));
#53135=CARTESIAN_POINT('',(-2.52982887637028,-1.,-3.35260583073571));
#53136=CARTESIAN_POINT('Ctrl Pts',(-2.36531447826213,-1.,-2.90994629141562));
#53137=CARTESIAN_POINT('Ctrl Pts',(-2.3653621118858,-1.,-2.90995756655558));
#53138=CARTESIAN_POINT('Ctrl Pts',(-2.36553202948741,-1.,-2.9100577052777));
#53139=CARTESIAN_POINT('Ctrl Pts',(-2.36599991765853,-1.,-2.91051690822262));
#53140=CARTESIAN_POINT('Ctrl Pts',(-2.36707658451709,-1.,-2.91181344022628));
#53141=CARTESIAN_POINT('Ctrl Pts',(-2.36919161373074,-1.,-2.91461249883016));
#53142=CARTESIAN_POINT('Ctrl Pts',(-2.37229381109939,-1.,-2.9189150379156));
#53143=CARTESIAN_POINT('Ctrl Pts',(-2.37606510524271,-1.,-2.92430340582912));
#53144=CARTESIAN_POINT('Ctrl Pts',(-2.3802898958232,-1.,-2.93049643640517));
#53145=CARTESIAN_POINT('Ctrl Pts',(-2.38472771516476,-1.,-2.93717903280599));
#53146=CARTESIAN_POINT('Ctrl Pts',(-2.38914929090806,-1.,-2.94404820669135));
#53147=CARTESIAN_POINT('Ctrl Pts',(-2.39337207631613,-1.,-2.95085857128372));
#53148=CARTESIAN_POINT('Ctrl Pts',(-2.39730553974412,-1.,-2.95748006482811));
#53149=CARTESIAN_POINT('Ctrl Pts',(-2.40095565711535,-1.,-2.96390432240181));
#53150=CARTESIAN_POINT('Ctrl Pts',(-2.40438604734848,-1.,-2.97019641312272));
#53151=CARTESIAN_POINT('Ctrl Pts',(-2.40768975073691,-1.,-2.97646002822395));
#53152=CARTESIAN_POINT('Ctrl Pts',(-2.41095909342591,-1.,-2.98280015815132));
#53153=CARTESIAN_POINT('Ctrl Pts',(-2.4142506419963,-1.,-2.98927983005851));
#53154=CARTESIAN_POINT('Ctrl Pts',(-2.4175732450056,-1.,-2.99590509293561));
#53155=CARTESIAN_POINT('Ctrl Pts',(-2.42090763946812,-1.,-3.00264868586038));
#53156=CARTESIAN_POINT('Ctrl Pts',(-2.42421849439625,-1.,-3.00946442616674));
#53157=CARTESIAN_POINT('Ctrl Pts',(-2.4274685626416,-1.,-3.01630420830494));
#53158=CARTESIAN_POINT('Ctrl Pts',(-2.43063415586615,-1.,-3.02313656035977));
#53159=CARTESIAN_POINT('Ctrl Pts',(-2.43371241361462,-1.,-3.02995534946946));
#53160=CARTESIAN_POINT('Ctrl Pts',(-2.43671278042394,-1.,-3.03676949672797));
#53161=CARTESIAN_POINT('Ctrl Pts',(-2.43965194061849,-1.,-3.04359685040545));
#53162=CARTESIAN_POINT('Ctrl Pts',(-2.44254768923109,-1.,-3.05045678021509));
#53163=CARTESIAN_POINT('Ctrl Pts',(-2.44541251892568,-1.,-3.05736242671521));
#53164=CARTESIAN_POINT('Ctrl Pts',(-2.44824970516558,-1.,-3.06431596421422));
#53165=CARTESIAN_POINT('Ctrl Pts',(-2.45105688854432,-1.,-3.0713129052131));
#53166=CARTESIAN_POINT('Ctrl Pts',(-2.45382826787795,-1.,-3.07834472886145));
#53167=CARTESIAN_POINT('Ctrl Pts',(-2.45655725437037,-1.,-3.08540206545313));
#53168=CARTESIAN_POINT('Ctrl Pts',(-2.45923912563875,-1.,-3.09247787931881));
#53169=CARTESIAN_POINT('Ctrl Pts',(-2.4618730850188,-1.,-3.09956993697048));
#53170=CARTESIAN_POINT('Ctrl Pts',(-2.46446082979645,-1.,-3.10667907901981));
#53171=CARTESIAN_POINT('Ctrl Pts',(-2.46700558843507,-1.,-3.11380805536124));
#53172=CARTESIAN_POINT('Ctrl Pts',(-2.4695109894747,-1.,-3.12096015766984));
#53173=CARTESIAN_POINT('Ctrl Pts',(-2.47197997765868,-1.,-3.12813790805948));
#53174=CARTESIAN_POINT('Ctrl Pts',(-2.47441378371923,-1.,-3.13534181229282));
#53175=CARTESIAN_POINT('Ctrl Pts',(-2.47681245356095,-1.,-3.14257099546531));
#53176=CARTESIAN_POINT('Ctrl Pts',(-2.47917529057016,-1.,-3.14982373241335));
#53177=CARTESIAN_POINT('Ctrl Pts',(-2.48150133566568,-1.,-3.15709802322735));
#53178=CARTESIAN_POINT('Ctrl Pts',(-2.48378981792739,-1.,-3.16439213290181));
#53179=CARTESIAN_POINT('Ctrl Pts',(-2.48604065348619,-1.,-3.17170518863357));
#53180=CARTESIAN_POINT('Ctrl Pts',(-2.48825428288243,-1.,-3.17903698136679));
#53181=CARTESIAN_POINT('Ctrl Pts',(-2.49043146334095,-1.,-3.18638771282315));
#53182=CARTESIAN_POINT('Ctrl Pts',(-2.4925730723986,-1.,-3.19375775555814));
#53183=CARTESIAN_POINT('Ctrl Pts',(-2.49467992057726,-1.,-3.20114742397549));
#53184=CARTESIAN_POINT('Ctrl Pts',(-2.49675252647298,-1.,-3.2085566984974));
#53185=CARTESIAN_POINT('Ctrl Pts',(-2.49879114599293,-1.,-3.21598526261157));
#53186=CARTESIAN_POINT('Ctrl Pts',(-2.5007958720187,-1.,-3.22343262620387));
#53187=CARTESIAN_POINT('Ctrl Pts',(-2.50276671338074,-1.,-3.23089822320596));
#53188=CARTESIAN_POINT('Ctrl Pts',(-2.50470367580078,-1.,-3.23838151080383));
#53189=CARTESIAN_POINT('Ctrl Pts',(-2.50660685940645,-1.,-3.24588208984042));
#53190=CARTESIAN_POINT('Ctrl Pts',(-2.50847647070936,-1.,-3.25339971461265));
#53191=CARTESIAN_POINT('Ctrl Pts',(-2.51031277813697,-1.,-3.26093423001716));
#53192=CARTESIAN_POINT('Ctrl Pts',(-2.51211608411539,-1.,-3.26848552888271));
#53193=CARTESIAN_POINT('Ctrl Pts',(-2.51388669270329,-1.,-3.27605350473048));
#53194=CARTESIAN_POINT('Ctrl Pts',(-2.51562487464215,-1.,-3.28363799702583));
#53195=CARTESIAN_POINT('Ctrl Pts',(-2.51733085123316,-1.,-3.2912387729863));
#53196=CARTESIAN_POINT('Ctrl Pts',(-2.51900480700548,-1.,-3.29885556387661));
#53197=CARTESIAN_POINT('Ctrl Pts',(-2.52064689568167,-1.,-3.30648808814986));
#53198=CARTESIAN_POINT('Ctrl Pts',(-2.52225724871375,-1.,-3.31413607874727));
#53199=CARTESIAN_POINT('Ctrl Pts',(-2.52383598396878,-1.,-3.32179931079521));
#53200=CARTESIAN_POINT('Ctrl Pts',(-2.52538321165774,-1.,-3.32947762189049));
#53201=CARTESIAN_POINT('Ctrl Pts',(-2.52689902691551,-1.,-3.33717090000955));
#53202=CARTESIAN_POINT('Ctrl Pts',(-2.52808660916879,-1.,-3.34333744117093));
#53203=CARTESIAN_POINT('Ctrl Pts',(-2.5289632161143,-1.,-3.34796903577628));
#53204=CARTESIAN_POINT('Ctrl Pts',(-2.52954136549357,-1.,-3.35105973714426));
#53205=CARTESIAN_POINT('Ctrl Pts',(-2.52982887637028,-1.,-3.35260583073571));
#53206=CARTESIAN_POINT('',(-2.40675750623143,-1.,-3.44202241512147));
#53207=CARTESIAN_POINT('',(-2.52982887637028,-1.,-3.35260583073571));
#53208=CARTESIAN_POINT('',(-2.03660101169715,-1.,-3.14877060440327));
#53209=CARTESIAN_POINT('Ctrl Pts',(-2.40675750623143,-1.,-3.44202241512147));
#53210=CARTESIAN_POINT('Ctrl Pts',(-2.4053759295909,-1.,-3.44127120683039));
#53211=CARTESIAN_POINT('Ctrl Pts',(-2.40261515589405,-1.,-3.43976627484234));
#53212=CARTESIAN_POINT('Ctrl Pts',(-2.39848113410292,-1.,-3.43750133064416));
#53213=CARTESIAN_POINT('Ctrl Pts',(-2.39298338804493,-1.,-3.4344663067854));
#53214=CARTESIAN_POINT('Ctrl Pts',(-2.38613505843552,-1.,-3.4306473271292));
#53215=CARTESIAN_POINT('Ctrl Pts',(-2.37931067028926,-1.,-3.42680309754399));
#53216=CARTESIAN_POINT('Ctrl Pts',(-2.37251035954292,-1.,-3.42293356216511));
#53217=CARTESIAN_POINT('Ctrl Pts',(-2.36573431470642,-1.,-3.41903866635852));
#53218=CARTESIAN_POINT('Ctrl Pts',(-2.35898278606946,-1.,-3.41511836751469));
#53219=CARTESIAN_POINT('Ctrl Pts',(-2.35225606824109,-1.,-3.41117262314119));
#53220=CARTESIAN_POINT('Ctrl Pts',(-2.34555447649188,-1.,-3.40720137404297));
#53221=CARTESIAN_POINT('Ctrl Pts',(-2.33887832342782,-1.,-3.40320452776743));
#53222=CARTESIAN_POINT('Ctrl Pts',(-2.33222789882489,-1.,-3.39918194577956));
#53223=CARTESIAN_POINT('Ctrl Pts',(-2.3256034390248,-1.,-3.39513342019756));
#53224=CARTESIAN_POINT('Ctrl Pts',(-2.31900513925424,-1.,-3.39105869474822));
#53225=CARTESIAN_POINT('Ctrl Pts',(-2.31243319489367,-1.,-3.38695751492462));
#53226=CARTESIAN_POINT('Ctrl Pts',(-2.30588783640343,-1.,-3.3828296733661));
#53227=CARTESIAN_POINT('Ctrl Pts',(-2.29936936127624,-1.,-3.37867504959433));
#53228=CARTESIAN_POINT('Ctrl Pts',(-2.29287818007393,-1.,-3.37449367172826));
#53229=CARTESIAN_POINT('Ctrl Pts',(-2.28641481081137,-1.,-3.37028570206488));
#53230=CARTESIAN_POINT('Ctrl Pts',(-2.27997979458037,-1.,-3.36605130713076));
#53231=CARTESIAN_POINT('Ctrl Pts',(-2.2735736262093,-1.,-3.36179055004409));
#53232=CARTESIAN_POINT('Ctrl Pts',(-2.2671966857991,-1.,-3.35750328523061));
#53233=CARTESIAN_POINT('Ctrl Pts',(-2.26084915222449,-1.,-3.35318902552626));
#53234=CARTESIAN_POINT('Ctrl Pts',(-2.25453097693483,-1.,-3.34884690292285));
#53235=CARTESIAN_POINT('Ctrl Pts',(-2.24824207678256,-1.,-3.34447596770723));
#53236=CARTESIAN_POINT('Ctrl Pts',(-2.24198249391422,-1.,-3.34007543738025));
#53237=CARTESIAN_POINT('Ctrl Pts',(-2.23575256328812,-1.,-3.33564495756482));
#53238=CARTESIAN_POINT('Ctrl Pts',(-2.22955308907233,-1.,-3.33118487773611));
#53239=CARTESIAN_POINT('Ctrl Pts',(-2.22338548312772,-1.,-3.3266964672289));
#53240=CARTESIAN_POINT('Ctrl Pts',(-2.21725135110898,-1.,-3.32218125618968));
#53241=CARTESIAN_POINT('Ctrl Pts',(-2.21115211847875,-1.,-3.31764044024235));
#53242=CARTESIAN_POINT('Ctrl Pts',(-2.20508863150607,-1.,-3.31307424608949));
#53243=CARTESIAN_POINT('Ctrl Pts',(-2.19906078949923,-1.,-3.30848134694595));
#53244=CARTESIAN_POINT('Ctrl Pts',(-2.19306710376111,-1.,-3.30385816281831));
#53245=CARTESIAN_POINT('Ctrl Pts',(-2.18710556500327,-1.,-3.29920022557639));
#53246=CARTESIAN_POINT('Ctrl Pts',(-2.18117455557065,-1.,-3.2945036150049));
#53247=CARTESIAN_POINT('Ctrl Pts',(-2.17527380048423,-1.,-3.28976645712568));
#53248=CARTESIAN_POINT('Ctrl Pts',(-2.16940517773455,-1.,-3.28499019979724));
#53249=CARTESIAN_POINT('Ctrl Pts',(-2.16357391934425,-1.,-3.280181508414));
#53250=CARTESIAN_POINT('Ctrl Pts',(-2.15778690038347,-1.,-3.27534954469187));
#53251=CARTESIAN_POINT('Ctrl Pts',(-2.15205043199808,-1.,-3.27050245897228));
#53252=CARTESIAN_POINT('Ctrl Pts',(-2.1463680529566,-1.,-3.26564388189759));
#53253=CARTESIAN_POINT('Ctrl Pts',(-2.14073870754264,-1.,-3.26077002641879));
#53254=CARTESIAN_POINT('Ctrl Pts',(-2.13515375878803,-1.,-3.25586495065054));
#53255=CARTESIAN_POINT('Ctrl Pts',(-2.12960028396832,-1.,-3.25090574494028));
#53256=CARTESIAN_POINT('Ctrl Pts',(-2.12406646410962,-1.,-3.24587102613376));
#53257=CARTESIAN_POINT('Ctrl Pts',(-2.11854673326979,-1.,-3.24074905517293));
#53258=CARTESIAN_POINT('Ctrl Pts',(-2.11304604021773,-1.,-3.23554444767099));
#53259=CARTESIAN_POINT('Ctrl Pts',(-2.10758699642451,-1.,-3.23028945793289));
#53260=CARTESIAN_POINT('Ctrl Pts',(-2.10220384298492,-1.,-3.22503437553434));
#53261=CARTESIAN_POINT('Ctrl Pts',(-2.09692958434895,-1.,-3.21982707347009));
#53262=CARTESIAN_POINT('Ctrl Pts',(-2.09178419460443,-1.,-3.21469429601654));
#53263=CARTESIAN_POINT('Ctrl Pts',(-2.08676465517455,-1.,-3.20962575845463));
#53264=CARTESIAN_POINT('Ctrl Pts',(-2.08182850370878,-1.,-3.2045481863073));
#53265=CARTESIAN_POINT('Ctrl Pts',(-2.07690441870722,-1.,-3.19934132836019));
#53266=CARTESIAN_POINT('Ctrl Pts',(-2.07192253497857,-1.,-3.19388465568252));
#53267=CARTESIAN_POINT('Ctrl Pts',(-2.06684062744112,-1.,-3.18809755562368));
#53268=CARTESIAN_POINT('Ctrl Pts',(-2.06166849827101,-1.,-3.18197692964614));
#53269=CARTESIAN_POINT('Ctrl Pts',(-2.05650186773132,-1.,-3.17564906975371));
#53270=CARTESIAN_POINT('Ctrl Pts',(-2.05151770247233,-1.,-3.16936341689527));
#53271=CARTESIAN_POINT('Ctrl Pts',(-2.04693331247446,-1.,-3.16343165058912));
#53272=CARTESIAN_POINT('Ctrl Pts',(-2.04297406404027,-1.,-3.15817983946367));
#53273=CARTESIAN_POINT('Ctrl Pts',(-2.03984073791519,-1.,-3.15389991674792));
#53274=CARTESIAN_POINT('Ctrl Pts',(-2.03783225495961,-1.,-3.15102344775328));
#53275=CARTESIAN_POINT('Ctrl Pts',(-2.03693188810544,-1.,-3.14959882629805));
#53276=CARTESIAN_POINT('Ctrl Pts',(-2.03663974554932,-1.,-3.1490119366901));
#53277=CARTESIAN_POINT('Ctrl Pts',(-2.03659701539259,-1.,-3.14881939088124));
#53278=CARTESIAN_POINT('Ctrl Pts',(-2.03660101169715,-1.,-3.14877060440328));
#53279=CARTESIAN_POINT('',(-1.88097764062697,-1.,-3.24413672884812));
#53280=CARTESIAN_POINT('Origin',(0.,-1.,0.));
#53281=CARTESIAN_POINT('',(-1.97421938526992,-1.,-3.70708211654725));
#53282=CARTESIAN_POINT('Ctrl Pts',(-1.88097764062697,-1.,-3.24413672884812));
#53283=CARTESIAN_POINT('Ctrl Pts',(-1.8810229239812,-1.,-3.24415531671284));
#53284=CARTESIAN_POINT('Ctrl Pts',(-1.88117508446775,-1.,-3.24428080353022));
#53285=CARTESIAN_POINT('Ctrl Pts',(-1.88156537699203,-1.,-3.24480754676064));
#53286=CARTESIAN_POINT('Ctrl Pts',(-1.88242596600454,-1.,-3.2462565441079));
#53287=CARTESIAN_POINT('Ctrl Pts',(-1.88407708646357,-1.,-3.24935200511918));
#53288=CARTESIAN_POINT('Ctrl Pts',(-1.88646802523466,-1.,-3.25408686339463));
#53289=CARTESIAN_POINT('Ctrl Pts',(-1.88934996203698,-1.,-3.25999885193947));
#53290=CARTESIAN_POINT('Ctrl Pts',(-1.89255393500965,-1.,-3.26677653888676));
#53291=CARTESIAN_POINT('Ctrl Pts',(-1.89589172903793,-1.,-3.27407108933139));
#53292=CARTESIAN_POINT('Ctrl Pts',(-1.89918429230462,-1.,-3.28154737912352));
#53293=CARTESIAN_POINT('Ctrl Pts',(-1.90228971247527,-1.,-3.2889344860029));
#53294=CARTESIAN_POINT('Ctrl Pts',(-1.90513891864087,-1.,-3.29608978722113));
#53295=CARTESIAN_POINT('Ctrl Pts',(-1.90773912171341,-1.,-3.30300595568195));
#53296=CARTESIAN_POINT('Ctrl Pts',(-1.91014297830446,-1.,-3.30975721158596));
#53297=CARTESIAN_POINT('Ctrl Pts',(-1.91242616234442,-1.,-3.31646052426364));
#53298=CARTESIAN_POINT('Ctrl Pts',(-1.91466343916628,-1.,-3.32323403454535));
#53299=CARTESIAN_POINT('Ctrl Pts',(-1.91690081930331,-1.,-3.33014884257873));
#53300=CARTESIAN_POINT('Ctrl Pts',(-1.9191460961021,-1.,-3.33721230710012));
#53301=CARTESIAN_POINT('Ctrl Pts',(-1.92138450828404,-1.,-3.34439448941961));
#53302=CARTESIAN_POINT('Ctrl Pts',(-1.92358838440528,-1.,-3.35164424847223));
#53303=CARTESIAN_POINT('Ctrl Pts',(-1.92572846125756,-1.,-3.35890824422965));
#53304=CARTESIAN_POINT('Ctrl Pts',(-1.92778626543786,-1.,-3.36615168657567));
#53305=CARTESIAN_POINT('Ctrl Pts',(-1.92975993109877,-1.,-3.37336807068043));
#53306=CARTESIAN_POINT('Ctrl Pts',(-1.93165739093276,-1.,-3.3805676852555));
#53307=CARTESIAN_POINT('Ctrl Pts',(-1.93349233176788,-1.,-3.38777076883256));
#53308=CARTESIAN_POINT('Ctrl Pts',(-1.93527929945985,-1.,-3.39499923640795));
#53309=CARTESIAN_POINT('Ctrl Pts',(-1.93702857723098,-1.,-3.40226802104109));
#53310=CARTESIAN_POINT('Ctrl Pts',(-1.93874306008143,-1.,-3.40957978266642));
#53311=CARTESIAN_POINT('Ctrl Pts',(-1.94042111965246,-1.,-3.41692971994096));
#53312=CARTESIAN_POINT('Ctrl Pts',(-1.94205835913696,-1.,-3.42430850941503));
#53313=CARTESIAN_POINT('Ctrl Pts',(-1.94364973660284,-1.,-3.43170586602434));
#53314=CARTESIAN_POINT('Ctrl Pts',(-1.94519168842879,-1.,-3.43911410197687));
#53315=CARTESIAN_POINT('Ctrl Pts',(-1.94668377715329,-1.,-3.44653088665681));
#53316=CARTESIAN_POINT('Ctrl Pts',(-1.94812754766524,-1.,-3.45395731584051));
#53317=CARTESIAN_POINT('Ctrl Pts',(-1.94952575850197,-1.,-3.46139661060962));
#53318=CARTESIAN_POINT('Ctrl Pts',(-1.95088147859877,-1.,-3.46885258974191));
#53319=CARTESIAN_POINT('Ctrl Pts',(-1.95219722189876,-1.,-3.47632820495921));
#53320=CARTESIAN_POINT('Ctrl Pts',(-1.95347412486309,-1.,-3.48382414832634));
#53321=CARTESIAN_POINT('Ctrl Pts',(-1.95471236969643,-1.,-3.49133956289133));
#53322=CARTESIAN_POINT('Ctrl Pts',(-1.95591153823661,-1.,-3.49887263575583));
#53323=CARTESIAN_POINT('Ctrl Pts',(-1.95707099606511,-1.,-3.50642124159909));
#53324=CARTESIAN_POINT('Ctrl Pts',(-1.95819025316779,-1.,-3.51398354617794));
#53325=CARTESIAN_POINT('Ctrl Pts',(-1.95926936324461,-1.,-3.52155867431486));
#53326=CARTESIAN_POINT('Ctrl Pts',(-1.96030879411566,-1.,-3.52914648844351));
#53327=CARTESIAN_POINT('Ctrl Pts',(-1.96130926212689,-1.,-3.53674730625813));
#53328=CARTESIAN_POINT('Ctrl Pts',(-1.96227157573067,-1.,-3.54436163300443));
#53329=CARTESIAN_POINT('Ctrl Pts',(-1.96319648628644,-1.,-3.55198990600886));
#53330=CARTESIAN_POINT('Ctrl Pts',(-1.96408450906812,-1.,-3.55963218706096));
#53331=CARTESIAN_POINT('Ctrl Pts',(-1.96493594634567,-1.,-3.56728820357791));
#53332=CARTESIAN_POINT('Ctrl Pts',(-1.96575096652789,-1.,-3.57495748600959));
#53333=CARTESIAN_POINT('Ctrl Pts',(-1.96652966688911,-1.,-3.58263947663829));
#53334=CARTESIAN_POINT('Ctrl Pts',(-1.96727213799544,-1.,-3.59033364022801));
#53335=CARTESIAN_POINT('Ctrl Pts',(-1.96797854118369,-1.,-3.59803959819938));
#53336=CARTESIAN_POINT('Ctrl Pts',(-1.9686491188594,-1.,-3.60575714017989));
#53337=CARTESIAN_POINT('Ctrl Pts',(-1.96928416040877,-1.,-3.61348615496704));
#53338=CARTESIAN_POINT('Ctrl Pts',(-1.96988398129978,-1.,-3.62122658401893));
#53339=CARTESIAN_POINT('Ctrl Pts',(-1.97044889850463,-1.,-3.62897836973293));
#53340=CARTESIAN_POINT('Ctrl Pts',(-1.97097920454464,-1.,-3.63674139590412));
#53341=CARTESIAN_POINT('Ctrl Pts',(-1.97147515441164,-1.,-3.64451546723514));
#53342=CARTESIAN_POINT('Ctrl Pts',(-1.9719369724024,-1.,-3.652300347166));
#53343=CARTESIAN_POINT('Ctrl Pts',(-1.9723648543905,-1.,-3.6600957816636));
#53344=CARTESIAN_POINT('Ctrl Pts',(-1.97275897198678,-1.,-3.66790152752075));
#53345=CARTESIAN_POINT('Ctrl Pts',(-1.97311947678517,-1.,-3.67571738107084));
#53346=CARTESIAN_POINT('Ctrl Pts',(-1.97344650304519,-1.,-3.68354319915092));
#53347=CARTESIAN_POINT('Ctrl Pts',(-1.97374016225483,-1.,-3.69137888599902));
#53348=CARTESIAN_POINT('Ctrl Pts',(-1.97394846383216,-1.,-3.6976552856004));
#53349=CARTESIAN_POINT('Ctrl Pts',(-1.97408973726715,-1.,-3.70236698912904));
#53350=CARTESIAN_POINT('Ctrl Pts',(-1.97417727645308,-1.,-3.70551008132332));
#53351=CARTESIAN_POINT('Ctrl Pts',(-1.97421938526992,-1.,-3.70708211654725));
#53352=CARTESIAN_POINT('',(-1.83867539237861,-1.,-3.77614523045147));
#53353=CARTESIAN_POINT('',(-1.97421938526992,-1.,-3.70708211654725));
#53354=CARTESIAN_POINT('',(-1.5189508286633,-1.,-3.42859860294306));
#53355=CARTESIAN_POINT('Ctrl Pts',(-1.83867539237861,-1.,-3.77614523045147));
#53356=CARTESIAN_POINT('Ctrl Pts',(-1.83742834010626,-1.,-3.77518714457833));
#53357=CARTESIAN_POINT('Ctrl Pts',(-1.83493697934534,-1.,-3.77326886064398));
#53358=CARTESIAN_POINT('Ctrl Pts',(-1.83120816955645,-1.,-3.77038509817999));
#53359=CARTESIAN_POINT('Ctrl Pts',(-1.82625289220915,-1.,-3.76652740353775));
#53360=CARTESIAN_POINT('Ctrl Pts',(-1.82008629694091,-1.,-3.76168412707948));
#53361=CARTESIAN_POINT('Ctrl Pts',(-1.8139472983358,-1.,-3.75681965683071));
#53362=CARTESIAN_POINT('Ctrl Pts',(-1.80783603939617,-1.,-3.75193395887977));
#53363=CARTESIAN_POINT('Ctrl Pts',(-1.8017527148577,-1.,-3.74702700875467));
#53364=CARTESIAN_POINT('Ctrl Pts',(-1.79569757859422,-1.,-3.74209880352445));
#53365=CARTESIAN_POINT('Ctrl Pts',(-1.78967092823491,-1.,-3.73714934730681));
#53366=CARTESIAN_POINT('Ctrl Pts',(-1.78367308442901,-1.,-3.7321786309547));
#53367=CARTESIAN_POINT('Ctrl Pts',(-1.77770437039658,-1.,-3.72718661205609));
#53368=CARTESIAN_POINT('Ctrl Pts',(-1.77176509401761,-1.,-3.72217319911254));
#53369=CARTESIAN_POINT('Ctrl Pts',(-1.76585552124394,-1.,-3.71713822377359));
#53370=CARTESIAN_POINT('Ctrl Pts',(-1.75997588498865,-1.,-3.71208146346136));
#53371=CARTESIAN_POINT('Ctrl Pts',(-1.75412641804042,-1.,-3.70700269736659));
#53372=CARTESIAN_POINT('Ctrl Pts',(-1.74830738046057,-1.,-3.7019017567335));
#53373=CARTESIAN_POINT('Ctrl Pts',(-1.74251908492617,-1.,-3.69677856910517));
#53374=CARTESIAN_POINT('Ctrl Pts',(-1.73676193254557,-1.,-3.69163322648036));
#53375=CARTESIAN_POINT('Ctrl Pts',(-1.73103640956717,-1.,-3.68646597019332));
#53376=CARTESIAN_POINT('Ctrl Pts',(-1.72534302437056,-1.,-3.68127704936579));
#53377=CARTESIAN_POINT('Ctrl Pts',(-1.71968225581808,-1.,-3.67606660374709));
#53378=CARTESIAN_POINT('Ctrl Pts',(-1.71405450210384,-1.,-3.67083454901611));
#53379=CARTESIAN_POINT('Ctrl Pts',(-1.70846001610956,-1.,-3.66558043198876));
#53380=CARTESIAN_POINT('Ctrl Pts',(-1.70289888566873,-1.,-3.66030338774847));
#53381=CARTESIAN_POINT('Ctrl Pts',(-1.69737117722534,-1.,-3.65500246526749));
#53382=CARTESIAN_POINT('Ctrl Pts',(-1.69187705481689,-1.,-3.64967689827371));
#53383=CARTESIAN_POINT('Ctrl Pts',(-1.68641690471457,-1.,-3.64432638915203));
#53384=CARTESIAN_POINT('Ctrl Pts',(-1.68099146651586,-1.,-3.63895140887462));
#53385=CARTESIAN_POINT('Ctrl Pts',(-1.67560193613156,-1.,-3.63355343201232));
#53386=CARTESIAN_POINT('Ctrl Pts',(-1.67024966008045,-1.,-3.62813422105271));
#53387=CARTESIAN_POINT('Ctrl Pts',(-1.66493585923855,-1.,-3.62269517989109));
#53388=CARTESIAN_POINT('Ctrl Pts',(-1.65966133399186,-1.,-3.61723666482456));
#53389=CARTESIAN_POINT('Ctrl Pts',(-1.65442619244325,-1.,-3.61175734965127));
#53390=CARTESIAN_POINT('Ctrl Pts',(-1.64922952425832,-1.,-3.60625346556992));
#53391=CARTESIAN_POINT('Ctrl Pts',(-1.64407004385582,-1.,-3.60072028513845));
#53392=CARTESIAN_POINT('Ctrl Pts',(-1.63894676675352,-1.,-3.59515368334893));
#53393=CARTESIAN_POINT('Ctrl Pts',(-1.6338597145126,-1.,-3.58955176627879));
#53394=CARTESIAN_POINT('Ctrl Pts',(-1.62881051550745,-1.,-3.58391625774343));
#53395=CARTESIAN_POINT('Ctrl Pts',(-1.62380329464844,-1.,-3.5782545595439));
#53396=CARTESIAN_POINT('Ctrl Pts',(-1.61884340915404,-1.,-3.57257679609806));
#53397=CARTESIAN_POINT('Ctrl Pts',(-1.61393581747514,-1.,-3.56689200468387));
#53398=CARTESIAN_POINT('Ctrl Pts',(-1.60908344685457,-1.,-3.5612043248298));
#53399=CARTESIAN_POINT('Ctrl Pts',(-1.60428584699853,-1.,-3.55550985096129));
#53400=CARTESIAN_POINT('Ctrl Pts',(-1.59953698113457,-1.,-3.54979148634454));
#53401=CARTESIAN_POINT('Ctrl Pts',(-1.59482766949766,-1.,-3.54402458182337));
#53402=CARTESIAN_POINT('Ctrl Pts',(-1.59014958368739,-1.,-3.53818616861077));
#53403=CARTESIAN_POINT('Ctrl Pts',(-1.58549906268088,-1.,-3.5322637814708));
#53404=CARTESIAN_POINT('Ctrl Pts',(-1.58088027227848,-1.,-3.52626275334881));
#53405=CARTESIAN_POINT('Ctrl Pts',(-1.57631049988158,-1.,-3.52021847865912));
#53406=CARTESIAN_POINT('Ctrl Pts',(-1.57181569799743,-1.,-3.51418598431665));
#53407=CARTESIAN_POINT('Ctrl Pts',(-1.56742097575012,-1.,-3.50821771695363));
#53408=CARTESIAN_POINT('Ctrl Pts',(-1.56314187758675,-1.,-3.50234321621578));
#53409=CARTESIAN_POINT('Ctrl Pts',(-1.55897703097874,-1.,-3.49655185179655));
#53410=CARTESIAN_POINT('Ctrl Pts',(-1.55489595901116,-1.,-3.4907646087742));
#53411=CARTESIAN_POINT('Ctrl Pts',(-1.55084702970452,-1.,-3.48485155928567));
#53412=CARTESIAN_POINT('Ctrl Pts',(-1.54678009290276,-1.,-3.47868272898751));
#53413=CARTESIAN_POINT('Ctrl Pts',(-1.54266605398187,-1.,-3.47217189224653));
#53414=CARTESIAN_POINT('Ctrl Pts',(-1.53851507915502,-1.,-3.46531752207153));
#53415=CARTESIAN_POINT('Ctrl Pts',(-1.53440195378792,-1.,-3.45825932955032));
#53416=CARTESIAN_POINT('Ctrl Pts',(-1.53046244461635,-1.,-3.45127136828305));
#53417=CARTESIAN_POINT('Ctrl Pts',(-1.52686242875556,-1.,-3.44469547526647));
#53418=CARTESIAN_POINT('Ctrl Pts',(-1.5237734895035,-1.,-3.4388889597401));
#53419=CARTESIAN_POINT('Ctrl Pts',(-1.52134826724293,-1.,-3.43417156977893));
#53420=CARTESIAN_POINT('Ctrl Pts',(-1.5198144909338,-1.,-3.43101631893414));
#53421=CARTESIAN_POINT('Ctrl Pts',(-1.51914806898491,-1.,-3.42946838852587));
#53422=CARTESIAN_POINT('Ctrl Pts',(-1.5189513329503,-1.,-3.42884302333841));
#53423=CARTESIAN_POINT('Ctrl Pts',(-1.51893924967331,-1.,-3.42864616361875));
#53424=CARTESIAN_POINT('Ctrl Pts',(-1.5189508286633,-1.,-3.42859860294306));
#53425=CARTESIAN_POINT('',(-1.35032489087269,-1.,-3.49844575334386));
#53426=CARTESIAN_POINT('Origin',(0.,-1.,0.));
#53427=CARTESIAN_POINT('',(-1.36999806084572,-1.,-3.97027773754922));
#53428=CARTESIAN_POINT('Ctrl Pts',(-1.35032489087269,-1.,-3.49844575334386));
#53429=CARTESIAN_POINT('Ctrl Pts',(-1.35036670893102,-1.,-3.49847119623841));
#53430=CARTESIAN_POINT('Ctrl Pts',(-1.35049736560633,-1.,-3.49861894124915));
#53431=CARTESIAN_POINT('Ctrl Pts',(-1.35080045218652,-1.,-3.49920025459856));
#53432=CARTESIAN_POINT('Ctrl Pts',(-1.35142377279535,-1.,-3.5007660381658));
#53433=CARTESIAN_POINT('Ctrl Pts',(-1.3525703284343,-1.,-3.50408168106113));
#53434=CARTESIAN_POINT('Ctrl Pts',(-1.35419113576022,-1.,-3.50913227060177));
#53435=CARTESIAN_POINT('Ctrl Pts',(-1.35611275237288,-1.,-3.51542230699919));
#53436=CARTESIAN_POINT('Ctrl Pts',(-1.35821701528975,-1.,-3.52261776117121));
#53437=CARTESIAN_POINT('Ctrl Pts',(-1.36037259643827,-1.,-3.53034464961849));
#53438=CARTESIAN_POINT('Ctrl Pts',(-1.36245507339334,-1.,-3.53824396425032));
#53439=CARTESIAN_POINT('Ctrl Pts',(-1.36436666257567,-1.,-3.54602591832893));
#53440=CARTESIAN_POINT('Ctrl Pts',(-1.36606145456711,-1.,-3.55353883995793));
#53441=CARTESIAN_POINT('Ctrl Pts',(-1.36754771771174,-1.,-3.56077662028492));
#53442=CARTESIAN_POINT('Ctrl Pts',(-1.36886584973349,-1.,-3.56782080304554));
#53443=CARTESIAN_POINT('Ctrl Pts',(-1.37007229485646,-1.,-3.57479875549453));
#53444=CARTESIAN_POINT('Ctrl Pts',(-1.37122241663073,-1.,-3.58183885982745));
#53445=CARTESIAN_POINT('Ctrl Pts',(-1.37235053661,-1.,-3.5890185384643));
#53446=CARTESIAN_POINT('Ctrl Pts',(-1.37346320103184,-1.,-3.59634627869117));
#53447=CARTESIAN_POINT('Ctrl Pts',(-1.37455051379642,-1.,-3.60379020124038));
#53448=CARTESIAN_POINT('Ctrl Pts',(-1.37559314436641,-1.,-3.61129546591082));
#53449=CARTESIAN_POINT('Ctrl Pts',(-1.37657053403102,-1.,-3.61880481160408));
#53450=CARTESIAN_POINT('Ctrl Pts',(-1.37746987919868,-1.,-3.62628098665112));
#53451=CARTESIAN_POINT('Ctrl Pts',(-1.37829035457324,-1.,-3.63371727442448));
#53452=CARTESIAN_POINT('Ctrl Pts',(-1.37903818567347,-1.,-3.64112507791112));
#53453=CARTESIAN_POINT('Ctrl Pts',(-1.37972372481598,-1.,-3.64852652756444));
#53454=CARTESIAN_POINT('Ctrl Pts',(-1.38035791051215,-1.,-3.65594554404396));
#53455=CARTESIAN_POINT('Ctrl Pts',(-1.38094856333558,-1.,-3.66339848520874));
#53456=CARTESIAN_POINT('Ctrl Pts',(-1.38149812653876,-1.,-3.67088843112282));
#53457=CARTESIAN_POINT('Ctrl Pts',(-1.38200574290626,-1.,-3.6784103848243));
#53458=CARTESIAN_POINT('Ctrl Pts',(-1.38246852827185,-1.,-3.68595444983844));
#53459=CARTESIAN_POINT('Ctrl Pts',(-1.38288311171649,-1.,-3.69350967899523));
#53460=CARTESIAN_POINT('Ctrl Pts',(-1.38324717612862,-1.,-3.70106792167894));
#53461=CARTESIAN_POINT('Ctrl Pts',(-1.38356065402122,-1.,-3.70862680753343));
#53462=CARTESIAN_POINT('Ctrl Pts',(-1.38382489984585,-1.,-3.7161876605181));
#53463=CARTESIAN_POINT('Ctrl Pts',(-1.3840421342895,-1.,-3.72375409358805));
#53464=CARTESIAN_POINT('Ctrl Pts',(-1.38421479111531,-1.,-3.73133035859283));
#53465=CARTESIAN_POINT('Ctrl Pts',(-1.38434489156456,-1.,-3.73891976418099));
#53466=CARTESIAN_POINT('Ctrl Pts',(-1.38443344984389,-1.,-3.7465231716786));
#53467=CARTESIAN_POINT('Ctrl Pts',(-1.38448077997155,-1.,-3.75413976318727));
#53468=CARTESIAN_POINT('Ctrl Pts',(-1.38448675253343,-1.,-3.76176768271347));
#53469=CARTESIAN_POINT('Ctrl Pts',(-1.38445107339517,-1.,-3.76940473185775));
#53470=CARTESIAN_POINT('Ctrl Pts',(-1.38437354551435,-1.,-3.77704902230441));
#53471=CARTESIAN_POINT('Ctrl Pts',(-1.38425435883773,-1.,-3.78469969805134));
#53472=CARTESIAN_POINT('Ctrl Pts',(-1.38409399694589,-1.,-3.79235669640907));
#53473=CARTESIAN_POINT('Ctrl Pts',(-1.38389311766701,-1.,-3.80002044322169));
#53474=CARTESIAN_POINT('Ctrl Pts',(-1.38365244046226,-1.,-3.80769156398429));
#53475=CARTESIAN_POINT('Ctrl Pts',(-1.38337263902766,-1.,-3.81537060817765));
#53476=CARTESIAN_POINT('Ctrl Pts',(-1.38305421262724,-1.,-3.82305771743715));
#53477=CARTESIAN_POINT('Ctrl Pts',(-1.38269750245086,-1.,-3.83075266982138));
#53478=CARTESIAN_POINT('Ctrl Pts',(-1.38230274828774,-1.,-3.83845502790609));
#53479=CARTESIAN_POINT('Ctrl Pts',(-1.38187013346089,-1.,-3.84616425605705));
#53480=CARTESIAN_POINT('Ctrl Pts',(-1.38139983115075,-1.,-3.85387983979557));
#53481=CARTESIAN_POINT('Ctrl Pts',(-1.38089205993067,-1.,-3.86160143044187));
#53482=CARTESIAN_POINT('Ctrl Pts',(-1.38034709213129,-1.,-3.86932885813403));
#53483=CARTESIAN_POINT('Ctrl Pts',(-1.37976523097187,-1.,-3.87706205830865));
#53484=CARTESIAN_POINT('Ctrl Pts',(-1.37914679719446,-1.,-3.88480102249461));
#53485=CARTESIAN_POINT('Ctrl Pts',(-1.37849211287981,-1.,-3.89254574338385));
#53486=CARTESIAN_POINT('Ctrl Pts',(-1.3778014851263,-1.,-3.90029615196255));
#53487=CARTESIAN_POINT('Ctrl Pts',(-1.3770751963376,-1.,-3.90805209522729));
#53488=CARTESIAN_POINT('Ctrl Pts',(-1.37631350505516,-1.,-3.91581337461825));
#53489=CARTESIAN_POINT('Ctrl Pts',(-1.37551664448057,-1.,-3.92357976987132));
#53490=CARTESIAN_POINT('Ctrl Pts',(-1.37468482215784,-1.,-3.93135106761941));
#53491=CARTESIAN_POINT('Ctrl Pts',(-1.37381821967499,-1.,-3.93912709041791));
#53492=CARTESIAN_POINT('Ctrl Pts',(-1.37291699203423,-1.,-3.94690771786926));
#53493=CARTESIAN_POINT('Ctrl Pts',(-1.37198126433139,-1.,-3.95469287283105));
#53494=CARTESIAN_POINT('Ctrl Pts',(-1.37120515615663,-1.,-3.96092458508407));
#53495=CARTESIAN_POINT('Ctrl Pts',(-1.37060761746027,-1.,-3.96560037975788));
#53496=CARTESIAN_POINT('Ctrl Pts',(-1.37020239094758,-1.,-3.9687184694173));
#53497=CARTESIAN_POINT('Ctrl Pts',(-1.36999806084572,-1.,-3.97027773754922));
#53498=CARTESIAN_POINT('',(-1.22531898815164,-1.,-4.01728681790024));
#53499=CARTESIAN_POINT('',(-1.36999806084572,-1.,-3.97027773754922));
#53500=CARTESIAN_POINT('',(-0.963899035118986,-1.,-3.62400312501199));
#53501=CARTESIAN_POINT('Ctrl Pts',(-1.22531898815164,-1.,-4.01728681790024));
#53502=CARTESIAN_POINT('Ctrl Pts',(-1.22423716681317,-1.,-4.01614544569895));
#53503=CARTESIAN_POINT('Ctrl Pts',(-1.22207656455845,-1.,-4.01386104433519));
#53504=CARTESIAN_POINT('Ctrl Pts',(-1.21884478244403,-1.,-4.01042947140789));
#53505=CARTESIAN_POINT('Ctrl Pts',(-1.21455398918133,-1.,-4.00584409522722));
#53506=CARTESIAN_POINT('Ctrl Pts',(-1.20922097029551,-1.,-4.00009577950721));
#53507=CARTESIAN_POINT('Ctrl Pts',(-1.20391852375139,-1.,-3.99433084799666));
#53508=CARTESIAN_POINT('Ctrl Pts',(-1.19864679609566,-1.,-3.98854928957189));
#53509=CARTESIAN_POINT('Ctrl Pts',(-1.19340598349475,-1.,-3.98275111052561));
#53510=CARTESIAN_POINT('Ctrl Pts',(-1.18819633715539,-1.,-3.97693634767754));
#53511=CARTESIAN_POINT('Ctrl Pts',(-1.18301815039831,-1.,-3.97110505165415));
#53512=CARTESIAN_POINT('Ctrl Pts',(-1.17787174135592,-1.,-3.96525726358159));
#53513=CARTESIAN_POINT('Ctrl Pts',(-1.17275743590361,-1.,-3.95939299213276));
#53514=CARTESIAN_POINT('Ctrl Pts',(-1.16767555244438,-1.,-3.95351219509876));
#53515=CARTESIAN_POINT('Ctrl Pts',(-1.16262637999157,-1.,-3.94761474780583));
#53516=CARTESIAN_POINT('Ctrl Pts',(-1.15761018340956,-1.,-3.94170046685203));
#53517=CARTESIAN_POINT('Ctrl Pts',(-1.1526272271632,-1.,-3.9357691705628));
#53518=CARTESIAN_POINT('Ctrl Pts',(-1.14767779451123,-1.,-3.92982073294257));
#53519=CARTESIAN_POINT('Ctrl Pts',(-1.14276220561593,-1.,-3.92385513133997));
#53520=CARTESIAN_POINT('Ctrl Pts',(-1.13788084225554,-1.,-3.91787251936827));
#53521=CARTESIAN_POINT('Ctrl Pts',(-1.13303414693896,-1.,-3.91187321145649));
#53522=CARTESIAN_POINT('Ctrl Pts',(-1.12822258281553,-1.,-3.90585753318737));
#53523=CARTESIAN_POINT('Ctrl Pts',(-1.12344660099043,-1.,-3.89982569750025));
#53524=CARTESIAN_POINT('Ctrl Pts',(-1.11870660794603,-1.,-3.89377768340344));
#53525=CARTESIAN_POINT('Ctrl Pts',(-1.11400292434429,-1.,-3.88771308285171));
#53526=CARTESIAN_POINT('Ctrl Pts',(-1.10933577224008,-1.,-3.88163105531724));
#53527=CARTESIAN_POINT('Ctrl Pts',(-1.10470536603287,-1.,-3.87553067187514));
#53528=CARTESIAN_POINT('Ctrl Pts',(-1.10011198761195,-1.,-3.86941120134849));
#53529=CARTESIAN_POINT('Ctrl Pts',(-1.09555606505013,-1.,-3.86327241021247));
#53530=CARTESIAN_POINT('Ctrl Pts',(-1.09103825516294,-1.,-3.85711487933931));
#53531=CARTESIAN_POINT('Ctrl Pts',(-1.08655950846384,-1.,-3.85094025222713));
#53532=CARTESIAN_POINT('Ctrl Pts',(-1.08212087917991,-1.,-3.8447504803063));
#53533=CARTESIAN_POINT('Ctrl Pts',(-1.07772335353858,-1.,-3.83854714117491));
#53534=CARTESIAN_POINT('Ctrl Pts',(-1.07336766633459,-1.,-3.83233071195144));
#53535=CARTESIAN_POINT('Ctrl Pts',(-1.06905413180359,-1.,-3.82609989967276));
#53536=CARTESIAN_POINT('Ctrl Pts',(-1.0647824403893,-1.,-3.81985083953012));
#53537=CARTESIAN_POINT('Ctrl Pts',(-1.06055206187299,-1.,-3.8135786611749));
#53538=CARTESIAN_POINT('Ctrl Pts',(-1.05636266918644,-1.,-3.80727913637791));
#53539=CARTESIAN_POINT('Ctrl Pts',(-1.05221457990016,-1.,-3.80095039790681));
#53540=CARTESIAN_POINT('Ctrl Pts',(-1.04810913267639,-1.,-3.79459440308786));
#53541=CARTESIAN_POINT('Ctrl Pts',(-1.04404924374422,-1.,-3.78821910787179));
#53542=CARTESIAN_POINT('Ctrl Pts',(-1.04003862055798,-1.,-3.7818353500817));
#53543=CARTESIAN_POINT('Ctrl Pts',(-1.03608074678008,-1.,-3.77545283140427));
#53544=CARTESIAN_POINT('Ctrl Pts',(-1.03217786604919,-1.,-3.76907609832516));
#53545=CARTESIAN_POINT('Ctrl Pts',(-1.02833014458184,-1.,-3.76270122291245));
#53546=CARTESIAN_POINT('Ctrl Pts',(-1.02453429444668,-1.,-3.75631037456224));
#53547=CARTESIAN_POINT('Ctrl Pts',(-1.02078510487439,-1.,-3.74987777155873));
#53548=CARTESIAN_POINT('Ctrl Pts',(-1.01707794311088,-1.,-3.74337942504993));
#53549=CARTESIAN_POINT('Ctrl Pts',(-1.01341114319906,-1.,-3.73680245055747));
#53550=CARTESIAN_POINT('Ctrl Pts',(-1.00978798539491,-1.,-3.73015276704407));
#53551=CARTESIAN_POINT('Ctrl Pts',(-1.00622000735696,-1.,-3.72346803750544));
#53552=CARTESIAN_POINT('Ctrl Pts',(-1.00272423396802,-1.,-3.71680667125047));
#53553=CARTESIAN_POINT('Ctrl Pts',(-0.999317260756344,-1.,-3.7102243971387));
#53554=CARTESIAN_POINT('Ctrl Pts',(-0.996009819772432,-1.,-3.70375282282107));
#53555=CARTESIAN_POINT('Ctrl Pts',(-0.992802218332104,-1.,-3.69738123415696));
#53556=CARTESIAN_POINT('Ctrl Pts',(-0.989676715398858,-1.,-3.69102682138955));
#53557=CARTESIAN_POINT('Ctrl Pts',(-0.986602639864286,-1.,-3.6845531792623));
#53558=CARTESIAN_POINT('Ctrl Pts',(-0.983550791470864,-1.,-3.67782408841876));
#53559=CARTESIAN_POINT('Ctrl Pts',(-0.980505922458494,-1.,-3.67074983340444));
#53560=CARTESIAN_POINT('Ctrl Pts',(-0.977478312751416,-1.,-3.66333049637403));
#53561=CARTESIAN_POINT('Ctrl Pts',(-0.974519971354139,-1.,-3.6557157673487));
#53562=CARTESIAN_POINT('Ctrl Pts',(-0.971722122060277,-1.,-3.64819756447072));
#53563=CARTESIAN_POINT('Ctrl Pts',(-0.969195124674829,-1.,-3.64113946505393));
#53564=CARTESIAN_POINT('Ctrl Pts',(-0.967052554540877,-1.,-3.6349212208096));
#53565=CARTESIAN_POINT('Ctrl Pts',(-0.965395153165716,-1.,-3.62988252139998));
#53566=CARTESIAN_POINT('Ctrl Pts',(-0.964373850166081,-1.,-3.62652618145252));
#53567=CARTESIAN_POINT('Ctrl Pts',(-0.963957782642589,-1.,-3.62489305727516));
#53568=CARTESIAN_POINT('Ctrl Pts',(-0.963861297423579,-1.,-3.62424461507455));
#53569=CARTESIAN_POINT('Ctrl Pts',(-0.963880158556713,-1.,-3.62404828878374));
#53570=CARTESIAN_POINT('Ctrl Pts',(-0.963899035118986,-1.,-3.62400312501199));
#53571=CARTESIAN_POINT('',(-0.786422660833743,-1.,-3.66661143271648));
#53572=CARTESIAN_POINT('Origin',(0.,-1.,0.));
#53573=CARTESIAN_POINT('',(-0.732042837400619,-1.,-4.13571194405636));
#53574=CARTESIAN_POINT('Ctrl Pts',(-0.786422660833743,-1.,-3.66661143271648));
#53575=CARTESIAN_POINT('Ctrl Pts',(-0.786459983896781,-1.,-3.66664310415236));
#53576=CARTESIAN_POINT('Ctrl Pts',(-0.78656591955989,-1.,-3.66680946938396));
#53577=CARTESIAN_POINT('Ctrl Pts',(-0.786774337198499,-1.,-3.66743103898844));
#53578=CARTESIAN_POINT('Ctrl Pts',(-0.787145041181589,-1.,-3.66907505398769));
#53579=CARTESIAN_POINT('Ctrl Pts',(-0.787758799995426,-1.,-3.672529236635));
#53580=CARTESIAN_POINT('Ctrl Pts',(-0.788569566220662,-1.,-3.67777119516438));
#53581=CARTESIAN_POINT('Ctrl Pts',(-0.789483546065158,-1.,-3.68428439784285));
#53582=CARTESIAN_POINT('Ctrl Pts',(-0.79043628498958,-1.,-3.69172044327754));
#53583=CARTESIAN_POINT('Ctrl Pts',(-0.791356575696509,-1.,-3.69968940808982));
#53584=CARTESIAN_POINT('Ctrl Pts',(-0.792177688845968,-1.,-3.70781724021879));
#53585=CARTESIAN_POINT('Ctrl Pts',(-0.792848377370115,-1.,-3.7158024239604));
#53586=CARTESIAN_POINT('Ctrl Pts',(-0.79334702378387,-1.,-3.7234879729357));
#53587=CARTESIAN_POINT('Ctrl Pts',(-0.793682750269347,-1.,-3.7308691469564));
#53588=CARTESIAN_POINT('Ctrl Pts',(-0.79388270093679,-1.,-3.73803280541576));
#53589=CARTESIAN_POINT('Ctrl Pts',(-0.79398270045988,-1.,-3.74511357728827));
#53590=CARTESIAN_POINT('Ctrl Pts',(-0.794017347371441,-1.,-3.75224692493895));
#53591=CARTESIAN_POINT('Ctrl Pts',(-0.794008429135047,-1.,-3.75951468666325));
#53592=CARTESIAN_POINT('Ctrl Pts',(-0.793961083689141,-1.,-3.76692626931184));
#53593=CARTESIAN_POINT('Ctrl Pts',(-0.793870523787515,-1.,-3.77444863801264));
#53594=CARTESIAN_POINT('Ctrl Pts',(-0.793726235781339,-1.,-3.78202460377617));
#53595=CARTESIAN_POINT('Ctrl Pts',(-0.793516871680966,-1.,-3.78959439439222));
#53596=CARTESIAN_POINT('Ctrl Pts',(-0.7932356129732,-1.,-3.79711921389862));
#53597=CARTESIAN_POINT('Ctrl Pts',(-0.792882695234693,-1.,-3.80459229925598));
#53598=CARTESIAN_POINT('Ctrl Pts',(-0.792462483517568,-1.,-3.81202588694726));
#53599=CARTESIAN_POINT('Ctrl Pts',(-0.791981740718606,-1.,-3.81944345442237));
#53600=CARTESIAN_POINT('Ctrl Pts',(-0.791447528662381,-1.,-3.82687033899799));
#53601=CARTESIAN_POINT('Ctrl Pts',(-0.79086501270534,-1.,-3.83432392054804));
#53602=CARTESIAN_POINT('Ctrl Pts',(-0.790236124191289,-1.,-3.84180762342476));
#53603=CARTESIAN_POINT('Ctrl Pts',(-0.789560798155619,-1.,-3.8493163780891));
#53604=CARTESIAN_POINT('Ctrl Pts',(-0.788837734090688,-1.,-3.85683995872536));
#53605=CARTESIAN_POINT('Ctrl Pts',(-0.788065315093771,-1.,-3.86436702561342));
#53606=CARTESIAN_POINT('Ctrl Pts',(-0.78724252761798,-1.,-3.87188916600905));
#53607=CARTESIAN_POINT('Ctrl Pts',(-0.786369675812592,-1.,-3.87940402818186));
#53608=CARTESIAN_POINT('Ctrl Pts',(-0.785447890340723,-1.,-3.88691313167399));
#53609=CARTESIAN_POINT('Ctrl Pts',(-0.784478799358336,-1.,-3.89442039235105));
#53610=CARTESIAN_POINT('Ctrl Pts',(-0.783464141529082,-1.,-3.90193039043971));
#53611=CARTESIAN_POINT('Ctrl Pts',(-0.782405395622759,-1.,-3.90944671004536));
#53612=CARTESIAN_POINT('Ctrl Pts',(-0.781303428618344,-1.,-3.9169703605466));
#53613=CARTESIAN_POINT('Ctrl Pts',(-0.780158678615507,-1.,-3.92450058323799));
#53614=CARTESIAN_POINT('Ctrl Pts',(-0.778971308134786,-1.,-3.93203552473153));
#53615=CARTESIAN_POINT('Ctrl Pts',(-0.77774137056855,-1.,-3.93957296768098));
#53616=CARTESIAN_POINT('Ctrl Pts',(-0.77646896669796,-1.,-3.94711101619471));
#53617=CARTESIAN_POINT('Ctrl Pts',(-0.775154418039441,-1.,-3.95464885452364));
#53618=CARTESIAN_POINT('Ctrl Pts',(-0.773798212026683,-1.,-3.96218649639876));
#53619=CARTESIAN_POINT('Ctrl Pts',(-0.772400931772239,-1.,-3.96972446532832));
#53620=CARTESIAN_POINT('Ctrl Pts',(-0.770963190030504,-1.,-3.97726349165507));
#53621=CARTESIAN_POINT('Ctrl Pts',(-0.769485566245459,-1.,-3.98480422348403));
#53622=CARTESIAN_POINT('Ctrl Pts',(-0.767968531377708,-1.,-3.99234687880892));
#53623=CARTESIAN_POINT('Ctrl Pts',(-0.766412457135786,-1.,-3.99989129179464));
#53624=CARTESIAN_POINT('Ctrl Pts',(-0.764817648784946,-1.,-4.00743706791366));
#53625=CARTESIAN_POINT('Ctrl Pts',(-0.763184371182827,-1.,-4.01498370680434));
#53626=CARTESIAN_POINT('Ctrl Pts',(-0.761512875859942,-1.,-4.02253072741347));
#53627=CARTESIAN_POINT('Ctrl Pts',(-0.759803433244166,-1.,-4.0300778195465));
#53628=CARTESIAN_POINT('Ctrl Pts',(-0.758056338885554,-1.,-4.03762485803468));
#53629=CARTESIAN_POINT('Ctrl Pts',(-0.756271902370187,-1.,-4.04517182654344));
#53630=CARTESIAN_POINT('Ctrl Pts',(-0.754450441816412,-1.,-4.05271876688106));
#53631=CARTESIAN_POINT('Ctrl Pts',(-0.752592276482869,-1.,-4.06026572221399));
#53632=CARTESIAN_POINT('Ctrl Pts',(-0.750697720483176,-1.,-4.06781267241886));
#53633=CARTESIAN_POINT('Ctrl Pts',(-0.748767076679177,-1.,-4.07535951055363));
#53634=CARTESIAN_POINT('Ctrl Pts',(-0.746800631490822,-1.,-4.08290608094789));
#53635=CARTESIAN_POINT('Ctrl Pts',(-0.744798649705514,-1.,-4.09045220253011));
#53636=CARTESIAN_POINT('Ctrl Pts',(-0.742761369690018,-1.,-4.09799769702712));
#53637=CARTESIAN_POINT('Ctrl Pts',(-0.740688998555152,-1.,-4.1055424175856));
#53638=CARTESIAN_POINT('Ctrl Pts',(-0.738581708229119,-1.,-4.11308626953795));
#53639=CARTESIAN_POINT('Ctrl Pts',(-0.736439634335347,-1.,-4.12062919626082));
#53640=CARTESIAN_POINT('Ctrl Pts',(-0.734698226767512,-1.,-4.12666277572794));
#53641=CARTESIAN_POINT('Ctrl Pts',(-0.733376589325634,-1.,-4.13118752796397));
#53642=CARTESIAN_POINT('Ctrl Pts',(-0.732488575135926,-1.,-4.13420383737278));
#53643=CARTESIAN_POINT('Ctrl Pts',(-0.732042837400619,-1.,-4.13571194405636));
#53644=CARTESIAN_POINT('',(-0.581791163835814,-1.,-4.15950947128175));
#53645=CARTESIAN_POINT('',(-0.732042837400619,-1.,-4.13571194405636));
#53646=CARTESIAN_POINT('',(-0.385112848332549,-1.,-3.73017266276632));
#53647=CARTESIAN_POINT('Ctrl Pts',(-0.581791163835814,-1.,-4.15950947128175));
#53648=CARTESIAN_POINT('Ctrl Pts',(-0.580901211462913,-1.,-4.15821291712391));
#53649=CARTESIAN_POINT('Ctrl Pts',(-0.579124568912543,-1.,-4.15561864787379));
#53650=CARTESIAN_POINT('Ctrl Pts',(-0.576469391673917,-1.,-4.1517237611974));
#53651=CARTESIAN_POINT('Ctrl Pts',(-0.572948736066277,-1.,-4.14652361065787));
#53652=CARTESIAN_POINT('Ctrl Pts',(-0.568580610187116,-1.,-4.14001179828669));
#53653=CARTESIAN_POINT('Ctrl Pts',(-0.564245279535705,-1.,-4.13348835726086));
#53654=CARTESIAN_POINT('Ctrl Pts',(-0.559942890594628,-1.,-4.12695329951859));
#53655=CARTESIAN_POINT('Ctrl Pts',(-0.555673636130778,-1.,-4.1204066619623));
#53656=CARTESIAN_POINT('Ctrl Pts',(-0.551437758498247,-1.,-4.11384852025578));
#53657=CARTESIAN_POINT('Ctrl Pts',(-0.54723553948676,-1.,-4.1072789702877));
#53658=CARTESIAN_POINT('Ctrl Pts',(-0.543067286878457,-1.,-4.10069810244473));
#53659=CARTESIAN_POINT('Ctrl Pts',(-0.538933321179921,-1.,-4.09410597627116));
#53660=CARTESIAN_POINT('Ctrl Pts',(-0.534833963476999,-1.,-4.08750259988693));
#53661=CARTESIAN_POINT('Ctrl Pts',(-0.530769518728075,-1.,-4.08088789536488));
#53662=CARTESIAN_POINT('Ctrl Pts',(-0.526740277227,-1.,-4.07426172299496));
#53663=CARTESIAN_POINT('Ctrl Pts',(-0.522746528602768,-1.,-4.06762394471075));
#53664=CARTESIAN_POINT('Ctrl Pts',(-0.51878857233681,-1.,-4.06097448037934));
#53665=CARTESIAN_POINT('Ctrl Pts',(-0.514866728193104,-1.,-4.05431335771261));
#53666=CARTESIAN_POINT('Ctrl Pts',(-0.510981349219174,-1.,-4.04764078815591));
#53667=CARTESIAN_POINT('Ctrl Pts',(-0.507132823288362,-1.,-4.04095715149074));
#53668=CARTESIAN_POINT('Ctrl Pts',(-0.503321556915514,-1.,-4.0342628417439));
#53669=CARTESIAN_POINT('Ctrl Pts',(-0.49954796234089,-1.,-4.0275581398015));
#53670=CARTESIAN_POINT('Ctrl Pts',(-0.495812444326223,-1.,-4.02084308851813));
#53671=CARTESIAN_POINT('Ctrl Pts',(-0.492115383417931,-1.,-4.01411733503486));
#53672=CARTESIAN_POINT('Ctrl Pts',(-0.488457130424531,-1.,-4.0073800839092));
#53673=CARTESIAN_POINT('Ctrl Pts',(-0.484838042421754,-1.,-4.00063045119234));
#53674=CARTESIAN_POINT('Ctrl Pts',(-0.481258512209638,-1.,-3.99386775880655));
#53675=CARTESIAN_POINT('Ctrl Pts',(-0.477718999122033,-1.,-3.98709184306743));
#53676=CARTESIAN_POINT('Ctrl Pts',(-0.474220061019542,-1.,-3.9803033804443));
#53677=CARTESIAN_POINT('Ctrl Pts',(-0.470762379613477,-1.,-3.97350414289415));
#53678=CARTESIAN_POINT('Ctrl Pts',(-0.467346690880672,-1.,-3.96669622273946));
#53679=CARTESIAN_POINT('Ctrl Pts',(-0.463973722115744,-1.,-3.95988133243543));
#53680=CARTESIAN_POINT('Ctrl Pts',(-0.460644124429119,-1.,-3.95306005817363));
#53681=CARTESIAN_POINT('Ctrl Pts',(-0.457358410451674,-1.,-3.94623117206675));
#53682=CARTESIAN_POINT('Ctrl Pts',(-0.454116879027576,-1.,-3.93939080846298));
#53683=CARTESIAN_POINT('Ctrl Pts',(-0.450919768356347,-1.,-3.93253407403128));
#53684=CARTESIAN_POINT('Ctrl Pts',(-0.447767416837297,-1.,-3.92565674143424));
#53685=CARTESIAN_POINT('Ctrl Pts',(-0.444660430230593,-1.,-3.91875701610721));
#53686=CARTESIAN_POINT('Ctrl Pts',(-0.441599824524047,-1.,-3.91183704069146));
#53687=CARTESIAN_POINT('Ctrl Pts',(-0.438587235458233,-1.,-3.90490512938546));
#53688=CARTESIAN_POINT('Ctrl Pts',(-0.435624629433506,-1.,-3.8979725665544));
#53689=CARTESIAN_POINT('Ctrl Pts',(-0.432713929544439,-1.,-3.89104947940592));
#53690=CARTESIAN_POINT('Ctrl Pts',(-0.429856640579734,-1.,-3.88414070943334));
#53691=CARTESIAN_POINT('Ctrl Pts',(-0.427053541173469,-1.,-3.87724240306609));
#53692=CARTESIAN_POINT('Ctrl Pts',(-0.424304173195142,-1.,-3.87033643487882));
#53693=CARTESIAN_POINT('Ctrl Pts',(-0.421607423177576,-1.,-3.86339652542749));
#53694=CARTESIAN_POINT('Ctrl Pts',(-0.41896246808681,-1.,-3.85639825648031));
#53695=CARTESIAN_POINT('Ctrl Pts',(-0.41636967805292,-1.,-3.8493286415751));
#53696=CARTESIAN_POINT('Ctrl Pts',(-0.413831367016727,-1.,-3.84219403994742));
#53697=CARTESIAN_POINT('Ctrl Pts',(-0.41135303879846,-1.,-3.83503345578645));
#53698=CARTESIAN_POINT('Ctrl Pts',(-0.408942371447377,-1.,-3.82790724256397));
#53699=CARTESIAN_POINT('Ctrl Pts',(-0.406607038258906,-1.,-3.82087303913741));
#53700=CARTESIAN_POINT('Ctrl Pts',(-0.404352694628236,-1.,-3.81396374287762));
#53701=CARTESIAN_POINT('Ctrl Pts',(-0.402181320148475,-1.,-3.80716881962763));
#53702=CARTESIAN_POINT('Ctrl Pts',(-0.400088346504727,-1.,-3.80040370384659));
#53703=CARTESIAN_POINT('Ctrl Pts',(-0.398064818684158,-1.,-3.79352887163457));
#53704=CARTESIAN_POINT('Ctrl Pts',(-0.396103205335029,-1.,-3.78640521279479));
#53705=CARTESIAN_POINT('Ctrl Pts',(-0.394202481011595,-1.,-3.77894173114368));
#53706=CARTESIAN_POINT('Ctrl Pts',(-0.392372786223347,-1.,-3.77114011595892));
#53707=CARTESIAN_POINT('Ctrl Pts',(-0.390642072979259,-1.,-3.76315635032993));
#53708=CARTESIAN_POINT('Ctrl Pts',(-0.389054775898251,-1.,-3.75529302894757));
#53709=CARTESIAN_POINT('Ctrl Pts',(-0.387663020050396,-1.,-3.74792651696269));
#53710=CARTESIAN_POINT('Ctrl Pts',(-0.386519576222035,-1.,-3.74144965781088));
#53711=CARTESIAN_POINT('Ctrl Pts',(-0.385670806454744,-1.,-3.73621371845475));
#53712=CARTESIAN_POINT('Ctrl Pts',(-0.385187124633965,-1.,-3.73273893363318));
#53713=CARTESIAN_POINT('Ctrl Pts',(-0.385031656499141,-1.,-3.73106082862399));
#53714=CARTESIAN_POINT('Ctrl Pts',(-0.385037797882046,-1.,-3.73040527620929));
#53715=CARTESIAN_POINT('Ctrl Pts',(-0.385087139001609,-1.,-3.73021431755218));
#53716=CARTESIAN_POINT('Ctrl Pts',(-0.385112848332549,-1.,-3.73017266276632));
#53717=CARTESIAN_POINT('',(-0.203156094897896,-1.,-3.74449296982994));
#53718=CARTESIAN_POINT('Origin',(0.,-1.,0.));
#53719=CARTESIAN_POINT('',(-0.0760622897878238,-1.,-4.19931119685982));
#53720=CARTESIAN_POINT('Ctrl Pts',(-0.203156094897896,-1.,-3.74449296982994));
#53721=CARTESIAN_POINT('Ctrl Pts',(-0.203188003947965,-1.,-3.74453008995129));
#53722=CARTESIAN_POINT('Ctrl Pts',(-0.203266610111264,-1.,-3.74471097893961));
#53723=CARTESIAN_POINT('Ctrl Pts',(-0.203375226874331,-1.,-3.74535749969262));
#53724=CARTESIAN_POINT('Ctrl Pts',(-0.203484186269315,-1.,-3.74703926501843));
#53725=CARTESIAN_POINT('Ctrl Pts',(-0.203550035479097,-1.,-3.75054693397716));
#53726=CARTESIAN_POINT('Ctrl Pts',(-0.203530796848404,-1.,-3.75585118707924));
#53727=CARTESIAN_POINT('Ctrl Pts',(-0.203414634707646,-1.,-3.76242717937273));
#53728=CARTESIAN_POINT('Ctrl Pts',(-0.203192390045337,-1.,-3.76992071595267));
#53729=CARTESIAN_POINT('Ctrl Pts',(-0.202854729699197,-1.,-3.77793553476879));
#53730=CARTESIAN_POINT('Ctrl Pts',(-0.202394260512193,-1.,-3.78609175019317));
#53731=CARTESIAN_POINT('Ctrl Pts',(-0.201807533800799,-1.,-3.79408354187274));
#53732=CARTESIAN_POINT('Ctrl Pts',(-0.201097756307252,-1.,-3.80175247447171));
#53733=CARTESIAN_POINT('Ctrl Pts',(-0.20027467943329,-1.,-3.80909529318501));
#53734=CARTESIAN_POINT('Ctrl Pts',(-0.199351525297396,-1.,-3.81620203429702));
#53735=CARTESIAN_POINT('Ctrl Pts',(-0.19834261690047,-1.,-3.82321127348981));
#53736=CARTESIAN_POINT('Ctrl Pts',(-0.197260935827375,-1.,-3.83026221776488));
#53737=CARTESIAN_POINT('Ctrl Pts',(-0.19611519897189,-1.,-3.83743910616265));
#53738=CARTESIAN_POINT('Ctrl Pts',(-0.194909009460255,-1.,-3.84475203347052));
#53739=CARTESIAN_POINT('Ctrl Pts',(-0.193642806777748,-1.,-3.85216762264019));
#53740=CARTESIAN_POINT('Ctrl Pts',(-0.19231515304498,-1.,-3.85962774407652));
#53741=CARTESIAN_POINT('Ctrl Pts',(-0.190924190418613,-1.,-3.8670715862477));
#53742=CARTESIAN_POINT('Ctrl Pts',(-0.189469253358254,-1.,-3.87445976418377));
#53743=CARTESIAN_POINT('Ctrl Pts',(-0.187951632512663,-1.,-3.88178563496187));
#53744=CARTESIAN_POINT('Ctrl Pts',(-0.186373724985263,-1.,-3.88906196725817));
#53745=CARTESIAN_POINT('Ctrl Pts',(-0.184738537728035,-1.,-3.89631300742633));
#53746=CARTESIAN_POINT('Ctrl Pts',(-0.183049081993193,-1.,-3.90356488555138));
#53747=CARTESIAN_POINT('Ctrl Pts',(-0.181307740731796,-1.,-3.91083557557193));
#53748=CARTESIAN_POINT('Ctrl Pts',(-0.179515885822895,-1.,-3.91812876180948));
#53749=CARTESIAN_POINT('Ctrl Pts',(-0.177674246152328,-1.,-3.92543942697672));
#53750=CARTESIAN_POINT('Ctrl Pts',(-0.175783136893873,-1.,-3.93275726771049));
#53751=CARTESIAN_POINT('Ctrl Pts',(-0.173842734974607,-1.,-3.94007083096214));
#53752=CARTESIAN_POINT('Ctrl Pts',(-0.171853355369233,-1.,-3.94737164900861));
#53753=CARTESIAN_POINT('Ctrl Pts',(-0.16981566637413,-1.,-3.95465744665263));
#53754=CARTESIAN_POINT('Ctrl Pts',(-0.167730547023312,-1.,-3.96192990160296));
#53755=CARTESIAN_POINT('Ctrl Pts',(-0.165598992851098,-1.,-3.9691931362141));
#53756=CARTESIAN_POINT('Ctrl Pts',(-0.163422004609999,-1.,-3.97645194630944));
#53757=CARTESIAN_POINT('Ctrl Pts',(-0.161200482186088,-1.,-3.98371010319866));
#53758=CARTESIAN_POINT('Ctrl Pts',(-0.158935123982796,-1.,-3.99096873945862));
#53759=CARTESIAN_POINT('Ctrl Pts',(-0.156626481393736,-1.,-3.99822717425869));
#53760=CARTESIAN_POINT('Ctrl Pts',(-0.15427500487231,-1.,-4.00548360245297));
#53761=CARTESIAN_POINT('Ctrl Pts',(-0.151881094022909,-1.,-4.01273584234684));
#53762=CARTESIAN_POINT('Ctrl Pts',(-0.149445144968708,-1.,-4.01998203715588));
#53763=CARTESIAN_POINT('Ctrl Pts',(-0.146967602878999,-1.,-4.02722143147048));
#53764=CARTESIAN_POINT('Ctrl Pts',(-0.144448947038352,-1.,-4.03445411510403));
#53765=CARTESIAN_POINT('Ctrl Pts',(-0.141889671485508,-1.,-4.04168069633842));
#53766=CARTESIAN_POINT('Ctrl Pts',(-0.13929026718006,-1.,-4.04890199238056));
#53767=CARTESIAN_POINT('Ctrl Pts',(-0.136651205046111,-1.,-4.05611873400122));
#53768=CARTESIAN_POINT('Ctrl Pts',(-0.133972916144225,-1.,-4.06333121018476));
#53769=CARTESIAN_POINT('Ctrl Pts',(-0.131255793548914,-1.,-4.07053931528579));
#53770=CARTESIAN_POINT('Ctrl Pts',(-0.128500200484814,-1.,-4.07774270738809));
#53771=CARTESIAN_POINT('Ctrl Pts',(-0.125706476822529,-1.,-4.08494093372315));
#53772=CARTESIAN_POINT('Ctrl Pts',(-0.122874946249119,-1.,-4.09213355850836));
#53773=CARTESIAN_POINT('Ctrl Pts',(-0.120005924388162,-1.,-4.09932031767243));
#53774=CARTESIAN_POINT('Ctrl Pts',(-0.117099722731705,-1.,-4.10650113382187));
#53775=CARTESIAN_POINT('Ctrl Pts',(-0.114156649609602,-1.,-4.11367603925313));
#53776=CARTESIAN_POINT('Ctrl Pts',(-0.111177012683377,-1.,-4.12084512502444));
#53777=CARTESIAN_POINT('Ctrl Pts',(-0.10816112052835,-1.,-4.12800848371386));
#53778=CARTESIAN_POINT('Ctrl Pts',(-0.105109286538864,-1.,-4.13516614458396));
#53779=CARTESIAN_POINT('Ctrl Pts',(-0.102021826577454,-1.,-4.14231804938737));
#53780=CARTESIAN_POINT('Ctrl Pts',(-0.0988990478899814,-1.,-4.1494640891762));
#53781=CARTESIAN_POINT('Ctrl Pts',(-0.095741240329707,-1.,-4.15660412653006));
#53782=CARTESIAN_POINT('Ctrl Pts',(-0.0925486672167692,-1.,-4.16373802265942));
#53783=CARTESIAN_POINT('Ctrl Pts',(-0.089321556085033,-1.,-4.17086566491823));
#53784=CARTESIAN_POINT('Ctrl Pts',(-0.0860600915552517,-1.,-4.17798698669991));
#53785=CARTESIAN_POINT('Ctrl Pts',(-0.0827644164389512,-1.,-4.1851019532944));
#53786=CARTESIAN_POINT('Ctrl Pts',(-0.0801005887117605,-1.,-4.19078883322483));
#53787=CARTESIAN_POINT('Ctrl Pts',(-0.0780873956244405,-1.,-4.19505112860624));
#53788=CARTESIAN_POINT('Ctrl Pts',(-0.0767384596142197,-1.,-4.19789138621624));
#53789=CARTESIAN_POINT('Ctrl Pts',(-0.0760622897878238,-1.,-4.19931119685982));
#53790=CARTESIAN_POINT('',(0.0760622897878244,-1.,-4.19931119685982));
#53791=CARTESIAN_POINT('',(-0.0760622897878238,-1.,-4.19931119685982));
#53792=CARTESIAN_POINT('',(0.2031560948961,-1.,-3.74449296983004));
#53793=CARTESIAN_POINT('Ctrl Pts',(0.0760622897878244,-1.,-4.19931119685982));
#53794=CARTESIAN_POINT('Ctrl Pts',(0.0767384596141462,-1.,-4.1978913862118));
#53795=CARTESIAN_POINT('Ctrl Pts',(0.0780873956242395,-1.,-4.19505112859416));
#53796=CARTESIAN_POINT('Ctrl Pts',(0.0801005887114317,-1.,-4.19078883320504));
#53797=CARTESIAN_POINT('Ctrl Pts',(0.0827644164385676,-1.,-4.18510195327123));
#53798=CARTESIAN_POINT('Ctrl Pts',(0.0860600915549394,-1.,-4.17798698668094));
#53799=CARTESIAN_POINT('Ctrl Pts',(0.0893215560848647,-1.,-4.17086566490794));
#53800=CARTESIAN_POINT('Ctrl Pts',(0.0925486672167528,-1.,-4.16373802265839));
#53801=CARTESIAN_POINT('Ctrl Pts',(0.0957412403298004,-1.,-4.15660412653577));
#53802=CARTESIAN_POINT('Ctrl Pts',(0.0988990478901223,-1.,-4.14946408918485));
#53803=CARTESIAN_POINT('Ctrl Pts',(0.102021826577584,-1.,-4.14231804939538));
#53804=CARTESIAN_POINT('Ctrl Pts',(0.105109286538945,-1.,-4.13516614458895));
#53805=CARTESIAN_POINT('Ctrl Pts',(0.108161120528369,-1.,-4.12800848371504));
#53806=CARTESIAN_POINT('Ctrl Pts',(0.111177012683346,-1.,-4.1208451250225));
#53807=CARTESIAN_POINT('Ctrl Pts',(0.114156649609545,-1.,-4.11367603924961));
#53808=CARTESIAN_POINT('Ctrl Pts',(0.117099722731648,-1.,-4.10650113381833));
#53809=CARTESIAN_POINT('Ctrl Pts',(0.120005924388124,-1.,-4.09932031767002));
#53810=CARTESIAN_POINT('Ctrl Pts',(0.122874946249107,-1.,-4.09213355850756));
#53811=CARTESIAN_POINT('Ctrl Pts',(0.12570647682254,-1.,-4.08494093372377));
#53812=CARTESIAN_POINT('Ctrl Pts',(0.128500200484837,-1.,-4.07774270738954));
#53813=CARTESIAN_POINT('Ctrl Pts',(0.13125579354894,-1.,-4.0705393152874));
#53814=CARTESIAN_POINT('Ctrl Pts',(0.133972916144245,-1.,-4.06333121018596));
#53815=CARTESIAN_POINT('Ctrl Pts',(0.136651205046119,-1.,-4.05611873400172));
#53816=CARTESIAN_POINT('Ctrl Pts',(0.139290267180057,-1.,-4.04890199238036));
#53817=CARTESIAN_POINT('Ctrl Pts',(0.1418896714855,-1.,-4.04168069633781));
#53818=CARTESIAN_POINT('Ctrl Pts',(0.144448947038344,-1.,-4.03445411510333));
#53819=CARTESIAN_POINT('Ctrl Pts',(0.146967602878994,-1.,-4.02722143146994));
#53820=CARTESIAN_POINT('Ctrl Pts',(0.149445144968707,-1.,-4.01998203715564));
#53821=CARTESIAN_POINT('Ctrl Pts',(0.15188109402291,-1.,-4.01273584234689));
#53822=CARTESIAN_POINT('Ctrl Pts',(0.15427500487231,-1.,-4.00548360245319));
#53823=CARTESIAN_POINT('Ctrl Pts',(0.156626481393734,-1.,-3.99822717425893));
#53824=CARTESIAN_POINT('Ctrl Pts',(0.158935123982793,-1.,-3.99096873945878));
#53825=CARTESIAN_POINT('Ctrl Pts',(0.161200482186084,-1.,-3.98371010319872));
#53826=CARTESIAN_POINT('Ctrl Pts',(0.163422004609999,-1.,-3.97645194630943));
#53827=CARTESIAN_POINT('Ctrl Pts',(0.165598992851102,-1.,-3.96919313621407));
#53828=CARTESIAN_POINT('Ctrl Pts',(0.167730547023319,-1.,-3.96192990160296));
#53829=CARTESIAN_POINT('Ctrl Pts',(0.169815666374139,-1.,-3.95465744665268));
#53830=CARTESIAN_POINT('Ctrl Pts',(0.17185335536924,-1.,-3.94737164900868));
#53831=CARTESIAN_POINT('Ctrl Pts',(0.173842734974609,-1.,-3.94007083096217));
#53832=CARTESIAN_POINT('Ctrl Pts',(0.175783136893868,-1.,-3.93275726771042));
#53833=CARTESIAN_POINT('Ctrl Pts',(0.177674246152317,-1.,-3.92543942697655));
#53834=CARTESIAN_POINT('Ctrl Pts',(0.179515885822881,-1.,-3.91812876180926));
#53835=CARTESIAN_POINT('Ctrl Pts',(0.181307740731785,-1.,-3.91083557557175));
#53836=CARTESIAN_POINT('Ctrl Pts',(0.18304908199319,-1.,-3.90356488555132));
#53837=CARTESIAN_POINT('Ctrl Pts',(0.184738537728043,-1.,-3.89631300742646));
#53838=CARTESIAN_POINT('Ctrl Pts',(0.18637372498528,-1.,-3.88906196725848));
#53839=CARTESIAN_POINT('Ctrl Pts',(0.187951632512685,-1.,-3.88178563496228));
#53840=CARTESIAN_POINT('Ctrl Pts',(0.189469253358272,-1.,-3.87445976418412));
#53841=CARTESIAN_POINT('Ctrl Pts',(0.19092419041862,-1.,-3.86707158624783));
#53842=CARTESIAN_POINT('Ctrl Pts',(0.19231515304497,-1.,-3.85962774407633));
#53843=CARTESIAN_POINT('Ctrl Pts',(0.193642806777723,-1.,-3.85216762263966));
#53844=CARTESIAN_POINT('Ctrl Pts',(0.19490900946022,-1.,-3.84475203346977));
#53845=CARTESIAN_POINT('Ctrl Pts',(0.196115198971859,-1.,-3.83743910616195));
#53846=CARTESIAN_POINT('Ctrl Pts',(0.197260935827361,-1.,-3.83026221776456));
#53847=CARTESIAN_POINT('Ctrl Pts',(0.198342616900486,-1.,-3.82321127349016));
#53848=CARTESIAN_POINT('Ctrl Pts',(0.199351525297447,-1.,-3.81620203429815));
#53849=CARTESIAN_POINT('Ctrl Pts',(0.200274679433364,-1.,-3.80909529318669));
#53850=CARTESIAN_POINT('Ctrl Pts',(0.201097756307326,-1.,-3.80175247447337));
#53851=CARTESIAN_POINT('Ctrl Pts',(0.201807533800837,-1.,-3.7940835418736));
#53852=CARTESIAN_POINT('Ctrl Pts',(0.20239426051216,-1.,-3.78609175019242));
#53853=CARTESIAN_POINT('Ctrl Pts',(0.202854729699081,-1.,-3.77793553476614));
#53854=CARTESIAN_POINT('Ctrl Pts',(0.203192390045164,-1.,-3.7699207159487));
#53855=CARTESIAN_POINT('Ctrl Pts',(0.203414634707478,-1.,-3.76242717936885));
#53856=CARTESIAN_POINT('Ctrl Pts',(0.203530796848321,-1.,-3.75585118707734));
#53857=CARTESIAN_POINT('Ctrl Pts',(0.203550035479166,-1.,-3.75054693397875));
#53858=CARTESIAN_POINT('Ctrl Pts',(0.203484186269415,-1.,-3.74703926501752));
#53859=CARTESIAN_POINT('Ctrl Pts',(0.203375226874121,-1.,-3.74535749969115));
#53860=CARTESIAN_POINT('Ctrl Pts',(0.203266610110531,-1.,-3.74471097893845));
#53861=CARTESIAN_POINT('Ctrl Pts',(0.203188003946657,-1.,-3.74453008995092));
#53862=CARTESIAN_POINT('Ctrl Pts',(0.2031560948961,-1.,-3.74449296983004));
#53863=CARTESIAN_POINT('',(0.385112848330761,-1.,-3.73017266276651));
#53864=CARTESIAN_POINT('Origin',(0.,-1.,0.));
#53865=CARTESIAN_POINT('',(0.581791163835815,-1.,-4.15950947128175));
#53866=CARTESIAN_POINT('Ctrl Pts',(0.385112848330761,-1.,-3.73017266276651));
#53867=CARTESIAN_POINT('Ctrl Pts',(0.385087139000374,-1.,-3.73021431755274));
#53868=CARTESIAN_POINT('Ctrl Pts',(0.385037797881504,-1.,-3.73040527621055));
#53869=CARTESIAN_POINT('Ctrl Pts',(0.385031656499164,-1.,-3.73106082862548));
#53870=CARTESIAN_POINT('Ctrl Pts',(0.385187124634206,-1.,-3.73273893363406));
#53871=CARTESIAN_POINT('Ctrl Pts',(0.385670806454565,-1.,-3.73621371845318));
#53872=CARTESIAN_POINT('Ctrl Pts',(0.386519576222251,-1.,-3.74144965781276));
#53873=CARTESIAN_POINT('Ctrl Pts',(0.387663020050836,-1.,-3.74792651696654));
#53874=CARTESIAN_POINT('Ctrl Pts',(0.389054775898701,-1.,-3.75529302895152));
#53875=CARTESIAN_POINT('Ctrl Pts',(0.390642072979559,-1.,-3.76315635033257));
#53876=CARTESIAN_POINT('Ctrl Pts',(0.392372786223432,-1.,-3.77114011595967));
#53877=CARTESIAN_POINT('Ctrl Pts',(0.394202481011499,-1.,-3.77894173114283));
#53878=CARTESIAN_POINT('Ctrl Pts',(0.39610320533484,-1.,-3.78640521279313));
#53879=CARTESIAN_POINT('Ctrl Pts',(0.398064818683969,-1.,-3.7935288716329));
#53880=CARTESIAN_POINT('Ctrl Pts',(0.4000883465046,-1.,-3.80040370384546));
#53881=CARTESIAN_POINT('Ctrl Pts',(0.402181320148435,-1.,-3.80716881962728));
#53882=CARTESIAN_POINT('Ctrl Pts',(0.404352694628273,-1.,-3.81396374287793));
#53883=CARTESIAN_POINT('Ctrl Pts',(0.406607038258985,-1.,-3.8208730391381));
#53884=CARTESIAN_POINT('Ctrl Pts',(0.408942371447459,-1.,-3.82790724256471));
#53885=CARTESIAN_POINT('Ctrl Pts',(0.411353038798518,-1.,-3.83503345578698));
#53886=CARTESIAN_POINT('Ctrl Pts',(0.413831367016748,-1.,-3.84219403994762));
#53887=CARTESIAN_POINT('Ctrl Pts',(0.416369678052906,-1.,-3.84932864157497));
#53888=CARTESIAN_POINT('Ctrl Pts',(0.418962468086773,-1.,-3.85639825647996));
#53889=CARTESIAN_POINT('Ctrl Pts',(0.421607423177534,-1.,-3.86339652542709));
#53890=CARTESIAN_POINT('Ctrl Pts',(0.42430417319511,-1.,-3.87033643487851));
#53891=CARTESIAN_POINT('Ctrl Pts',(0.427053541173457,-1.,-3.87724240306597));
#53892=CARTESIAN_POINT('Ctrl Pts',(0.429856640579741,-1.,-3.88414070943341));
#53893=CARTESIAN_POINT('Ctrl Pts',(0.432713929544458,-1.,-3.89104947940611));
#53894=CARTESIAN_POINT('Ctrl Pts',(0.435624629433527,-1.,-3.89797256655462));
#53895=CARTESIAN_POINT('Ctrl Pts',(0.438587235458249,-1.,-3.90490512938563));
#53896=CARTESIAN_POINT('Ctrl Pts',(0.441599824524054,-1.,-3.91183704069153));
#53897=CARTESIAN_POINT('Ctrl Pts',(0.44466043023059,-1.,-3.91875701610719));
#53898=CARTESIAN_POINT('Ctrl Pts',(0.447767416837292,-1.,-3.92565674143416));
#53899=CARTESIAN_POINT('Ctrl Pts',(0.450919768356348,-1.,-3.93253407403123));
#53900=CARTESIAN_POINT('Ctrl Pts',(0.454116879027584,-1.,-3.93939080846298));
#53901=CARTESIAN_POINT('Ctrl Pts',(0.457358410451682,-1.,-3.94623117206678));
#53902=CARTESIAN_POINT('Ctrl Pts',(0.460644124429121,-1.,-3.95306005817364));
#53903=CARTESIAN_POINT('Ctrl Pts',(0.463973722115733,-1.,-3.95988133243538));
#53904=CARTESIAN_POINT('Ctrl Pts',(0.467346690880643,-1.,-3.9666962227393));
#53905=CARTESIAN_POINT('Ctrl Pts',(0.470762379613439,-1.,-3.97350414289392));
#53906=CARTESIAN_POINT('Ctrl Pts',(0.474220061019509,-1.,-3.98030338044409));
#53907=CARTESIAN_POINT('Ctrl Pts',(0.477718999122027,-1.,-3.98709184306738));
#53908=CARTESIAN_POINT('Ctrl Pts',(0.481258512209675,-1.,-3.99386775880679));
#53909=CARTESIAN_POINT('Ctrl Pts',(0.484838042421834,-1.,-4.00063045119288));
#53910=CARTESIAN_POINT('Ctrl Pts',(0.488457130424633,-1.,-4.0073800839099));
#53911=CARTESIAN_POINT('Ctrl Pts',(0.492115383418018,-1.,-4.01411733503546));
#53912=CARTESIAN_POINT('Ctrl Pts',(0.495812444326251,-1.,-4.02084308851832));
#53913=CARTESIAN_POINT('Ctrl Pts',(0.499547962340821,-1.,-4.02755813980101));
#53914=CARTESIAN_POINT('Ctrl Pts',(0.503321556915346,-1.,-4.03426284174272));
#53915=CARTESIAN_POINT('Ctrl Pts',(0.507132823288136,-1.,-4.04095715148915));
#53916=CARTESIAN_POINT('Ctrl Pts',(0.51098134921897,-1.,-4.04764078815447));
#53917=CARTESIAN_POINT('Ctrl Pts',(0.514866728193016,-1.,-4.05431335771199));
#53918=CARTESIAN_POINT('Ctrl Pts',(0.518788572336923,-1.,-4.06097448038013));
#53919=CARTESIAN_POINT('Ctrl Pts',(0.522746528603107,-1.,-4.06762394471314));
#53920=CARTESIAN_POINT('Ctrl Pts',(0.526740277227498,-1.,-4.07426172299847));
#53921=CARTESIAN_POINT('Ctrl Pts',(0.53076951872857,-1.,-4.08088789536836));
#53922=CARTESIAN_POINT('Ctrl Pts',(0.534833963477273,-1.,-4.08750259988885));
#53923=CARTESIAN_POINT('Ctrl Pts',(0.538933321179755,-1.,-4.09410597627));
#53924=CARTESIAN_POINT('Ctrl Pts',(0.543067286877757,-1.,-4.10069810243979));
#53925=CARTESIAN_POINT('Ctrl Pts',(0.547235539485636,-1.,-4.10727897027977));
#53926=CARTESIAN_POINT('Ctrl Pts',(0.551437758497032,-1.,-4.11384852024721));
#53927=CARTESIAN_POINT('Ctrl Pts',(0.555673636129977,-1.,-4.12040666195664));
#53928=CARTESIAN_POINT('Ctrl Pts',(0.559942890594773,-1.,-4.12695329951961));
#53929=CARTESIAN_POINT('Ctrl Pts',(0.564245279537148,-1.,-4.13348835727104));
#53930=CARTESIAN_POINT('Ctrl Pts',(0.568580610189774,-1.,-4.14001179830547));
#53931=CARTESIAN_POINT('Ctrl Pts',(0.572948736069522,-1.,-4.14652361068081));
#53932=CARTESIAN_POINT('Ctrl Pts',(0.576469391676688,-1.,-4.151723761217));
#53933=CARTESIAN_POINT('Ctrl Pts',(0.579124568914235,-1.,-4.15561864788576));
#53934=CARTESIAN_POINT('Ctrl Pts',(0.580901211463535,-1.,-4.1582129171283));
#53935=CARTESIAN_POINT('Ctrl Pts',(0.581791163835815,-1.,-4.15950947128175));
#53936=CARTESIAN_POINT('',(0.73204283740062,-1.,-4.13571194405636));
#53937=CARTESIAN_POINT('',(0.581791163835815,-1.,-4.15950947128175));
#53938=CARTESIAN_POINT('',(0.786422660831985,-1.,-3.66661143271685));
#53939=CARTESIAN_POINT('Ctrl Pts',(0.73204283740062,-1.,-4.13571194405636));
#53940=CARTESIAN_POINT('Ctrl Pts',(0.732488575135159,-1.,-4.1342038373684));
#53941=CARTESIAN_POINT('Ctrl Pts',(0.733376589323546,-1.,-4.13118752795207));
#53942=CARTESIAN_POINT('Ctrl Pts',(0.734698226764092,-1.,-4.12666277570844));
#53943=CARTESIAN_POINT('Ctrl Pts',(0.736439634331344,-1.,-4.120629196238));
#53944=CARTESIAN_POINT('Ctrl Pts',(0.738581708225843,-1.,-4.11308626951927));
#53945=CARTESIAN_POINT('Ctrl Pts',(0.740688998553376,-1.,-4.10554241757547));
#53946=CARTESIAN_POINT('Ctrl Pts',(0.742761369689841,-1.,-4.09799769702611));
#53947=CARTESIAN_POINT('Ctrl Pts',(0.7447986497065,-1.,-4.09045220253573));
#53948=CARTESIAN_POINT('Ctrl Pts',(0.746800631492315,-1.,-4.08290608095642));
#53949=CARTESIAN_POINT('Ctrl Pts',(0.748767076680557,-1.,-4.07535951056152));
#53950=CARTESIAN_POINT('Ctrl Pts',(0.750697720484036,-1.,-4.06781267242378));
#53951=CARTESIAN_POINT('Ctrl Pts',(0.752592276483072,-1.,-4.06026572221515));
#53952=CARTESIAN_POINT('Ctrl Pts',(0.754450441816078,-1.,-4.05271876687915));
#53953=CARTESIAN_POINT('Ctrl Pts',(0.75627190236958,-1.,-4.04517182653997));
#53954=CARTESIAN_POINT('Ctrl Pts',(0.758056338884944,-1.,-4.03762485803119));
#53955=CARTESIAN_POINT('Ctrl Pts',(0.759803433243751,-1.,-4.03007781954412));
#53956=CARTESIAN_POINT('Ctrl Pts',(0.761512875859804,-1.,-4.02253072741268));
#53957=CARTESIAN_POINT('Ctrl Pts',(0.763184371182935,-1.,-4.01498370680496));
#53958=CARTESIAN_POINT('Ctrl Pts',(0.764817648785197,-1.,-4.00743706791509));
#53959=CARTESIAN_POINT('Ctrl Pts',(0.766412457136063,-1.,-3.99989129179622));
#53960=CARTESIAN_POINT('Ctrl Pts',(0.767968531377914,-1.,-3.9923468788101));
#53961=CARTESIAN_POINT('Ctrl Pts',(0.769485566245544,-1.,-3.98480422348451));
#53962=CARTESIAN_POINT('Ctrl Pts',(0.77096319003047,-1.,-3.97726349165488));
#53963=CARTESIAN_POINT('Ctrl Pts',(0.772400931772136,-1.,-3.96972446532772));
#53964=CARTESIAN_POINT('Ctrl Pts',(0.773798212026565,-1.,-3.96218649639807));
#53965=CARTESIAN_POINT('Ctrl Pts',(0.775154418039351,-1.,-3.9546488545231));
#53966=CARTESIAN_POINT('Ctrl Pts',(0.776468966697921,-1.,-3.94711101619447));
#53967=CARTESIAN_POINT('Ctrl Pts',(0.777741370568558,-1.,-3.93957296768103));
#53968=CARTESIAN_POINT('Ctrl Pts',(0.77897130813482,-1.,-3.93203552473174));
#53969=CARTESIAN_POINT('Ctrl Pts',(0.780158678615542,-1.,-3.92450058323823));
#53970=CARTESIAN_POINT('Ctrl Pts',(0.781303428618366,-1.,-3.91697036054676));
#53971=CARTESIAN_POINT('Ctrl Pts',(0.782405395622764,-1.,-3.90944671004542));
#53972=CARTESIAN_POINT('Ctrl Pts',(0.783464141529081,-1.,-3.9019303904397));
#53973=CARTESIAN_POINT('Ctrl Pts',(0.784478799358336,-1.,-3.89442039235103));
#53974=CARTESIAN_POINT('Ctrl Pts',(0.78544789034073,-1.,-3.88691313167398));
#53975=CARTESIAN_POINT('Ctrl Pts',(0.786369675812608,-1.,-3.8794040281819));
#53976=CARTESIAN_POINT('Ctrl Pts',(0.787242527617999,-1.,-3.87188916600912));
#53977=CARTESIAN_POINT('Ctrl Pts',(0.788065315093777,-1.,-3.86436702561345));
#53978=CARTESIAN_POINT('Ctrl Pts',(0.788837734090671,-1.,-3.85683995872529));
#53979=CARTESIAN_POINT('Ctrl Pts',(0.789560798155582,-1.,-3.84931637808894));
#53980=CARTESIAN_POINT('Ctrl Pts',(0.790236124191242,-1.,-3.84180762342454));
#53981=CARTESIAN_POINT('Ctrl Pts',(0.7908650127053,-1.,-3.83432392054786));
#53982=CARTESIAN_POINT('Ctrl Pts',(0.791447528662369,-1.,-3.82687033899792));
#53983=CARTESIAN_POINT('Ctrl Pts',(0.791981740718634,-1.,-3.81944345442249));
#53984=CARTESIAN_POINT('Ctrl Pts',(0.792462483517634,-1.,-3.81202588694756));
#53985=CARTESIAN_POINT('Ctrl Pts',(0.792882695234777,-1.,-3.80459229925637));
#53986=CARTESIAN_POINT('Ctrl Pts',(0.793235612973273,-1.,-3.79711921389897));
#53987=CARTESIAN_POINT('Ctrl Pts',(0.793516871680993,-1.,-3.78959439439235));
#53988=CARTESIAN_POINT('Ctrl Pts',(0.7937262357813,-1.,-3.78202460377598));
#53989=CARTESIAN_POINT('Ctrl Pts',(0.793870523787407,-1.,-3.77444863801212));
#53990=CARTESIAN_POINT('Ctrl Pts',(0.793961083688991,-1.,-3.76692626931111));
#53991=CARTESIAN_POINT('Ctrl Pts',(0.794008429134907,-1.,-3.75951468666257));
#53992=CARTESIAN_POINT('Ctrl Pts',(0.794017347371377,-1.,-3.75224692493864));
#53993=CARTESIAN_POINT('Ctrl Pts',(0.793982700459951,-1.,-3.74511357728861));
#53994=CARTESIAN_POINT('Ctrl Pts',(0.793882700937016,-1.,-3.73803280541687));
#53995=CARTESIAN_POINT('Ctrl Pts',(0.793682750269684,-1.,-3.73086914695805));
#53996=CARTESIAN_POINT('Ctrl Pts',(0.793347023784204,-1.,-3.72348797293734));
#53997=CARTESIAN_POINT('Ctrl Pts',(0.792848377370287,-1.,-3.71580242396124));
#53998=CARTESIAN_POINT('Ctrl Pts',(0.792177688845817,-1.,-3.70781724021806));
#53999=CARTESIAN_POINT('Ctrl Pts',(0.79135657569598,-1.,-3.69968940808721));
#54000=CARTESIAN_POINT('Ctrl Pts',(0.790436284988787,-1.,-3.69172044327364));
#54001=CARTESIAN_POINT('Ctrl Pts',(0.789483546064386,-1.,-3.68428439783905));
#54002=CARTESIAN_POINT('Ctrl Pts',(0.788569566220285,-1.,-3.67777119516252));
#54003=CARTESIAN_POINT('Ctrl Pts',(0.787758799995742,-1.,-3.67252923663655));
#54004=CARTESIAN_POINT('Ctrl Pts',(0.787145041181545,-1.,-3.66907505398677));
#54005=CARTESIAN_POINT('Ctrl Pts',(0.786774337198062,-1.,-3.66743103898702));
#54006=CARTESIAN_POINT('Ctrl Pts',(0.786565919558984,-1.,-3.66680946938292));
#54007=CARTESIAN_POINT('Ctrl Pts',(0.786459983895431,-1.,-3.6666431041522));
#54008=CARTESIAN_POINT('Ctrl Pts',(0.786422660831985,-1.,-3.66661143271685));
#54009=CARTESIAN_POINT('',(0.963899035117249,-1.,-3.62400312501245));
#54010=CARTESIAN_POINT('Origin',(0.,-1.,0.));
#54011=CARTESIAN_POINT('',(1.22531898815164,-1.,-4.01728681790024));
#54012=CARTESIAN_POINT('Ctrl Pts',(0.963899035117249,-1.,-3.62400312501245));
#54013=CARTESIAN_POINT('Ctrl Pts',(0.963880158555582,-1.,-3.6240482887845));
#54014=CARTESIAN_POINT('Ctrl Pts',(0.963861297423241,-1.,-3.62424461507588));
#54015=CARTESIAN_POINT('Ctrl Pts',(0.963957782642843,-1.,-3.62489305727662));
#54016=CARTESIAN_POINT('Ctrl Pts',(0.964373850166457,-1.,-3.62652618145335));
#54017=CARTESIAN_POINT('Ctrl Pts',(0.965395153165293,-1.,-3.62988252139846));
#54018=CARTESIAN_POINT('Ctrl Pts',(0.967052554541385,-1.,-3.63492122081143));
#54019=CARTESIAN_POINT('Ctrl Pts',(0.969195124675865,-1.,-3.64113946505766));
#54020=CARTESIAN_POINT('Ctrl Pts',(0.971722122061341,-1.,-3.64819756447455));
#54021=CARTESIAN_POINT('Ctrl Pts',(0.974519971354848,-1.,-3.65571576735126));
#54022=CARTESIAN_POINT('Ctrl Pts',(0.977478312751618,-1.,-3.66333049637475));
#54023=CARTESIAN_POINT('Ctrl Pts',(0.980505922458267,-1.,-3.67074983340361));
#54024=CARTESIAN_POINT('Ctrl Pts',(0.983550791470419,-1.,-3.67782408841715));
#54025=CARTESIAN_POINT('Ctrl Pts',(0.986602639863837,-1.,-3.68455317926068));
#54026=CARTESIAN_POINT('Ctrl Pts',(0.989676715398558,-1.,-3.69102682138847));
#54027=CARTESIAN_POINT('Ctrl Pts',(0.99280221833201,-1.,-3.69738123415662));
#54028=CARTESIAN_POINT('Ctrl Pts',(0.996009819772518,-1.,-3.70375282282138));
#54029=CARTESIAN_POINT('Ctrl Pts',(0.99931726075653,-1.,-3.71022439713938));
#54030=CARTESIAN_POINT('Ctrl Pts',(1.00272423396822,-1.,-3.71680667125119));
#54031=CARTESIAN_POINT('Ctrl Pts',(1.0062200073571,-1.,-3.72346803750596));
#54032=CARTESIAN_POINT('Ctrl Pts',(1.00978798539496,-1.,-3.73015276704426));
#54033=CARTESIAN_POINT('Ctrl Pts',(1.01341114319903,-1.,-3.73680245055734));
#54034=CARTESIAN_POINT('Ctrl Pts',(1.01707794311079,-1.,-3.74337942504959));
#54035=CARTESIAN_POINT('Ctrl Pts',(1.02078510487428,-1.,-3.74987777155834));
#54036=CARTESIAN_POINT('Ctrl Pts',(1.0245342944466,-1.,-3.75631037456194));
#54037=CARTESIAN_POINT('Ctrl Pts',(1.02833014458181,-1.,-3.76270122291232));
#54038=CARTESIAN_POINT('Ctrl Pts',(1.0321778660492,-1.,-3.76907609832522));
#54039=CARTESIAN_POINT('Ctrl Pts',(1.03608074678013,-1.,-3.77545283140445));
#54040=CARTESIAN_POINT('Ctrl Pts',(1.04003862055804,-1.,-3.78183535008192));
#54041=CARTESIAN_POINT('Ctrl Pts',(1.04404924374426,-1.,-3.78821910787195));
#54042=CARTESIAN_POINT('Ctrl Pts',(1.04810913267641,-1.,-3.79459440308793));
#54043=CARTESIAN_POINT('Ctrl Pts',(1.05221457990015,-1.,-3.80095039790678));
#54044=CARTESIAN_POINT('Ctrl Pts',(1.05636266918643,-1.,-3.80727913637784));
#54045=CARTESIAN_POINT('Ctrl Pts',(1.06055206187298,-1.,-3.81357866117485));
#54046=CARTESIAN_POINT('Ctrl Pts',(1.06478244038931,-1.,-3.81985083953012));
#54047=CARTESIAN_POINT('Ctrl Pts',(1.0690541318036,-1.,-3.82609989967278));
#54048=CARTESIAN_POINT('Ctrl Pts',(1.0733676663346,-1.,-3.83233071195145));
#54049=CARTESIAN_POINT('Ctrl Pts',(1.07772335353856,-1.,-3.83854714117486));
#54050=CARTESIAN_POINT('Ctrl Pts',(1.08212087917986,-1.,-3.84475048030615));
#54051=CARTESIAN_POINT('Ctrl Pts',(1.08655950846377,-1.,-3.85094025222691));
#54052=CARTESIAN_POINT('Ctrl Pts',(1.09103825516288,-1.,-3.85711487933911));
#54053=CARTESIAN_POINT('Ctrl Pts',(1.09555606505012,-1.,-3.86327241021242));
#54054=CARTESIAN_POINT('Ctrl Pts',(1.10011198761202,-1.,-3.86941120134872));
#54055=CARTESIAN_POINT('Ctrl Pts',(1.10470536603303,-1.,-3.87553067187566));
#54056=CARTESIAN_POINT('Ctrl Pts',(1.10933577224029,-1.,-3.88163105531791));
#54057=CARTESIAN_POINT('Ctrl Pts',(1.11400292434447,-1.,-3.88771308285229));
#54058=CARTESIAN_POINT('Ctrl Pts',(1.11870660794609,-1.,-3.89377768340362));
#54059=CARTESIAN_POINT('Ctrl Pts',(1.12344660099029,-1.,-3.89982569749978));
#54060=CARTESIAN_POINT('Ctrl Pts',(1.12822258281518,-1.,-3.90585753318622));
#54061=CARTESIAN_POINT('Ctrl Pts',(1.13303414693849,-1.,-3.91187321145495));
#54062=CARTESIAN_POINT('Ctrl Pts',(1.13788084225511,-1.,-3.91787251936688));
#54063=CARTESIAN_POINT('Ctrl Pts',(1.14276220561575,-1.,-3.92385513133937));
#54064=CARTESIAN_POINT('Ctrl Pts',(1.14767779451147,-1.,-3.92982073294334));
#54065=CARTESIAN_POINT('Ctrl Pts',(1.1526272271639,-1.,-3.9357691705651));
#54066=CARTESIAN_POINT('Ctrl Pts',(1.1576101834106,-1.,-3.94170046685542));
#54067=CARTESIAN_POINT('Ctrl Pts',(1.16262637999261,-1.,-3.9476147478092));
#54068=CARTESIAN_POINT('Ctrl Pts',(1.16767555244495,-1.,-3.95351219510062));
#54069=CARTESIAN_POINT('Ctrl Pts',(1.17275743590327,-1.,-3.95939299213164));
#54070=CARTESIAN_POINT('Ctrl Pts',(1.17787174135445,-1.,-3.96525726357682));
#54071=CARTESIAN_POINT('Ctrl Pts',(1.18301815039596,-1.,-3.9711050516465));
#54072=CARTESIAN_POINT('Ctrl Pts',(1.18819633715285,-1.,-3.97693634766926));
#54073=CARTESIAN_POINT('Ctrl Pts',(1.19340598349307,-1.,-3.98275111052015));
#54074=CARTESIAN_POINT('Ctrl Pts',(1.19864679609596,-1.,-3.98854928957287));
#54075=CARTESIAN_POINT('Ctrl Pts',(1.2039185237544,-1.,-3.99433084800649));
#54076=CARTESIAN_POINT('Ctrl Pts',(1.20922097030107,-1.,-4.00009577952534));
#54077=CARTESIAN_POINT('Ctrl Pts',(1.21455398918813,-1.,-4.00584409524937));
#54078=CARTESIAN_POINT('Ctrl Pts',(1.21884478244983,-1.,-4.01042947142681));
#54079=CARTESIAN_POINT('Ctrl Pts',(1.22207656456199,-1.,-4.01386104434674));
#54080=CARTESIAN_POINT('Ctrl Pts',(1.22423716681447,-1.,-4.0161454457032));
#54081=CARTESIAN_POINT('Ctrl Pts',(1.22531898815164,-1.,-4.01728681790024));
#54082=CARTESIAN_POINT('',(1.36999806084572,-1.,-3.97027773754922));
#54083=CARTESIAN_POINT('',(1.22531898815164,-1.,-4.01728681790024));
#54084=CARTESIAN_POINT('',(1.35032489087101,-1.,-3.4984457533445));
#54085=CARTESIAN_POINT('Ctrl Pts',(1.36999806084572,-1.,-3.97027773754922));
#54086=CARTESIAN_POINT('Ctrl Pts',(1.37020239094614,-1.,-3.9687184694131));
#54087=CARTESIAN_POINT('Ctrl Pts',(1.37060761745635,-1.,-3.96560037974645));
#54088=CARTESIAN_POINT('Ctrl Pts',(1.3712051561502,-1.,-3.96092458506535));
#54089=CARTESIAN_POINT('Ctrl Pts',(1.37198126432386,-1.,-3.95469287280914));
#54090=CARTESIAN_POINT('Ctrl Pts',(1.37291699202807,-1.,-3.94690771785133));
#54091=CARTESIAN_POINT('Ctrl Pts',(1.37381821967165,-1.,-3.93912709040818));
#54092=CARTESIAN_POINT('Ctrl Pts',(1.37468482215751,-1.,-3.93135106761844));
#54093=CARTESIAN_POINT('Ctrl Pts',(1.37551664448242,-1.,-3.92357976987672));
#54094=CARTESIAN_POINT('Ctrl Pts',(1.37631350505797,-1.,-3.91581337462644));
#54095=CARTESIAN_POINT('Ctrl Pts',(1.3770751963402,-1.,-3.90805209523486));
#54096=CARTESIAN_POINT('Ctrl Pts',(1.37780148512792,-1.,-3.90029615196727));
#54097=CARTESIAN_POINT('Ctrl Pts',(1.3784921128802,-1.,-3.89254574338496));
#54098=CARTESIAN_POINT('Ctrl Pts',(1.37914679719383,-1.,-3.88480102249278));
#54099=CARTESIAN_POINT('Ctrl Pts',(1.37976523097073,-1.,-3.87706205830532));
#54100=CARTESIAN_POINT('Ctrl Pts',(1.38034709213014,-1.,-3.86932885813068));
#54101=CARTESIAN_POINT('Ctrl Pts',(1.38089205992989,-1.,-3.86160143043959));
#54102=CARTESIAN_POINT('Ctrl Pts',(1.38139983115049,-1.,-3.85387983979481));
#54103=CARTESIAN_POINT('Ctrl Pts',(1.38187013346109,-1.,-3.84616425605764));
#54104=CARTESIAN_POINT('Ctrl Pts',(1.38230274828821,-1.,-3.83845502790746));
#54105=CARTESIAN_POINT('Ctrl Pts',(1.38269750245138,-1.,-3.8307526698229));
#54106=CARTESIAN_POINT('Ctrl Pts',(1.38305421262763,-1.,-3.82305771743829));
#54107=CARTESIAN_POINT('Ctrl Pts',(1.38337263902782,-1.,-3.81537060817811));
#54108=CARTESIAN_POINT('Ctrl Pts',(1.3836524404622,-1.,-3.80769156398411));
#54109=CARTESIAN_POINT('Ctrl Pts',(1.38389311766682,-1.,-3.80002044322111));
#54110=CARTESIAN_POINT('Ctrl Pts',(1.38409399694566,-1.,-3.79235669640841));
#54111=CARTESIAN_POINT('Ctrl Pts',(1.38425435883756,-1.,-3.78469969805082));
#54112=CARTESIAN_POINT('Ctrl Pts',(1.38437354551428,-1.,-3.77704902230418));
#54113=CARTESIAN_POINT('Ctrl Pts',(1.38445107339518,-1.,-3.76940473185779));
#54114=CARTESIAN_POINT('Ctrl Pts',(1.3844867525335,-1.,-3.76176768271367));
#54115=CARTESIAN_POINT('Ctrl Pts',(1.38448077997163,-1.,-3.7541397631875));
#54116=CARTESIAN_POINT('Ctrl Pts',(1.38443344984394,-1.,-3.74652317167876));
#54117=CARTESIAN_POINT('Ctrl Pts',(1.38434489156458,-1.,-3.73891976418104));
#54118=CARTESIAN_POINT('Ctrl Pts',(1.38421479111531,-1.,-3.73133035859282));
#54119=CARTESIAN_POINT('Ctrl Pts',(1.3840421342895,-1.,-3.72375409358803));
#54120=CARTESIAN_POINT('Ctrl Pts',(1.38382489984586,-1.,-3.7161876605181));
#54121=CARTESIAN_POINT('Ctrl Pts',(1.38356065402124,-1.,-3.70862680753347));
#54122=CARTESIAN_POINT('Ctrl Pts',(1.38324717612865,-1.,-3.701067921679));
#54123=CARTESIAN_POINT('Ctrl Pts',(1.3828831117165,-1.,-3.69350967899526));
#54124=CARTESIAN_POINT('Ctrl Pts',(1.38246852827182,-1.,-3.68595444983838));
#54125=CARTESIAN_POINT('Ctrl Pts',(1.3820057429062,-1.,-3.67841038482414));
#54126=CARTESIAN_POINT('Ctrl Pts',(1.38149812653868,-1.,-3.67088843112262));
#54127=CARTESIAN_POINT('Ctrl Pts',(1.38094856333552,-1.,-3.66339848520857));
#54128=CARTESIAN_POINT('Ctrl Pts',(1.38035791051212,-1.,-3.6559455440439));
#54129=CARTESIAN_POINT('Ctrl Pts',(1.37972372481603,-1.,-3.64852652756456));
#54130=CARTESIAN_POINT('Ctrl Pts',(1.37903818567359,-1.,-3.64112507791141));
#54131=CARTESIAN_POINT('Ctrl Pts',(1.37829035457339,-1.,-3.63371727442486));
#54132=CARTESIAN_POINT('Ctrl Pts',(1.37746987919881,-1.,-3.62628098665145));
#54133=CARTESIAN_POINT('Ctrl Pts',(1.37657053403107,-1.,-3.61880481160421));
#54134=CARTESIAN_POINT('Ctrl Pts',(1.37559314436634,-1.,-3.61129546591064));
#54135=CARTESIAN_POINT('Ctrl Pts',(1.37455051379623,-1.,-3.60379020123988));
#54136=CARTESIAN_POINT('Ctrl Pts',(1.37346320103157,-1.,-3.59634627869048));
#54137=CARTESIAN_POINT('Ctrl Pts',(1.37235053660976,-1.,-3.58901853846365));
#54138=CARTESIAN_POINT('Ctrl Pts',(1.37122241663062,-1.,-3.58183885982715));
#54139=CARTESIAN_POINT('Ctrl Pts',(1.37007229485659,-1.,-3.57479875549486));
#54140=CARTESIAN_POINT('Ctrl Pts',(1.36886584973389,-1.,-3.5678208030466));
#54141=CARTESIAN_POINT('Ctrl Pts',(1.36754771771233,-1.,-3.56077662028649));
#54142=CARTESIAN_POINT('Ctrl Pts',(1.3660614545677,-1.,-3.55353883995949));
#54143=CARTESIAN_POINT('Ctrl Pts',(1.36436666257597,-1.,-3.54602591832973));
#54144=CARTESIAN_POINT('Ctrl Pts',(1.36245507339307,-1.,-3.53824396424961));
#54145=CARTESIAN_POINT('Ctrl Pts',(1.36037259643734,-1.,-3.530344649616));
#54146=CARTESIAN_POINT('Ctrl Pts',(1.35821701528836,-1.,-3.52261776116748));
#54147=CARTESIAN_POINT('Ctrl Pts',(1.35611275237152,-1.,-3.51542230699556));
#54148=CARTESIAN_POINT('Ctrl Pts',(1.35419113575956,-1.,-3.50913227059999));
#54149=CARTESIAN_POINT('Ctrl Pts',(1.35257032843486,-1.,-3.50408168106261));
#54150=CARTESIAN_POINT('Ctrl Pts',(1.35142377279517,-1.,-3.5007660381649));
#54151=CARTESIAN_POINT('Ctrl Pts',(1.35080045218586,-1.,-3.49920025459723));
#54152=CARTESIAN_POINT('Ctrl Pts',(1.35049736560527,-1.,-3.49861894124827));
#54153=CARTESIAN_POINT('Ctrl Pts',(1.35036670892966,-1.,-3.49847119623846));
#54154=CARTESIAN_POINT('Ctrl Pts',(1.35032489087101,-1.,-3.4984457533445));
#54155=CARTESIAN_POINT('',(1.51895082866166,-1.,-3.42859860294378));
#54156=CARTESIAN_POINT('Origin',(0.,-1.,0.));
#54157=CARTESIAN_POINT('',(1.83867539237861,-1.,-3.77614523045147));
#54158=CARTESIAN_POINT('Ctrl Pts',(1.51895082866166,-1.,-3.42859860294378));
#54159=CARTESIAN_POINT('Ctrl Pts',(1.51893924967231,-1.,-3.42864616361967));
#54160=CARTESIAN_POINT('Ctrl Pts',(1.51895133295017,-1.,-3.42884302333978));
#54161=CARTESIAN_POINT('Ctrl Pts',(1.51914806898539,-1.,-3.42946838852728));
#54162=CARTESIAN_POINT('Ctrl Pts',(1.5198144909343,-1.,-3.43101631893491));
#54163=CARTESIAN_POINT('Ctrl Pts',(1.52134826724227,-1.,-3.43417156977749));
#54164=CARTESIAN_POINT('Ctrl Pts',(1.52377348950429,-1.,-3.43888895974182));
#54165=CARTESIAN_POINT('Ctrl Pts',(1.52686242875717,-1.,-3.44469547527));
#54166=CARTESIAN_POINT('Ctrl Pts',(1.530462444618,-1.,-3.45127136828667));
#54167=CARTESIAN_POINT('Ctrl Pts',(1.53440195378902,-1.,-3.45825932955273));
#54168=CARTESIAN_POINT('Ctrl Pts',(1.53851507915533,-1.,-3.46531752207222));
#54169=CARTESIAN_POINT('Ctrl Pts',(1.54266605398152,-1.,-3.47217189224576));
#54170=CARTESIAN_POINT('Ctrl Pts',(1.54678009290206,-1.,-3.47868272898599));
#54171=CARTESIAN_POINT('Ctrl Pts',(1.55084702970382,-1.,-3.48485155928414));
#54172=CARTESIAN_POINT('Ctrl Pts',(1.5548959590107,-1.,-3.49076460877317));
#54173=CARTESIAN_POINT('Ctrl Pts',(1.55897703097859,-1.,-3.49655185179623));
#54174=CARTESIAN_POINT('Ctrl Pts',(1.56314187758689,-1.,-3.50234321621607));
#54175=CARTESIAN_POINT('Ctrl Pts',(1.56742097575041,-1.,-3.50821771695427));
#54176=CARTESIAN_POINT('Ctrl Pts',(1.57181569799774,-1.,-3.51418598431733));
#54177=CARTESIAN_POINT('Ctrl Pts',(1.5763104998818,-1.,-3.52021847865961));
#54178=CARTESIAN_POINT('Ctrl Pts',(1.58088027227856,-1.,-3.52626275334899));
#54179=CARTESIAN_POINT('Ctrl Pts',(1.58549906268083,-1.,-3.53226378147068));
#54180=CARTESIAN_POINT('Ctrl Pts',(1.59014958368725,-1.,-3.53818616861045));
#54181=CARTESIAN_POINT('Ctrl Pts',(1.5948276694975,-1.,-3.544024581823));
#54182=CARTESIAN_POINT('Ctrl Pts',(1.59953698113444,-1.,-3.54979148634426));
#54183=CARTESIAN_POINT('Ctrl Pts',(1.60428584699848,-1.,-3.55550985096117));
#54184=CARTESIAN_POINT('Ctrl Pts',(1.60908344685459,-1.,-3.56120432482986));
#54185=CARTESIAN_POINT('Ctrl Pts',(1.61393581747522,-1.,-3.56689200468404));
#54186=CARTESIAN_POINT('Ctrl Pts',(1.61884340915412,-1.,-3.57257679609826));
#54187=CARTESIAN_POINT('Ctrl Pts',(1.62380329464851,-1.,-3.57825455954405));
#54188=CARTESIAN_POINT('Ctrl Pts',(1.62881051550748,-1.,-3.5839162577435));
#54189=CARTESIAN_POINT('Ctrl Pts',(1.63385971451259,-1.,-3.58955176627876));
#54190=CARTESIAN_POINT('Ctrl Pts',(1.63894676675349,-1.,-3.59515368334887));
#54191=CARTESIAN_POINT('Ctrl Pts',(1.6440700438558,-1.,-3.6007202851384));
#54192=CARTESIAN_POINT('Ctrl Pts',(1.64922952425833,-1.,-3.60625346556992));
#54193=CARTESIAN_POINT('Ctrl Pts',(1.65442619244327,-1.,-3.61175734965129));
#54194=CARTESIAN_POINT('Ctrl Pts',(1.65966133399186,-1.,-3.61723666482457));
#54195=CARTESIAN_POINT('Ctrl Pts',(1.66493585923853,-1.,-3.62269517989104));
#54196=CARTESIAN_POINT('Ctrl Pts',(1.67024966008037,-1.,-3.62813422105257));
#54197=CARTESIAN_POINT('Ctrl Pts',(1.67560193613145,-1.,-3.63355343201211));
#54198=CARTESIAN_POINT('Ctrl Pts',(1.68099146651577,-1.,-3.63895140887443));
#54199=CARTESIAN_POINT('Ctrl Pts',(1.68641690471455,-1.,-3.64432638915199));
#54200=CARTESIAN_POINT('Ctrl Pts',(1.691877054817,-1.,-3.64967689827393));
#54201=CARTESIAN_POINT('Ctrl Pts',(1.69737117722558,-1.,-3.65500246526798));
#54202=CARTESIAN_POINT('Ctrl Pts',(1.70289888566904,-1.,-3.6603033877491));
#54203=CARTESIAN_POINT('Ctrl Pts',(1.70846001610983,-1.,-3.6655804319893));
#54204=CARTESIAN_POINT('Ctrl Pts',(1.71405450210392,-1.,-3.67083454901629));
#54205=CARTESIAN_POINT('Ctrl Pts',(1.71968225581787,-1.,-3.67606660374665));
#54206=CARTESIAN_POINT('Ctrl Pts',(1.72534302437003,-1.,-3.68127704936472));
#54207=CARTESIAN_POINT('Ctrl Pts',(1.73103640956647,-1.,-3.68646597019188));
#54208=CARTESIAN_POINT('Ctrl Pts',(1.73676193254493,-1.,-3.69163322647906));
#54209=CARTESIAN_POINT('Ctrl Pts',(1.74251908492589,-1.,-3.6967785691046));
#54210=CARTESIAN_POINT('Ctrl Pts',(1.74830738046092,-1.,-3.70190175673422));
#54211=CARTESIAN_POINT('Ctrl Pts',(1.75412641804148,-1.,-3.70700269736876));
#54212=CARTESIAN_POINT('Ctrl Pts',(1.75997588499021,-1.,-3.71208146346455));
#54213=CARTESIAN_POINT('Ctrl Pts',(1.76585552124549,-1.,-3.71713822377676));
#54214=CARTESIAN_POINT('Ctrl Pts',(1.77176509401846,-1.,-3.72217319911429));
#54215=CARTESIAN_POINT('Ctrl Pts',(1.77770437039606,-1.,-3.72718661205504));
#54216=CARTESIAN_POINT('Ctrl Pts',(1.78367308442682,-1.,-3.73217863095022));
#54217=CARTESIAN_POINT('Ctrl Pts',(1.78967092823139,-1.,-3.73714934729962));
#54218=CARTESIAN_POINT('Ctrl Pts',(1.79569757859041,-1.,-3.74209880351667));
#54219=CARTESIAN_POINT('Ctrl Pts',(1.80175271485519,-1.,-3.74702700874954));
#54220=CARTESIAN_POINT('Ctrl Pts',(1.80783603939662,-1.,-3.75193395888069));
#54221=CARTESIAN_POINT('Ctrl Pts',(1.81394729834032,-1.,-3.75681965683995));
#54222=CARTESIAN_POINT('Ctrl Pts',(1.82008629694924,-1.,-3.76168412709652));
#54223=CARTESIAN_POINT('Ctrl Pts',(1.82625289221933,-1.,-3.76652740355856));
#54224=CARTESIAN_POINT('Ctrl Pts',(1.83120816956515,-1.,-3.77038509819777));
#54225=CARTESIAN_POINT('Ctrl Pts',(1.83493697935064,-1.,-3.77326886065484));
#54226=CARTESIAN_POINT('Ctrl Pts',(1.83742834010821,-1.,-3.77518714458232));
#54227=CARTESIAN_POINT('Ctrl Pts',(1.83867539237861,-1.,-3.77614523045147));
#54228=CARTESIAN_POINT('',(1.97421938526992,-1.,-3.70708211654725));
#54229=CARTESIAN_POINT('',(1.83867539237861,-1.,-3.77614523045147));
#54230=CARTESIAN_POINT('',(1.88097764062541,-1.,-3.24413672884902));
#54231=CARTESIAN_POINT('Ctrl Pts',(1.97421938526992,-1.,-3.70708211654725));
#54232=CARTESIAN_POINT('Ctrl Pts',(1.974177276451,-1.,-3.7055100813194));
#54233=CARTESIAN_POINT('Ctrl Pts',(1.97408973726149,-1.,-3.70236698911837));
#54234=CARTESIAN_POINT('Ctrl Pts',(1.97394846382288,-1.,-3.69765528558292));
#54235=CARTESIAN_POINT('Ctrl Pts',(1.97374016224397,-1.,-3.69137888597855));
#54236=CARTESIAN_POINT('Ctrl Pts',(1.9734465030363,-1.,-3.68354319913416));
#54237=CARTESIAN_POINT('Ctrl Pts',(1.97311947678035,-1.,-3.67571738106175));
#54238=CARTESIAN_POINT('Ctrl Pts',(1.9727589719863,-1.,-3.66790152751984));
#54239=CARTESIAN_POINT('Ctrl Pts',(1.97236485439317,-1.,-3.66009578166865));
#54240=CARTESIAN_POINT('Ctrl Pts',(1.97193697240645,-1.,-3.65230034717364));
#54241=CARTESIAN_POINT('Ctrl Pts',(1.97147515441539,-1.,-3.64451546724222));
#54242=CARTESIAN_POINT('Ctrl Pts',(1.97097920454698,-1.,-3.63674139590853));
#54243=CARTESIAN_POINT('Ctrl Pts',(1.97044889850518,-1.,-3.62897836973397));
#54244=CARTESIAN_POINT('Ctrl Pts',(1.96988398129888,-1.,-3.62122658401722));
#54245=CARTESIAN_POINT('Ctrl Pts',(1.96928416040712,-1.,-3.61348615496393));
#54246=CARTESIAN_POINT('Ctrl Pts',(1.96864911885775,-1.,-3.60575714017676));
#54247=CARTESIAN_POINT('Ctrl Pts',(1.96797854118257,-1.,-3.59803959819725));
#54248=CARTESIAN_POINT('Ctrl Pts',(1.96727213799507,-1.,-3.5903336402273));
#54249=CARTESIAN_POINT('Ctrl Pts',(1.9665296668894,-1.,-3.58263947663884));
#54250=CARTESIAN_POINT('Ctrl Pts',(1.96575096652857,-1.,-3.57495748601088));
#54251=CARTESIAN_POINT('Ctrl Pts',(1.96493594634643,-1.,-3.56728820357933));
#54252=CARTESIAN_POINT('Ctrl Pts',(1.96408450906868,-1.,-3.55963218706201));
#54253=CARTESIAN_POINT('Ctrl Pts',(1.96319648628667,-1.,-3.55198990600929));
#54254=CARTESIAN_POINT('Ctrl Pts',(1.96227157573058,-1.,-3.54436163300425));
#54255=CARTESIAN_POINT('Ctrl Pts',(1.96130926212661,-1.,-3.53674730625759));
#54256=CARTESIAN_POINT('Ctrl Pts',(1.96030879411534,-1.,-3.52914648844289));
#54257=CARTESIAN_POINT('Ctrl Pts',(1.95926936324436,-1.,-3.52155867431438));
#54258=CARTESIAN_POINT('Ctrl Pts',(1.95819025316768,-1.,-3.51398354617773));
#54259=CARTESIAN_POINT('Ctrl Pts',(1.95707099606513,-1.,-3.50642124159913));
#54260=CARTESIAN_POINT('Ctrl Pts',(1.9559115382367,-1.,-3.49887263575602));
#54261=CARTESIAN_POINT('Ctrl Pts',(1.95471236969653,-1.,-3.49133956289154));
#54262=CARTESIAN_POINT('Ctrl Pts',(1.95347412486316,-1.,-3.48382414832649));
#54263=CARTESIAN_POINT('Ctrl Pts',(1.95219722189878,-1.,-3.47632820495926));
#54264=CARTESIAN_POINT('Ctrl Pts',(1.95088147859876,-1.,-3.4688525897419));
#54265=CARTESIAN_POINT('Ctrl Pts',(1.94952575850196,-1.,-3.46139661060959));
#54266=CARTESIAN_POINT('Ctrl Pts',(1.94812754766524,-1.,-3.45395731584051));
#54267=CARTESIAN_POINT('Ctrl Pts',(1.94668377715332,-1.,-3.44653088665685));
#54268=CARTESIAN_POINT('Ctrl Pts',(1.94519168842883,-1.,-3.43911410197693));
#54269=CARTESIAN_POINT('Ctrl Pts',(1.94364973660285,-1.,-3.43170586602436));
#54270=CARTESIAN_POINT('Ctrl Pts',(1.94205835913692,-1.,-3.42430850941497));
#54271=CARTESIAN_POINT('Ctrl Pts',(1.94042111965237,-1.,-3.41692971994082));
#54272=CARTESIAN_POINT('Ctrl Pts',(1.93874306008132,-1.,-3.40957978266623));
#54273=CARTESIAN_POINT('Ctrl Pts',(1.93702857723089,-1.,-3.40226802104093));
#54274=CARTESIAN_POINT('Ctrl Pts',(1.93527929945982,-1.,-3.39499923640789));
#54275=CARTESIAN_POINT('Ctrl Pts',(1.93349233176794,-1.,-3.38777076883267));
#54276=CARTESIAN_POINT('Ctrl Pts',(1.93165739093292,-1.,-3.38056768525577));
#54277=CARTESIAN_POINT('Ctrl Pts',(1.92975993109897,-1.,-3.37336807068078));
#54278=CARTESIAN_POINT('Ctrl Pts',(1.92778626543803,-1.,-3.36615168657597));
#54279=CARTESIAN_POINT('Ctrl Pts',(1.92572846125763,-1.,-3.35890824422976));
#54280=CARTESIAN_POINT('Ctrl Pts',(1.92358838440518,-1.,-3.35164424847207));
#54281=CARTESIAN_POINT('Ctrl Pts',(1.92138450828378,-1.,-3.34439448941915));
#54282=CARTESIAN_POINT('Ctrl Pts',(1.91914609610173,-1.,-3.33721230709948));
#54283=CARTESIAN_POINT('Ctrl Pts',(1.91690081930297,-1.,-3.33014884257812));
#54284=CARTESIAN_POINT('Ctrl Pts',(1.91466343916612,-1.,-3.32323403454507));
#54285=CARTESIAN_POINT('Ctrl Pts',(1.91242616234459,-1.,-3.31646052426395));
#54286=CARTESIAN_POINT('Ctrl Pts',(1.91014297830502,-1.,-3.30975721158694));
#54287=CARTESIAN_POINT('Ctrl Pts',(1.90773912171424,-1.,-3.30300595568341));
#54288=CARTESIAN_POINT('Ctrl Pts',(1.9051389186417,-1.,-3.29608978722258));
#54289=CARTESIAN_POINT('Ctrl Pts',(1.9022897124757,-1.,-3.28893448600364));
#54290=CARTESIAN_POINT('Ctrl Pts',(1.89918429230424,-1.,-3.28154737912287));
#54291=CARTESIAN_POINT('Ctrl Pts',(1.89589172903662,-1.,-3.27407108932908));
#54292=CARTESIAN_POINT('Ctrl Pts',(1.89255393500769,-1.,-3.2667765388833));
#54293=CARTESIAN_POINT('Ctrl Pts',(1.88934996203508,-1.,-3.2599988519361));
#54294=CARTESIAN_POINT('Ctrl Pts',(1.88646802523372,-1.,-3.25408686339298));
#54295=CARTESIAN_POINT('Ctrl Pts',(1.88407708646435,-1.,-3.24935200512055));
#54296=CARTESIAN_POINT('Ctrl Pts',(1.88242596600422,-1.,-3.24625654410705));
#54297=CARTESIAN_POINT('Ctrl Pts',(1.88156537699118,-1.,-3.24480754675942));
#54298=CARTESIAN_POINT('Ctrl Pts',(1.88117508446657,-1.,-3.24428080352952));
#54299=CARTESIAN_POINT('Ctrl Pts',(1.88102292397987,-1.,-3.24415531671311));
#54300=CARTESIAN_POINT('Ctrl Pts',(1.88097764062541,-1.,-3.24413672884902));
#54301=CARTESIAN_POINT('',(2.03660101169564,-1.,-3.14877060440425));
#54302=CARTESIAN_POINT('Origin',(0.,-1.,0.));
#54303=CARTESIAN_POINT('',(2.40675750623143,-1.,-3.44202241512147));
#54304=CARTESIAN_POINT('Ctrl Pts',(2.03660101169564,-1.,-3.14877060440425));
#54305=CARTESIAN_POINT('Ctrl Pts',(2.03659701539175,-1.,-3.1488193908823));
#54306=CARTESIAN_POINT('Ctrl Pts',(2.03663974554941,-1.,-3.14901193669147));
#54307=CARTESIAN_POINT('Ctrl Pts',(2.03693188810614,-1.,-3.14959882629936));
#54308=CARTESIAN_POINT('Ctrl Pts',(2.03783225496023,-1.,-3.15102344775396));
#54309=CARTESIAN_POINT('Ctrl Pts',(2.03984073791432,-1.,-3.1538999167466));
#54310=CARTESIAN_POINT('Ctrl Pts',(2.04297406404132,-1.,-3.15817983946525));
#54311=CARTESIAN_POINT('Ctrl Pts',(2.0469333124766,-1.,-3.16343165059235));
#54312=CARTESIAN_POINT('Ctrl Pts',(2.05151770247452,-1.,-3.16936341689859));
#54313=CARTESIAN_POINT('Ctrl Pts',(2.05650186773279,-1.,-3.17564906975592));
#54314=CARTESIAN_POINT('Ctrl Pts',(2.06166849827143,-1.,-3.18197692964677));
#54315=CARTESIAN_POINT('Ctrl Pts',(2.06684062744065,-1.,-3.18809755562297));
#54316=CARTESIAN_POINT('Ctrl Pts',(2.07192253497765,-1.,-3.19388465568113));
#54317=CARTESIAN_POINT('Ctrl Pts',(2.0769044187063,-1.,-3.19934132835879));
#54318=CARTESIAN_POINT('Ctrl Pts',(2.08182850370816,-1.,-3.20454818630635));
#54319=CARTESIAN_POINT('Ctrl Pts',(2.08676465517435,-1.,-3.20962575845433));
#54320=CARTESIAN_POINT('Ctrl Pts',(2.0917841946046,-1.,-3.2146942960168));
#54321=CARTESIAN_POINT('Ctrl Pts',(2.09692958434933,-1.,-3.21982707347067));
#54322=CARTESIAN_POINT('Ctrl Pts',(2.10220384298533,-1.,-3.22503437553496));
#54323=CARTESIAN_POINT('Ctrl Pts',(2.1075869964248,-1.,-3.23028945793334));
#54324=CARTESIAN_POINT('Ctrl Pts',(2.11304604021784,-1.,-3.23554444767115));
#54325=CARTESIAN_POINT('Ctrl Pts',(2.11854673326972,-1.,-3.24074905517282));
#54326=CARTESIAN_POINT('Ctrl Pts',(2.12406646410943,-1.,-3.24587102613347));
#54327=CARTESIAN_POINT('Ctrl Pts',(2.1296002839681,-1.,-3.25090574493994));
#54328=CARTESIAN_POINT('Ctrl Pts',(2.13515375878786,-1.,-3.25586495065027));
#54329=CARTESIAN_POINT('Ctrl Pts',(2.14073870754257,-1.,-3.26077002641868));
#54330=CARTESIAN_POINT('Ctrl Pts',(2.14636805295663,-1.,-3.26564388189764));
#54331=CARTESIAN_POINT('Ctrl Pts',(2.15205043199818,-1.,-3.27050245897244));
#54332=CARTESIAN_POINT('Ctrl Pts',(2.15778690038359,-1.,-3.27534954469206));
#54333=CARTESIAN_POINT('Ctrl Pts',(2.16357391934434,-1.,-3.28018150841414));
#54334=CARTESIAN_POINT('Ctrl Pts',(2.16940517773459,-1.,-3.2849901997973));
#54335=CARTESIAN_POINT('Ctrl Pts',(2.17527380048422,-1.,-3.28976645712566));
#54336=CARTESIAN_POINT('Ctrl Pts',(2.18117455557062,-1.,-3.29450361500484));
#54337=CARTESIAN_POINT('Ctrl Pts',(2.18710556500325,-1.,-3.29920022557635));
#54338=CARTESIAN_POINT('Ctrl Pts',(2.19306710376112,-1.,-3.30385816281831));
#54339=CARTESIAN_POINT('Ctrl Pts',(2.19906078949924,-1.,-3.30848134694597));
#54340=CARTESIAN_POINT('Ctrl Pts',(2.20508863150608,-1.,-3.3130742460895));
#54341=CARTESIAN_POINT('Ctrl Pts',(2.21115211847872,-1.,-3.31764044024231));
#54342=CARTESIAN_POINT('Ctrl Pts',(2.21725135110889,-1.,-3.32218125618955));
#54343=CARTESIAN_POINT('Ctrl Pts',(2.22338548312758,-1.,-3.32669646722871));
#54344=CARTESIAN_POINT('Ctrl Pts',(2.22955308907221,-1.,-3.33118487773593));
#54345=CARTESIAN_POINT('Ctrl Pts',(2.23575256328809,-1.,-3.33564495756478));
#54346=CARTESIAN_POINT('Ctrl Pts',(2.24198249391437,-1.,-3.34007543738044));
#54347=CARTESIAN_POINT('Ctrl Pts',(2.24824207678287,-1.,-3.34447596770768));
#54348=CARTESIAN_POINT('Ctrl Pts',(2.25453097693524,-1.,-3.34884690292342));
#54349=CARTESIAN_POINT('Ctrl Pts',(2.26084915222484,-1.,-3.35318902552676));
#54350=CARTESIAN_POINT('Ctrl Pts',(2.26719668579921,-1.,-3.35750328523077));
#54351=CARTESIAN_POINT('Ctrl Pts',(2.27357362620902,-1.,-3.36179055004369));
#54352=CARTESIAN_POINT('Ctrl Pts',(2.27997979457968,-1.,-3.36605130712978));
#54353=CARTESIAN_POINT('Ctrl Pts',(2.28641481081045,-1.,-3.37028570206357));
#54354=CARTESIAN_POINT('Ctrl Pts',(2.2928781800731,-1.,-3.37449367172707));
#54355=CARTESIAN_POINT('Ctrl Pts',(2.29936936127588,-1.,-3.37867504959382));
#54356=CARTESIAN_POINT('Ctrl Pts',(2.30588783640389,-1.,-3.38282967336676));
#54357=CARTESIAN_POINT('Ctrl Pts',(2.31243319489505,-1.,-3.38695751492659));
#54358=CARTESIAN_POINT('Ctrl Pts',(2.31900513925627,-1.,-3.39105869475112));
#54359=CARTESIAN_POINT('Ctrl Pts',(2.32560343902683,-1.,-3.39513342020045));
#54360=CARTESIAN_POINT('Ctrl Pts',(2.33222789882601,-1.,-3.39918194578115));
#54361=CARTESIAN_POINT('Ctrl Pts',(2.33887832342715,-1.,-3.40320452776646));
#54362=CARTESIAN_POINT('Ctrl Pts',(2.34555447648901,-1.,-3.40720137403888));
#54363=CARTESIAN_POINT('Ctrl Pts',(2.35225606823649,-1.,-3.41117262313464));
#54364=CARTESIAN_POINT('Ctrl Pts',(2.35898278606449,-1.,-3.4151183675076));
#54365=CARTESIAN_POINT('Ctrl Pts',(2.36573431470313,-1.,-3.41903866635384));
#54366=CARTESIAN_POINT('Ctrl Pts',(2.37251035954351,-1.,-3.42293356216595));
#54367=CARTESIAN_POINT('Ctrl Pts',(2.37931067029517,-1.,-3.42680309755241));
#54368=CARTESIAN_POINT('Ctrl Pts',(2.38613505844641,-1.,-3.43064732714472));
#54369=CARTESIAN_POINT('Ctrl Pts',(2.39298338805823,-1.,-3.43446630680436));
#54370=CARTESIAN_POINT('Ctrl Pts',(2.39848113411428,-1.,-3.43750133066037));
#54371=CARTESIAN_POINT('Ctrl Pts',(2.40261515590099,-1.,-3.43976627485223));
#54372=CARTESIAN_POINT('Ctrl Pts',(2.40537592959345,-1.,-3.44127120683402));
#54373=CARTESIAN_POINT('Ctrl Pts',(2.40675750623143,-1.,-3.44202241512147));
#54374=CARTESIAN_POINT('',(2.52982887637028,-1.,-3.35260583073571));
#54375=CARTESIAN_POINT('',(2.40675750623143,-1.,-3.44202241512147));
#54376=CARTESIAN_POINT('',(2.36531447826073,-1.,-2.90994629141676));
#54377=CARTESIAN_POINT('Ctrl Pts',(2.52982887637028,-1.,-3.35260583073571));
#54378=CARTESIAN_POINT('Ctrl Pts',(2.5295413654909,-1.,-3.35105973714072));
#54379=CARTESIAN_POINT('Ctrl Pts',(2.52896321610703,-1.,-3.34796903576663));
#54380=CARTESIAN_POINT('Ctrl Pts',(2.52808660915689,-1.,-3.34333744115511));
#54381=CARTESIAN_POINT('Ctrl Pts',(2.52689902690158,-1.,-3.33717089999103));
#54382=CARTESIAN_POINT('Ctrl Pts',(2.52538321164634,-1.,-3.32947762187533));
#54383=CARTESIAN_POINT('Ctrl Pts',(2.5238359839626,-1.,-3.32179931078699));
#54384=CARTESIAN_POINT('Ctrl Pts',(2.52225724871313,-1.,-3.31413607874645));
#54385=CARTESIAN_POINT('Ctrl Pts',(2.52064689568511,-1.,-3.30648808815443));
#54386=CARTESIAN_POINT('Ctrl Pts',(2.51900480701068,-1.,-3.29885556388353));
#54387=CARTESIAN_POINT('Ctrl Pts',(2.51733085123797,-1.,-3.2912387729927));
#54388=CARTESIAN_POINT('Ctrl Pts',(2.51562487464514,-1.,-3.28363799702982));
#54389=CARTESIAN_POINT('Ctrl Pts',(2.513886692704,-1.,-3.27605350473142));
#54390=CARTESIAN_POINT('Ctrl Pts',(2.51211608411423,-1.,-3.26848552888116));
#54391=CARTESIAN_POINT('Ctrl Pts',(2.51031277813486,-1.,-3.26093423001434));
#54392=CARTESIAN_POINT('Ctrl Pts',(2.50847647070723,-1.,-3.25339971460982));
#54393=CARTESIAN_POINT('Ctrl Pts',(2.506606859405,-1.,-3.24588208983849));
#54394=CARTESIAN_POINT('Ctrl Pts',(2.5047036758003,-1.,-3.23838151080319));
#54395=CARTESIAN_POINT('Ctrl Pts',(2.50276671338111,-1.,-3.23089822320646));
#54396=CARTESIAN_POINT('Ctrl Pts',(2.50079587201957,-1.,-3.22343262620503));
#54397=CARTESIAN_POINT('Ctrl Pts',(2.4987911459939,-1.,-3.21598526261286));
#54398=CARTESIAN_POINT('Ctrl Pts',(2.4967525264737,-1.,-3.20855669849836));
#54399=CARTESIAN_POINT('Ctrl Pts',(2.49467992057755,-1.,-3.20114742397588));
#54400=CARTESIAN_POINT('Ctrl Pts',(2.49257307239848,-1.,-3.19375775555798));
#54401=CARTESIAN_POINT('Ctrl Pts',(2.49043146334059,-1.,-3.18638771282266));
#54402=CARTESIAN_POINT('Ctrl Pts',(2.48825428288201,-1.,-3.17903698136622));
#54403=CARTESIAN_POINT('Ctrl Pts',(2.48604065348587,-1.,-3.17170518863313));
#54404=CARTESIAN_POINT('Ctrl Pts',(2.48378981792725,-1.,-3.16439213290161));
#54405=CARTESIAN_POINT('Ctrl Pts',(2.48150133566571,-1.,-3.15709802322739));
#54406=CARTESIAN_POINT('Ctrl Pts',(2.47917529057029,-1.,-3.14982373241352));
#54407=CARTESIAN_POINT('Ctrl Pts',(2.47681245356109,-1.,-3.1425709954655));
#54408=CARTESIAN_POINT('Ctrl Pts',(2.47441378371932,-1.,-3.13534181229295));
#54409=CARTESIAN_POINT('Ctrl Pts',(2.47197997765871,-1.,-3.12813790805952));
#54410=CARTESIAN_POINT('Ctrl Pts',(2.46951098947469,-1.,-3.12096015766983));
#54411=CARTESIAN_POINT('Ctrl Pts',(2.46700558843506,-1.,-3.11380805536122));
#54412=CARTESIAN_POINT('Ctrl Pts',(2.46446082979646,-1.,-3.1066790790198));
#54413=CARTESIAN_POINT('Ctrl Pts',(2.46187308501884,-1.,-3.09956993697052));
#54414=CARTESIAN_POINT('Ctrl Pts',(2.4592391256388,-1.,-3.09247787931887));
#54415=CARTESIAN_POINT('Ctrl Pts',(2.45655725437039,-1.,-3.08540206545315));
#54416=CARTESIAN_POINT('Ctrl Pts',(2.4538282678779,-1.,-3.07834472886139));
#54417=CARTESIAN_POINT('Ctrl Pts',(2.45105688854422,-1.,-3.07131290521297));
#54418=CARTESIAN_POINT('Ctrl Pts',(2.44824970516543,-1.,-3.06431596421405));
#54419=CARTESIAN_POINT('Ctrl Pts',(2.44541251892556,-1.,-3.05736242671506));
#54420=CARTESIAN_POINT('Ctrl Pts',(2.44254768923105,-1.,-3.05045678021504));
#54421=CARTESIAN_POINT('Ctrl Pts',(2.43965194061857,-1.,-3.04359685040555));
#54422=CARTESIAN_POINT('Ctrl Pts',(2.43671278042414,-1.,-3.03676949672822));
#54423=CARTESIAN_POINT('Ctrl Pts',(2.43371241361488,-1.,-3.02995534946978));
#54424=CARTESIAN_POINT('Ctrl Pts',(2.43063415586637,-1.,-3.02313656036004));
#54425=CARTESIAN_POINT('Ctrl Pts',(2.42746856264168,-1.,-3.01630420830504));
#54426=CARTESIAN_POINT('Ctrl Pts',(2.42421849439613,-1.,-3.00946442616659));
#54427=CARTESIAN_POINT('Ctrl Pts',(2.42090763946779,-1.,-3.00264868585996));
#54428=CARTESIAN_POINT('Ctrl Pts',(2.41757324500514,-1.,-2.99590509293503));
#54429=CARTESIAN_POINT('Ctrl Pts',(2.41425064199586,-1.,-2.98927983005796));
#54430=CARTESIAN_POINT('Ctrl Pts',(2.41095909342571,-1.,-2.98280015815107));
#54431=CARTESIAN_POINT('Ctrl Pts',(2.40768975073713,-1.,-2.97646002822422));
#54432=CARTESIAN_POINT('Ctrl Pts',(2.40438604734919,-1.,-2.9701964131236));
#54433=CARTESIAN_POINT('Ctrl Pts',(2.4009556571164,-1.,-2.96390432240312));
#54434=CARTESIAN_POINT('Ctrl Pts',(2.39730553974516,-1.,-2.95748006482942));
#54435=CARTESIAN_POINT('Ctrl Pts',(2.39337207631667,-1.,-2.95085857128439));
#54436=CARTESIAN_POINT('Ctrl Pts',(2.38914929090759,-1.,-2.94404820669076));
#54437=CARTESIAN_POINT('Ctrl Pts',(2.38472771516311,-1.,-2.93717903280391));
#54438=CARTESIAN_POINT('Ctrl Pts',(2.38028989582073,-1.,-2.93049643640206));
#54439=CARTESIAN_POINT('Ctrl Pts',(2.3760651052403,-1.,-2.92430340582608));
#54440=CARTESIAN_POINT('Ctrl Pts',(2.37229381109821,-1.,-2.91891503791411));
#54441=CARTESIAN_POINT('Ctrl Pts',(2.36919161373173,-1.,-2.9146124988314));
#54442=CARTESIAN_POINT('Ctrl Pts',(2.36707658451664,-1.,-2.91181344022549));
#54443=CARTESIAN_POINT('Ctrl Pts',(2.36599991765749,-1.,-2.91051690822156));
#54444=CARTESIAN_POINT('Ctrl Pts',(2.36553202948613,-1.,-2.91005770527719));
#54445=CARTESIAN_POINT('Ctrl Pts',(2.36536211188453,-1.,-2.90995756655606));
#54446=CARTESIAN_POINT('Ctrl Pts',(2.36531447826073,-1.,-2.90994629141676));
#54447=CARTESIAN_POINT('',(2.50410331873042,-1.,-2.79140942341378));
#54448=CARTESIAN_POINT('Origin',(0.,-1.,0.));
#54449=CARTESIAN_POINT('',(2.91557726271063,-1.,-3.02314558451372));
#54450=CARTESIAN_POINT('Ctrl Pts',(2.50410331873042,-1.,-2.79140942341378));
#54451=CARTESIAN_POINT('Ctrl Pts',(2.50410700351426,-1.,-2.79145823440899));
#54452=CARTESIAN_POINT('Ctrl Pts',(2.50417932839343,-1.,-2.79164172519039));
#54453=CARTESIAN_POINT('Ctrl Pts',(2.50455968395235,-1.,-2.79217568804874));
#54454=CARTESIAN_POINT('Ctrl Pts',(2.50567182569153,-1.,-2.79344192164204));
#54455=CARTESIAN_POINT('Ctrl Pts',(2.50810555977564,-1.,-2.7959687805717));
#54456=CARTESIAN_POINT('Ctrl Pts',(2.51186983687947,-1.,-2.79970585014308));
#54457=CARTESIAN_POINT('Ctrl Pts',(2.51660190466067,-1.,-2.80427363984939));
#54458=CARTESIAN_POINT('Ctrl Pts',(2.52205778589922,-1.,-2.80941521967234));
#54459=CARTESIAN_POINT('Ctrl Pts',(2.52796388055457,-1.,-2.8148437904867));
#54460=CARTESIAN_POINT('Ctrl Pts',(2.53405679667463,-1.,-2.82028550483744));
#54461=CARTESIAN_POINT('Ctrl Pts',(2.54012272520141,-1.,-2.82552167649157));
#54462=CARTESIAN_POINT('Ctrl Pts',(2.54604736792542,-1.,-2.83044254225794));
#54463=CARTESIAN_POINT('Ctrl Pts',(2.55182152806964,-1.,-2.83505269592412));
#54464=CARTESIAN_POINT('Ctrl Pts',(2.55749952145165,-1.,-2.83942515220699));
#54465=CARTESIAN_POINT('Ctrl Pts',(2.56316920798489,-1.,-2.84366802680211));
#54466=CARTESIAN_POINT('Ctrl Pts',(2.56891984251743,-1.,-2.84788893329091));
#54467=CARTESIAN_POINT('Ctrl Pts',(2.57480482727128,-1.,-2.85215360144483));
#54468=CARTESIAN_POINT('Ctrl Pts',(2.58082875254407,-1.,-2.85647171715147));
#54469=CARTESIAN_POINT('Ctrl Pts',(2.5869677064356,-1.,-2.86081999003668));
#54470=CARTESIAN_POINT('Ctrl Pts',(2.59318160184921,-1.,-2.86515629953528));
#54471=CARTESIAN_POINT('Ctrl Pts',(2.59942875223202,-1.,-2.86943633170712));
#54472=CARTESIAN_POINT('Ctrl Pts',(2.6056817788128,-1.,-2.87363176656475));
#54473=CARTESIAN_POINT('Ctrl Pts',(2.61193507170928,-1.,-2.87773881947885));
#54474=CARTESIAN_POINT('Ctrl Pts',(2.61819596473087,-1.,-2.88176821427502));
#54475=CARTESIAN_POINT('Ctrl Pts',(2.62447947640253,-1.,-2.88573922195049));
#54476=CARTESIAN_POINT('Ctrl Pts',(2.63080195420771,-1.,-2.88967244854243));
#54477=CARTESIAN_POINT('Ctrl Pts',(2.63717442263944,-1.,-2.89358228854557));
#54478=CARTESIAN_POINT('Ctrl Pts',(2.64359851684146,-1.,-2.89747231723361));
#54479=CARTESIAN_POINT('Ctrl Pts',(2.65007017365576,-1.,-2.90133950224879));
#54480=CARTESIAN_POINT('Ctrl Pts',(2.65658188464287,-1.,-2.90517678087467));
#54481=CARTESIAN_POINT('Ctrl Pts',(2.66312542616808,-1.,-2.90897617968921));
#54482=CARTESIAN_POINT('Ctrl Pts',(2.66969458792627,-1.,-2.91273193382876));
#54483=CARTESIAN_POINT('Ctrl Pts',(2.67628728855309,-1.,-2.91644290704281));
#54484=CARTESIAN_POINT('Ctrl Pts',(2.68290409279689,-1.,-2.92011090722152));
#54485=CARTESIAN_POINT('Ctrl Pts',(2.68954721165342,-1.,-2.92373955325876));
#54486=CARTESIAN_POINT('Ctrl Pts',(2.69621932864302,-1.,-2.92733294395268));
#54487=CARTESIAN_POINT('Ctrl Pts',(2.70292247416881,-1.,-2.93089438233746));
#54488=CARTESIAN_POINT('Ctrl Pts',(2.70965695523776,-1.,-2.93442516311168));
#54489=CARTESIAN_POINT('Ctrl Pts',(2.71642190053575,-1.,-2.93792519474955));
#54490=CARTESIAN_POINT('Ctrl Pts',(2.72321571511322,-1.,-2.94139351933882));
#54491=CARTESIAN_POINT('Ctrl Pts',(2.73003657371613,-1.,-2.94482887675139));
#54492=CARTESIAN_POINT('Ctrl Pts',(2.73688288329825,-1.,-2.94823023414381));
#54493=CARTESIAN_POINT('Ctrl Pts',(2.7437537949221,-1.,-2.95159737214305));
#54494=CARTESIAN_POINT('Ctrl Pts',(2.75064903318996,-1.,-2.95493069316211));
#54495=CARTESIAN_POINT('Ctrl Pts',(2.75756867888393,-1.,-2.9582309766594));
#54496=CARTESIAN_POINT('Ctrl Pts',(2.76451296269571,-1.,-2.96149914764832));
#54497=CARTESIAN_POINT('Ctrl Pts',(2.77148206836464,-1.,-2.96473605585548));
#54498=CARTESIAN_POINT('Ctrl Pts',(2.77847589542767,-1.,-2.9679422104295));
#54499=CARTESIAN_POINT('Ctrl Pts',(2.78549409123657,-1.,-2.97111781461349));
#54500=CARTESIAN_POINT('Ctrl Pts',(2.79253615718147,-1.,-2.97426288347475));
#54501=CARTESIAN_POINT('Ctrl Pts',(2.79960153278186,-1.,-2.97737733718242));
#54502=CARTESIAN_POINT('Ctrl Pts',(2.80668968101162,-1.,-2.98046109647299));
#54503=CARTESIAN_POINT('Ctrl Pts',(2.81380019196454,-1.,-2.9835141977994));
#54504=CARTESIAN_POINT('Ctrl Pts',(2.82093279065704,-1.,-2.98653680669434));
#54505=CARTESIAN_POINT('Ctrl Pts',(2.82808728190402,-1.,-2.98952916401699));
#54506=CARTESIAN_POINT('Ctrl Pts',(2.83526351254383,-1.,-2.99249155170479));
#54507=CARTESIAN_POINT('Ctrl Pts',(2.84246132984334,-1.,-2.995424253416));
#54508=CARTESIAN_POINT('Ctrl Pts',(2.84968053289104,-1.,-2.99832751144566));
#54509=CARTESIAN_POINT('Ctrl Pts',(2.85692085715129,-1.,-3.0012015079552));
#54510=CARTESIAN_POINT('Ctrl Pts',(2.86418200833065,-1.,-3.00404638316245));
#54511=CARTESIAN_POINT('Ctrl Pts',(2.87146368430104,-1.,-3.00686224485374));
#54512=CARTESIAN_POINT('Ctrl Pts',(2.87876560072799,-1.,-3.0096491810855));
#54513=CARTESIAN_POINT('Ctrl Pts',(2.88608751706796,-1.,-3.01240727309568));
#54514=CARTESIAN_POINT('Ctrl Pts',(2.8934292556764,-1.,-3.01513660433291));
#54515=CARTESIAN_POINT('Ctrl Pts',(2.90079069102661,-1.,-3.01783725123646));
#54516=CARTESIAN_POINT('Ctrl Pts',(2.90669553303902,-1.,-3.01997487194926));
#54517=CARTESIAN_POINT('Ctrl Pts',(2.91113297349052,-1.,-3.02156522743299));
#54518=CARTESIAN_POINT('Ctrl Pts',(2.91409518070707,-1.,-3.02261975104912));
#54519=CARTESIAN_POINT('Ctrl Pts',(2.91557726271063,-1.,-3.02314558451372));
#54520=CARTESIAN_POINT('',(3.02314558451372,-1.,-2.91557726271063));
#54521=CARTESIAN_POINT('',(2.91557726271063,-1.,-3.02314558451372));
#54522=CARTESIAN_POINT('',(2.79140942341258,-1.,-2.50410331873176));
#54523=CARTESIAN_POINT('Ctrl Pts',(3.02314558451372,-1.,-2.91557726271063));
#54524=CARTESIAN_POINT('Ctrl Pts',(3.02261975104593,-1.,-2.91409518070399));
#54525=CARTESIAN_POINT('Ctrl Pts',(3.02156522742431,-1.,-2.91113297348212));
#54526=CARTESIAN_POINT('Ctrl Pts',(3.01997487193503,-1.,-2.90669553302526));
#54527=CARTESIAN_POINT('Ctrl Pts',(3.01783725121981,-1.,-2.9007906910105));
#54528=CARTESIAN_POINT('Ctrl Pts',(3.01513660431928,-1.,-2.89342925566321));
#54529=CARTESIAN_POINT('Ctrl Pts',(3.01240727308829,-1.,-2.8860875170608));
#54530=CARTESIAN_POINT('Ctrl Pts',(3.00964918108476,-1.,-2.87876560072727));
#54531=CARTESIAN_POINT('Ctrl Pts',(3.00686224485784,-1.,-2.87146368430502));
#54532=CARTESIAN_POINT('Ctrl Pts',(3.00404638316867,-1.,-2.86418200833667));
#54533=CARTESIAN_POINT('Ctrl Pts',(3.00120150796095,-1.,-2.85692085715686));
#54534=CARTESIAN_POINT('Ctrl Pts',(2.99832751144925,-1.,-2.84968053289451));
#54535=CARTESIAN_POINT('Ctrl Pts',(2.99542425341685,-1.,-2.84246132984415));
#54536=CARTESIAN_POINT('Ctrl Pts',(2.99249155170339,-1.,-2.83526351254248));
#54537=CARTESIAN_POINT('Ctrl Pts',(2.98952916401446,-1.,-2.82808728190157));
#54538=CARTESIAN_POINT('Ctrl Pts',(2.9865368066918,-1.,-2.82093279065457));
#54539=CARTESIAN_POINT('Ctrl Pts',(2.98351419779767,-1.,-2.81380019196286));
#54540=CARTESIAN_POINT('Ctrl Pts',(2.98046109647241,-1.,-2.80668968101106));
#54541=CARTESIAN_POINT('Ctrl Pts',(2.97737733718287,-1.,-2.7996015327823));
#54542=CARTESIAN_POINT('Ctrl Pts',(2.9742628834758,-1.,-2.79253615718248));
#54543=CARTESIAN_POINT('Ctrl Pts',(2.97111781461465,-1.,-2.78549409123769));
#54544=CARTESIAN_POINT('Ctrl Pts',(2.96794221043036,-1.,-2.7784758954285));
#54545=CARTESIAN_POINT('Ctrl Pts',(2.96473605585583,-1.,-2.77148206836498));
#54546=CARTESIAN_POINT('Ctrl Pts',(2.96149914764818,-1.,-2.76451296269557));
#54547=CARTESIAN_POINT('Ctrl Pts',(2.95823097665896,-1.,-2.7575686788835));
#54548=CARTESIAN_POINT('Ctrl Pts',(2.95493069316161,-1.,-2.75064903318947));
#54549=CARTESIAN_POINT('Ctrl Pts',(2.95159737214266,-1.,-2.74375379492172));
#54550=CARTESIAN_POINT('Ctrl Pts',(2.94823023414364,-1.,-2.73688288329808));
#54551=CARTESIAN_POINT('Ctrl Pts',(2.94482887675143,-1.,-2.73003657371617));
#54552=CARTESIAN_POINT('Ctrl Pts',(2.94139351933897,-1.,-2.72321571511337));
#54553=CARTESIAN_POINT('Ctrl Pts',(2.93792519474972,-1.,-2.71642190053592));
#54554=CARTESIAN_POINT('Ctrl Pts',(2.93442516311179,-1.,-2.70965695523787));
#54555=CARTESIAN_POINT('Ctrl Pts',(2.93089438233749,-1.,-2.70292247416885));
#54556=CARTESIAN_POINT('Ctrl Pts',(2.92733294395267,-1.,-2.69621932864301));
#54557=CARTESIAN_POINT('Ctrl Pts',(2.92373955325875,-1.,-2.68954721165339));
#54558=CARTESIAN_POINT('Ctrl Pts',(2.92011090722152,-1.,-2.68290409279688));
#54559=CARTESIAN_POINT('Ctrl Pts',(2.91644290704285,-1.,-2.67628728855312));
#54560=CARTESIAN_POINT('Ctrl Pts',(2.91273193382882,-1.,-2.66969458792631));
#54561=CARTESIAN_POINT('Ctrl Pts',(2.90897617968923,-1.,-2.6631254261681));
#54562=CARTESIAN_POINT('Ctrl Pts',(2.90517678087461,-1.,-2.65658188464282));
#54563=CARTESIAN_POINT('Ctrl Pts',(2.90133950224867,-1.,-2.65007017365564));
#54564=CARTESIAN_POINT('Ctrl Pts',(2.89747231723345,-1.,-2.64359851684131));
#54565=CARTESIAN_POINT('Ctrl Pts',(2.89358228854544,-1.,-2.63717442263932));
#54566=CARTESIAN_POINT('Ctrl Pts',(2.88967244854239,-1.,-2.63080195420767));
#54567=CARTESIAN_POINT('Ctrl Pts',(2.88573922195059,-1.,-2.62447947640262));
#54568=CARTESIAN_POINT('Ctrl Pts',(2.88176821427525,-1.,-2.61819596473108));
#54569=CARTESIAN_POINT('Ctrl Pts',(2.87773881947915,-1.,-2.61193507170955));
#54570=CARTESIAN_POINT('Ctrl Pts',(2.87363176656501,-1.,-2.60568177881303));
#54571=CARTESIAN_POINT('Ctrl Pts',(2.86943633170722,-1.,-2.5994287522321));
#54572=CARTESIAN_POINT('Ctrl Pts',(2.86515629953513,-1.,-2.59318160184908));
#54573=CARTESIAN_POINT('Ctrl Pts',(2.86081999003629,-1.,-2.58696770643524));
#54574=CARTESIAN_POINT('Ctrl Pts',(2.85647171715092,-1.,-2.58082875254357));
#54575=CARTESIAN_POINT('Ctrl Pts',(2.85215360144431,-1.,-2.57480482727081));
#54576=CARTESIAN_POINT('Ctrl Pts',(2.84788893329067,-1.,-2.56891984251721));
#54577=CARTESIAN_POINT('Ctrl Pts',(2.84366802680237,-1.,-2.56316920798513));
#54578=CARTESIAN_POINT('Ctrl Pts',(2.83942515220782,-1.,-2.55749952145241));
#54579=CARTESIAN_POINT('Ctrl Pts',(2.83505269592536,-1.,-2.55182152807077));
#54580=CARTESIAN_POINT('Ctrl Pts',(2.83044254225917,-1.,-2.54604736792655));
#54581=CARTESIAN_POINT('Ctrl Pts',(2.8255216764922,-1.,-2.54012272520199));
#54582=CARTESIAN_POINT('Ctrl Pts',(2.82028550483689,-1.,-2.53405679667412));
#54583=CARTESIAN_POINT('Ctrl Pts',(2.81484379048475,-1.,-2.52796388055278));
#54584=CARTESIAN_POINT('Ctrl Pts',(2.80941521966941,-1.,-2.52205778589653));
#54585=CARTESIAN_POINT('Ctrl Pts',(2.80427363984653,-1.,-2.51660190465805));
#54586=CARTESIAN_POINT('Ctrl Pts',(2.79970585014168,-1.,-2.51186983687818));
#54587=CARTESIAN_POINT('Ctrl Pts',(2.79596878057287,-1.,-2.50810555977671));
#54588=CARTESIAN_POINT('Ctrl Pts',(2.79344192164147,-1.,-2.50567182569081));
#54589=CARTESIAN_POINT('Ctrl Pts',(2.79217568804755,-1.,-2.50455968395146));
#54590=CARTESIAN_POINT('Ctrl Pts',(2.79164172518905,-1.,-2.50417932839313));
#54591=CARTESIAN_POINT('Ctrl Pts',(2.79145823440781,-1.,-2.50410700351493));
#54592=CARTESIAN_POINT('Ctrl Pts',(2.79140942341258,-1.,-2.50410331873176));
#54593=CARTESIAN_POINT('',(2.90994629141562,-1.,-2.36531447826213));
#54594=CARTESIAN_POINT('Origin',(0.,-1.,0.));
#54595=CARTESIAN_POINT('',(3.35260583073571,-1.,-2.52982887637028));
#54596=CARTESIAN_POINT('Ctrl Pts',(2.90994629141562,-1.,-2.36531447826213));
#54597=CARTESIAN_POINT('Ctrl Pts',(2.90995756655558,-1.,-2.3653621118858));
#54598=CARTESIAN_POINT('Ctrl Pts',(2.9100577052777,-1.,-2.36553202948741));
#54599=CARTESIAN_POINT('Ctrl Pts',(2.91051690822262,-1.,-2.36599991765853));
#54600=CARTESIAN_POINT('Ctrl Pts',(2.91181344022628,-1.,-2.36707658451709));
#54601=CARTESIAN_POINT('Ctrl Pts',(2.91461249883016,-1.,-2.36919161373074));
#54602=CARTESIAN_POINT('Ctrl Pts',(2.9189150379156,-1.,-2.37229381109939));
#54603=CARTESIAN_POINT('Ctrl Pts',(2.92430340582912,-1.,-2.37606510524271));
#54604=CARTESIAN_POINT('Ctrl Pts',(2.93049643640517,-1.,-2.3802898958232));
#54605=CARTESIAN_POINT('Ctrl Pts',(2.93717903280599,-1.,-2.38472771516476));
#54606=CARTESIAN_POINT('Ctrl Pts',(2.94404820669135,-1.,-2.38914929090806));
#54607=CARTESIAN_POINT('Ctrl Pts',(2.95085857128372,-1.,-2.39337207631613));
#54608=CARTESIAN_POINT('Ctrl Pts',(2.95748006482811,-1.,-2.39730553974412));
#54609=CARTESIAN_POINT('Ctrl Pts',(2.9639043224018,-1.,-2.40095565711535));
#54610=CARTESIAN_POINT('Ctrl Pts',(2.97019641312272,-1.,-2.40438604734848));
#54611=CARTESIAN_POINT('Ctrl Pts',(2.97646002822395,-1.,-2.40768975073691));
#54612=CARTESIAN_POINT('Ctrl Pts',(2.98280015815132,-1.,-2.41095909342591));
#54613=CARTESIAN_POINT('Ctrl Pts',(2.98927983005851,-1.,-2.4142506419963));
#54614=CARTESIAN_POINT('Ctrl Pts',(2.99590509293561,-1.,-2.4175732450056));
#54615=CARTESIAN_POINT('Ctrl Pts',(3.00264868586038,-1.,-2.42090763946812));
#54616=CARTESIAN_POINT('Ctrl Pts',(3.00946442616674,-1.,-2.42421849439625));
#54617=CARTESIAN_POINT('Ctrl Pts',(3.01630420830493,-1.,-2.4274685626416));
#54618=CARTESIAN_POINT('Ctrl Pts',(3.02313656035977,-1.,-2.43063415586615));
#54619=CARTESIAN_POINT('Ctrl Pts',(3.02995534946946,-1.,-2.43371241361462));
#54620=CARTESIAN_POINT('Ctrl Pts',(3.03676949672797,-1.,-2.43671278042394));
#54621=CARTESIAN_POINT('Ctrl Pts',(3.04359685040545,-1.,-2.43965194061849));
#54622=CARTESIAN_POINT('Ctrl Pts',(3.05045678021509,-1.,-2.44254768923109));
#54623=CARTESIAN_POINT('Ctrl Pts',(3.05736242671521,-1.,-2.44541251892568));
#54624=CARTESIAN_POINT('Ctrl Pts',(3.06431596421422,-1.,-2.44824970516558));
#54625=CARTESIAN_POINT('Ctrl Pts',(3.0713129052131,-1.,-2.45105688854432));
#54626=CARTESIAN_POINT('Ctrl Pts',(3.07834472886145,-1.,-2.45382826787795));
#54627=CARTESIAN_POINT('Ctrl Pts',(3.08540206545313,-1.,-2.45655725437037));
#54628=CARTESIAN_POINT('Ctrl Pts',(3.09247787931881,-1.,-2.45923912563875));
#54629=CARTESIAN_POINT('Ctrl Pts',(3.09956993697048,-1.,-2.4618730850188));
#54630=CARTESIAN_POINT('Ctrl Pts',(3.10667907901981,-1.,-2.46446082979645));
#54631=CARTESIAN_POINT('Ctrl Pts',(3.11380805536124,-1.,-2.46700558843507));
#54632=CARTESIAN_POINT('Ctrl Pts',(3.12096015766984,-1.,-2.4695109894747));
#54633=CARTESIAN_POINT('Ctrl Pts',(3.12813790805948,-1.,-2.47197997765868));
#54634=CARTESIAN_POINT('Ctrl Pts',(3.13534181229282,-1.,-2.47441378371923));
#54635=CARTESIAN_POINT('Ctrl Pts',(3.14257099546531,-1.,-2.47681245356095));
#54636=CARTESIAN_POINT('Ctrl Pts',(3.14982373241335,-1.,-2.47917529057016));
#54637=CARTESIAN_POINT('Ctrl Pts',(3.15709802322735,-1.,-2.48150133566568));
#54638=CARTESIAN_POINT('Ctrl Pts',(3.16439213290181,-1.,-2.48378981792739));
#54639=CARTESIAN_POINT('Ctrl Pts',(3.17170518863357,-1.,-2.48604065348619));
#54640=CARTESIAN_POINT('Ctrl Pts',(3.17903698136678,-1.,-2.48825428288243));
#54641=CARTESIAN_POINT('Ctrl Pts',(3.18638771282315,-1.,-2.49043146334095));
#54642=CARTESIAN_POINT('Ctrl Pts',(3.19375775555814,-1.,-2.4925730723986));
#54643=CARTESIAN_POINT('Ctrl Pts',(3.20114742397549,-1.,-2.49467992057726));
#54644=CARTESIAN_POINT('Ctrl Pts',(3.2085566984974,-1.,-2.49675252647298));
#54645=CARTESIAN_POINT('Ctrl Pts',(3.21598526261157,-1.,-2.49879114599293));
#54646=CARTESIAN_POINT('Ctrl Pts',(3.22343262620387,-1.,-2.5007958720187));
#54647=CARTESIAN_POINT('Ctrl Pts',(3.23089822320596,-1.,-2.50276671338074));
#54648=CARTESIAN_POINT('Ctrl Pts',(3.23838151080383,-1.,-2.50470367580078));
#54649=CARTESIAN_POINT('Ctrl Pts',(3.24588208984042,-1.,-2.50660685940645));
#54650=CARTESIAN_POINT('Ctrl Pts',(3.25339971461265,-1.,-2.50847647070936));
#54651=CARTESIAN_POINT('Ctrl Pts',(3.26093423001716,-1.,-2.51031277813697));
#54652=CARTESIAN_POINT('Ctrl Pts',(3.26848552888271,-1.,-2.51211608411539));
#54653=CARTESIAN_POINT('Ctrl Pts',(3.27605350473048,-1.,-2.51388669270329));
#54654=CARTESIAN_POINT('Ctrl Pts',(3.28363799702583,-1.,-2.51562487464215));
#54655=CARTESIAN_POINT('Ctrl Pts',(3.2912387729863,-1.,-2.51733085123316));
#54656=CARTESIAN_POINT('Ctrl Pts',(3.29885556387661,-1.,-2.51900480700548));
#54657=CARTESIAN_POINT('Ctrl Pts',(3.30648808814986,-1.,-2.52064689568167));
#54658=CARTESIAN_POINT('Ctrl Pts',(3.31413607874727,-1.,-2.52225724871375));
#54659=CARTESIAN_POINT('Ctrl Pts',(3.32179931079521,-1.,-2.52383598396878));
#54660=CARTESIAN_POINT('Ctrl Pts',(3.32947762189049,-1.,-2.52538321165774));
#54661=CARTESIAN_POINT('Ctrl Pts',(3.33717090000955,-1.,-2.52689902691551));
#54662=CARTESIAN_POINT('Ctrl Pts',(3.34333744117093,-1.,-2.52808660916879));
#54663=CARTESIAN_POINT('Ctrl Pts',(3.34796903577628,-1.,-2.5289632161143));
#54664=CARTESIAN_POINT('Ctrl Pts',(3.35105973714426,-1.,-2.52954136549357));
#54665=CARTESIAN_POINT('Ctrl Pts',(3.35260583073571,-1.,-2.52982887637028));
#54666=CARTESIAN_POINT('',(3.44202241512147,-1.,-2.40675750623143));
#54667=CARTESIAN_POINT('',(3.35260583073571,-1.,-2.52982887637028));
#54668=CARTESIAN_POINT('',(3.14877060440327,-1.,-2.03660101169714));
#54669=CARTESIAN_POINT('Ctrl Pts',(3.44202241512147,-1.,-2.40675750623143));
#54670=CARTESIAN_POINT('Ctrl Pts',(3.44127120683039,-1.,-2.4053759295909));
#54671=CARTESIAN_POINT('Ctrl Pts',(3.43976627484234,-1.,-2.40261515589405));
#54672=CARTESIAN_POINT('Ctrl Pts',(3.43750133064416,-1.,-2.39848113410292));
#54673=CARTESIAN_POINT('Ctrl Pts',(3.4344663067854,-1.,-2.39298338804493));
#54674=CARTESIAN_POINT('Ctrl Pts',(3.43064732712919,-1.,-2.38613505843552));
#54675=CARTESIAN_POINT('Ctrl Pts',(3.42680309754399,-1.,-2.37931067028926));
#54676=CARTESIAN_POINT('Ctrl Pts',(3.42293356216511,-1.,-2.37251035954292));
#54677=CARTESIAN_POINT('Ctrl Pts',(3.41903866635852,-1.,-2.36573431470642));
#54678=CARTESIAN_POINT('Ctrl Pts',(3.41511836751469,-1.,-2.35898278606946));
#54679=CARTESIAN_POINT('Ctrl Pts',(3.41117262314119,-1.,-2.35225606824109));
#54680=CARTESIAN_POINT('Ctrl Pts',(3.40720137404297,-1.,-2.34555447649188));
#54681=CARTESIAN_POINT('Ctrl Pts',(3.40320452776743,-1.,-2.33887832342782));
#54682=CARTESIAN_POINT('Ctrl Pts',(3.39918194577956,-1.,-2.33222789882489));
#54683=CARTESIAN_POINT('Ctrl Pts',(3.39513342019756,-1.,-2.3256034390248));
#54684=CARTESIAN_POINT('Ctrl Pts',(3.39105869474822,-1.,-2.31900513925424));
#54685=CARTESIAN_POINT('Ctrl Pts',(3.38695751492462,-1.,-2.31243319489367));
#54686=CARTESIAN_POINT('Ctrl Pts',(3.3828296733661,-1.,-2.30588783640343));
#54687=CARTESIAN_POINT('Ctrl Pts',(3.37867504959433,-1.,-2.29936936127624));
#54688=CARTESIAN_POINT('Ctrl Pts',(3.37449367172826,-1.,-2.29287818007393));
#54689=CARTESIAN_POINT('Ctrl Pts',(3.37028570206488,-1.,-2.28641481081137));
#54690=CARTESIAN_POINT('Ctrl Pts',(3.36605130713076,-1.,-2.27997979458037));
#54691=CARTESIAN_POINT('Ctrl Pts',(3.36179055004409,-1.,-2.2735736262093));
#54692=CARTESIAN_POINT('Ctrl Pts',(3.35750328523061,-1.,-2.2671966857991));
#54693=CARTESIAN_POINT('Ctrl Pts',(3.35318902552626,-1.,-2.26084915222449));
#54694=CARTESIAN_POINT('Ctrl Pts',(3.34884690292285,-1.,-2.25453097693483));
#54695=CARTESIAN_POINT('Ctrl Pts',(3.34447596770723,-1.,-2.24824207678256));
#54696=CARTESIAN_POINT('Ctrl Pts',(3.34007543738025,-1.,-2.24198249391422));
#54697=CARTESIAN_POINT('Ctrl Pts',(3.33564495756481,-1.,-2.23575256328812));
#54698=CARTESIAN_POINT('Ctrl Pts',(3.33118487773611,-1.,-2.22955308907233));
#54699=CARTESIAN_POINT('Ctrl Pts',(3.3266964672289,-1.,-2.22338548312772));
#54700=CARTESIAN_POINT('Ctrl Pts',(3.32218125618968,-1.,-2.21725135110898));
#54701=CARTESIAN_POINT('Ctrl Pts',(3.31764044024235,-1.,-2.21115211847875));
#54702=CARTESIAN_POINT('Ctrl Pts',(3.31307424608949,-1.,-2.20508863150607));
#54703=CARTESIAN_POINT('Ctrl Pts',(3.30848134694595,-1.,-2.19906078949923));
#54704=CARTESIAN_POINT('Ctrl Pts',(3.30385816281831,-1.,-2.19306710376111));
#54705=CARTESIAN_POINT('Ctrl Pts',(3.29920022557639,-1.,-2.18710556500327));
#54706=CARTESIAN_POINT('Ctrl Pts',(3.2945036150049,-1.,-2.18117455557065));
#54707=CARTESIAN_POINT('Ctrl Pts',(3.28976645712568,-1.,-2.17527380048423));
#54708=CARTESIAN_POINT('Ctrl Pts',(3.28499019979724,-1.,-2.16940517773455));
#54709=CARTESIAN_POINT('Ctrl Pts',(3.280181508414,-1.,-2.16357391934425));
#54710=CARTESIAN_POINT('Ctrl Pts',(3.27534954469187,-1.,-2.15778690038347));
#54711=CARTESIAN_POINT('Ctrl Pts',(3.27050245897228,-1.,-2.15205043199808));
#54712=CARTESIAN_POINT('Ctrl Pts',(3.26564388189759,-1.,-2.1463680529566));
#54713=CARTESIAN_POINT('Ctrl Pts',(3.26077002641879,-1.,-2.14073870754264));
#54714=CARTESIAN_POINT('Ctrl Pts',(3.25586495065054,-1.,-2.13515375878803));
#54715=CARTESIAN_POINT('Ctrl Pts',(3.25090574494028,-1.,-2.12960028396832));
#54716=CARTESIAN_POINT('Ctrl Pts',(3.24587102613376,-1.,-2.12406646410962));
#54717=CARTESIAN_POINT('Ctrl Pts',(3.24074905517293,-1.,-2.11854673326979));
#54718=CARTESIAN_POINT('Ctrl Pts',(3.23554444767099,-1.,-2.11304604021773));
#54719=CARTESIAN_POINT('Ctrl Pts',(3.23028945793289,-1.,-2.10758699642451));
#54720=CARTESIAN_POINT('Ctrl Pts',(3.22503437553434,-1.,-2.10220384298492));
#54721=CARTESIAN_POINT('Ctrl Pts',(3.21982707347009,-1.,-2.09692958434895));
#54722=CARTESIAN_POINT('Ctrl Pts',(3.21469429601654,-1.,-2.09178419460443));
#54723=CARTESIAN_POINT('Ctrl Pts',(3.20962575845463,-1.,-2.08676465517455));
#54724=CARTESIAN_POINT('Ctrl Pts',(3.2045481863073,-1.,-2.08182850370878));
#54725=CARTESIAN_POINT('Ctrl Pts',(3.19934132836019,-1.,-2.07690441870722));
#54726=CARTESIAN_POINT('Ctrl Pts',(3.19388465568252,-1.,-2.07192253497857));
#54727=CARTESIAN_POINT('Ctrl Pts',(3.18809755562368,-1.,-2.06684062744112));
#54728=CARTESIAN_POINT('Ctrl Pts',(3.18197692964614,-1.,-2.06166849827101));
#54729=CARTESIAN_POINT('Ctrl Pts',(3.17564906975371,-1.,-2.05650186773132));
#54730=CARTESIAN_POINT('Ctrl Pts',(3.16936341689527,-1.,-2.05151770247233));
#54731=CARTESIAN_POINT('Ctrl Pts',(3.16343165058912,-1.,-2.04693331247446));
#54732=CARTESIAN_POINT('Ctrl Pts',(3.15817983946367,-1.,-2.04297406404027));
#54733=CARTESIAN_POINT('Ctrl Pts',(3.15389991674792,-1.,-2.03984073791519));
#54734=CARTESIAN_POINT('Ctrl Pts',(3.15102344775328,-1.,-2.03783225495961));
#54735=CARTESIAN_POINT('Ctrl Pts',(3.14959882629805,-1.,-2.03693188810545));
#54736=CARTESIAN_POINT('Ctrl Pts',(3.1490119366901,-1.,-2.03663974554932));
#54737=CARTESIAN_POINT('Ctrl Pts',(3.14881939088124,-1.,-2.03659701539259));
#54738=CARTESIAN_POINT('Ctrl Pts',(3.14877060440327,-1.,-2.03660101169714));
#54739=CARTESIAN_POINT('',(3.24413672884812,-1.,-1.88097764062697));
#54740=CARTESIAN_POINT('Origin',(0.,-1.,0.));
#54741=CARTESIAN_POINT('',(3.70708211654725,-1.,-1.97421938526992));
#54742=CARTESIAN_POINT('Ctrl Pts',(3.24413672884812,-1.,-1.88097764062697));
#54743=CARTESIAN_POINT('Ctrl Pts',(3.24415531671284,-1.,-1.8810229239812));
#54744=CARTESIAN_POINT('Ctrl Pts',(3.24428080353022,-1.,-1.88117508446775));
#54745=CARTESIAN_POINT('Ctrl Pts',(3.24480754676064,-1.,-1.88156537699203));
#54746=CARTESIAN_POINT('Ctrl Pts',(3.2462565441079,-1.,-1.88242596600454));
#54747=CARTESIAN_POINT('Ctrl Pts',(3.24935200511918,-1.,-1.88407708646357));
#54748=CARTESIAN_POINT('Ctrl Pts',(3.25408686339463,-1.,-1.88646802523466));
#54749=CARTESIAN_POINT('Ctrl Pts',(3.25999885193947,-1.,-1.88934996203698));
#54750=CARTESIAN_POINT('Ctrl Pts',(3.26677653888676,-1.,-1.89255393500965));
#54751=CARTESIAN_POINT('Ctrl Pts',(3.27407108933139,-1.,-1.89589172903793));
#54752=CARTESIAN_POINT('Ctrl Pts',(3.28154737912352,-1.,-1.89918429230462));
#54753=CARTESIAN_POINT('Ctrl Pts',(3.2889344860029,-1.,-1.90228971247527));
#54754=CARTESIAN_POINT('Ctrl Pts',(3.29608978722113,-1.,-1.90513891864087));
#54755=CARTESIAN_POINT('Ctrl Pts',(3.30300595568195,-1.,-1.90773912171341));
#54756=CARTESIAN_POINT('Ctrl Pts',(3.30975721158596,-1.,-1.91014297830446));
#54757=CARTESIAN_POINT('Ctrl Pts',(3.31646052426364,-1.,-1.91242616234442));
#54758=CARTESIAN_POINT('Ctrl Pts',(3.32323403454535,-1.,-1.91466343916628));
#54759=CARTESIAN_POINT('Ctrl Pts',(3.33014884257873,-1.,-1.91690081930332));
#54760=CARTESIAN_POINT('Ctrl Pts',(3.33721230710012,-1.,-1.9191460961021));
#54761=CARTESIAN_POINT('Ctrl Pts',(3.34439448941961,-1.,-1.92138450828404));
#54762=CARTESIAN_POINT('Ctrl Pts',(3.35164424847223,-1.,-1.92358838440528));
#54763=CARTESIAN_POINT('Ctrl Pts',(3.35890824422965,-1.,-1.92572846125756));
#54764=CARTESIAN_POINT('Ctrl Pts',(3.36615168657567,-1.,-1.92778626543786));
#54765=CARTESIAN_POINT('Ctrl Pts',(3.37336807068043,-1.,-1.92975993109877));
#54766=CARTESIAN_POINT('Ctrl Pts',(3.3805676852555,-1.,-1.93165739093276));
#54767=CARTESIAN_POINT('Ctrl Pts',(3.38777076883256,-1.,-1.93349233176788));
#54768=CARTESIAN_POINT('Ctrl Pts',(3.39499923640795,-1.,-1.93527929945985));
#54769=CARTESIAN_POINT('Ctrl Pts',(3.40226802104109,-1.,-1.93702857723098));
#54770=CARTESIAN_POINT('Ctrl Pts',(3.40957978266642,-1.,-1.93874306008143));
#54771=CARTESIAN_POINT('Ctrl Pts',(3.41692971994096,-1.,-1.94042111965246));
#54772=CARTESIAN_POINT('Ctrl Pts',(3.42430850941503,-1.,-1.94205835913696));
#54773=CARTESIAN_POINT('Ctrl Pts',(3.43170586602434,-1.,-1.94364973660284));
#54774=CARTESIAN_POINT('Ctrl Pts',(3.43911410197687,-1.,-1.94519168842879));
#54775=CARTESIAN_POINT('Ctrl Pts',(3.44653088665681,-1.,-1.94668377715329));
#54776=CARTESIAN_POINT('Ctrl Pts',(3.45395731584051,-1.,-1.94812754766524));
#54777=CARTESIAN_POINT('Ctrl Pts',(3.46139661060962,-1.,-1.94952575850197));
#54778=CARTESIAN_POINT('Ctrl Pts',(3.46885258974191,-1.,-1.95088147859877));
#54779=CARTESIAN_POINT('Ctrl Pts',(3.47632820495921,-1.,-1.95219722189876));
#54780=CARTESIAN_POINT('Ctrl Pts',(3.48382414832634,-1.,-1.95347412486309));
#54781=CARTESIAN_POINT('Ctrl Pts',(3.49133956289133,-1.,-1.95471236969643));
#54782=CARTESIAN_POINT('Ctrl Pts',(3.49887263575583,-1.,-1.95591153823661));
#54783=CARTESIAN_POINT('Ctrl Pts',(3.50642124159909,-1.,-1.95707099606511));
#54784=CARTESIAN_POINT('Ctrl Pts',(3.51398354617794,-1.,-1.95819025316779));
#54785=CARTESIAN_POINT('Ctrl Pts',(3.52155867431486,-1.,-1.95926936324461));
#54786=CARTESIAN_POINT('Ctrl Pts',(3.52914648844351,-1.,-1.96030879411566));
#54787=CARTESIAN_POINT('Ctrl Pts',(3.53674730625813,-1.,-1.96130926212689));
#54788=CARTESIAN_POINT('Ctrl Pts',(3.54436163300443,-1.,-1.96227157573067));
#54789=CARTESIAN_POINT('Ctrl Pts',(3.55198990600886,-1.,-1.96319648628644));
#54790=CARTESIAN_POINT('Ctrl Pts',(3.55963218706096,-1.,-1.96408450906812));
#54791=CARTESIAN_POINT('Ctrl Pts',(3.56728820357791,-1.,-1.96493594634567));
#54792=CARTESIAN_POINT('Ctrl Pts',(3.57495748600959,-1.,-1.96575096652789));
#54793=CARTESIAN_POINT('Ctrl Pts',(3.58263947663829,-1.,-1.96652966688911));
#54794=CARTESIAN_POINT('Ctrl Pts',(3.59033364022801,-1.,-1.96727213799544));
#54795=CARTESIAN_POINT('Ctrl Pts',(3.59803959819938,-1.,-1.96797854118369));
#54796=CARTESIAN_POINT('Ctrl Pts',(3.60575714017989,-1.,-1.9686491188594));
#54797=CARTESIAN_POINT('Ctrl Pts',(3.61348615496704,-1.,-1.96928416040877));
#54798=CARTESIAN_POINT('Ctrl Pts',(3.62122658401893,-1.,-1.96988398129978));
#54799=CARTESIAN_POINT('Ctrl Pts',(3.62897836973293,-1.,-1.97044889850463));
#54800=CARTESIAN_POINT('Ctrl Pts',(3.63674139590412,-1.,-1.97097920454464));
#54801=CARTESIAN_POINT('Ctrl Pts',(3.64451546723514,-1.,-1.97147515441164));
#54802=CARTESIAN_POINT('Ctrl Pts',(3.652300347166,-1.,-1.9719369724024));
#54803=CARTESIAN_POINT('Ctrl Pts',(3.6600957816636,-1.,-1.9723648543905));
#54804=CARTESIAN_POINT('Ctrl Pts',(3.66790152752075,-1.,-1.97275897198678));
#54805=CARTESIAN_POINT('Ctrl Pts',(3.67571738107084,-1.,-1.97311947678517));
#54806=CARTESIAN_POINT('Ctrl Pts',(3.68354319915092,-1.,-1.97344650304519));
#54807=CARTESIAN_POINT('Ctrl Pts',(3.69137888599902,-1.,-1.97374016225483));
#54808=CARTESIAN_POINT('Ctrl Pts',(3.6976552856004,-1.,-1.97394846383216));
#54809=CARTESIAN_POINT('Ctrl Pts',(3.70236698912904,-1.,-1.97408973726715));
#54810=CARTESIAN_POINT('Ctrl Pts',(3.70551008132332,-1.,-1.97417727645308));
#54811=CARTESIAN_POINT('Ctrl Pts',(3.70708211654725,-1.,-1.97421938526992));
#54812=CARTESIAN_POINT('',(3.77614523045147,-1.,-1.83867539237861));
#54813=CARTESIAN_POINT('',(3.70708211654725,-1.,-1.97421938526992));
#54814=CARTESIAN_POINT('',(3.42859860294305,-1.,-1.5189508286633));
#54815=CARTESIAN_POINT('Ctrl Pts',(3.77614523045147,-1.,-1.83867539237861));
#54816=CARTESIAN_POINT('Ctrl Pts',(3.77518714457833,-1.,-1.83742834010626));
#54817=CARTESIAN_POINT('Ctrl Pts',(3.77326886064398,-1.,-1.83493697934534));
#54818=CARTESIAN_POINT('Ctrl Pts',(3.77038509817999,-1.,-1.83120816955646));
#54819=CARTESIAN_POINT('Ctrl Pts',(3.76652740353775,-1.,-1.82625289220915));
#54820=CARTESIAN_POINT('Ctrl Pts',(3.76168412707948,-1.,-1.82008629694091));
#54821=CARTESIAN_POINT('Ctrl Pts',(3.75681965683071,-1.,-1.8139472983358));
#54822=CARTESIAN_POINT('Ctrl Pts',(3.75193395887977,-1.,-1.80783603939617));
#54823=CARTESIAN_POINT('Ctrl Pts',(3.74702700875467,-1.,-1.8017527148577));
#54824=CARTESIAN_POINT('Ctrl Pts',(3.74209880352445,-1.,-1.79569757859422));
#54825=CARTESIAN_POINT('Ctrl Pts',(3.73714934730681,-1.,-1.78967092823491));
#54826=CARTESIAN_POINT('Ctrl Pts',(3.7321786309547,-1.,-1.78367308442901));
#54827=CARTESIAN_POINT('Ctrl Pts',(3.72718661205609,-1.,-1.77770437039658));
#54828=CARTESIAN_POINT('Ctrl Pts',(3.72217319911254,-1.,-1.77176509401761));
#54829=CARTESIAN_POINT('Ctrl Pts',(3.71713822377359,-1.,-1.76585552124394));
#54830=CARTESIAN_POINT('Ctrl Pts',(3.71208146346136,-1.,-1.75997588498865));
#54831=CARTESIAN_POINT('Ctrl Pts',(3.70700269736659,-1.,-1.75412641804042));
#54832=CARTESIAN_POINT('Ctrl Pts',(3.7019017567335,-1.,-1.74830738046057));
#54833=CARTESIAN_POINT('Ctrl Pts',(3.69677856910517,-1.,-1.74251908492617));
#54834=CARTESIAN_POINT('Ctrl Pts',(3.69163322648036,-1.,-1.73676193254557));
#54835=CARTESIAN_POINT('Ctrl Pts',(3.68646597019332,-1.,-1.73103640956717));
#54836=CARTESIAN_POINT('Ctrl Pts',(3.68127704936579,-1.,-1.72534302437056));
#54837=CARTESIAN_POINT('Ctrl Pts',(3.67606660374709,-1.,-1.71968225581808));
#54838=CARTESIAN_POINT('Ctrl Pts',(3.67083454901611,-1.,-1.71405450210384));
#54839=CARTESIAN_POINT('Ctrl Pts',(3.66558043198876,-1.,-1.70846001610956));
#54840=CARTESIAN_POINT('Ctrl Pts',(3.66030338774847,-1.,-1.70289888566873));
#54841=CARTESIAN_POINT('Ctrl Pts',(3.65500246526749,-1.,-1.69737117722534));
#54842=CARTESIAN_POINT('Ctrl Pts',(3.64967689827371,-1.,-1.69187705481689));
#54843=CARTESIAN_POINT('Ctrl Pts',(3.64432638915203,-1.,-1.68641690471457));
#54844=CARTESIAN_POINT('Ctrl Pts',(3.63895140887462,-1.,-1.68099146651586));
#54845=CARTESIAN_POINT('Ctrl Pts',(3.63355343201232,-1.,-1.67560193613156));
#54846=CARTESIAN_POINT('Ctrl Pts',(3.62813422105271,-1.,-1.67024966008045));
#54847=CARTESIAN_POINT('Ctrl Pts',(3.62269517989109,-1.,-1.66493585923855));
#54848=CARTESIAN_POINT('Ctrl Pts',(3.61723666482456,-1.,-1.65966133399186));
#54849=CARTESIAN_POINT('Ctrl Pts',(3.61175734965127,-1.,-1.65442619244325));
#54850=CARTESIAN_POINT('Ctrl Pts',(3.60625346556992,-1.,-1.64922952425832));
#54851=CARTESIAN_POINT('Ctrl Pts',(3.60072028513845,-1.,-1.64407004385582));
#54852=CARTESIAN_POINT('Ctrl Pts',(3.59515368334893,-1.,-1.63894676675352));
#54853=CARTESIAN_POINT('Ctrl Pts',(3.58955176627879,-1.,-1.6338597145126));
#54854=CARTESIAN_POINT('Ctrl Pts',(3.58391625774343,-1.,-1.62881051550745));
#54855=CARTESIAN_POINT('Ctrl Pts',(3.5782545595439,-1.,-1.62380329464844));
#54856=CARTESIAN_POINT('Ctrl Pts',(3.57257679609806,-1.,-1.61884340915404));
#54857=CARTESIAN_POINT('Ctrl Pts',(3.56689200468387,-1.,-1.61393581747514));
#54858=CARTESIAN_POINT('Ctrl Pts',(3.5612043248298,-1.,-1.60908344685457));
#54859=CARTESIAN_POINT('Ctrl Pts',(3.55550985096129,-1.,-1.60428584699853));
#54860=CARTESIAN_POINT('Ctrl Pts',(3.54979148634454,-1.,-1.59953698113457));
#54861=CARTESIAN_POINT('Ctrl Pts',(3.54402458182337,-1.,-1.59482766949766));
#54862=CARTESIAN_POINT('Ctrl Pts',(3.53818616861077,-1.,-1.59014958368739));
#54863=CARTESIAN_POINT('Ctrl Pts',(3.5322637814708,-1.,-1.58549906268088));
#54864=CARTESIAN_POINT('Ctrl Pts',(3.52626275334881,-1.,-1.58088027227848));
#54865=CARTESIAN_POINT('Ctrl Pts',(3.52021847865912,-1.,-1.57631049988158));
#54866=CARTESIAN_POINT('Ctrl Pts',(3.51418598431665,-1.,-1.57181569799743));
#54867=CARTESIAN_POINT('Ctrl Pts',(3.50821771695363,-1.,-1.56742097575012));
#54868=CARTESIAN_POINT('Ctrl Pts',(3.50234321621578,-1.,-1.56314187758675));
#54869=CARTESIAN_POINT('Ctrl Pts',(3.49655185179655,-1.,-1.55897703097874));
#54870=CARTESIAN_POINT('Ctrl Pts',(3.4907646087742,-1.,-1.55489595901116));
#54871=CARTESIAN_POINT('Ctrl Pts',(3.48485155928567,-1.,-1.55084702970452));
#54872=CARTESIAN_POINT('Ctrl Pts',(3.47868272898751,-1.,-1.54678009290276));
#54873=CARTESIAN_POINT('Ctrl Pts',(3.47217189224653,-1.,-1.54266605398188));
#54874=CARTESIAN_POINT('Ctrl Pts',(3.46531752207153,-1.,-1.53851507915502));
#54875=CARTESIAN_POINT('Ctrl Pts',(3.45825932955032,-1.,-1.53440195378792));
#54876=CARTESIAN_POINT('Ctrl Pts',(3.45127136828305,-1.,-1.53046244461635));
#54877=CARTESIAN_POINT('Ctrl Pts',(3.44469547526647,-1.,-1.52686242875556));
#54878=CARTESIAN_POINT('Ctrl Pts',(3.4388889597401,-1.,-1.5237734895035));
#54879=CARTESIAN_POINT('Ctrl Pts',(3.43417156977893,-1.,-1.52134826724293));
#54880=CARTESIAN_POINT('Ctrl Pts',(3.43101631893414,-1.,-1.5198144909338));
#54881=CARTESIAN_POINT('Ctrl Pts',(3.42946838852587,-1.,-1.51914806898491));
#54882=CARTESIAN_POINT('Ctrl Pts',(3.42884302333841,-1.,-1.5189513329503));
#54883=CARTESIAN_POINT('Ctrl Pts',(3.42864616361875,-1.,-1.51893924967331));
#54884=CARTESIAN_POINT('Ctrl Pts',(3.42859860294305,-1.,-1.5189508286633));
#54885=CARTESIAN_POINT('',(3.49844575334386,-1.,-1.35032489087269));
#54886=CARTESIAN_POINT('Origin',(0.,-1.,0.));
#54887=CARTESIAN_POINT('',(3.97027773754922,-1.,-1.36999806084572));
#54888=CARTESIAN_POINT('Ctrl Pts',(3.49844575334386,-1.,-1.35032489087269));
#54889=CARTESIAN_POINT('Ctrl Pts',(3.49847119623841,-1.,-1.35036670893102));
#54890=CARTESIAN_POINT('Ctrl Pts',(3.49861894124915,-1.,-1.35049736560633));
#54891=CARTESIAN_POINT('Ctrl Pts',(3.49920025459856,-1.,-1.35080045218652));
#54892=CARTESIAN_POINT('Ctrl Pts',(3.5007660381658,-1.,-1.35142377279535));
#54893=CARTESIAN_POINT('Ctrl Pts',(3.50408168106113,-1.,-1.3525703284343));
#54894=CARTESIAN_POINT('Ctrl Pts',(3.50913227060177,-1.,-1.35419113576022));
#54895=CARTESIAN_POINT('Ctrl Pts',(3.51542230699919,-1.,-1.35611275237288));
#54896=CARTESIAN_POINT('Ctrl Pts',(3.52261776117121,-1.,-1.35821701528975));
#54897=CARTESIAN_POINT('Ctrl Pts',(3.53034464961849,-1.,-1.36037259643827));
#54898=CARTESIAN_POINT('Ctrl Pts',(3.53824396425032,-1.,-1.36245507339334));
#54899=CARTESIAN_POINT('Ctrl Pts',(3.54602591832893,-1.,-1.36436666257568));
#54900=CARTESIAN_POINT('Ctrl Pts',(3.55353883995793,-1.,-1.36606145456711));
#54901=CARTESIAN_POINT('Ctrl Pts',(3.56077662028492,-1.,-1.36754771771174));
#54902=CARTESIAN_POINT('Ctrl Pts',(3.56782080304554,-1.,-1.36886584973349));
#54903=CARTESIAN_POINT('Ctrl Pts',(3.57479875549453,-1.,-1.37007229485646));
#54904=CARTESIAN_POINT('Ctrl Pts',(3.58183885982745,-1.,-1.37122241663073));
#54905=CARTESIAN_POINT('Ctrl Pts',(3.5890185384643,-1.,-1.37235053661));
#54906=CARTESIAN_POINT('Ctrl Pts',(3.59634627869117,-1.,-1.37346320103184));
#54907=CARTESIAN_POINT('Ctrl Pts',(3.60379020124038,-1.,-1.37455051379642));
#54908=CARTESIAN_POINT('Ctrl Pts',(3.61129546591082,-1.,-1.37559314436641));
#54909=CARTESIAN_POINT('Ctrl Pts',(3.61880481160408,-1.,-1.37657053403102));
#54910=CARTESIAN_POINT('Ctrl Pts',(3.62628098665112,-1.,-1.37746987919868));
#54911=CARTESIAN_POINT('Ctrl Pts',(3.63371727442448,-1.,-1.37829035457325));
#54912=CARTESIAN_POINT('Ctrl Pts',(3.64112507791112,-1.,-1.37903818567347));
#54913=CARTESIAN_POINT('Ctrl Pts',(3.64852652756444,-1.,-1.37972372481598));
#54914=CARTESIAN_POINT('Ctrl Pts',(3.65594554404396,-1.,-1.38035791051215));
#54915=CARTESIAN_POINT('Ctrl Pts',(3.66339848520874,-1.,-1.38094856333558));
#54916=CARTESIAN_POINT('Ctrl Pts',(3.67088843112282,-1.,-1.38149812653876));
#54917=CARTESIAN_POINT('Ctrl Pts',(3.6784103848243,-1.,-1.38200574290626));
#54918=CARTESIAN_POINT('Ctrl Pts',(3.68595444983844,-1.,-1.38246852827185));
#54919=CARTESIAN_POINT('Ctrl Pts',(3.69350967899523,-1.,-1.38288311171649));
#54920=CARTESIAN_POINT('Ctrl Pts',(3.70106792167894,-1.,-1.38324717612862));
#54921=CARTESIAN_POINT('Ctrl Pts',(3.70862680753343,-1.,-1.38356065402122));
#54922=CARTESIAN_POINT('Ctrl Pts',(3.7161876605181,-1.,-1.38382489984585));
#54923=CARTESIAN_POINT('Ctrl Pts',(3.72375409358805,-1.,-1.3840421342895));
#54924=CARTESIAN_POINT('Ctrl Pts',(3.73133035859283,-1.,-1.38421479111531));
#54925=CARTESIAN_POINT('Ctrl Pts',(3.73891976418099,-1.,-1.38434489156456));
#54926=CARTESIAN_POINT('Ctrl Pts',(3.7465231716786,-1.,-1.38443344984389));
#54927=CARTESIAN_POINT('Ctrl Pts',(3.75413976318727,-1.,-1.38448077997155));
#54928=CARTESIAN_POINT('Ctrl Pts',(3.76176768271347,-1.,-1.38448675253343));
#54929=CARTESIAN_POINT('Ctrl Pts',(3.76940473185775,-1.,-1.38445107339517));
#54930=CARTESIAN_POINT('Ctrl Pts',(3.77704902230441,-1.,-1.38437354551435));
#54931=CARTESIAN_POINT('Ctrl Pts',(3.78469969805134,-1.,-1.38425435883773));
#54932=CARTESIAN_POINT('Ctrl Pts',(3.79235669640907,-1.,-1.38409399694589));
#54933=CARTESIAN_POINT('Ctrl Pts',(3.80002044322169,-1.,-1.38389311766701));
#54934=CARTESIAN_POINT('Ctrl Pts',(3.80769156398429,-1.,-1.38365244046226));
#54935=CARTESIAN_POINT('Ctrl Pts',(3.81537060817765,-1.,-1.38337263902766));
#54936=CARTESIAN_POINT('Ctrl Pts',(3.82305771743715,-1.,-1.38305421262724));
#54937=CARTESIAN_POINT('Ctrl Pts',(3.83075266982138,-1.,-1.38269750245086));
#54938=CARTESIAN_POINT('Ctrl Pts',(3.83845502790609,-1.,-1.38230274828774));
#54939=CARTESIAN_POINT('Ctrl Pts',(3.84616425605705,-1.,-1.38187013346089));
#54940=CARTESIAN_POINT('Ctrl Pts',(3.85387983979557,-1.,-1.38139983115075));
#54941=CARTESIAN_POINT('Ctrl Pts',(3.86160143044187,-1.,-1.38089205993068));
#54942=CARTESIAN_POINT('Ctrl Pts',(3.86932885813403,-1.,-1.38034709213129));
#54943=CARTESIAN_POINT('Ctrl Pts',(3.87706205830865,-1.,-1.37976523097187));
#54944=CARTESIAN_POINT('Ctrl Pts',(3.88480102249461,-1.,-1.37914679719446));
#54945=CARTESIAN_POINT('Ctrl Pts',(3.89254574338385,-1.,-1.37849211287981));
#54946=CARTESIAN_POINT('Ctrl Pts',(3.90029615196255,-1.,-1.3778014851263));
#54947=CARTESIAN_POINT('Ctrl Pts',(3.90805209522729,-1.,-1.3770751963376));
#54948=CARTESIAN_POINT('Ctrl Pts',(3.91581337461825,-1.,-1.37631350505516));
#54949=CARTESIAN_POINT('Ctrl Pts',(3.92357976987132,-1.,-1.37551664448057));
#54950=CARTESIAN_POINT('Ctrl Pts',(3.93135106761941,-1.,-1.37468482215784));
#54951=CARTESIAN_POINT('Ctrl Pts',(3.93912709041791,-1.,-1.37381821967499));
#54952=CARTESIAN_POINT('Ctrl Pts',(3.94690771786926,-1.,-1.37291699203423));
#54953=CARTESIAN_POINT('Ctrl Pts',(3.95469287283105,-1.,-1.37198126433139));
#54954=CARTESIAN_POINT('Ctrl Pts',(3.96092458508407,-1.,-1.37120515615663));
#54955=CARTESIAN_POINT('Ctrl Pts',(3.96560037975788,-1.,-1.37060761746027));
#54956=CARTESIAN_POINT('Ctrl Pts',(3.9687184694173,-1.,-1.37020239094758));
#54957=CARTESIAN_POINT('Ctrl Pts',(3.97027773754922,-1.,-1.36999806084572));
#54958=CARTESIAN_POINT('',(4.01728681790024,-1.,-1.22531898815164));
#54959=CARTESIAN_POINT('',(3.97027773754922,-1.,-1.36999806084572));
#54960=CARTESIAN_POINT('',(3.62400312501199,-1.,-0.963899035118986));
#54961=CARTESIAN_POINT('Ctrl Pts',(4.01728681790024,-1.,-1.22531898815164));
#54962=CARTESIAN_POINT('Ctrl Pts',(4.01614544569895,-1.,-1.22423716681317));
#54963=CARTESIAN_POINT('Ctrl Pts',(4.01386104433519,-1.,-1.22207656455845));
#54964=CARTESIAN_POINT('Ctrl Pts',(4.01042947140789,-1.,-1.21884478244403));
#54965=CARTESIAN_POINT('Ctrl Pts',(4.00584409522722,-1.,-1.21455398918133));
#54966=CARTESIAN_POINT('Ctrl Pts',(4.00009577950721,-1.,-1.20922097029551));
#54967=CARTESIAN_POINT('Ctrl Pts',(3.99433084799666,-1.,-1.20391852375139));
#54968=CARTESIAN_POINT('Ctrl Pts',(3.98854928957189,-1.,-1.19864679609566));
#54969=CARTESIAN_POINT('Ctrl Pts',(3.98275111052561,-1.,-1.19340598349475));
#54970=CARTESIAN_POINT('Ctrl Pts',(3.97693634767754,-1.,-1.18819633715539));
#54971=CARTESIAN_POINT('Ctrl Pts',(3.97110505165415,-1.,-1.18301815039831));
#54972=CARTESIAN_POINT('Ctrl Pts',(3.96525726358159,-1.,-1.17787174135592));
#54973=CARTESIAN_POINT('Ctrl Pts',(3.95939299213276,-1.,-1.17275743590361));
#54974=CARTESIAN_POINT('Ctrl Pts',(3.95351219509876,-1.,-1.16767555244438));
#54975=CARTESIAN_POINT('Ctrl Pts',(3.94761474780583,-1.,-1.16262637999157));
#54976=CARTESIAN_POINT('Ctrl Pts',(3.94170046685203,-1.,-1.15761018340956));
#54977=CARTESIAN_POINT('Ctrl Pts',(3.9357691705628,-1.,-1.1526272271632));
#54978=CARTESIAN_POINT('Ctrl Pts',(3.92982073294257,-1.,-1.14767779451124));
#54979=CARTESIAN_POINT('Ctrl Pts',(3.92385513133997,-1.,-1.14276220561593));
#54980=CARTESIAN_POINT('Ctrl Pts',(3.91787251936827,-1.,-1.13788084225554));
#54981=CARTESIAN_POINT('Ctrl Pts',(3.91187321145649,-1.,-1.13303414693896));
#54982=CARTESIAN_POINT('Ctrl Pts',(3.90585753318737,-1.,-1.12822258281553));
#54983=CARTESIAN_POINT('Ctrl Pts',(3.89982569750025,-1.,-1.12344660099043));
#54984=CARTESIAN_POINT('Ctrl Pts',(3.89377768340344,-1.,-1.11870660794603));
#54985=CARTESIAN_POINT('Ctrl Pts',(3.88771308285171,-1.,-1.11400292434429));
#54986=CARTESIAN_POINT('Ctrl Pts',(3.88163105531724,-1.,-1.10933577224008));
#54987=CARTESIAN_POINT('Ctrl Pts',(3.87553067187514,-1.,-1.10470536603287));
#54988=CARTESIAN_POINT('Ctrl Pts',(3.86941120134849,-1.,-1.10011198761195));
#54989=CARTESIAN_POINT('Ctrl Pts',(3.86327241021247,-1.,-1.09555606505013));
#54990=CARTESIAN_POINT('Ctrl Pts',(3.85711487933931,-1.,-1.09103825516294));
#54991=CARTESIAN_POINT('Ctrl Pts',(3.85094025222713,-1.,-1.08655950846384));
#54992=CARTESIAN_POINT('Ctrl Pts',(3.8447504803063,-1.,-1.08212087917991));
#54993=CARTESIAN_POINT('Ctrl Pts',(3.83854714117491,-1.,-1.07772335353858));
#54994=CARTESIAN_POINT('Ctrl Pts',(3.83233071195144,-1.,-1.07336766633459));
#54995=CARTESIAN_POINT('Ctrl Pts',(3.82609989967276,-1.,-1.06905413180359));
#54996=CARTESIAN_POINT('Ctrl Pts',(3.81985083953012,-1.,-1.0647824403893));
#54997=CARTESIAN_POINT('Ctrl Pts',(3.8135786611749,-1.,-1.06055206187299));
#54998=CARTESIAN_POINT('Ctrl Pts',(3.80727913637791,-1.,-1.05636266918644));
#54999=CARTESIAN_POINT('Ctrl Pts',(3.80095039790681,-1.,-1.05221457990016));
#55000=CARTESIAN_POINT('Ctrl Pts',(3.79459440308786,-1.,-1.04810913267639));
#55001=CARTESIAN_POINT('Ctrl Pts',(3.78821910787179,-1.,-1.04404924374422));
#55002=CARTESIAN_POINT('Ctrl Pts',(3.7818353500817,-1.,-1.04003862055798));
#55003=CARTESIAN_POINT('Ctrl Pts',(3.77545283140427,-1.,-1.03608074678008));
#55004=CARTESIAN_POINT('Ctrl Pts',(3.76907609832516,-1.,-1.03217786604919));
#55005=CARTESIAN_POINT('Ctrl Pts',(3.76270122291245,-1.,-1.02833014458184));
#55006=CARTESIAN_POINT('Ctrl Pts',(3.75631037456224,-1.,-1.02453429444668));
#55007=CARTESIAN_POINT('Ctrl Pts',(3.74987777155873,-1.,-1.02078510487439));
#55008=CARTESIAN_POINT('Ctrl Pts',(3.74337942504993,-1.,-1.01707794311088));
#55009=CARTESIAN_POINT('Ctrl Pts',(3.73680245055747,-1.,-1.01341114319906));
#55010=CARTESIAN_POINT('Ctrl Pts',(3.73015276704407,-1.,-1.00978798539491));
#55011=CARTESIAN_POINT('Ctrl Pts',(3.72346803750544,-1.,-1.00622000735696));
#55012=CARTESIAN_POINT('Ctrl Pts',(3.71680667125047,-1.,-1.00272423396802));
#55013=CARTESIAN_POINT('Ctrl Pts',(3.7102243971387,-1.,-0.999317260756345));
#55014=CARTESIAN_POINT('Ctrl Pts',(3.70375282282107,-1.,-0.996009819772432));
#55015=CARTESIAN_POINT('Ctrl Pts',(3.69738123415696,-1.,-0.992802218332104));
#55016=CARTESIAN_POINT('Ctrl Pts',(3.69102682138955,-1.,-0.989676715398859));
#55017=CARTESIAN_POINT('Ctrl Pts',(3.6845531792623,-1.,-0.986602639864286));
#55018=CARTESIAN_POINT('Ctrl Pts',(3.67782408841876,-1.,-0.983550791470865));
#55019=CARTESIAN_POINT('Ctrl Pts',(3.67074983340444,-1.,-0.980505922458495));
#55020=CARTESIAN_POINT('Ctrl Pts',(3.66333049637403,-1.,-0.977478312751416));
#55021=CARTESIAN_POINT('Ctrl Pts',(3.6557157673487,-1.,-0.974519971354139));
#55022=CARTESIAN_POINT('Ctrl Pts',(3.64819756447072,-1.,-0.971722122060278));
#55023=CARTESIAN_POINT('Ctrl Pts',(3.64113946505393,-1.,-0.969195124674829));
#55024=CARTESIAN_POINT('Ctrl Pts',(3.6349212208096,-1.,-0.967052554540878));
#55025=CARTESIAN_POINT('Ctrl Pts',(3.62988252139998,-1.,-0.965395153165716));
#55026=CARTESIAN_POINT('Ctrl Pts',(3.62652618145252,-1.,-0.964373850166081));
#55027=CARTESIAN_POINT('Ctrl Pts',(3.62489305727516,-1.,-0.963957782642589));
#55028=CARTESIAN_POINT('Ctrl Pts',(3.62424461507455,-1.,-0.963861297423579));
#55029=CARTESIAN_POINT('Ctrl Pts',(3.62404828878374,-1.,-0.963880158556713));
#55030=CARTESIAN_POINT('Ctrl Pts',(3.62400312501199,-1.,-0.963899035118986));
#55031=CARTESIAN_POINT('',(3.66661143271648,-1.,-0.786422660833743));
#55032=CARTESIAN_POINT('Origin',(0.,-1.,0.));
#55033=CARTESIAN_POINT('',(4.13571194405636,-1.,-0.73204283740062));
#55034=CARTESIAN_POINT('Ctrl Pts',(3.66661143271648,-1.,-0.786422660833743));
#55035=CARTESIAN_POINT('Ctrl Pts',(3.66664310415236,-1.,-0.786459983896781));
#55036=CARTESIAN_POINT('Ctrl Pts',(3.66680946938396,-1.,-0.78656591955989));
#55037=CARTESIAN_POINT('Ctrl Pts',(3.66743103898844,-1.,-0.7867743371985));
#55038=CARTESIAN_POINT('Ctrl Pts',(3.66907505398769,-1.,-0.787145041181589));
#55039=CARTESIAN_POINT('Ctrl Pts',(3.672529236635,-1.,-0.787758799995427));
#55040=CARTESIAN_POINT('Ctrl Pts',(3.67777119516438,-1.,-0.788569566220663));
#55041=CARTESIAN_POINT('Ctrl Pts',(3.68428439784285,-1.,-0.789483546065159));
#55042=CARTESIAN_POINT('Ctrl Pts',(3.69172044327754,-1.,-0.79043628498958));
#55043=CARTESIAN_POINT('Ctrl Pts',(3.69968940808982,-1.,-0.791356575696509));
#55044=CARTESIAN_POINT('Ctrl Pts',(3.70781724021879,-1.,-0.792177688845968));
#55045=CARTESIAN_POINT('Ctrl Pts',(3.7158024239604,-1.,-0.792848377370116));
#55046=CARTESIAN_POINT('Ctrl Pts',(3.7234879729357,-1.,-0.793347023783871));
#55047=CARTESIAN_POINT('Ctrl Pts',(3.7308691469564,-1.,-0.793682750269348));
#55048=CARTESIAN_POINT('Ctrl Pts',(3.73803280541576,-1.,-0.793882700936791));
#55049=CARTESIAN_POINT('Ctrl Pts',(3.74511357728827,-1.,-0.79398270045988));
#55050=CARTESIAN_POINT('Ctrl Pts',(3.75224692493895,-1.,-0.794017347371441));
#55051=CARTESIAN_POINT('Ctrl Pts',(3.75951468666325,-1.,-0.794008429135047));
#55052=CARTESIAN_POINT('Ctrl Pts',(3.76692626931184,-1.,-0.793961083689141));
#55053=CARTESIAN_POINT('Ctrl Pts',(3.77444863801264,-1.,-0.793870523787515));
#55054=CARTESIAN_POINT('Ctrl Pts',(3.78202460377617,-1.,-0.79372623578134));
#55055=CARTESIAN_POINT('Ctrl Pts',(3.78959439439222,-1.,-0.793516871680966));
#55056=CARTESIAN_POINT('Ctrl Pts',(3.79711921389862,-1.,-0.793235612973201));
#55057=CARTESIAN_POINT('Ctrl Pts',(3.80459229925598,-1.,-0.792882695234693));
#55058=CARTESIAN_POINT('Ctrl Pts',(3.81202588694726,-1.,-0.792462483517568));
#55059=CARTESIAN_POINT('Ctrl Pts',(3.81944345442237,-1.,-0.791981740718607));
#55060=CARTESIAN_POINT('Ctrl Pts',(3.82687033899799,-1.,-0.791447528662381));
#55061=CARTESIAN_POINT('Ctrl Pts',(3.83432392054804,-1.,-0.79086501270534));
#55062=CARTESIAN_POINT('Ctrl Pts',(3.84180762342476,-1.,-0.790236124191289));
#55063=CARTESIAN_POINT('Ctrl Pts',(3.8493163780891,-1.,-0.789560798155619));
#55064=CARTESIAN_POINT('Ctrl Pts',(3.85683995872536,-1.,-0.788837734090688));
#55065=CARTESIAN_POINT('Ctrl Pts',(3.86436702561342,-1.,-0.788065315093771));
#55066=CARTESIAN_POINT('Ctrl Pts',(3.87188916600905,-1.,-0.787242527617981));
#55067=CARTESIAN_POINT('Ctrl Pts',(3.87940402818186,-1.,-0.786369675812592));
#55068=CARTESIAN_POINT('Ctrl Pts',(3.88691313167399,-1.,-0.785447890340723));
#55069=CARTESIAN_POINT('Ctrl Pts',(3.89442039235105,-1.,-0.784478799358336));
#55070=CARTESIAN_POINT('Ctrl Pts',(3.90193039043971,-1.,-0.783464141529083));
#55071=CARTESIAN_POINT('Ctrl Pts',(3.90944671004536,-1.,-0.782405395622759));
#55072=CARTESIAN_POINT('Ctrl Pts',(3.9169703605466,-1.,-0.781303428618344));
#55073=CARTESIAN_POINT('Ctrl Pts',(3.92450058323799,-1.,-0.780158678615507));
#55074=CARTESIAN_POINT('Ctrl Pts',(3.93203552473153,-1.,-0.778971308134786));
#55075=CARTESIAN_POINT('Ctrl Pts',(3.93957296768098,-1.,-0.77774137056855));
#55076=CARTESIAN_POINT('Ctrl Pts',(3.94711101619471,-1.,-0.77646896669796));
#55077=CARTESIAN_POINT('Ctrl Pts',(3.95464885452364,-1.,-0.775154418039442));
#55078=CARTESIAN_POINT('Ctrl Pts',(3.96218649639876,-1.,-0.773798212026683));
#55079=CARTESIAN_POINT('Ctrl Pts',(3.96972446532832,-1.,-0.772400931772239));
#55080=CARTESIAN_POINT('Ctrl Pts',(3.97726349165507,-1.,-0.770963190030504));
#55081=CARTESIAN_POINT('Ctrl Pts',(3.98480422348403,-1.,-0.76948556624546));
#55082=CARTESIAN_POINT('Ctrl Pts',(3.99234687880892,-1.,-0.767968531377708));
#55083=CARTESIAN_POINT('Ctrl Pts',(3.99989129179464,-1.,-0.766412457135786));
#55084=CARTESIAN_POINT('Ctrl Pts',(4.00743706791366,-1.,-0.764817648784947));
#55085=CARTESIAN_POINT('Ctrl Pts',(4.01498370680434,-1.,-0.763184371182827));
#55086=CARTESIAN_POINT('Ctrl Pts',(4.02253072741347,-1.,-0.761512875859942));
#55087=CARTESIAN_POINT('Ctrl Pts',(4.0300778195465,-1.,-0.759803433244166));
#55088=CARTESIAN_POINT('Ctrl Pts',(4.03762485803468,-1.,-0.758056338885554));
#55089=CARTESIAN_POINT('Ctrl Pts',(4.04517182654344,-1.,-0.756271902370187));
#55090=CARTESIAN_POINT('Ctrl Pts',(4.05271876688106,-1.,-0.754450441816412));
#55091=CARTESIAN_POINT('Ctrl Pts',(4.06026572221399,-1.,-0.752592276482869));
#55092=CARTESIAN_POINT('Ctrl Pts',(4.06781267241886,-1.,-0.750697720483176));
#55093=CARTESIAN_POINT('Ctrl Pts',(4.07535951055363,-1.,-0.748767076679177));
#55094=CARTESIAN_POINT('Ctrl Pts',(4.08290608094789,-1.,-0.746800631490822));
#55095=CARTESIAN_POINT('Ctrl Pts',(4.09045220253011,-1.,-0.744798649705514));
#55096=CARTESIAN_POINT('Ctrl Pts',(4.09799769702712,-1.,-0.742761369690018));
#55097=CARTESIAN_POINT('Ctrl Pts',(4.1055424175856,-1.,-0.740688998555152));
#55098=CARTESIAN_POINT('Ctrl Pts',(4.11308626953795,-1.,-0.738581708229119));
#55099=CARTESIAN_POINT('Ctrl Pts',(4.12062919626082,-1.,-0.736439634335347));
#55100=CARTESIAN_POINT('Ctrl Pts',(4.12666277572794,-1.,-0.734698226767513));
#55101=CARTESIAN_POINT('Ctrl Pts',(4.13118752796397,-1.,-0.733376589325634));
#55102=CARTESIAN_POINT('Ctrl Pts',(4.13420383737278,-1.,-0.732488575135926));
#55103=CARTESIAN_POINT('Ctrl Pts',(4.13571194405636,-1.,-0.73204283740062));
#55104=CARTESIAN_POINT('',(4.15950947128175,-1.,-0.581791163835815));
#55105=CARTESIAN_POINT('',(4.13571194405636,-1.,-0.73204283740062));
#55106=CARTESIAN_POINT('',(3.73017266276632,-1.,-0.385112848332549));
#55107=CARTESIAN_POINT('Ctrl Pts',(4.15950947128175,-1.,-0.581791163835815));
#55108=CARTESIAN_POINT('Ctrl Pts',(4.15821291712391,-1.,-0.580901211462913));
#55109=CARTESIAN_POINT('Ctrl Pts',(4.15561864787379,-1.,-0.579124568912544));
#55110=CARTESIAN_POINT('Ctrl Pts',(4.1517237611974,-1.,-0.576469391673917));
#55111=CARTESIAN_POINT('Ctrl Pts',(4.14652361065787,-1.,-0.572948736066277));
#55112=CARTESIAN_POINT('Ctrl Pts',(4.14001179828669,-1.,-0.568580610187116));
#55113=CARTESIAN_POINT('Ctrl Pts',(4.13348835726086,-1.,-0.564245279535706));
#55114=CARTESIAN_POINT('Ctrl Pts',(4.12695329951859,-1.,-0.559942890594628));
#55115=CARTESIAN_POINT('Ctrl Pts',(4.1204066619623,-1.,-0.555673636130778));
#55116=CARTESIAN_POINT('Ctrl Pts',(4.11384852025578,-1.,-0.551437758498247));
#55117=CARTESIAN_POINT('Ctrl Pts',(4.1072789702877,-1.,-0.54723553948676));
#55118=CARTESIAN_POINT('Ctrl Pts',(4.10069810244473,-1.,-0.543067286878457));
#55119=CARTESIAN_POINT('Ctrl Pts',(4.09410597627116,-1.,-0.538933321179921));
#55120=CARTESIAN_POINT('Ctrl Pts',(4.08750259988693,-1.,-0.534833963477));
#55121=CARTESIAN_POINT('Ctrl Pts',(4.08088789536488,-1.,-0.530769518728076));
#55122=CARTESIAN_POINT('Ctrl Pts',(4.07426172299496,-1.,-0.526740277227));
#55123=CARTESIAN_POINT('Ctrl Pts',(4.06762394471075,-1.,-0.522746528602768));
#55124=CARTESIAN_POINT('Ctrl Pts',(4.06097448037934,-1.,-0.51878857233681));
#55125=CARTESIAN_POINT('Ctrl Pts',(4.05431335771261,-1.,-0.514866728193104));
#55126=CARTESIAN_POINT('Ctrl Pts',(4.04764078815591,-1.,-0.510981349219174));
#55127=CARTESIAN_POINT('Ctrl Pts',(4.04095715149074,-1.,-0.507132823288362));
#55128=CARTESIAN_POINT('Ctrl Pts',(4.0342628417439,-1.,-0.503321556915514));
#55129=CARTESIAN_POINT('Ctrl Pts',(4.0275581398015,-1.,-0.49954796234089));
#55130=CARTESIAN_POINT('Ctrl Pts',(4.02084308851813,-1.,-0.495812444326223));
#55131=CARTESIAN_POINT('Ctrl Pts',(4.01411733503486,-1.,-0.492115383417931));
#55132=CARTESIAN_POINT('Ctrl Pts',(4.0073800839092,-1.,-0.488457130424531));
#55133=CARTESIAN_POINT('Ctrl Pts',(4.00063045119234,-1.,-0.484838042421754));
#55134=CARTESIAN_POINT('Ctrl Pts',(3.99386775880655,-1.,-0.481258512209638));
#55135=CARTESIAN_POINT('Ctrl Pts',(3.98709184306743,-1.,-0.477718999122033));
#55136=CARTESIAN_POINT('Ctrl Pts',(3.9803033804443,-1.,-0.474220061019542));
#55137=CARTESIAN_POINT('Ctrl Pts',(3.97350414289415,-1.,-0.470762379613478));
#55138=CARTESIAN_POINT('Ctrl Pts',(3.96669622273946,-1.,-0.467346690880672));
#55139=CARTESIAN_POINT('Ctrl Pts',(3.95988133243543,-1.,-0.463973722115745));
#55140=CARTESIAN_POINT('Ctrl Pts',(3.95306005817363,-1.,-0.460644124429119));
#55141=CARTESIAN_POINT('Ctrl Pts',(3.94623117206675,-1.,-0.457358410451674));
#55142=CARTESIAN_POINT('Ctrl Pts',(3.93939080846298,-1.,-0.454116879027576));
#55143=CARTESIAN_POINT('Ctrl Pts',(3.93253407403128,-1.,-0.450919768356347));
#55144=CARTESIAN_POINT('Ctrl Pts',(3.92565674143424,-1.,-0.447767416837297));
#55145=CARTESIAN_POINT('Ctrl Pts',(3.91875701610721,-1.,-0.444660430230593));
#55146=CARTESIAN_POINT('Ctrl Pts',(3.91183704069146,-1.,-0.441599824524048));
#55147=CARTESIAN_POINT('Ctrl Pts',(3.90490512938546,-1.,-0.438587235458234));
#55148=CARTESIAN_POINT('Ctrl Pts',(3.8979725665544,-1.,-0.435624629433506));
#55149=CARTESIAN_POINT('Ctrl Pts',(3.89104947940592,-1.,-0.43271392954444));
#55150=CARTESIAN_POINT('Ctrl Pts',(3.88414070943334,-1.,-0.429856640579734));
#55151=CARTESIAN_POINT('Ctrl Pts',(3.87724240306609,-1.,-0.427053541173469));
#55152=CARTESIAN_POINT('Ctrl Pts',(3.87033643487882,-1.,-0.424304173195143));
#55153=CARTESIAN_POINT('Ctrl Pts',(3.86339652542749,-1.,-0.421607423177576));
#55154=CARTESIAN_POINT('Ctrl Pts',(3.85639825648031,-1.,-0.41896246808681));
#55155=CARTESIAN_POINT('Ctrl Pts',(3.8493286415751,-1.,-0.41636967805292));
#55156=CARTESIAN_POINT('Ctrl Pts',(3.84219403994742,-1.,-0.413831367016727));
#55157=CARTESIAN_POINT('Ctrl Pts',(3.83503345578645,-1.,-0.41135303879846));
#55158=CARTESIAN_POINT('Ctrl Pts',(3.82790724256397,-1.,-0.408942371447377));
#55159=CARTESIAN_POINT('Ctrl Pts',(3.82087303913741,-1.,-0.406607038258907));
#55160=CARTESIAN_POINT('Ctrl Pts',(3.81396374287762,-1.,-0.404352694628237));
#55161=CARTESIAN_POINT('Ctrl Pts',(3.80716881962763,-1.,-0.402181320148475));
#55162=CARTESIAN_POINT('Ctrl Pts',(3.80040370384659,-1.,-0.400088346504727));
#55163=CARTESIAN_POINT('Ctrl Pts',(3.79352887163457,-1.,-0.398064818684159));
#55164=CARTESIAN_POINT('Ctrl Pts',(3.78640521279479,-1.,-0.396103205335029));
#55165=CARTESIAN_POINT('Ctrl Pts',(3.77894173114368,-1.,-0.394202481011595));
#55166=CARTESIAN_POINT('Ctrl Pts',(3.77114011595892,-1.,-0.392372786223347));
#55167=CARTESIAN_POINT('Ctrl Pts',(3.76315635032993,-1.,-0.390642072979259));
#55168=CARTESIAN_POINT('Ctrl Pts',(3.75529302894757,-1.,-0.389054775898251));
#55169=CARTESIAN_POINT('Ctrl Pts',(3.74792651696269,-1.,-0.387663020050396));
#55170=CARTESIAN_POINT('Ctrl Pts',(3.74144965781088,-1.,-0.386519576222036));
#55171=CARTESIAN_POINT('Ctrl Pts',(3.73621371845475,-1.,-0.385670806454744));
#55172=CARTESIAN_POINT('Ctrl Pts',(3.73273893363318,-1.,-0.385187124633965));
#55173=CARTESIAN_POINT('Ctrl Pts',(3.73106082862399,-1.,-0.385031656499142));
#55174=CARTESIAN_POINT('Ctrl Pts',(3.73040527620929,-1.,-0.385037797882046));
#55175=CARTESIAN_POINT('Ctrl Pts',(3.73021431755218,-1.,-0.385087139001609));
#55176=CARTESIAN_POINT('Ctrl Pts',(3.73017266276632,-1.,-0.385112848332549));
#55177=CARTESIAN_POINT('',(3.74449296982994,-1.,-0.203156094897896));
#55178=CARTESIAN_POINT('Origin',(0.,-1.,0.));
#55179=CARTESIAN_POINT('',(4.19931119685982,-1.,-0.0760622897878241));
#55180=CARTESIAN_POINT('Ctrl Pts',(3.74449296982994,-1.,-0.203156094897896));
#55181=CARTESIAN_POINT('Ctrl Pts',(3.74453008995129,-1.,-0.203188003947965));
#55182=CARTESIAN_POINT('Ctrl Pts',(3.74471097893961,-1.,-0.203266610111264));
#55183=CARTESIAN_POINT('Ctrl Pts',(3.74535749969262,-1.,-0.203375226874332));
#55184=CARTESIAN_POINT('Ctrl Pts',(3.74703926501843,-1.,-0.203484186269315));
#55185=CARTESIAN_POINT('Ctrl Pts',(3.75054693397716,-1.,-0.203550035479097));
#55186=CARTESIAN_POINT('Ctrl Pts',(3.75585118707924,-1.,-0.203530796848404));
#55187=CARTESIAN_POINT('Ctrl Pts',(3.76242717937273,-1.,-0.203414634707647));
#55188=CARTESIAN_POINT('Ctrl Pts',(3.76992071595267,-1.,-0.203192390045338));
#55189=CARTESIAN_POINT('Ctrl Pts',(3.77793553476879,-1.,-0.202854729699197));
#55190=CARTESIAN_POINT('Ctrl Pts',(3.78609175019317,-1.,-0.202394260512193));
#55191=CARTESIAN_POINT('Ctrl Pts',(3.79408354187274,-1.,-0.201807533800799));
#55192=CARTESIAN_POINT('Ctrl Pts',(3.80175247447171,-1.,-0.201097756307252));
#55193=CARTESIAN_POINT('Ctrl Pts',(3.80909529318501,-1.,-0.20027467943329));
#55194=CARTESIAN_POINT('Ctrl Pts',(3.81620203429702,-1.,-0.199351525297397));
#55195=CARTESIAN_POINT('Ctrl Pts',(3.82321127348981,-1.,-0.19834261690047));
#55196=CARTESIAN_POINT('Ctrl Pts',(3.83026221776488,-1.,-0.197260935827375));
#55197=CARTESIAN_POINT('Ctrl Pts',(3.83743910616265,-1.,-0.19611519897189));
#55198=CARTESIAN_POINT('Ctrl Pts',(3.84475203347052,-1.,-0.194909009460255));
#55199=CARTESIAN_POINT('Ctrl Pts',(3.85216762264019,-1.,-0.193642806777748));
#55200=CARTESIAN_POINT('Ctrl Pts',(3.85962774407652,-1.,-0.19231515304498));
#55201=CARTESIAN_POINT('Ctrl Pts',(3.8670715862477,-1.,-0.190924190418613));
#55202=CARTESIAN_POINT('Ctrl Pts',(3.87445976418377,-1.,-0.189469253358255));
#55203=CARTESIAN_POINT('Ctrl Pts',(3.88178563496187,-1.,-0.187951632512664));
#55204=CARTESIAN_POINT('Ctrl Pts',(3.88906196725817,-1.,-0.186373724985263));
#55205=CARTESIAN_POINT('Ctrl Pts',(3.89631300742633,-1.,-0.184738537728035));
#55206=CARTESIAN_POINT('Ctrl Pts',(3.90356488555138,-1.,-0.183049081993193));
#55207=CARTESIAN_POINT('Ctrl Pts',(3.91083557557193,-1.,-0.181307740731796));
#55208=CARTESIAN_POINT('Ctrl Pts',(3.91812876180948,-1.,-0.179515885822895));
#55209=CARTESIAN_POINT('Ctrl Pts',(3.92543942697672,-1.,-0.177674246152328));
#55210=CARTESIAN_POINT('Ctrl Pts',(3.93275726771049,-1.,-0.175783136893873));
#55211=CARTESIAN_POINT('Ctrl Pts',(3.94007083096214,-1.,-0.173842734974608));
#55212=CARTESIAN_POINT('Ctrl Pts',(3.94737164900861,-1.,-0.171853355369233));
#55213=CARTESIAN_POINT('Ctrl Pts',(3.95465744665263,-1.,-0.16981566637413));
#55214=CARTESIAN_POINT('Ctrl Pts',(3.96192990160296,-1.,-0.167730547023312));
#55215=CARTESIAN_POINT('Ctrl Pts',(3.9691931362141,-1.,-0.165598992851098));
#55216=CARTESIAN_POINT('Ctrl Pts',(3.97645194630944,-1.,-0.163422004609999));
#55217=CARTESIAN_POINT('Ctrl Pts',(3.98371010319866,-1.,-0.161200482186088));
#55218=CARTESIAN_POINT('Ctrl Pts',(3.99096873945862,-1.,-0.158935123982796));
#55219=CARTESIAN_POINT('Ctrl Pts',(3.99822717425869,-1.,-0.156626481393736));
#55220=CARTESIAN_POINT('Ctrl Pts',(4.00548360245297,-1.,-0.15427500487231));
#55221=CARTESIAN_POINT('Ctrl Pts',(4.01273584234684,-1.,-0.151881094022909));
#55222=CARTESIAN_POINT('Ctrl Pts',(4.01998203715588,-1.,-0.149445144968708));
#55223=CARTESIAN_POINT('Ctrl Pts',(4.02722143147048,-1.,-0.146967602878999));
#55224=CARTESIAN_POINT('Ctrl Pts',(4.03445411510403,-1.,-0.144448947038352));
#55225=CARTESIAN_POINT('Ctrl Pts',(4.04168069633842,-1.,-0.141889671485508));
#55226=CARTESIAN_POINT('Ctrl Pts',(4.04890199238056,-1.,-0.13929026718006));
#55227=CARTESIAN_POINT('Ctrl Pts',(4.05611873400122,-1.,-0.136651205046111));
#55228=CARTESIAN_POINT('Ctrl Pts',(4.06333121018476,-1.,-0.133972916144225));
#55229=CARTESIAN_POINT('Ctrl Pts',(4.07053931528579,-1.,-0.131255793548914));
#55230=CARTESIAN_POINT('Ctrl Pts',(4.07774270738809,-1.,-0.128500200484814));
#55231=CARTESIAN_POINT('Ctrl Pts',(4.08494093372315,-1.,-0.12570647682253));
#55232=CARTESIAN_POINT('Ctrl Pts',(4.09213355850836,-1.,-0.122874946249119));
#55233=CARTESIAN_POINT('Ctrl Pts',(4.09932031767243,-1.,-0.120005924388162));
#55234=CARTESIAN_POINT('Ctrl Pts',(4.10650113382187,-1.,-0.117099722731705));
#55235=CARTESIAN_POINT('Ctrl Pts',(4.11367603925313,-1.,-0.114156649609602));
#55236=CARTESIAN_POINT('Ctrl Pts',(4.12084512502444,-1.,-0.111177012683378));
#55237=CARTESIAN_POINT('Ctrl Pts',(4.12800848371386,-1.,-0.10816112052835));
#55238=CARTESIAN_POINT('Ctrl Pts',(4.13516614458396,-1.,-0.105109286538864));
#55239=CARTESIAN_POINT('Ctrl Pts',(4.14231804938737,-1.,-0.102021826577454));
#55240=CARTESIAN_POINT('Ctrl Pts',(4.1494640891762,-1.,-0.0988990478899816));
#55241=CARTESIAN_POINT('Ctrl Pts',(4.15660412653006,-1.,-0.0957412403297072));
#55242=CARTESIAN_POINT('Ctrl Pts',(4.16373802265942,-1.,-0.0925486672167695));
#55243=CARTESIAN_POINT('Ctrl Pts',(4.17086566491823,-1.,-0.0893215560850332));
#55244=CARTESIAN_POINT('Ctrl Pts',(4.17798698669991,-1.,-0.086060091555252));
#55245=CARTESIAN_POINT('Ctrl Pts',(4.1851019532944,-1.,-0.0827644164389515));
#55246=CARTESIAN_POINT('Ctrl Pts',(4.19078883322483,-1.,-0.0801005887117608));
#55247=CARTESIAN_POINT('Ctrl Pts',(4.19505112860624,-1.,-0.0780873956244407));
#55248=CARTESIAN_POINT('Ctrl Pts',(4.19789138621624,-1.,-0.07673845961422));
#55249=CARTESIAN_POINT('Ctrl Pts',(4.19931119685982,-1.,-0.0760622897878241));
#55250=CARTESIAN_POINT('',(4.19931119685982,-1.,0.0760622897878241));
#55251=CARTESIAN_POINT('',(4.19931119685982,-1.,-0.0760622897878241));
#55252=CARTESIAN_POINT('',(3.74449296983004,-1.,0.2031560948961));
#55253=CARTESIAN_POINT('Ctrl Pts',(4.19931119685982,-1.,0.0760622897878241));
#55254=CARTESIAN_POINT('Ctrl Pts',(4.1978913862118,-1.,0.0767384596141459));
#55255=CARTESIAN_POINT('Ctrl Pts',(4.19505112859416,-1.,0.0780873956242392));
#55256=CARTESIAN_POINT('Ctrl Pts',(4.19078883320504,-1.,0.0801005887114315));
#55257=CARTESIAN_POINT('Ctrl Pts',(4.18510195327123,-1.,0.0827644164385674));
#55258=CARTESIAN_POINT('Ctrl Pts',(4.17798698668094,-1.,0.0860600915549391));
#55259=CARTESIAN_POINT('Ctrl Pts',(4.17086566490794,-1.,0.0893215560848644));
#55260=CARTESIAN_POINT('Ctrl Pts',(4.16373802265839,-1.,0.0925486672167526));
#55261=CARTESIAN_POINT('Ctrl Pts',(4.15660412653577,-1.,0.0957412403298002));
#55262=CARTESIAN_POINT('Ctrl Pts',(4.14946408918485,-1.,0.0988990478901221));
#55263=CARTESIAN_POINT('Ctrl Pts',(4.14231804939538,-1.,0.102021826577583));
#55264=CARTESIAN_POINT('Ctrl Pts',(4.13516614458895,-1.,0.105109286538945));
#55265=CARTESIAN_POINT('Ctrl Pts',(4.12800848371504,-1.,0.108161120528369));
#55266=CARTESIAN_POINT('Ctrl Pts',(4.1208451250225,-1.,0.111177012683346));
#55267=CARTESIAN_POINT('Ctrl Pts',(4.11367603924961,-1.,0.114156649609545));
#55268=CARTESIAN_POINT('Ctrl Pts',(4.10650113381833,-1.,0.117099722731648));
#55269=CARTESIAN_POINT('Ctrl Pts',(4.09932031767002,-1.,0.120005924388124));
#55270=CARTESIAN_POINT('Ctrl Pts',(4.09213355850756,-1.,0.122874946249106));
#55271=CARTESIAN_POINT('Ctrl Pts',(4.08494093372377,-1.,0.125706476822539));
#55272=CARTESIAN_POINT('Ctrl Pts',(4.07774270738954,-1.,0.128500200484837));
#55273=CARTESIAN_POINT('Ctrl Pts',(4.0705393152874,-1.,0.13125579354894));
#55274=CARTESIAN_POINT('Ctrl Pts',(4.06333121018596,-1.,0.133972916144244));
#55275=CARTESIAN_POINT('Ctrl Pts',(4.05611873400172,-1.,0.136651205046119));
#55276=CARTESIAN_POINT('Ctrl Pts',(4.04890199238036,-1.,0.139290267180057));
#55277=CARTESIAN_POINT('Ctrl Pts',(4.04168069633781,-1.,0.1418896714855));
#55278=CARTESIAN_POINT('Ctrl Pts',(4.03445411510333,-1.,0.144448947038344));
#55279=CARTESIAN_POINT('Ctrl Pts',(4.02722143146994,-1.,0.146967602878994));
#55280=CARTESIAN_POINT('Ctrl Pts',(4.01998203715564,-1.,0.149445144968706));
#55281=CARTESIAN_POINT('Ctrl Pts',(4.01273584234689,-1.,0.15188109402291));
#55282=CARTESIAN_POINT('Ctrl Pts',(4.00548360245319,-1.,0.15427500487231));
#55283=CARTESIAN_POINT('Ctrl Pts',(3.99822717425893,-1.,0.156626481393734));
#55284=CARTESIAN_POINT('Ctrl Pts',(3.99096873945878,-1.,0.158935123982793));
#55285=CARTESIAN_POINT('Ctrl Pts',(3.98371010319872,-1.,0.161200482186084));
#55286=CARTESIAN_POINT('Ctrl Pts',(3.97645194630943,-1.,0.163422004609999));
#55287=CARTESIAN_POINT('Ctrl Pts',(3.96919313621407,-1.,0.165598992851102));
#55288=CARTESIAN_POINT('Ctrl Pts',(3.96192990160296,-1.,0.167730547023319));
#55289=CARTESIAN_POINT('Ctrl Pts',(3.95465744665268,-1.,0.169815666374138));
#55290=CARTESIAN_POINT('Ctrl Pts',(3.94737164900868,-1.,0.17185335536924));
#55291=CARTESIAN_POINT('Ctrl Pts',(3.94007083096217,-1.,0.173842734974609));
#55292=CARTESIAN_POINT('Ctrl Pts',(3.93275726771042,-1.,0.175783136893867));
#55293=CARTESIAN_POINT('Ctrl Pts',(3.92543942697655,-1.,0.177674246152317));
#55294=CARTESIAN_POINT('Ctrl Pts',(3.91812876180926,-1.,0.179515885822881));
#55295=CARTESIAN_POINT('Ctrl Pts',(3.91083557557175,-1.,0.181307740731785));
#55296=CARTESIAN_POINT('Ctrl Pts',(3.90356488555132,-1.,0.18304908199319));
#55297=CARTESIAN_POINT('Ctrl Pts',(3.89631300742646,-1.,0.184738537728042));
#55298=CARTESIAN_POINT('Ctrl Pts',(3.88906196725848,-1.,0.18637372498528));
#55299=CARTESIAN_POINT('Ctrl Pts',(3.88178563496228,-1.,0.187951632512684));
#55300=CARTESIAN_POINT('Ctrl Pts',(3.87445976418412,-1.,0.189469253358272));
#55301=CARTESIAN_POINT('Ctrl Pts',(3.86707158624783,-1.,0.190924190418619));
#55302=CARTESIAN_POINT('Ctrl Pts',(3.85962774407633,-1.,0.19231515304497));
#55303=CARTESIAN_POINT('Ctrl Pts',(3.85216762263966,-1.,0.193642806777722));
#55304=CARTESIAN_POINT('Ctrl Pts',(3.84475203346977,-1.,0.19490900946022));
#55305=CARTESIAN_POINT('Ctrl Pts',(3.83743910616195,-1.,0.196115198971858));
#55306=CARTESIAN_POINT('Ctrl Pts',(3.83026221776456,-1.,0.197260935827361));
#55307=CARTESIAN_POINT('Ctrl Pts',(3.82321127349016,-1.,0.198342616900486));
#55308=CARTESIAN_POINT('Ctrl Pts',(3.81620203429815,-1.,0.199351525297447));
#55309=CARTESIAN_POINT('Ctrl Pts',(3.80909529318669,-1.,0.200274679433364));
#55310=CARTESIAN_POINT('Ctrl Pts',(3.80175247447337,-1.,0.201097756307325));
#55311=CARTESIAN_POINT('Ctrl Pts',(3.7940835418736,-1.,0.201807533800837));
#55312=CARTESIAN_POINT('Ctrl Pts',(3.78609175019242,-1.,0.20239426051216));
#55313=CARTESIAN_POINT('Ctrl Pts',(3.77793553476614,-1.,0.20285472969908));
#55314=CARTESIAN_POINT('Ctrl Pts',(3.7699207159487,-1.,0.203192390045164));
#55315=CARTESIAN_POINT('Ctrl Pts',(3.76242717936885,-1.,0.203414634707478));
#55316=CARTESIAN_POINT('Ctrl Pts',(3.75585118707734,-1.,0.203530796848321));
#55317=CARTESIAN_POINT('Ctrl Pts',(3.75054693397875,-1.,0.203550035479166));
#55318=CARTESIAN_POINT('Ctrl Pts',(3.74703926501752,-1.,0.203484186269415));
#55319=CARTESIAN_POINT('Ctrl Pts',(3.74535749969115,-1.,0.203375226874121));
#55320=CARTESIAN_POINT('Ctrl Pts',(3.74471097893845,-1.,0.20326661011053));
#55321=CARTESIAN_POINT('Ctrl Pts',(3.74453008995092,-1.,0.203188003946656));
#55322=CARTESIAN_POINT('Ctrl Pts',(3.74449296983004,-1.,0.2031560948961));
#55323=CARTESIAN_POINT('',(3.73017266276651,-1.,0.385112848330762));
#55324=CARTESIAN_POINT('Origin',(0.,-1.,0.));
#55325=CARTESIAN_POINT('',(4.15950947128175,-1.,0.581791163835816));
#55326=CARTESIAN_POINT('Ctrl Pts',(3.73017266276651,-1.,0.385112848330762));
#55327=CARTESIAN_POINT('Ctrl Pts',(3.73021431755274,-1.,0.385087139000375));
#55328=CARTESIAN_POINT('Ctrl Pts',(3.73040527621055,-1.,0.385037797881504));
#55329=CARTESIAN_POINT('Ctrl Pts',(3.73106082862548,-1.,0.385031656499164));
#55330=CARTESIAN_POINT('Ctrl Pts',(3.73273893363406,-1.,0.385187124634207));
#55331=CARTESIAN_POINT('Ctrl Pts',(3.73621371845318,-1.,0.385670806454566));
#55332=CARTESIAN_POINT('Ctrl Pts',(3.74144965781276,-1.,0.386519576222252));
#55333=CARTESIAN_POINT('Ctrl Pts',(3.74792651696654,-1.,0.387663020050836));
#55334=CARTESIAN_POINT('Ctrl Pts',(3.75529302895152,-1.,0.389054775898702));
#55335=CARTESIAN_POINT('Ctrl Pts',(3.76315635033257,-1.,0.39064207297956));
#55336=CARTESIAN_POINT('Ctrl Pts',(3.77114011595967,-1.,0.392372786223433));
#55337=CARTESIAN_POINT('Ctrl Pts',(3.77894173114283,-1.,0.3942024810115));
#55338=CARTESIAN_POINT('Ctrl Pts',(3.78640521279313,-1.,0.396103205334841));
#55339=CARTESIAN_POINT('Ctrl Pts',(3.7935288716329,-1.,0.39806481868397));
#55340=CARTESIAN_POINT('Ctrl Pts',(3.80040370384546,-1.,0.400088346504601));
#55341=CARTESIAN_POINT('Ctrl Pts',(3.80716881962728,-1.,0.402181320148436));
#55342=CARTESIAN_POINT('Ctrl Pts',(3.81396374287793,-1.,0.404352694628274));
#55343=CARTESIAN_POINT('Ctrl Pts',(3.8208730391381,-1.,0.406607038258986));
#55344=CARTESIAN_POINT('Ctrl Pts',(3.82790724256471,-1.,0.40894237144746));
#55345=CARTESIAN_POINT('Ctrl Pts',(3.83503345578698,-1.,0.411353038798519));
#55346=CARTESIAN_POINT('Ctrl Pts',(3.84219403994762,-1.,0.413831367016748));
#55347=CARTESIAN_POINT('Ctrl Pts',(3.84932864157497,-1.,0.416369678052907));
#55348=CARTESIAN_POINT('Ctrl Pts',(3.85639825647996,-1.,0.418962468086773));
#55349=CARTESIAN_POINT('Ctrl Pts',(3.86339652542709,-1.,0.421607423177534));
#55350=CARTESIAN_POINT('Ctrl Pts',(3.87033643487851,-1.,0.424304173195111));
#55351=CARTESIAN_POINT('Ctrl Pts',(3.87724240306597,-1.,0.427053541173458));
#55352=CARTESIAN_POINT('Ctrl Pts',(3.88414070943341,-1.,0.429856640579741));
#55353=CARTESIAN_POINT('Ctrl Pts',(3.89104947940611,-1.,0.432713929544459));
#55354=CARTESIAN_POINT('Ctrl Pts',(3.89797256655462,-1.,0.435624629433528));
#55355=CARTESIAN_POINT('Ctrl Pts',(3.90490512938563,-1.,0.43858723545825));
#55356=CARTESIAN_POINT('Ctrl Pts',(3.91183704069153,-1.,0.441599824524055));
#55357=CARTESIAN_POINT('Ctrl Pts',(3.91875701610719,-1.,0.444660430230591));
#55358=CARTESIAN_POINT('Ctrl Pts',(3.92565674143416,-1.,0.447767416837293));
#55359=CARTESIAN_POINT('Ctrl Pts',(3.93253407403123,-1.,0.450919768356349));
#55360=CARTESIAN_POINT('Ctrl Pts',(3.93939080846298,-1.,0.454116879027584));
#55361=CARTESIAN_POINT('Ctrl Pts',(3.94623117206678,-1.,0.457358410451683));
#55362=CARTESIAN_POINT('Ctrl Pts',(3.95306005817364,-1.,0.460644124429122));
#55363=CARTESIAN_POINT('Ctrl Pts',(3.95988133243538,-1.,0.463973722115734));
#55364=CARTESIAN_POINT('Ctrl Pts',(3.9666962227393,-1.,0.467346690880644));
#55365=CARTESIAN_POINT('Ctrl Pts',(3.97350414289392,-1.,0.47076237961344));
#55366=CARTESIAN_POINT('Ctrl Pts',(3.98030338044409,-1.,0.47422006101951));
#55367=CARTESIAN_POINT('Ctrl Pts',(3.98709184306738,-1.,0.477718999122028));
#55368=CARTESIAN_POINT('Ctrl Pts',(3.99386775880679,-1.,0.481258512209676));
#55369=CARTESIAN_POINT('Ctrl Pts',(4.00063045119288,-1.,0.484838042421835));
#55370=CARTESIAN_POINT('Ctrl Pts',(4.0073800839099,-1.,0.488457130424634));
#55371=CARTESIAN_POINT('Ctrl Pts',(4.01411733503546,-1.,0.492115383418019));
#55372=CARTESIAN_POINT('Ctrl Pts',(4.02084308851832,-1.,0.495812444326251));
#55373=CARTESIAN_POINT('Ctrl Pts',(4.02755813980101,-1.,0.499547962340822));
#55374=CARTESIAN_POINT('Ctrl Pts',(4.03426284174272,-1.,0.503321556915346));
#55375=CARTESIAN_POINT('Ctrl Pts',(4.04095715148915,-1.,0.507132823288137));
#55376=CARTESIAN_POINT('Ctrl Pts',(4.04764078815447,-1.,0.510981349218971));
#55377=CARTESIAN_POINT('Ctrl Pts',(4.05431335771199,-1.,0.514866728193017));
#55378=CARTESIAN_POINT('Ctrl Pts',(4.06097448038013,-1.,0.518788572336924));
#55379=CARTESIAN_POINT('Ctrl Pts',(4.06762394471314,-1.,0.522746528603108));
#55380=CARTESIAN_POINT('Ctrl Pts',(4.07426172299847,-1.,0.526740277227498));
#55381=CARTESIAN_POINT('Ctrl Pts',(4.08088789536836,-1.,0.530769518728571));
#55382=CARTESIAN_POINT('Ctrl Pts',(4.08750259988885,-1.,0.534833963477273));
#55383=CARTESIAN_POINT('Ctrl Pts',(4.09410597627,-1.,0.538933321179756));
#55384=CARTESIAN_POINT('Ctrl Pts',(4.10069810243979,-1.,0.543067286877758));
#55385=CARTESIAN_POINT('Ctrl Pts',(4.10727897027977,-1.,0.547235539485637));
#55386=CARTESIAN_POINT('Ctrl Pts',(4.11384852024721,-1.,0.551437758497033));
#55387=CARTESIAN_POINT('Ctrl Pts',(4.12040666195664,-1.,0.555673636129978));
#55388=CARTESIAN_POINT('Ctrl Pts',(4.12695329951961,-1.,0.559942890594774));
#55389=CARTESIAN_POINT('Ctrl Pts',(4.13348835727104,-1.,0.564245279537149));
#55390=CARTESIAN_POINT('Ctrl Pts',(4.14001179830547,-1.,0.568580610189775));
#55391=CARTESIAN_POINT('Ctrl Pts',(4.14652361068081,-1.,0.572948736069523));
#55392=CARTESIAN_POINT('Ctrl Pts',(4.151723761217,-1.,0.576469391676689));
#55393=CARTESIAN_POINT('Ctrl Pts',(4.15561864788576,-1.,0.579124568914236));
#55394=CARTESIAN_POINT('Ctrl Pts',(4.1582129171283,-1.,0.580901211463535));
#55395=CARTESIAN_POINT('Ctrl Pts',(4.15950947128175,-1.,0.581791163835816));
#55396=CARTESIAN_POINT('',(4.13571194405636,-1.,0.732042837400621));
#55397=CARTESIAN_POINT('',(4.15950947128175,-1.,0.581791163835816));
#55398=CARTESIAN_POINT('Ctrl Pts',(4.13571194405636,-1.,0.732042837400621));
#55399=CARTESIAN_POINT('Ctrl Pts',(4.1342038373684,-1.,0.73248857513516));
#55400=CARTESIAN_POINT('Ctrl Pts',(4.13118752795207,-1.,0.733376589323547));
#55401=CARTESIAN_POINT('Ctrl Pts',(4.12666277570844,-1.,0.734698226764093));
#55402=CARTESIAN_POINT('Ctrl Pts',(4.120629196238,-1.,0.736439634331345));
#55403=CARTESIAN_POINT('Ctrl Pts',(4.11308626951927,-1.,0.738581708225844));
#55404=CARTESIAN_POINT('Ctrl Pts',(4.10554241757547,-1.,0.740688998553377));
#55405=CARTESIAN_POINT('Ctrl Pts',(4.09799769702611,-1.,0.742761369689842));
#55406=CARTESIAN_POINT('Ctrl Pts',(4.09045220253573,-1.,0.744798649706501));
#55407=CARTESIAN_POINT('Ctrl Pts',(4.08290608095642,-1.,0.746800631492316));
#55408=CARTESIAN_POINT('Ctrl Pts',(4.07535951056152,-1.,0.748767076680558));
#55409=CARTESIAN_POINT('Ctrl Pts',(4.06781267242378,-1.,0.750697720484037));
#55410=CARTESIAN_POINT('Ctrl Pts',(4.06026572221515,-1.,0.752592276483073));
#55411=CARTESIAN_POINT('Ctrl Pts',(4.05271876687915,-1.,0.754450441816078));
#55412=CARTESIAN_POINT('Ctrl Pts',(4.04517182653997,-1.,0.756271902369581));
#55413=CARTESIAN_POINT('Ctrl Pts',(4.03762485803119,-1.,0.758056338884945));
#55414=CARTESIAN_POINT('Ctrl Pts',(4.03007781954412,-1.,0.759803433243752));
#55415=CARTESIAN_POINT('Ctrl Pts',(4.02253072741268,-1.,0.761512875859805));
#55416=CARTESIAN_POINT('Ctrl Pts',(4.01498370680496,-1.,0.763184371182936));
#55417=CARTESIAN_POINT('Ctrl Pts',(4.00743706791509,-1.,0.764817648785198));
#55418=CARTESIAN_POINT('Ctrl Pts',(3.99989129179622,-1.,0.766412457136064));
#55419=CARTESIAN_POINT('Ctrl Pts',(3.9923468788101,-1.,0.767968531377915));
#55420=CARTESIAN_POINT('Ctrl Pts',(3.98480422348451,-1.,0.769485566245545));
#55421=CARTESIAN_POINT('Ctrl Pts',(3.97726349165488,-1.,0.770963190030471));
#55422=CARTESIAN_POINT('Ctrl Pts',(3.96972446532772,-1.,0.772400931772137));
#55423=CARTESIAN_POINT('Ctrl Pts',(3.96218649639807,-1.,0.773798212026566));
#55424=CARTESIAN_POINT('Ctrl Pts',(3.9546488545231,-1.,0.775154418039352));
#55425=CARTESIAN_POINT('Ctrl Pts',(3.94711101619447,-1.,0.776468966697922));
#55426=CARTESIAN_POINT('Ctrl Pts',(3.93957296768103,-1.,0.777741370568559));
#55427=CARTESIAN_POINT('Ctrl Pts',(3.93203552473174,-1.,0.778971308134821));
#55428=CARTESIAN_POINT('Ctrl Pts',(3.92450058323823,-1.,0.780158678615543));
#55429=CARTESIAN_POINT('Ctrl Pts',(3.91697036054676,-1.,0.781303428618367));
#55430=CARTESIAN_POINT('Ctrl Pts',(3.90944671004542,-1.,0.782405395622765));
#55431=CARTESIAN_POINT('Ctrl Pts',(3.9019303904397,-1.,0.783464141529082));
#55432=CARTESIAN_POINT('Ctrl Pts',(3.89442039235103,-1.,0.784478799358337));
#55433=CARTESIAN_POINT('Ctrl Pts',(3.88691313167398,-1.,0.785447890340731));
#55434=CARTESIAN_POINT('Ctrl Pts',(3.8794040281819,-1.,0.786369675812609));
#55435=CARTESIAN_POINT('Ctrl Pts',(3.87188916600912,-1.,0.787242527617999));
#55436=CARTESIAN_POINT('Ctrl Pts',(3.86436702561345,-1.,0.788065315093778));
#55437=CARTESIAN_POINT('Ctrl Pts',(3.85683995872529,-1.,0.788837734090672));
#55438=CARTESIAN_POINT('Ctrl Pts',(3.84931637808894,-1.,0.789560798155583));
#55439=CARTESIAN_POINT('Ctrl Pts',(3.84180762342454,-1.,0.790236124191243));
#55440=CARTESIAN_POINT('Ctrl Pts',(3.83432392054786,-1.,0.790865012705301));
#55441=CARTESIAN_POINT('Ctrl Pts',(3.82687033899792,-1.,0.791447528662369));
#55442=CARTESIAN_POINT('Ctrl Pts',(3.81944345442249,-1.,0.791981740718635));
#55443=CARTESIAN_POINT('Ctrl Pts',(3.81202588694756,-1.,0.792462483517635));
#55444=CARTESIAN_POINT('Ctrl Pts',(3.80459229925637,-1.,0.792882695234778));
#55445=CARTESIAN_POINT('Ctrl Pts',(3.79711921389897,-1.,0.793235612973274));
#55446=CARTESIAN_POINT('Ctrl Pts',(3.78959439439235,-1.,0.793516871680994));
#55447=CARTESIAN_POINT('Ctrl Pts',(3.78202460377598,-1.,0.793726235781301));
#55448=CARTESIAN_POINT('Ctrl Pts',(3.77444863801212,-1.,0.793870523787408));
#55449=CARTESIAN_POINT('Ctrl Pts',(3.76692626931111,-1.,0.793961083688992));
#55450=CARTESIAN_POINT('Ctrl Pts',(3.75951468666257,-1.,0.794008429134908));
#55451=CARTESIAN_POINT('Ctrl Pts',(3.75224692493864,-1.,0.794017347371378));
#55452=CARTESIAN_POINT('Ctrl Pts',(3.74511357728861,-1.,0.793982700459952));
#55453=CARTESIAN_POINT('Ctrl Pts',(3.73803280541687,-1.,0.793882700937017));
#55454=CARTESIAN_POINT('Ctrl Pts',(3.73086914695805,-1.,0.793682750269684));
#55455=CARTESIAN_POINT('Ctrl Pts',(3.72348797293734,-1.,0.793347023784205));
#55456=CARTESIAN_POINT('Ctrl Pts',(3.71580242396124,-1.,0.792848377370287));
#55457=CARTESIAN_POINT('Ctrl Pts',(3.70781724021806,-1.,0.792177688845818));
#55458=CARTESIAN_POINT('Ctrl Pts',(3.69968940808721,-1.,0.79135657569598));
#55459=CARTESIAN_POINT('Ctrl Pts',(3.69172044327364,-1.,0.790436284988788));
#55460=CARTESIAN_POINT('Ctrl Pts',(3.68428439783905,-1.,0.789483546064387));
#55461=CARTESIAN_POINT('Ctrl Pts',(3.67777119516252,-1.,0.788569566220286));
#55462=CARTESIAN_POINT('Ctrl Pts',(3.67252923663655,-1.,0.787758799995743));
#55463=CARTESIAN_POINT('Ctrl Pts',(3.66907505398677,-1.,0.787145041181546));
#55464=CARTESIAN_POINT('Ctrl Pts',(3.66743103898702,-1.,0.786774337198063));
#55465=CARTESIAN_POINT('Ctrl Pts',(3.66680946938292,-1.,0.786565919558984));
#55466=CARTESIAN_POINT('Ctrl Pts',(3.6666431041522,-1.,0.786459983895432));
#55467=CARTESIAN_POINT('Ctrl Pts',(3.66661143271685,-1.,0.786422660831985));
#55468=CARTESIAN_POINT('Origin',(0.,-1.,0.));
#55469=CARTESIAN_POINT('Origin',(0.,0.,0.));
#55470=CARTESIAN_POINT('Origin',(0.,2.2,0.));
#55471=CARTESIAN_POINT('Origin',(0.,1.,0.));
#55472=CARTESIAN_POINT('',(-2.,2.2,2.44929359829471E-16));
#55473=CARTESIAN_POINT('Origin',(0.,2.2,0.));
#55474=CARTESIAN_POINT('',(-2.,1.,2.44929359829471E-16));
#55475=CARTESIAN_POINT('',(-2.,1.,2.44929359829471E-16));
#55476=CARTESIAN_POINT('Origin',(0.,1.,0.));
#55477=CARTESIAN_POINT('Origin',(0.,2.2,0.));
#55478=CARTESIAN_POINT('Ctrl Pts',(4.15950947128175,-1.,0.581791163835816));
#55479=CARTESIAN_POINT('Ctrl Pts',(4.15950947128175,1.,0.581791163835816));
#55480=CARTESIAN_POINT('Ctrl Pts',(4.1582129171283,-1.,0.580901211463535));
#55481=CARTESIAN_POINT('Ctrl Pts',(4.1582129171283,1.,0.580901211463535));
#55482=CARTESIAN_POINT('Ctrl Pts',(4.15561864788576,-1.,0.579124568914236));
#55483=CARTESIAN_POINT('Ctrl Pts',(4.15561864788576,1.,0.579124568914236));
#55484=CARTESIAN_POINT('Ctrl Pts',(4.151723761217,-1.,0.576469391676689));
#55485=CARTESIAN_POINT('Ctrl Pts',(4.151723761217,1.,0.576469391676689));
#55486=CARTESIAN_POINT('Ctrl Pts',(4.14652361068081,-1.,0.572948736069523));
#55487=CARTESIAN_POINT('Ctrl Pts',(4.14652361068081,1.,0.572948736069523));
#55488=CARTESIAN_POINT('Ctrl Pts',(4.14001179830547,-1.,0.568580610189775));
#55489=CARTESIAN_POINT('Ctrl Pts',(4.14001179830547,1.,0.568580610189775));
#55490=CARTESIAN_POINT('Ctrl Pts',(4.13348835727104,-1.,0.564245279537149));
#55491=CARTESIAN_POINT('Ctrl Pts',(4.13348835727104,1.,0.564245279537149));
#55492=CARTESIAN_POINT('Ctrl Pts',(4.12695329951961,-1.,0.559942890594774));
#55493=CARTESIAN_POINT('Ctrl Pts',(4.12695329951961,1.,0.559942890594774));
#55494=CARTESIAN_POINT('Ctrl Pts',(4.12040666195664,-1.,0.555673636129978));
#55495=CARTESIAN_POINT('Ctrl Pts',(4.12040666195664,1.,0.555673636129978));
#55496=CARTESIAN_POINT('Ctrl Pts',(4.11384852024721,-1.,0.551437758497033));
#55497=CARTESIAN_POINT('Ctrl Pts',(4.11384852024721,1.,0.551437758497033));
#55498=CARTESIAN_POINT('Ctrl Pts',(4.10727897027977,-1.,0.547235539485637));
#55499=CARTESIAN_POINT('Ctrl Pts',(4.10727897027977,1.,0.547235539485637));
#55500=CARTESIAN_POINT('Ctrl Pts',(4.10069810243979,-1.,0.543067286877758));
#55501=CARTESIAN_POINT('Ctrl Pts',(4.10069810243979,1.,0.543067286877758));
#55502=CARTESIAN_POINT('Ctrl Pts',(4.09410597627,-1.,0.538933321179756));
#55503=CARTESIAN_POINT('Ctrl Pts',(4.09410597627,1.,0.538933321179756));
#55504=CARTESIAN_POINT('Ctrl Pts',(4.08750259988885,-1.,0.534833963477273));
#55505=CARTESIAN_POINT('Ctrl Pts',(4.08750259988885,1.,0.534833963477273));
#55506=CARTESIAN_POINT('Ctrl Pts',(4.08088789536836,-1.,0.530769518728571));
#55507=CARTESIAN_POINT('Ctrl Pts',(4.08088789536836,1.,0.530769518728571));
#55508=CARTESIAN_POINT('Ctrl Pts',(4.07426172299847,-1.,0.526740277227498));
#55509=CARTESIAN_POINT('Ctrl Pts',(4.07426172299847,1.,0.526740277227498));
#55510=CARTESIAN_POINT('Ctrl Pts',(4.06762394471314,-1.,0.522746528603108));
#55511=CARTESIAN_POINT('Ctrl Pts',(4.06762394471314,1.,0.522746528603108));
#55512=CARTESIAN_POINT('Ctrl Pts',(4.06097448038013,-1.,0.518788572336924));
#55513=CARTESIAN_POINT('Ctrl Pts',(4.06097448038013,1.,0.518788572336924));
#55514=CARTESIAN_POINT('Ctrl Pts',(4.05431335771199,-1.,0.514866728193017));
#55515=CARTESIAN_POINT('Ctrl Pts',(4.05431335771199,1.,0.514866728193017));
#55516=CARTESIAN_POINT('Ctrl Pts',(4.04764078815447,-1.,0.510981349218971));
#55517=CARTESIAN_POINT('Ctrl Pts',(4.04764078815447,1.,0.510981349218971));
#55518=CARTESIAN_POINT('Ctrl Pts',(4.04095715148915,-1.,0.507132823288137));
#55519=CARTESIAN_POINT('Ctrl Pts',(4.04095715148915,1.,0.507132823288137));
#55520=CARTESIAN_POINT('Ctrl Pts',(4.03426284174272,-1.,0.503321556915346));
#55521=CARTESIAN_POINT('Ctrl Pts',(4.03426284174272,1.,0.503321556915346));
#55522=CARTESIAN_POINT('Ctrl Pts',(4.02755813980101,-1.,0.499547962340822));
#55523=CARTESIAN_POINT('Ctrl Pts',(4.02755813980101,1.,0.499547962340822));
#55524=CARTESIAN_POINT('Ctrl Pts',(4.02084308851832,-1.,0.495812444326251));
#55525=CARTESIAN_POINT('Ctrl Pts',(4.02084308851832,1.,0.495812444326251));
#55526=CARTESIAN_POINT('Ctrl Pts',(4.01411733503546,-1.,0.492115383418019));
#55527=CARTESIAN_POINT('Ctrl Pts',(4.01411733503546,1.,0.492115383418019));
#55528=CARTESIAN_POINT('Ctrl Pts',(4.0073800839099,-1.,0.488457130424634));
#55529=CARTESIAN_POINT('Ctrl Pts',(4.0073800839099,1.,0.488457130424634));
#55530=CARTESIAN_POINT('Ctrl Pts',(4.00063045119288,-1.,0.484838042421835));
#55531=CARTESIAN_POINT('Ctrl Pts',(4.00063045119288,1.,0.484838042421835));
#55532=CARTESIAN_POINT('Ctrl Pts',(3.99386775880679,-1.,0.481258512209676));
#55533=CARTESIAN_POINT('Ctrl Pts',(3.99386775880679,1.,0.481258512209676));
#55534=CARTESIAN_POINT('Ctrl Pts',(3.98709184306738,-1.,0.477718999122028));
#55535=CARTESIAN_POINT('Ctrl Pts',(3.98709184306738,1.,0.477718999122028));
#55536=CARTESIAN_POINT('Ctrl Pts',(3.98030338044409,-1.,0.47422006101951));
#55537=CARTESIAN_POINT('Ctrl Pts',(3.98030338044409,1.,0.47422006101951));
#55538=CARTESIAN_POINT('Ctrl Pts',(3.97350414289392,-1.,0.47076237961344));
#55539=CARTESIAN_POINT('Ctrl Pts',(3.97350414289392,1.,0.47076237961344));
#55540=CARTESIAN_POINT('Ctrl Pts',(3.9666962227393,-1.,0.467346690880644));
#55541=CARTESIAN_POINT('Ctrl Pts',(3.9666962227393,1.,0.467346690880644));
#55542=CARTESIAN_POINT('Ctrl Pts',(3.95988133243538,-1.,0.463973722115734));
#55543=CARTESIAN_POINT('Ctrl Pts',(3.95988133243538,1.,0.463973722115734));
#55544=CARTESIAN_POINT('Ctrl Pts',(3.95306005817364,-1.,0.460644124429122));
#55545=CARTESIAN_POINT('Ctrl Pts',(3.95306005817364,1.,0.460644124429122));
#55546=CARTESIAN_POINT('Ctrl Pts',(3.94623117206678,-1.,0.457358410451683));
#55547=CARTESIAN_POINT('Ctrl Pts',(3.94623117206678,1.,0.457358410451683));
#55548=CARTESIAN_POINT('Ctrl Pts',(3.93939080846298,-1.,0.454116879027584));
#55549=CARTESIAN_POINT('Ctrl Pts',(3.93939080846298,1.,0.454116879027584));
#55550=CARTESIAN_POINT('Ctrl Pts',(3.93253407403123,-1.,0.450919768356349));
#55551=CARTESIAN_POINT('Ctrl Pts',(3.93253407403123,1.,0.450919768356349));
#55552=CARTESIAN_POINT('Ctrl Pts',(3.92565674143416,-1.,0.447767416837293));
#55553=CARTESIAN_POINT('Ctrl Pts',(3.92565674143416,1.,0.447767416837293));
#55554=CARTESIAN_POINT('Ctrl Pts',(3.91875701610719,-1.,0.444660430230591));
#55555=CARTESIAN_POINT('Ctrl Pts',(3.91875701610719,1.,0.444660430230591));
#55556=CARTESIAN_POINT('Ctrl Pts',(3.91183704069153,-1.,0.441599824524055));
#55557=CARTESIAN_POINT('Ctrl Pts',(3.91183704069153,1.,0.441599824524055));
#55558=CARTESIAN_POINT('Ctrl Pts',(3.90490512938563,-1.,0.43858723545825));
#55559=CARTESIAN_POINT('Ctrl Pts',(3.90490512938563,1.,0.43858723545825));
#55560=CARTESIAN_POINT('Ctrl Pts',(3.89797256655462,-1.,0.435624629433528));
#55561=CARTESIAN_POINT('Ctrl Pts',(3.89797256655462,1.,0.435624629433528));
#55562=CARTESIAN_POINT('Ctrl Pts',(3.89104947940611,-1.,0.432713929544459));
#55563=CARTESIAN_POINT('Ctrl Pts',(3.89104947940611,1.,0.432713929544459));
#55564=CARTESIAN_POINT('Ctrl Pts',(3.88414070943341,-1.,0.429856640579741));
#55565=CARTESIAN_POINT('Ctrl Pts',(3.88414070943341,1.,0.429856640579741));
#55566=CARTESIAN_POINT('Ctrl Pts',(3.87724240306597,-1.,0.427053541173458));
#55567=CARTESIAN_POINT('Ctrl Pts',(3.87724240306597,1.,0.427053541173458));
#55568=CARTESIAN_POINT('Ctrl Pts',(3.87033643487851,-1.,0.424304173195111));
#55569=CARTESIAN_POINT('Ctrl Pts',(3.87033643487851,1.,0.424304173195111));
#55570=CARTESIAN_POINT('Ctrl Pts',(3.86339652542709,-1.,0.421607423177534));
#55571=CARTESIAN_POINT('Ctrl Pts',(3.86339652542709,1.,0.421607423177534));
#55572=CARTESIAN_POINT('Ctrl Pts',(3.85639825647996,-1.,0.418962468086773));
#55573=CARTESIAN_POINT('Ctrl Pts',(3.85639825647996,1.,0.418962468086773));
#55574=CARTESIAN_POINT('Ctrl Pts',(3.84932864157497,-1.,0.416369678052907));
#55575=CARTESIAN_POINT('Ctrl Pts',(3.84932864157497,1.,0.416369678052907));
#55576=CARTESIAN_POINT('Ctrl Pts',(3.84219403994762,-1.,0.413831367016748));
#55577=CARTESIAN_POINT('Ctrl Pts',(3.84219403994762,1.,0.413831367016748));
#55578=CARTESIAN_POINT('Ctrl Pts',(3.83503345578698,-1.,0.411353038798519));
#55579=CARTESIAN_POINT('Ctrl Pts',(3.83503345578698,1.,0.411353038798519));
#55580=CARTESIAN_POINT('Ctrl Pts',(3.82790724256471,-1.,0.40894237144746));
#55581=CARTESIAN_POINT('Ctrl Pts',(3.82790724256471,1.,0.40894237144746));
#55582=CARTESIAN_POINT('Ctrl Pts',(3.8208730391381,-1.,0.406607038258986));
#55583=CARTESIAN_POINT('Ctrl Pts',(3.8208730391381,1.,0.406607038258986));
#55584=CARTESIAN_POINT('Ctrl Pts',(3.81396374287793,-1.,0.404352694628274));
#55585=CARTESIAN_POINT('Ctrl Pts',(3.81396374287793,1.,0.404352694628274));
#55586=CARTESIAN_POINT('Ctrl Pts',(3.80716881962728,-1.,0.402181320148436));
#55587=CARTESIAN_POINT('Ctrl Pts',(3.80716881962728,1.,0.402181320148436));
#55588=CARTESIAN_POINT('Ctrl Pts',(3.80040370384546,-1.,0.400088346504601));
#55589=CARTESIAN_POINT('Ctrl Pts',(3.80040370384546,1.,0.400088346504601));
#55590=CARTESIAN_POINT('Ctrl Pts',(3.7935288716329,-1.,0.39806481868397));
#55591=CARTESIAN_POINT('Ctrl Pts',(3.7935288716329,1.,0.39806481868397));
#55592=CARTESIAN_POINT('Ctrl Pts',(3.78640521279313,-1.,0.396103205334841));
#55593=CARTESIAN_POINT('Ctrl Pts',(3.78640521279313,1.,0.396103205334841));
#55594=CARTESIAN_POINT('Ctrl Pts',(3.77894173114283,-1.,0.3942024810115));
#55595=CARTESIAN_POINT('Ctrl Pts',(3.77894173114283,1.,0.3942024810115));
#55596=CARTESIAN_POINT('Ctrl Pts',(3.77114011595967,-1.,0.392372786223433));
#55597=CARTESIAN_POINT('Ctrl Pts',(3.77114011595967,1.,0.392372786223433));
#55598=CARTESIAN_POINT('Ctrl Pts',(3.76315635033257,-1.,0.39064207297956));
#55599=CARTESIAN_POINT('Ctrl Pts',(3.76315635033257,1.,0.39064207297956));
#55600=CARTESIAN_POINT('Ctrl Pts',(3.75529302895152,-1.,0.389054775898702));
#55601=CARTESIAN_POINT('Ctrl Pts',(3.75529302895152,1.,0.389054775898702));
#55602=CARTESIAN_POINT('Ctrl Pts',(3.74792651696654,-1.,0.387663020050836));
#55603=CARTESIAN_POINT('Ctrl Pts',(3.74792651696654,1.,0.387663020050836));
#55604=CARTESIAN_POINT('Ctrl Pts',(3.74144965781276,-1.,0.386519576222252));
#55605=CARTESIAN_POINT('Ctrl Pts',(3.74144965781276,1.,0.386519576222252));
#55606=CARTESIAN_POINT('Ctrl Pts',(3.73621371845318,-1.,0.385670806454566));
#55607=CARTESIAN_POINT('Ctrl Pts',(3.73621371845318,1.,0.385670806454566));
#55608=CARTESIAN_POINT('Ctrl Pts',(3.73245705638843,-1.,0.385147887988952));
#55609=CARTESIAN_POINT('Ctrl Pts',(3.73245705638843,1.,0.385147887988952));
#55610=CARTESIAN_POINT('Ctrl Pts',(3.73072465900175,-1.,0.385001870183213));
#55611=CARTESIAN_POINT('Ctrl Pts',(3.73072465900175,1.,0.385001870183213));
#55612=CARTESIAN_POINT('Ctrl Pts',(3.73015851028356,-1.,0.385047711603463));
#55613=CARTESIAN_POINT('Ctrl Pts',(3.73015851028356,1.,0.385047711603463));
#55614=CARTESIAN_POINT('Ctrl Pts',(3.73010668803042,-1.,0.385147278814643));
#55615=CARTESIAN_POINT('Ctrl Pts',(3.73010668803042,1.,0.385147278814643));
#55616=CARTESIAN_POINT('Ctrl Pts',(3.73016218570874,-1.,0.38521431477633));
#55617=CARTESIAN_POINT('Ctrl Pts',(3.73016218570874,1.,0.38521431477633));
#55618=CARTESIAN_POINT('',(3.73017266276651,1.,0.385112848330762));
#55619=CARTESIAN_POINT('Ctrl Pts',(3.73017266276651,1.,0.385112848330762));
#55620=CARTESIAN_POINT('Ctrl Pts',(3.73017266276651,0.666666666666667,0.385112848330762));
#55621=CARTESIAN_POINT('Ctrl Pts',(3.73017266276651,0.333333333333333,0.385112848330762));
#55622=CARTESIAN_POINT('Ctrl Pts',(3.73017266276651,-0.333333333333333,
0.385112848330762));
#55623=CARTESIAN_POINT('Ctrl Pts',(3.73017266276651,-0.666666666666667,
0.385112848330763));
#55624=CARTESIAN_POINT('Ctrl Pts',(3.73017266276651,-1.,0.385112848330763));
#55625=CARTESIAN_POINT('',(4.15950947128175,1.,0.581791163835816));
#55626=CARTESIAN_POINT('Ctrl Pts',(4.15950947128175,1.,0.581791163835816));
#55627=CARTESIAN_POINT('Ctrl Pts',(4.1582129171283,1.,0.580901211463535));
#55628=CARTESIAN_POINT('Ctrl Pts',(4.15561864788576,1.,0.579124568914236));
#55629=CARTESIAN_POINT('Ctrl Pts',(4.151723761217,1.,0.576469391676689));
#55630=CARTESIAN_POINT('Ctrl Pts',(4.14652361068081,1.,0.572948736069523));
#55631=CARTESIAN_POINT('Ctrl Pts',(4.14001179830547,1.,0.568580610189775));
#55632=CARTESIAN_POINT('Ctrl Pts',(4.13348835727104,1.,0.564245279537149));
#55633=CARTESIAN_POINT('Ctrl Pts',(4.12695329951961,1.,0.559942890594774));
#55634=CARTESIAN_POINT('Ctrl Pts',(4.12040666195664,1.,0.555673636129978));
#55635=CARTESIAN_POINT('Ctrl Pts',(4.11384852024721,1.,0.551437758497033));
#55636=CARTESIAN_POINT('Ctrl Pts',(4.10727897027977,1.,0.547235539485637));
#55637=CARTESIAN_POINT('Ctrl Pts',(4.10069810243979,1.,0.543067286877758));
#55638=CARTESIAN_POINT('Ctrl Pts',(4.09410597627,1.,0.538933321179756));
#55639=CARTESIAN_POINT('Ctrl Pts',(4.08750259988885,1.,0.534833963477273));
#55640=CARTESIAN_POINT('Ctrl Pts',(4.08088789536836,1.,0.530769518728571));
#55641=CARTESIAN_POINT('Ctrl Pts',(4.07426172299847,1.,0.526740277227498));
#55642=CARTESIAN_POINT('Ctrl Pts',(4.06762394471314,1.,0.522746528603108));
#55643=CARTESIAN_POINT('Ctrl Pts',(4.06097448038013,1.,0.518788572336924));
#55644=CARTESIAN_POINT('Ctrl Pts',(4.05431335771199,1.,0.514866728193017));
#55645=CARTESIAN_POINT('Ctrl Pts',(4.04764078815447,1.,0.510981349218971));
#55646=CARTESIAN_POINT('Ctrl Pts',(4.04095715148915,1.,0.507132823288137));
#55647=CARTESIAN_POINT('Ctrl Pts',(4.03426284174272,1.,0.503321556915346));
#55648=CARTESIAN_POINT('Ctrl Pts',(4.02755813980101,1.,0.499547962340822));
#55649=CARTESIAN_POINT('Ctrl Pts',(4.02084308851832,1.,0.495812444326251));
#55650=CARTESIAN_POINT('Ctrl Pts',(4.01411733503546,1.,0.492115383418019));
#55651=CARTESIAN_POINT('Ctrl Pts',(4.0073800839099,1.,0.488457130424634));
#55652=CARTESIAN_POINT('Ctrl Pts',(4.00063045119288,1.,0.484838042421835));
#55653=CARTESIAN_POINT('Ctrl Pts',(3.99386775880679,1.,0.481258512209676));
#55654=CARTESIAN_POINT('Ctrl Pts',(3.98709184306738,1.,0.477718999122028));
#55655=CARTESIAN_POINT('Ctrl Pts',(3.98030338044409,1.,0.47422006101951));
#55656=CARTESIAN_POINT('Ctrl Pts',(3.97350414289392,1.,0.47076237961344));
#55657=CARTESIAN_POINT('Ctrl Pts',(3.9666962227393,1.,0.467346690880644));
#55658=CARTESIAN_POINT('Ctrl Pts',(3.95988133243538,1.,0.463973722115734));
#55659=CARTESIAN_POINT('Ctrl Pts',(3.95306005817364,1.,0.460644124429122));
#55660=CARTESIAN_POINT('Ctrl Pts',(3.94623117206678,1.,0.457358410451683));
#55661=CARTESIAN_POINT('Ctrl Pts',(3.93939080846298,1.,0.454116879027584));
#55662=CARTESIAN_POINT('Ctrl Pts',(3.93253407403123,1.,0.450919768356349));
#55663=CARTESIAN_POINT('Ctrl Pts',(3.92565674143416,1.,0.447767416837293));
#55664=CARTESIAN_POINT('Ctrl Pts',(3.91875701610719,1.,0.444660430230591));
#55665=CARTESIAN_POINT('Ctrl Pts',(3.91183704069153,1.,0.441599824524055));
#55666=CARTESIAN_POINT('Ctrl Pts',(3.90490512938563,1.,0.43858723545825));
#55667=CARTESIAN_POINT('Ctrl Pts',(3.89797256655462,1.,0.435624629433528));
#55668=CARTESIAN_POINT('Ctrl Pts',(3.89104947940611,1.,0.432713929544459));
#55669=CARTESIAN_POINT('Ctrl Pts',(3.88414070943341,1.,0.429856640579741));
#55670=CARTESIAN_POINT('Ctrl Pts',(3.87724240306597,1.,0.427053541173458));
#55671=CARTESIAN_POINT('Ctrl Pts',(3.87033643487851,1.,0.424304173195111));
#55672=CARTESIAN_POINT('Ctrl Pts',(3.86339652542709,1.,0.421607423177534));
#55673=CARTESIAN_POINT('Ctrl Pts',(3.85639825647996,1.,0.418962468086773));
#55674=CARTESIAN_POINT('Ctrl Pts',(3.84932864157497,1.,0.416369678052907));
#55675=CARTESIAN_POINT('Ctrl Pts',(3.84219403994762,1.,0.413831367016748));
#55676=CARTESIAN_POINT('Ctrl Pts',(3.83503345578698,1.,0.411353038798519));
#55677=CARTESIAN_POINT('Ctrl Pts',(3.82790724256471,1.,0.40894237144746));
#55678=CARTESIAN_POINT('Ctrl Pts',(3.8208730391381,1.,0.406607038258986));
#55679=CARTESIAN_POINT('Ctrl Pts',(3.81396374287793,1.,0.404352694628274));
#55680=CARTESIAN_POINT('Ctrl Pts',(3.80716881962728,1.,0.402181320148436));
#55681=CARTESIAN_POINT('Ctrl Pts',(3.80040370384546,1.,0.400088346504601));
#55682=CARTESIAN_POINT('Ctrl Pts',(3.7935288716329,1.,0.39806481868397));
#55683=CARTESIAN_POINT('Ctrl Pts',(3.78640521279313,1.,0.396103205334841));
#55684=CARTESIAN_POINT('Ctrl Pts',(3.77894173114283,1.,0.3942024810115));
#55685=CARTESIAN_POINT('Ctrl Pts',(3.77114011595967,1.,0.392372786223433));
#55686=CARTESIAN_POINT('Ctrl Pts',(3.76315635033257,1.,0.39064207297956));
#55687=CARTESIAN_POINT('Ctrl Pts',(3.75529302895152,1.,0.389054775898702));
#55688=CARTESIAN_POINT('Ctrl Pts',(3.74792651696654,1.,0.387663020050836));
#55689=CARTESIAN_POINT('Ctrl Pts',(3.74144965781276,1.,0.386519576222252));
#55690=CARTESIAN_POINT('Ctrl Pts',(3.73621371845318,1.,0.385670806454566));
#55691=CARTESIAN_POINT('Ctrl Pts',(3.73273893363406,1.,0.385187124634207));
#55692=CARTESIAN_POINT('Ctrl Pts',(3.73106082862548,1.,0.385031656499164));
#55693=CARTESIAN_POINT('Ctrl Pts',(3.73040527621055,1.,0.385037797881504));
#55694=CARTESIAN_POINT('Ctrl Pts',(3.73021431755274,1.,0.385087139000375));
#55695=CARTESIAN_POINT('Ctrl Pts',(3.73017266276651,1.,0.385112848330762));
#55696=CARTESIAN_POINT('',(4.15950947128175,0.,0.581791163835816));
#55697=CARTESIAN_POINT('Ctrl Pts',(3.66663282329846,-1.,0.7863229229206));
#55698=CARTESIAN_POINT('Ctrl Pts',(3.66663282329846,1.,0.7863229229206));
#55699=CARTESIAN_POINT('Ctrl Pts',(3.66655932661986,-1.,0.786369528183326));
#55700=CARTESIAN_POINT('Ctrl Pts',(3.66655932661986,1.,0.786369528183326));
#55701=CARTESIAN_POINT('Ctrl Pts',(3.66657784455334,-1.,0.786480236185697));
#55702=CARTESIAN_POINT('Ctrl Pts',(3.66657784455334,1.,0.786480236185697));
#55703=CARTESIAN_POINT('Ctrl Pts',(3.66710211820482,-1.,0.786698783542764));
#55704=CARTESIAN_POINT('Ctrl Pts',(3.66710211820482,1.,0.786698783542764));
#55705=CARTESIAN_POINT('Ctrl Pts',(3.66879484801113,-1.,0.787095252590501));
#55706=CARTESIAN_POINT('Ctrl Pts',(3.66879484801113,1.,0.787095252590501));
#55707=CARTESIAN_POINT('Ctrl Pts',(3.67252923663655,-1.,0.787758799995743));
#55708=CARTESIAN_POINT('Ctrl Pts',(3.67252923663655,1.,0.787758799995743));
#55709=CARTESIAN_POINT('Ctrl Pts',(3.67777119516252,-1.,0.788569566220286));
#55710=CARTESIAN_POINT('Ctrl Pts',(3.67777119516252,1.,0.788569566220286));
#55711=CARTESIAN_POINT('Ctrl Pts',(3.68428439783905,-1.,0.789483546064387));
#55712=CARTESIAN_POINT('Ctrl Pts',(3.68428439783905,1.,0.789483546064387));
#55713=CARTESIAN_POINT('Ctrl Pts',(3.69172044327364,-1.,0.790436284988788));
#55714=CARTESIAN_POINT('Ctrl Pts',(3.69172044327364,1.,0.790436284988788));
#55715=CARTESIAN_POINT('Ctrl Pts',(3.69968940808721,-1.,0.79135657569598));
#55716=CARTESIAN_POINT('Ctrl Pts',(3.69968940808721,1.,0.79135657569598));
#55717=CARTESIAN_POINT('Ctrl Pts',(3.70781724021806,-1.,0.792177688845818));
#55718=CARTESIAN_POINT('Ctrl Pts',(3.70781724021806,1.,0.792177688845818));
#55719=CARTESIAN_POINT('Ctrl Pts',(3.71580242396124,-1.,0.792848377370287));
#55720=CARTESIAN_POINT('Ctrl Pts',(3.71580242396124,1.,0.792848377370287));
#55721=CARTESIAN_POINT('Ctrl Pts',(3.72348797293734,-1.,0.793347023784205));
#55722=CARTESIAN_POINT('Ctrl Pts',(3.72348797293734,1.,0.793347023784205));
#55723=CARTESIAN_POINT('Ctrl Pts',(3.73086914695805,-1.,0.793682750269684));
#55724=CARTESIAN_POINT('Ctrl Pts',(3.73086914695805,1.,0.793682750269684));
#55725=CARTESIAN_POINT('Ctrl Pts',(3.73803280541687,-1.,0.793882700937017));
#55726=CARTESIAN_POINT('Ctrl Pts',(3.73803280541687,1.,0.793882700937017));
#55727=CARTESIAN_POINT('Ctrl Pts',(3.74511357728861,-1.,0.793982700459952));
#55728=CARTESIAN_POINT('Ctrl Pts',(3.74511357728861,1.,0.793982700459952));
#55729=CARTESIAN_POINT('Ctrl Pts',(3.75224692493864,-1.,0.794017347371378));
#55730=CARTESIAN_POINT('Ctrl Pts',(3.75224692493864,1.,0.794017347371378));
#55731=CARTESIAN_POINT('Ctrl Pts',(3.75951468666257,-1.,0.794008429134908));
#55732=CARTESIAN_POINT('Ctrl Pts',(3.75951468666257,1.,0.794008429134908));
#55733=CARTESIAN_POINT('Ctrl Pts',(3.76692626931111,-1.,0.793961083688992));
#55734=CARTESIAN_POINT('Ctrl Pts',(3.76692626931111,1.,0.793961083688992));
#55735=CARTESIAN_POINT('Ctrl Pts',(3.77444863801212,-1.,0.793870523787408));
#55736=CARTESIAN_POINT('Ctrl Pts',(3.77444863801212,1.,0.793870523787408));
#55737=CARTESIAN_POINT('Ctrl Pts',(3.78202460377598,-1.,0.793726235781301));
#55738=CARTESIAN_POINT('Ctrl Pts',(3.78202460377598,1.,0.793726235781301));
#55739=CARTESIAN_POINT('Ctrl Pts',(3.78959439439235,-1.,0.793516871680994));
#55740=CARTESIAN_POINT('Ctrl Pts',(3.78959439439235,1.,0.793516871680994));
#55741=CARTESIAN_POINT('Ctrl Pts',(3.79711921389897,-1.,0.793235612973274));
#55742=CARTESIAN_POINT('Ctrl Pts',(3.79711921389897,1.,0.793235612973274));
#55743=CARTESIAN_POINT('Ctrl Pts',(3.80459229925637,-1.,0.792882695234778));
#55744=CARTESIAN_POINT('Ctrl Pts',(3.80459229925637,1.,0.792882695234778));
#55745=CARTESIAN_POINT('Ctrl Pts',(3.81202588694756,-1.,0.792462483517635));
#55746=CARTESIAN_POINT('Ctrl Pts',(3.81202588694756,1.,0.792462483517635));
#55747=CARTESIAN_POINT('Ctrl Pts',(3.81944345442249,-1.,0.791981740718635));
#55748=CARTESIAN_POINT('Ctrl Pts',(3.81944345442249,1.,0.791981740718635));
#55749=CARTESIAN_POINT('Ctrl Pts',(3.82687033899792,-1.,0.791447528662369));
#55750=CARTESIAN_POINT('Ctrl Pts',(3.82687033899792,1.,0.791447528662369));
#55751=CARTESIAN_POINT('Ctrl Pts',(3.83432392054786,-1.,0.790865012705301));
#55752=CARTESIAN_POINT('Ctrl Pts',(3.83432392054786,1.,0.790865012705301));
#55753=CARTESIAN_POINT('Ctrl Pts',(3.84180762342454,-1.,0.790236124191243));
#55754=CARTESIAN_POINT('Ctrl Pts',(3.84180762342454,1.,0.790236124191243));
#55755=CARTESIAN_POINT('Ctrl Pts',(3.84931637808894,-1.,0.789560798155583));
#55756=CARTESIAN_POINT('Ctrl Pts',(3.84931637808894,1.,0.789560798155583));
#55757=CARTESIAN_POINT('Ctrl Pts',(3.85683995872529,-1.,0.788837734090672));
#55758=CARTESIAN_POINT('Ctrl Pts',(3.85683995872529,1.,0.788837734090672));
#55759=CARTESIAN_POINT('Ctrl Pts',(3.86436702561345,-1.,0.788065315093778));
#55760=CARTESIAN_POINT('Ctrl Pts',(3.86436702561345,1.,0.788065315093778));
#55761=CARTESIAN_POINT('Ctrl Pts',(3.87188916600912,-1.,0.787242527617999));
#55762=CARTESIAN_POINT('Ctrl Pts',(3.87188916600912,1.,0.787242527617999));
#55763=CARTESIAN_POINT('Ctrl Pts',(3.8794040281819,-1.,0.786369675812609));
#55764=CARTESIAN_POINT('Ctrl Pts',(3.8794040281819,1.,0.786369675812609));
#55765=CARTESIAN_POINT('Ctrl Pts',(3.88691313167398,-1.,0.785447890340731));
#55766=CARTESIAN_POINT('Ctrl Pts',(3.88691313167398,1.,0.785447890340731));
#55767=CARTESIAN_POINT('Ctrl Pts',(3.89442039235103,-1.,0.784478799358337));
#55768=CARTESIAN_POINT('Ctrl Pts',(3.89442039235103,1.,0.784478799358337));
#55769=CARTESIAN_POINT('Ctrl Pts',(3.9019303904397,-1.,0.783464141529082));
#55770=CARTESIAN_POINT('Ctrl Pts',(3.9019303904397,1.,0.783464141529082));
#55771=CARTESIAN_POINT('Ctrl Pts',(3.90944671004542,-1.,0.782405395622765));
#55772=CARTESIAN_POINT('Ctrl Pts',(3.90944671004542,1.,0.782405395622765));
#55773=CARTESIAN_POINT('Ctrl Pts',(3.91697036054676,-1.,0.781303428618367));
#55774=CARTESIAN_POINT('Ctrl Pts',(3.91697036054676,1.,0.781303428618367));
#55775=CARTESIAN_POINT('Ctrl Pts',(3.92450058323823,-1.,0.780158678615543));
#55776=CARTESIAN_POINT('Ctrl Pts',(3.92450058323823,1.,0.780158678615543));
#55777=CARTESIAN_POINT('Ctrl Pts',(3.93203552473174,-1.,0.778971308134821));
#55778=CARTESIAN_POINT('Ctrl Pts',(3.93203552473174,1.,0.778971308134821));
#55779=CARTESIAN_POINT('Ctrl Pts',(3.93957296768103,-1.,0.777741370568559));
#55780=CARTESIAN_POINT('Ctrl Pts',(3.93957296768103,1.,0.777741370568559));
#55781=CARTESIAN_POINT('Ctrl Pts',(3.94711101619447,-1.,0.776468966697922));
#55782=CARTESIAN_POINT('Ctrl Pts',(3.94711101619447,1.,0.776468966697922));
#55783=CARTESIAN_POINT('Ctrl Pts',(3.9546488545231,-1.,0.775154418039352));
#55784=CARTESIAN_POINT('Ctrl Pts',(3.9546488545231,1.,0.775154418039352));
#55785=CARTESIAN_POINT('Ctrl Pts',(3.96218649639807,-1.,0.773798212026566));
#55786=CARTESIAN_POINT('Ctrl Pts',(3.96218649639807,1.,0.773798212026566));
#55787=CARTESIAN_POINT('Ctrl Pts',(3.96972446532772,-1.,0.772400931772137));
#55788=CARTESIAN_POINT('Ctrl Pts',(3.96972446532772,1.,0.772400931772137));
#55789=CARTESIAN_POINT('Ctrl Pts',(3.97726349165488,-1.,0.770963190030471));
#55790=CARTESIAN_POINT('Ctrl Pts',(3.97726349165488,1.,0.770963190030471));
#55791=CARTESIAN_POINT('Ctrl Pts',(3.98480422348451,-1.,0.769485566245545));
#55792=CARTESIAN_POINT('Ctrl Pts',(3.98480422348451,1.,0.769485566245545));
#55793=CARTESIAN_POINT('Ctrl Pts',(3.9923468788101,-1.,0.767968531377915));
#55794=CARTESIAN_POINT('Ctrl Pts',(3.9923468788101,1.,0.767968531377915));
#55795=CARTESIAN_POINT('Ctrl Pts',(3.99989129179622,-1.,0.766412457136064));
#55796=CARTESIAN_POINT('Ctrl Pts',(3.99989129179622,1.,0.766412457136064));
#55797=CARTESIAN_POINT('Ctrl Pts',(4.00743706791509,-1.,0.764817648785198));
#55798=CARTESIAN_POINT('Ctrl Pts',(4.00743706791509,1.,0.764817648785198));
#55799=CARTESIAN_POINT('Ctrl Pts',(4.01498370680496,-1.,0.763184371182936));
#55800=CARTESIAN_POINT('Ctrl Pts',(4.01498370680496,1.,0.763184371182936));
#55801=CARTESIAN_POINT('Ctrl Pts',(4.02253072741268,-1.,0.761512875859805));
#55802=CARTESIAN_POINT('Ctrl Pts',(4.02253072741268,1.,0.761512875859805));
#55803=CARTESIAN_POINT('Ctrl Pts',(4.03007781954412,-1.,0.759803433243752));
#55804=CARTESIAN_POINT('Ctrl Pts',(4.03007781954412,1.,0.759803433243752));
#55805=CARTESIAN_POINT('Ctrl Pts',(4.03762485803119,-1.,0.758056338884945));
#55806=CARTESIAN_POINT('Ctrl Pts',(4.03762485803119,1.,0.758056338884945));
#55807=CARTESIAN_POINT('Ctrl Pts',(4.04517182653997,-1.,0.756271902369581));
#55808=CARTESIAN_POINT('Ctrl Pts',(4.04517182653997,1.,0.756271902369581));
#55809=CARTESIAN_POINT('Ctrl Pts',(4.05271876687915,-1.,0.754450441816078));
#55810=CARTESIAN_POINT('Ctrl Pts',(4.05271876687915,1.,0.754450441816078));
#55811=CARTESIAN_POINT('Ctrl Pts',(4.06026572221515,-1.,0.752592276483073));
#55812=CARTESIAN_POINT('Ctrl Pts',(4.06026572221515,1.,0.752592276483073));
#55813=CARTESIAN_POINT('Ctrl Pts',(4.06781267242378,-1.,0.750697720484037));
#55814=CARTESIAN_POINT('Ctrl Pts',(4.06781267242378,1.,0.750697720484037));
#55815=CARTESIAN_POINT('Ctrl Pts',(4.07535951056152,-1.,0.748767076680558));
#55816=CARTESIAN_POINT('Ctrl Pts',(4.07535951056152,1.,0.748767076680558));
#55817=CARTESIAN_POINT('Ctrl Pts',(4.08290608095642,-1.,0.746800631492316));
#55818=CARTESIAN_POINT('Ctrl Pts',(4.08290608095642,1.,0.746800631492316));
#55819=CARTESIAN_POINT('Ctrl Pts',(4.09045220253573,-1.,0.744798649706501));
#55820=CARTESIAN_POINT('Ctrl Pts',(4.09045220253573,1.,0.744798649706501));
#55821=CARTESIAN_POINT('Ctrl Pts',(4.09799769702611,-1.,0.742761369689842));
#55822=CARTESIAN_POINT('Ctrl Pts',(4.09799769702611,1.,0.742761369689842));
#55823=CARTESIAN_POINT('Ctrl Pts',(4.10554241757547,-1.,0.740688998553377));
#55824=CARTESIAN_POINT('Ctrl Pts',(4.10554241757547,1.,0.740688998553377));
#55825=CARTESIAN_POINT('Ctrl Pts',(4.11308626951927,-1.,0.738581708225844));
#55826=CARTESIAN_POINT('Ctrl Pts',(4.11308626951927,1.,0.738581708225844));
#55827=CARTESIAN_POINT('Ctrl Pts',(4.120629196238,-1.,0.736439634331345));
#55828=CARTESIAN_POINT('Ctrl Pts',(4.120629196238,1.,0.736439634331345));
#55829=CARTESIAN_POINT('Ctrl Pts',(4.12666277570844,-1.,0.734698226764093));
#55830=CARTESIAN_POINT('Ctrl Pts',(4.12666277570844,1.,0.734698226764093));
#55831=CARTESIAN_POINT('Ctrl Pts',(4.13118752795207,-1.,0.733376589323547));
#55832=CARTESIAN_POINT('Ctrl Pts',(4.13118752795207,1.,0.733376589323547));
#55833=CARTESIAN_POINT('Ctrl Pts',(4.1342038373684,-1.,0.73248857513516));
#55834=CARTESIAN_POINT('Ctrl Pts',(4.1342038373684,1.,0.73248857513516));
#55835=CARTESIAN_POINT('Ctrl Pts',(4.13571194405636,-1.,0.732042837400621));
#55836=CARTESIAN_POINT('Ctrl Pts',(4.13571194405636,1.,0.732042837400621));
#55837=CARTESIAN_POINT('',(3.66661143271685,1.,0.786422660831985));
#55838=CARTESIAN_POINT('Ctrl Pts',(3.66661143271685,-1.,0.786422660831986));
#55839=CARTESIAN_POINT('Ctrl Pts',(3.66661143271685,-0.666666666666667,
0.786422660831986));
#55840=CARTESIAN_POINT('Ctrl Pts',(3.66661143271685,-0.333333333333333,
0.786422660831986));
#55841=CARTESIAN_POINT('Ctrl Pts',(3.66661143271685,0.333333333333333,0.786422660831986));
#55842=CARTESIAN_POINT('Ctrl Pts',(3.66661143271685,0.666666666666667,0.786422660831986));
#55843=CARTESIAN_POINT('Ctrl Pts',(3.66661143271685,1.,0.786422660831986));
#55844=CARTESIAN_POINT('',(4.13571194405636,1.,0.732042837400621));
#55845=CARTESIAN_POINT('',(4.13571194405636,0.,0.732042837400621));
#55846=CARTESIAN_POINT('Ctrl Pts',(3.66661143271685,1.,0.786422660831985));
#55847=CARTESIAN_POINT('Ctrl Pts',(3.6666431041522,1.,0.786459983895432));
#55848=CARTESIAN_POINT('Ctrl Pts',(3.66680946938292,1.,0.786565919558984));
#55849=CARTESIAN_POINT('Ctrl Pts',(3.66743103898702,1.,0.786774337198063));
#55850=CARTESIAN_POINT('Ctrl Pts',(3.66907505398677,1.,0.787145041181546));
#55851=CARTESIAN_POINT('Ctrl Pts',(3.67252923663655,1.,0.787758799995743));
#55852=CARTESIAN_POINT('Ctrl Pts',(3.67777119516252,1.,0.788569566220286));
#55853=CARTESIAN_POINT('Ctrl Pts',(3.68428439783905,1.,0.789483546064387));
#55854=CARTESIAN_POINT('Ctrl Pts',(3.69172044327364,1.,0.790436284988788));
#55855=CARTESIAN_POINT('Ctrl Pts',(3.69968940808721,1.,0.79135657569598));
#55856=CARTESIAN_POINT('Ctrl Pts',(3.70781724021806,1.,0.792177688845818));
#55857=CARTESIAN_POINT('Ctrl Pts',(3.71580242396124,1.,0.792848377370287));
#55858=CARTESIAN_POINT('Ctrl Pts',(3.72348797293734,1.,0.793347023784205));
#55859=CARTESIAN_POINT('Ctrl Pts',(3.73086914695805,1.,0.793682750269684));
#55860=CARTESIAN_POINT('Ctrl Pts',(3.73803280541687,1.,0.793882700937017));
#55861=CARTESIAN_POINT('Ctrl Pts',(3.74511357728861,1.,0.793982700459952));
#55862=CARTESIAN_POINT('Ctrl Pts',(3.75224692493864,1.,0.794017347371378));
#55863=CARTESIAN_POINT('Ctrl Pts',(3.75951468666257,1.,0.794008429134908));
#55864=CARTESIAN_POINT('Ctrl Pts',(3.76692626931111,1.,0.793961083688992));
#55865=CARTESIAN_POINT('Ctrl Pts',(3.77444863801212,1.,0.793870523787408));
#55866=CARTESIAN_POINT('Ctrl Pts',(3.78202460377598,1.,0.793726235781301));
#55867=CARTESIAN_POINT('Ctrl Pts',(3.78959439439235,1.,0.793516871680994));
#55868=CARTESIAN_POINT('Ctrl Pts',(3.79711921389897,1.,0.793235612973274));
#55869=CARTESIAN_POINT('Ctrl Pts',(3.80459229925637,1.,0.792882695234778));
#55870=CARTESIAN_POINT('Ctrl Pts',(3.81202588694756,1.,0.792462483517635));
#55871=CARTESIAN_POINT('Ctrl Pts',(3.81944345442249,1.,0.791981740718635));
#55872=CARTESIAN_POINT('Ctrl Pts',(3.82687033899792,1.,0.791447528662369));
#55873=CARTESIAN_POINT('Ctrl Pts',(3.83432392054786,1.,0.790865012705301));
#55874=CARTESIAN_POINT('Ctrl Pts',(3.84180762342454,1.,0.790236124191243));
#55875=CARTESIAN_POINT('Ctrl Pts',(3.84931637808894,1.,0.789560798155583));
#55876=CARTESIAN_POINT('Ctrl Pts',(3.85683995872529,1.,0.788837734090672));
#55877=CARTESIAN_POINT('Ctrl Pts',(3.86436702561345,1.,0.788065315093778));
#55878=CARTESIAN_POINT('Ctrl Pts',(3.87188916600912,1.,0.787242527617999));
#55879=CARTESIAN_POINT('Ctrl Pts',(3.8794040281819,1.,0.786369675812609));
#55880=CARTESIAN_POINT('Ctrl Pts',(3.88691313167398,1.,0.785447890340731));
#55881=CARTESIAN_POINT('Ctrl Pts',(3.89442039235103,1.,0.784478799358337));
#55882=CARTESIAN_POINT('Ctrl Pts',(3.9019303904397,1.,0.783464141529082));
#55883=CARTESIAN_POINT('Ctrl Pts',(3.90944671004542,1.,0.782405395622765));
#55884=CARTESIAN_POINT('Ctrl Pts',(3.91697036054676,1.,0.781303428618367));
#55885=CARTESIAN_POINT('Ctrl Pts',(3.92450058323823,1.,0.780158678615543));
#55886=CARTESIAN_POINT('Ctrl Pts',(3.93203552473174,1.,0.778971308134821));
#55887=CARTESIAN_POINT('Ctrl Pts',(3.93957296768103,1.,0.777741370568559));
#55888=CARTESIAN_POINT('Ctrl Pts',(3.94711101619447,1.,0.776468966697922));
#55889=CARTESIAN_POINT('Ctrl Pts',(3.9546488545231,1.,0.775154418039352));
#55890=CARTESIAN_POINT('Ctrl Pts',(3.96218649639807,1.,0.773798212026566));
#55891=CARTESIAN_POINT('Ctrl Pts',(3.96972446532772,1.,0.772400931772137));
#55892=CARTESIAN_POINT('Ctrl Pts',(3.97726349165488,1.,0.770963190030471));
#55893=CARTESIAN_POINT('Ctrl Pts',(3.98480422348451,1.,0.769485566245545));
#55894=CARTESIAN_POINT('Ctrl Pts',(3.9923468788101,1.,0.767968531377915));
#55895=CARTESIAN_POINT('Ctrl Pts',(3.99989129179622,1.,0.766412457136064));
#55896=CARTESIAN_POINT('Ctrl Pts',(4.00743706791509,1.,0.764817648785198));
#55897=CARTESIAN_POINT('Ctrl Pts',(4.01498370680496,1.,0.763184371182936));
#55898=CARTESIAN_POINT('Ctrl Pts',(4.02253072741268,1.,0.761512875859805));
#55899=CARTESIAN_POINT('Ctrl Pts',(4.03007781954412,1.,0.759803433243752));
#55900=CARTESIAN_POINT('Ctrl Pts',(4.03762485803119,1.,0.758056338884945));
#55901=CARTESIAN_POINT('Ctrl Pts',(4.04517182653997,1.,0.756271902369581));
#55902=CARTESIAN_POINT('Ctrl Pts',(4.05271876687915,1.,0.754450441816078));
#55903=CARTESIAN_POINT('Ctrl Pts',(4.06026572221515,1.,0.752592276483073));
#55904=CARTESIAN_POINT('Ctrl Pts',(4.06781267242378,1.,0.750697720484037));
#55905=CARTESIAN_POINT('Ctrl Pts',(4.07535951056152,1.,0.748767076680558));
#55906=CARTESIAN_POINT('Ctrl Pts',(4.08290608095642,1.,0.746800631492316));
#55907=CARTESIAN_POINT('Ctrl Pts',(4.09045220253573,1.,0.744798649706501));
#55908=CARTESIAN_POINT('Ctrl Pts',(4.09799769702611,1.,0.742761369689842));
#55909=CARTESIAN_POINT('Ctrl Pts',(4.10554241757547,1.,0.740688998553377));
#55910=CARTESIAN_POINT('Ctrl Pts',(4.11308626951927,1.,0.738581708225844));
#55911=CARTESIAN_POINT('Ctrl Pts',(4.120629196238,1.,0.736439634331345));
#55912=CARTESIAN_POINT('Ctrl Pts',(4.12666277570844,1.,0.734698226764093));
#55913=CARTESIAN_POINT('Ctrl Pts',(4.13118752795207,1.,0.733376589323547));
#55914=CARTESIAN_POINT('Ctrl Pts',(4.1342038373684,1.,0.73248857513516));
#55915=CARTESIAN_POINT('Ctrl Pts',(4.13571194405636,1.,0.732042837400621));
#55916=CARTESIAN_POINT('Origin',(4.13571194405636,0.,0.732042837400621));
#55917=CARTESIAN_POINT('',(4.15950947128175,1.,0.581791163835816));
#55918=CARTESIAN_POINT('Origin',(0.,0.,0.));
#55919=CARTESIAN_POINT('',(3.62400312501245,1.,0.963899035117249));
#55920=CARTESIAN_POINT('Origin',(0.,1.,0.));
#55921=CARTESIAN_POINT('Ctrl Pts',(3.62400312501245,1.,0.963899035117249));
#55922=CARTESIAN_POINT('Ctrl Pts',(3.62400312501245,0.666666666666667,0.963899035117249));
#55923=CARTESIAN_POINT('Ctrl Pts',(3.62400312501245,0.333333333333333,0.963899035117249));
#55924=CARTESIAN_POINT('Ctrl Pts',(3.62400312501245,-0.333333333333333,
0.963899035117249));
#55925=CARTESIAN_POINT('Ctrl Pts',(3.62400312501245,-0.666666666666667,
0.96389903511725));
#55926=CARTESIAN_POINT('Ctrl Pts',(3.62400312501245,-1.,0.96389903511725));
#55927=CARTESIAN_POINT('Ctrl Pts',(4.01728681790024,-1.,1.22531898815164));
#55928=CARTESIAN_POINT('Ctrl Pts',(4.01728681790024,1.,1.22531898815164));
#55929=CARTESIAN_POINT('Ctrl Pts',(4.0161454457032,-1.,1.22423716681447));
#55930=CARTESIAN_POINT('Ctrl Pts',(4.0161454457032,1.,1.22423716681447));
#55931=CARTESIAN_POINT('Ctrl Pts',(4.01386104434674,-1.,1.22207656456199));
#55932=CARTESIAN_POINT('Ctrl Pts',(4.01386104434674,1.,1.22207656456199));
#55933=CARTESIAN_POINT('Ctrl Pts',(4.01042947142681,-1.,1.21884478244983));
#55934=CARTESIAN_POINT('Ctrl Pts',(4.01042947142681,1.,1.21884478244983));
#55935=CARTESIAN_POINT('Ctrl Pts',(4.00584409524937,-1.,1.21455398918813));
#55936=CARTESIAN_POINT('Ctrl Pts',(4.00584409524937,1.,1.21455398918813));
#55937=CARTESIAN_POINT('Ctrl Pts',(4.00009577952534,-1.,1.20922097030107));
#55938=CARTESIAN_POINT('Ctrl Pts',(4.00009577952534,1.,1.20922097030107));
#55939=CARTESIAN_POINT('Ctrl Pts',(3.99433084800649,-1.,1.2039185237544));
#55940=CARTESIAN_POINT('Ctrl Pts',(3.99433084800649,1.,1.2039185237544));
#55941=CARTESIAN_POINT('Ctrl Pts',(3.98854928957287,-1.,1.19864679609596));
#55942=CARTESIAN_POINT('Ctrl Pts',(3.98854928957287,1.,1.19864679609596));
#55943=CARTESIAN_POINT('Ctrl Pts',(3.98275111052015,-1.,1.19340598349307));
#55944=CARTESIAN_POINT('Ctrl Pts',(3.98275111052015,1.,1.19340598349307));
#55945=CARTESIAN_POINT('Ctrl Pts',(3.97693634766926,-1.,1.18819633715285));
#55946=CARTESIAN_POINT('Ctrl Pts',(3.97693634766926,1.,1.18819633715285));
#55947=CARTESIAN_POINT('Ctrl Pts',(3.9711050516465,-1.,1.18301815039596));
#55948=CARTESIAN_POINT('Ctrl Pts',(3.9711050516465,1.,1.18301815039596));
#55949=CARTESIAN_POINT('Ctrl Pts',(3.96525726357682,-1.,1.17787174135446));
#55950=CARTESIAN_POINT('Ctrl Pts',(3.96525726357682,1.,1.17787174135446));
#55951=CARTESIAN_POINT('Ctrl Pts',(3.95939299213164,-1.,1.17275743590327));
#55952=CARTESIAN_POINT('Ctrl Pts',(3.95939299213164,1.,1.17275743590327));
#55953=CARTESIAN_POINT('Ctrl Pts',(3.95351219510062,-1.,1.16767555244495));
#55954=CARTESIAN_POINT('Ctrl Pts',(3.95351219510062,1.,1.16767555244495));
#55955=CARTESIAN_POINT('Ctrl Pts',(3.9476147478092,-1.,1.16262637999261));
#55956=CARTESIAN_POINT('Ctrl Pts',(3.9476147478092,1.,1.16262637999261));
#55957=CARTESIAN_POINT('Ctrl Pts',(3.94170046685542,-1.,1.15761018341061));
#55958=CARTESIAN_POINT('Ctrl Pts',(3.94170046685542,1.,1.15761018341061));
#55959=CARTESIAN_POINT('Ctrl Pts',(3.9357691705651,-1.,1.15262722716391));
#55960=CARTESIAN_POINT('Ctrl Pts',(3.9357691705651,1.,1.15262722716391));
#55961=CARTESIAN_POINT('Ctrl Pts',(3.92982073294334,-1.,1.14767779451147));
#55962=CARTESIAN_POINT('Ctrl Pts',(3.92982073294334,1.,1.14767779451147));
#55963=CARTESIAN_POINT('Ctrl Pts',(3.92385513133937,-1.,1.14276220561575));
#55964=CARTESIAN_POINT('Ctrl Pts',(3.92385513133937,1.,1.14276220561575));
#55965=CARTESIAN_POINT('Ctrl Pts',(3.91787251936688,-1.,1.13788084225511));
#55966=CARTESIAN_POINT('Ctrl Pts',(3.91787251936688,1.,1.13788084225511));
#55967=CARTESIAN_POINT('Ctrl Pts',(3.91187321145495,-1.,1.13303414693849));
#55968=CARTESIAN_POINT('Ctrl Pts',(3.91187321145495,1.,1.13303414693849));
#55969=CARTESIAN_POINT('Ctrl Pts',(3.90585753318622,-1.,1.12822258281518));
#55970=CARTESIAN_POINT('Ctrl Pts',(3.90585753318622,1.,1.12822258281518));
#55971=CARTESIAN_POINT('Ctrl Pts',(3.89982569749978,-1.,1.12344660099029));
#55972=CARTESIAN_POINT('Ctrl Pts',(3.89982569749978,1.,1.12344660099029));
#55973=CARTESIAN_POINT('Ctrl Pts',(3.89377768340362,-1.,1.11870660794609));
#55974=CARTESIAN_POINT('Ctrl Pts',(3.89377768340362,1.,1.11870660794609));
#55975=CARTESIAN_POINT('Ctrl Pts',(3.88771308285229,-1.,1.11400292434447));
#55976=CARTESIAN_POINT('Ctrl Pts',(3.88771308285229,1.,1.11400292434447));
#55977=CARTESIAN_POINT('Ctrl Pts',(3.88163105531791,-1.,1.10933577224029));
#55978=CARTESIAN_POINT('Ctrl Pts',(3.88163105531791,1.,1.10933577224029));
#55979=CARTESIAN_POINT('Ctrl Pts',(3.87553067187566,-1.,1.10470536603303));
#55980=CARTESIAN_POINT('Ctrl Pts',(3.87553067187566,1.,1.10470536603303));
#55981=CARTESIAN_POINT('Ctrl Pts',(3.86941120134872,-1.,1.10011198761203));
#55982=CARTESIAN_POINT('Ctrl Pts',(3.86941120134872,1.,1.10011198761203));
#55983=CARTESIAN_POINT('Ctrl Pts',(3.86327241021242,-1.,1.09555606505012));
#55984=CARTESIAN_POINT('Ctrl Pts',(3.86327241021242,1.,1.09555606505012));
#55985=CARTESIAN_POINT('Ctrl Pts',(3.85711487933911,-1.,1.09103825516288));
#55986=CARTESIAN_POINT('Ctrl Pts',(3.85711487933911,1.,1.09103825516288));
#55987=CARTESIAN_POINT('Ctrl Pts',(3.8509402522269,-1.,1.08655950846377));
#55988=CARTESIAN_POINT('Ctrl Pts',(3.8509402522269,1.,1.08655950846377));
#55989=CARTESIAN_POINT('Ctrl Pts',(3.84475048030615,-1.,1.08212087917986));
#55990=CARTESIAN_POINT('Ctrl Pts',(3.84475048030615,1.,1.08212087917986));
#55991=CARTESIAN_POINT('Ctrl Pts',(3.83854714117486,-1.,1.07772335353856));
#55992=CARTESIAN_POINT('Ctrl Pts',(3.83854714117486,1.,1.07772335353856));
#55993=CARTESIAN_POINT('Ctrl Pts',(3.83233071195145,-1.,1.0733676663346));
#55994=CARTESIAN_POINT('Ctrl Pts',(3.83233071195145,1.,1.0733676663346));
#55995=CARTESIAN_POINT('Ctrl Pts',(3.82609989967278,-1.,1.0690541318036));
#55996=CARTESIAN_POINT('Ctrl Pts',(3.82609989967278,1.,1.0690541318036));
#55997=CARTESIAN_POINT('Ctrl Pts',(3.81985083953012,-1.,1.06478244038931));
#55998=CARTESIAN_POINT('Ctrl Pts',(3.81985083953012,1.,1.06478244038931));
#55999=CARTESIAN_POINT('Ctrl Pts',(3.81357866117485,-1.,1.06055206187298));
#56000=CARTESIAN_POINT('Ctrl Pts',(3.81357866117485,1.,1.06055206187298));
#56001=CARTESIAN_POINT('Ctrl Pts',(3.80727913637784,-1.,1.05636266918643));
#56002=CARTESIAN_POINT('Ctrl Pts',(3.80727913637784,1.,1.05636266918643));
#56003=CARTESIAN_POINT('Ctrl Pts',(3.80095039790678,-1.,1.05221457990015));
#56004=CARTESIAN_POINT('Ctrl Pts',(3.80095039790678,1.,1.05221457990015));
#56005=CARTESIAN_POINT('Ctrl Pts',(3.79459440308793,-1.,1.04810913267641));
#56006=CARTESIAN_POINT('Ctrl Pts',(3.79459440308793,1.,1.04810913267641));
#56007=CARTESIAN_POINT('Ctrl Pts',(3.78821910787195,-1.,1.04404924374426));
#56008=CARTESIAN_POINT('Ctrl Pts',(3.78821910787195,1.,1.04404924374426));
#56009=CARTESIAN_POINT('Ctrl Pts',(3.78183535008192,-1.,1.04003862055804));
#56010=CARTESIAN_POINT('Ctrl Pts',(3.78183535008192,1.,1.04003862055804));
#56011=CARTESIAN_POINT('Ctrl Pts',(3.77545283140445,-1.,1.03608074678013));
#56012=CARTESIAN_POINT('Ctrl Pts',(3.77545283140445,1.,1.03608074678013));
#56013=CARTESIAN_POINT('Ctrl Pts',(3.76907609832522,-1.,1.0321778660492));
#56014=CARTESIAN_POINT('Ctrl Pts',(3.76907609832522,1.,1.0321778660492));
#56015=CARTESIAN_POINT('Ctrl Pts',(3.76270122291232,-1.,1.02833014458181));
#56016=CARTESIAN_POINT('Ctrl Pts',(3.76270122291232,1.,1.02833014458181));
#56017=CARTESIAN_POINT('Ctrl Pts',(3.75631037456194,-1.,1.0245342944466));
#56018=CARTESIAN_POINT('Ctrl Pts',(3.75631037456194,1.,1.0245342944466));
#56019=CARTESIAN_POINT('Ctrl Pts',(3.74987777155834,-1.,1.02078510487428));
#56020=CARTESIAN_POINT('Ctrl Pts',(3.74987777155834,1.,1.02078510487428));
#56021=CARTESIAN_POINT('Ctrl Pts',(3.74337942504959,-1.,1.01707794311079));
#56022=CARTESIAN_POINT('Ctrl Pts',(3.74337942504959,1.,1.01707794311079));
#56023=CARTESIAN_POINT('Ctrl Pts',(3.73680245055734,-1.,1.01341114319903));
#56024=CARTESIAN_POINT('Ctrl Pts',(3.73680245055734,1.,1.01341114319903));
#56025=CARTESIAN_POINT('Ctrl Pts',(3.73015276704426,-1.,1.00978798539496));
#56026=CARTESIAN_POINT('Ctrl Pts',(3.73015276704426,1.,1.00978798539496));
#56027=CARTESIAN_POINT('Ctrl Pts',(3.72346803750595,-1.,1.0062200073571));
#56028=CARTESIAN_POINT('Ctrl Pts',(3.72346803750595,1.,1.0062200073571));
#56029=CARTESIAN_POINT('Ctrl Pts',(3.71680667125118,-1.,1.00272423396822));
#56030=CARTESIAN_POINT('Ctrl Pts',(3.71680667125118,1.,1.00272423396822));
#56031=CARTESIAN_POINT('Ctrl Pts',(3.71022439713938,-1.,0.999317260756531));
#56032=CARTESIAN_POINT('Ctrl Pts',(3.71022439713938,1.,0.999317260756531));
#56033=CARTESIAN_POINT('Ctrl Pts',(3.70375282282138,-1.,0.996009819772518));
#56034=CARTESIAN_POINT('Ctrl Pts',(3.70375282282138,1.,0.996009819772518));
#56035=CARTESIAN_POINT('Ctrl Pts',(3.69738123415662,-1.,0.992802218332011));
#56036=CARTESIAN_POINT('Ctrl Pts',(3.69738123415662,1.,0.992802218332011));
#56037=CARTESIAN_POINT('Ctrl Pts',(3.69102682138846,-1.,0.989676715398559));
#56038=CARTESIAN_POINT('Ctrl Pts',(3.69102682138846,1.,0.989676715398559));
#56039=CARTESIAN_POINT('Ctrl Pts',(3.68455317926068,-1.,0.986602639863838));
#56040=CARTESIAN_POINT('Ctrl Pts',(3.68455317926068,1.,0.986602639863838));
#56041=CARTESIAN_POINT('Ctrl Pts',(3.67782408841715,-1.,0.98355079147042));
#56042=CARTESIAN_POINT('Ctrl Pts',(3.67782408841715,1.,0.98355079147042));
#56043=CARTESIAN_POINT('Ctrl Pts',(3.67074983340361,-1.,0.980505922458267));
#56044=CARTESIAN_POINT('Ctrl Pts',(3.67074983340361,1.,0.980505922458267));
#56045=CARTESIAN_POINT('Ctrl Pts',(3.66333049637475,-1.,0.977478312751618));
#56046=CARTESIAN_POINT('Ctrl Pts',(3.66333049637475,1.,0.977478312751618));
#56047=CARTESIAN_POINT('Ctrl Pts',(3.65571576735126,-1.,0.974519971354849));
#56048=CARTESIAN_POINT('Ctrl Pts',(3.65571576735126,1.,0.974519971354849));
#56049=CARTESIAN_POINT('Ctrl Pts',(3.64819756447455,-1.,0.971722122061341));
#56050=CARTESIAN_POINT('Ctrl Pts',(3.64819756447455,1.,0.971722122061341));
#56051=CARTESIAN_POINT('Ctrl Pts',(3.64113946505766,-1.,0.969195124675866));
#56052=CARTESIAN_POINT('Ctrl Pts',(3.64113946505766,1.,0.969195124675866));
#56053=CARTESIAN_POINT('Ctrl Pts',(3.63492122081143,-1.,0.967052554541386));
#56054=CARTESIAN_POINT('Ctrl Pts',(3.63492122081143,1.,0.967052554541386));
#56055=CARTESIAN_POINT('Ctrl Pts',(3.62988252139846,-1.,0.965395153165294));
#56056=CARTESIAN_POINT('Ctrl Pts',(3.62988252139846,1.,0.965395153165294));
#56057=CARTESIAN_POINT('Ctrl Pts',(3.62625391254797,-1.,0.964291001273288));
#56058=CARTESIAN_POINT('Ctrl Pts',(3.62625391254797,1.,0.964291001273288));
#56059=CARTESIAN_POINT('Ctrl Pts',(3.6245656860652,-1.,0.96387577453062));
#56060=CARTESIAN_POINT('Ctrl Pts',(3.6245656860652,1.,0.96387577453062));
#56061=CARTESIAN_POINT('Ctrl Pts',(3.62399933639914,-1.,0.963832486395052));
#56062=CARTESIAN_POINT('Ctrl Pts',(3.62399933639914,1.,0.963832486395052));
#56063=CARTESIAN_POINT('Ctrl Pts',(3.62393257642052,-1.,0.963922720982194));
#56064=CARTESIAN_POINT('Ctrl Pts',(3.62393257642052,1.,0.963922720982194));
#56065=CARTESIAN_POINT('Ctrl Pts',(3.62397690409552,-1.,0.963997613369571));
#56066=CARTESIAN_POINT('Ctrl Pts',(3.62397690409552,1.,0.963997613369571));
#56067=CARTESIAN_POINT('',(4.01728681790024,1.,1.22531898815164));
#56068=CARTESIAN_POINT('Ctrl Pts',(4.01728681790024,1.,1.22531898815164));
#56069=CARTESIAN_POINT('Ctrl Pts',(4.0161454457032,1.,1.22423716681447));
#56070=CARTESIAN_POINT('Ctrl Pts',(4.01386104434674,1.,1.22207656456199));
#56071=CARTESIAN_POINT('Ctrl Pts',(4.01042947142681,1.,1.21884478244983));
#56072=CARTESIAN_POINT('Ctrl Pts',(4.00584409524937,1.,1.21455398918813));
#56073=CARTESIAN_POINT('Ctrl Pts',(4.00009577952534,1.,1.20922097030107));
#56074=CARTESIAN_POINT('Ctrl Pts',(3.99433084800649,1.,1.2039185237544));
#56075=CARTESIAN_POINT('Ctrl Pts',(3.98854928957287,1.,1.19864679609596));
#56076=CARTESIAN_POINT('Ctrl Pts',(3.98275111052015,1.,1.19340598349307));
#56077=CARTESIAN_POINT('Ctrl Pts',(3.97693634766926,1.,1.18819633715285));
#56078=CARTESIAN_POINT('Ctrl Pts',(3.9711050516465,1.,1.18301815039596));
#56079=CARTESIAN_POINT('Ctrl Pts',(3.96525726357682,1.,1.17787174135446));
#56080=CARTESIAN_POINT('Ctrl Pts',(3.95939299213164,1.,1.17275743590327));
#56081=CARTESIAN_POINT('Ctrl Pts',(3.95351219510062,1.,1.16767555244495));
#56082=CARTESIAN_POINT('Ctrl Pts',(3.9476147478092,1.,1.16262637999261));
#56083=CARTESIAN_POINT('Ctrl Pts',(3.94170046685542,1.,1.15761018341061));
#56084=CARTESIAN_POINT('Ctrl Pts',(3.9357691705651,1.,1.15262722716391));
#56085=CARTESIAN_POINT('Ctrl Pts',(3.92982073294334,1.,1.14767779451147));
#56086=CARTESIAN_POINT('Ctrl Pts',(3.92385513133937,1.,1.14276220561575));
#56087=CARTESIAN_POINT('Ctrl Pts',(3.91787251936688,1.,1.13788084225511));
#56088=CARTESIAN_POINT('Ctrl Pts',(3.91187321145495,1.,1.13303414693849));
#56089=CARTESIAN_POINT('Ctrl Pts',(3.90585753318622,1.,1.12822258281518));
#56090=CARTESIAN_POINT('Ctrl Pts',(3.89982569749978,1.,1.12344660099029));
#56091=CARTESIAN_POINT('Ctrl Pts',(3.89377768340362,1.,1.11870660794609));
#56092=CARTESIAN_POINT('Ctrl Pts',(3.88771308285229,1.,1.11400292434447));
#56093=CARTESIAN_POINT('Ctrl Pts',(3.88163105531791,1.,1.10933577224029));
#56094=CARTESIAN_POINT('Ctrl Pts',(3.87553067187566,1.,1.10470536603303));
#56095=CARTESIAN_POINT('Ctrl Pts',(3.86941120134872,1.,1.10011198761203));
#56096=CARTESIAN_POINT('Ctrl Pts',(3.86327241021242,1.,1.09555606505012));
#56097=CARTESIAN_POINT('Ctrl Pts',(3.85711487933911,1.,1.09103825516288));
#56098=CARTESIAN_POINT('Ctrl Pts',(3.8509402522269,1.,1.08655950846377));
#56099=CARTESIAN_POINT('Ctrl Pts',(3.84475048030615,1.,1.08212087917986));
#56100=CARTESIAN_POINT('Ctrl Pts',(3.83854714117486,1.,1.07772335353856));
#56101=CARTESIAN_POINT('Ctrl Pts',(3.83233071195145,1.,1.0733676663346));
#56102=CARTESIAN_POINT('Ctrl Pts',(3.82609989967278,1.,1.0690541318036));
#56103=CARTESIAN_POINT('Ctrl Pts',(3.81985083953012,1.,1.06478244038931));
#56104=CARTESIAN_POINT('Ctrl Pts',(3.81357866117485,1.,1.06055206187298));
#56105=CARTESIAN_POINT('Ctrl Pts',(3.80727913637784,1.,1.05636266918643));
#56106=CARTESIAN_POINT('Ctrl Pts',(3.80095039790678,1.,1.05221457990015));
#56107=CARTESIAN_POINT('Ctrl Pts',(3.79459440308793,1.,1.04810913267641));
#56108=CARTESIAN_POINT('Ctrl Pts',(3.78821910787195,1.,1.04404924374426));
#56109=CARTESIAN_POINT('Ctrl Pts',(3.78183535008192,1.,1.04003862055804));
#56110=CARTESIAN_POINT('Ctrl Pts',(3.77545283140445,1.,1.03608074678013));
#56111=CARTESIAN_POINT('Ctrl Pts',(3.76907609832522,1.,1.0321778660492));
#56112=CARTESIAN_POINT('Ctrl Pts',(3.76270122291232,1.,1.02833014458181));
#56113=CARTESIAN_POINT('Ctrl Pts',(3.75631037456194,1.,1.0245342944466));
#56114=CARTESIAN_POINT('Ctrl Pts',(3.74987777155834,1.,1.02078510487428));
#56115=CARTESIAN_POINT('Ctrl Pts',(3.74337942504959,1.,1.01707794311079));
#56116=CARTESIAN_POINT('Ctrl Pts',(3.73680245055734,1.,1.01341114319903));
#56117=CARTESIAN_POINT('Ctrl Pts',(3.73015276704426,1.,1.00978798539496));
#56118=CARTESIAN_POINT('Ctrl Pts',(3.72346803750595,1.,1.0062200073571));
#56119=CARTESIAN_POINT('Ctrl Pts',(3.71680667125118,1.,1.00272423396822));
#56120=CARTESIAN_POINT('Ctrl Pts',(3.71022439713938,1.,0.999317260756531));
#56121=CARTESIAN_POINT('Ctrl Pts',(3.70375282282138,1.,0.996009819772518));
#56122=CARTESIAN_POINT('Ctrl Pts',(3.69738123415662,1.,0.992802218332011));
#56123=CARTESIAN_POINT('Ctrl Pts',(3.69102682138846,1.,0.989676715398559));
#56124=CARTESIAN_POINT('Ctrl Pts',(3.68455317926068,1.,0.986602639863838));
#56125=CARTESIAN_POINT('Ctrl Pts',(3.67782408841715,1.,0.98355079147042));
#56126=CARTESIAN_POINT('Ctrl Pts',(3.67074983340361,1.,0.980505922458267));
#56127=CARTESIAN_POINT('Ctrl Pts',(3.66333049637475,1.,0.977478312751618));
#56128=CARTESIAN_POINT('Ctrl Pts',(3.65571576735126,1.,0.974519971354849));
#56129=CARTESIAN_POINT('Ctrl Pts',(3.64819756447455,1.,0.971722122061341));
#56130=CARTESIAN_POINT('Ctrl Pts',(3.64113946505766,1.,0.969195124675866));
#56131=CARTESIAN_POINT('Ctrl Pts',(3.63492122081143,1.,0.967052554541386));
#56132=CARTESIAN_POINT('Ctrl Pts',(3.62988252139846,1.,0.965395153165294));
#56133=CARTESIAN_POINT('Ctrl Pts',(3.62652618145335,1.,0.964373850166458));
#56134=CARTESIAN_POINT('Ctrl Pts',(3.62489305727662,1.,0.963957782642844));
#56135=CARTESIAN_POINT('Ctrl Pts',(3.62424461507588,1.,0.963861297423241));
#56136=CARTESIAN_POINT('Ctrl Pts',(3.6240482887845,1.,0.963880158555582));
#56137=CARTESIAN_POINT('Ctrl Pts',(3.62400312501245,1.,0.963899035117249));
#56138=CARTESIAN_POINT('',(4.01728681790024,0.,1.22531898815164));
#56139=CARTESIAN_POINT('Ctrl Pts',(3.49848248301936,-1.,1.35022972712301));
#56140=CARTESIAN_POINT('Ctrl Pts',(3.49848248301936,1.,1.35022972712301));
#56141=CARTESIAN_POINT('Ctrl Pts',(3.4984026005375,-1.,1.35026426118402));
#56142=CARTESIAN_POINT('Ctrl Pts',(3.4984026005375,1.,1.35026426118402));
#56143=CARTESIAN_POINT('Ctrl Pts',(3.49840357193736,-1.,1.35037650303019));
#56144=CARTESIAN_POINT('Ctrl Pts',(3.49840357193736,1.,1.35037650303019));
#56145=CARTESIAN_POINT('Ctrl Pts',(3.49888720257132,-1.,1.35067437417484));
#56146=CARTESIAN_POINT('Ctrl Pts',(3.49888720257132,1.,1.35067437417484));
#56147=CARTESIAN_POINT('Ctrl Pts',(3.5004970706414,-1.,1.3513307633124));
#56148=CARTESIAN_POINT('Ctrl Pts',(3.5004970706414,1.,1.3513307633124));
#56149=CARTESIAN_POINT('Ctrl Pts',(3.50408168106261,-1.,1.35257032843486));
#56150=CARTESIAN_POINT('Ctrl Pts',(3.50408168106261,1.,1.35257032843486));
#56151=CARTESIAN_POINT('Ctrl Pts',(3.50913227059999,-1.,1.35419113575956));
#56152=CARTESIAN_POINT('Ctrl Pts',(3.50913227059999,1.,1.35419113575956));
#56153=CARTESIAN_POINT('Ctrl Pts',(3.51542230699556,-1.,1.35611275237152));
#56154=CARTESIAN_POINT('Ctrl Pts',(3.51542230699556,1.,1.35611275237152));
#56155=CARTESIAN_POINT('Ctrl Pts',(3.52261776116748,-1.,1.35821701528836));
#56156=CARTESIAN_POINT('Ctrl Pts',(3.52261776116748,1.,1.35821701528836));
#56157=CARTESIAN_POINT('Ctrl Pts',(3.530344649616,-1.,1.36037259643734));
#56158=CARTESIAN_POINT('Ctrl Pts',(3.530344649616,1.,1.36037259643734));
#56159=CARTESIAN_POINT('Ctrl Pts',(3.53824396424961,-1.,1.36245507339307));
#56160=CARTESIAN_POINT('Ctrl Pts',(3.53824396424961,1.,1.36245507339307));
#56161=CARTESIAN_POINT('Ctrl Pts',(3.54602591832973,-1.,1.36436666257598));
#56162=CARTESIAN_POINT('Ctrl Pts',(3.54602591832973,1.,1.36436666257598));
#56163=CARTESIAN_POINT('Ctrl Pts',(3.55353883995949,-1.,1.3660614545677));
#56164=CARTESIAN_POINT('Ctrl Pts',(3.55353883995949,1.,1.3660614545677));
#56165=CARTESIAN_POINT('Ctrl Pts',(3.56077662028649,-1.,1.36754771771233));
#56166=CARTESIAN_POINT('Ctrl Pts',(3.56077662028649,1.,1.36754771771233));
#56167=CARTESIAN_POINT('Ctrl Pts',(3.5678208030466,-1.,1.36886584973389));
#56168=CARTESIAN_POINT('Ctrl Pts',(3.5678208030466,1.,1.36886584973389));
#56169=CARTESIAN_POINT('Ctrl Pts',(3.57479875549486,-1.,1.37007229485659));
#56170=CARTESIAN_POINT('Ctrl Pts',(3.57479875549486,1.,1.37007229485659));
#56171=CARTESIAN_POINT('Ctrl Pts',(3.58183885982715,-1.,1.37122241663062));
#56172=CARTESIAN_POINT('Ctrl Pts',(3.58183885982715,1.,1.37122241663062));
#56173=CARTESIAN_POINT('Ctrl Pts',(3.58901853846365,-1.,1.37235053660976));
#56174=CARTESIAN_POINT('Ctrl Pts',(3.58901853846365,1.,1.37235053660976));
#56175=CARTESIAN_POINT('Ctrl Pts',(3.59634627869048,-1.,1.37346320103157));
#56176=CARTESIAN_POINT('Ctrl Pts',(3.59634627869048,1.,1.37346320103157));
#56177=CARTESIAN_POINT('Ctrl Pts',(3.60379020123988,-1.,1.37455051379623));
#56178=CARTESIAN_POINT('Ctrl Pts',(3.60379020123988,1.,1.37455051379623));
#56179=CARTESIAN_POINT('Ctrl Pts',(3.61129546591064,-1.,1.37559314436634));
#56180=CARTESIAN_POINT('Ctrl Pts',(3.61129546591064,1.,1.37559314436634));
#56181=CARTESIAN_POINT('Ctrl Pts',(3.6188048116042,-1.,1.37657053403107));
#56182=CARTESIAN_POINT('Ctrl Pts',(3.6188048116042,1.,1.37657053403107));
#56183=CARTESIAN_POINT('Ctrl Pts',(3.62628098665145,-1.,1.37746987919881));
#56184=CARTESIAN_POINT('Ctrl Pts',(3.62628098665145,1.,1.37746987919881));
#56185=CARTESIAN_POINT('Ctrl Pts',(3.63371727442486,-1.,1.37829035457339));
#56186=CARTESIAN_POINT('Ctrl Pts',(3.63371727442486,1.,1.37829035457339));
#56187=CARTESIAN_POINT('Ctrl Pts',(3.64112507791141,-1.,1.37903818567359));
#56188=CARTESIAN_POINT('Ctrl Pts',(3.64112507791141,1.,1.37903818567359));
#56189=CARTESIAN_POINT('Ctrl Pts',(3.64852652756456,-1.,1.37972372481603));
#56190=CARTESIAN_POINT('Ctrl Pts',(3.64852652756456,1.,1.37972372481603));
#56191=CARTESIAN_POINT('Ctrl Pts',(3.6559455440439,-1.,1.38035791051213));
#56192=CARTESIAN_POINT('Ctrl Pts',(3.6559455440439,1.,1.38035791051213));
#56193=CARTESIAN_POINT('Ctrl Pts',(3.66339848520857,-1.,1.38094856333552));
#56194=CARTESIAN_POINT('Ctrl Pts',(3.66339848520857,1.,1.38094856333552));
#56195=CARTESIAN_POINT('Ctrl Pts',(3.67088843112262,-1.,1.38149812653868));
#56196=CARTESIAN_POINT('Ctrl Pts',(3.67088843112262,1.,1.38149812653868));
#56197=CARTESIAN_POINT('Ctrl Pts',(3.67841038482414,-1.,1.3820057429062));
#56198=CARTESIAN_POINT('Ctrl Pts',(3.67841038482414,1.,1.3820057429062));
#56199=CARTESIAN_POINT('Ctrl Pts',(3.68595444983837,-1.,1.38246852827182));
#56200=CARTESIAN_POINT('Ctrl Pts',(3.68595444983837,1.,1.38246852827182));
#56201=CARTESIAN_POINT('Ctrl Pts',(3.69350967899526,-1.,1.38288311171651));
#56202=CARTESIAN_POINT('Ctrl Pts',(3.69350967899526,1.,1.38288311171651));
#56203=CARTESIAN_POINT('Ctrl Pts',(3.701067921679,-1.,1.38324717612865));
#56204=CARTESIAN_POINT('Ctrl Pts',(3.701067921679,1.,1.38324717612865));
#56205=CARTESIAN_POINT('Ctrl Pts',(3.70862680753347,-1.,1.38356065402124));
#56206=CARTESIAN_POINT('Ctrl Pts',(3.70862680753347,1.,1.38356065402124));
#56207=CARTESIAN_POINT('Ctrl Pts',(3.7161876605181,-1.,1.38382489984586));
#56208=CARTESIAN_POINT('Ctrl Pts',(3.7161876605181,1.,1.38382489984586));
#56209=CARTESIAN_POINT('Ctrl Pts',(3.72375409358803,-1.,1.3840421342895));
#56210=CARTESIAN_POINT('Ctrl Pts',(3.72375409358803,1.,1.3840421342895));
#56211=CARTESIAN_POINT('Ctrl Pts',(3.73133035859282,-1.,1.38421479111531));
#56212=CARTESIAN_POINT('Ctrl Pts',(3.73133035859282,1.,1.38421479111531));
#56213=CARTESIAN_POINT('Ctrl Pts',(3.73891976418104,-1.,1.38434489156458));
#56214=CARTESIAN_POINT('Ctrl Pts',(3.73891976418104,1.,1.38434489156458));
#56215=CARTESIAN_POINT('Ctrl Pts',(3.74652317167876,-1.,1.38443344984394));
#56216=CARTESIAN_POINT('Ctrl Pts',(3.74652317167876,1.,1.38443344984394));
#56217=CARTESIAN_POINT('Ctrl Pts',(3.7541397631875,-1.,1.38448077997163));
#56218=CARTESIAN_POINT('Ctrl Pts',(3.7541397631875,1.,1.38448077997163));
#56219=CARTESIAN_POINT('Ctrl Pts',(3.76176768271367,-1.,1.3844867525335));
#56220=CARTESIAN_POINT('Ctrl Pts',(3.76176768271367,1.,1.3844867525335));
#56221=CARTESIAN_POINT('Ctrl Pts',(3.76940473185779,-1.,1.38445107339518));
#56222=CARTESIAN_POINT('Ctrl Pts',(3.76940473185779,1.,1.38445107339518));
#56223=CARTESIAN_POINT('Ctrl Pts',(3.77704902230418,-1.,1.38437354551428));
#56224=CARTESIAN_POINT('Ctrl Pts',(3.77704902230418,1.,1.38437354551428));
#56225=CARTESIAN_POINT('Ctrl Pts',(3.78469969805082,-1.,1.38425435883756));
#56226=CARTESIAN_POINT('Ctrl Pts',(3.78469969805082,1.,1.38425435883756));
#56227=CARTESIAN_POINT('Ctrl Pts',(3.79235669640841,-1.,1.38409399694566));
#56228=CARTESIAN_POINT('Ctrl Pts',(3.79235669640841,1.,1.38409399694566));
#56229=CARTESIAN_POINT('Ctrl Pts',(3.80002044322111,-1.,1.38389311766682));
#56230=CARTESIAN_POINT('Ctrl Pts',(3.80002044322111,1.,1.38389311766682));
#56231=CARTESIAN_POINT('Ctrl Pts',(3.80769156398411,-1.,1.3836524404622));
#56232=CARTESIAN_POINT('Ctrl Pts',(3.80769156398411,1.,1.3836524404622));
#56233=CARTESIAN_POINT('Ctrl Pts',(3.81537060817811,-1.,1.38337263902782));
#56234=CARTESIAN_POINT('Ctrl Pts',(3.81537060817811,1.,1.38337263902782));
#56235=CARTESIAN_POINT('Ctrl Pts',(3.82305771743829,-1.,1.38305421262763));
#56236=CARTESIAN_POINT('Ctrl Pts',(3.82305771743829,1.,1.38305421262763));
#56237=CARTESIAN_POINT('Ctrl Pts',(3.8307526698229,-1.,1.38269750245138));
#56238=CARTESIAN_POINT('Ctrl Pts',(3.8307526698229,1.,1.38269750245138));
#56239=CARTESIAN_POINT('Ctrl Pts',(3.83845502790746,-1.,1.38230274828822));
#56240=CARTESIAN_POINT('Ctrl Pts',(3.83845502790746,1.,1.38230274828822));
#56241=CARTESIAN_POINT('Ctrl Pts',(3.84616425605764,-1.,1.38187013346109));
#56242=CARTESIAN_POINT('Ctrl Pts',(3.84616425605764,1.,1.38187013346109));
#56243=CARTESIAN_POINT('Ctrl Pts',(3.85387983979481,-1.,1.3813998311505));
#56244=CARTESIAN_POINT('Ctrl Pts',(3.85387983979481,1.,1.3813998311505));
#56245=CARTESIAN_POINT('Ctrl Pts',(3.86160143043959,-1.,1.3808920599299));
#56246=CARTESIAN_POINT('Ctrl Pts',(3.86160143043959,1.,1.3808920599299));
#56247=CARTESIAN_POINT('Ctrl Pts',(3.86932885813068,-1.,1.38034709213014));
#56248=CARTESIAN_POINT('Ctrl Pts',(3.86932885813068,1.,1.38034709213014));
#56249=CARTESIAN_POINT('Ctrl Pts',(3.87706205830532,-1.,1.37976523097073));
#56250=CARTESIAN_POINT('Ctrl Pts',(3.87706205830532,1.,1.37976523097073));
#56251=CARTESIAN_POINT('Ctrl Pts',(3.88480102249277,-1.,1.37914679719383));
#56252=CARTESIAN_POINT('Ctrl Pts',(3.88480102249277,1.,1.37914679719383));
#56253=CARTESIAN_POINT('Ctrl Pts',(3.89254574338496,-1.,1.3784921128802));
#56254=CARTESIAN_POINT('Ctrl Pts',(3.89254574338496,1.,1.3784921128802));
#56255=CARTESIAN_POINT('Ctrl Pts',(3.90029615196727,-1.,1.37780148512792));
#56256=CARTESIAN_POINT('Ctrl Pts',(3.90029615196727,1.,1.37780148512792));
#56257=CARTESIAN_POINT('Ctrl Pts',(3.90805209523486,-1.,1.3770751963402));
#56258=CARTESIAN_POINT('Ctrl Pts',(3.90805209523486,1.,1.3770751963402));
#56259=CARTESIAN_POINT('Ctrl Pts',(3.91581337462644,-1.,1.37631350505797));
#56260=CARTESIAN_POINT('Ctrl Pts',(3.91581337462644,1.,1.37631350505797));
#56261=CARTESIAN_POINT('Ctrl Pts',(3.92357976987672,-1.,1.37551664448242));
#56262=CARTESIAN_POINT('Ctrl Pts',(3.92357976987672,1.,1.37551664448242));
#56263=CARTESIAN_POINT('Ctrl Pts',(3.93135106761844,-1.,1.37468482215751));
#56264=CARTESIAN_POINT('Ctrl Pts',(3.93135106761844,1.,1.37468482215751));
#56265=CARTESIAN_POINT('Ctrl Pts',(3.93912709040818,-1.,1.37381821967165));
#56266=CARTESIAN_POINT('Ctrl Pts',(3.93912709040818,1.,1.37381821967165));
#56267=CARTESIAN_POINT('Ctrl Pts',(3.94690771785133,-1.,1.37291699202807));
#56268=CARTESIAN_POINT('Ctrl Pts',(3.94690771785133,1.,1.37291699202807));
#56269=CARTESIAN_POINT('Ctrl Pts',(3.95469287280914,-1.,1.37198126432386));
#56270=CARTESIAN_POINT('Ctrl Pts',(3.95469287280914,1.,1.37198126432386));
#56271=CARTESIAN_POINT('Ctrl Pts',(3.96092458506535,-1.,1.3712051561502));
#56272=CARTESIAN_POINT('Ctrl Pts',(3.96092458506535,1.,1.3712051561502));
#56273=CARTESIAN_POINT('Ctrl Pts',(3.96560037974645,-1.,1.37060761745635));
#56274=CARTESIAN_POINT('Ctrl Pts',(3.96560037974645,1.,1.37060761745635));
#56275=CARTESIAN_POINT('Ctrl Pts',(3.9687184694131,-1.,1.37020239094614));
#56276=CARTESIAN_POINT('Ctrl Pts',(3.9687184694131,1.,1.37020239094614));
#56277=CARTESIAN_POINT('Ctrl Pts',(3.97027773754922,-1.,1.36999806084573));
#56278=CARTESIAN_POINT('Ctrl Pts',(3.97027773754922,1.,1.36999806084573));
#56279=CARTESIAN_POINT('',(3.4984457533445,1.,1.35032489087101));
#56280=CARTESIAN_POINT('Ctrl Pts',(3.4984457533445,-1.,1.35032489087101));
#56281=CARTESIAN_POINT('Ctrl Pts',(3.4984457533445,-0.666666666666667,1.35032489087101));
#56282=CARTESIAN_POINT('Ctrl Pts',(3.4984457533445,-0.333333333333333,1.35032489087101));
#56283=CARTESIAN_POINT('Ctrl Pts',(3.4984457533445,0.333333333333333,1.35032489087101));
#56284=CARTESIAN_POINT('Ctrl Pts',(3.4984457533445,0.666666666666667,1.35032489087101));
#56285=CARTESIAN_POINT('Ctrl Pts',(3.4984457533445,1.,1.35032489087101));
#56286=CARTESIAN_POINT('',(3.97027773754922,1.,1.36999806084573));
#56287=CARTESIAN_POINT('',(3.97027773754922,0.,1.36999806084573));
#56288=CARTESIAN_POINT('Ctrl Pts',(3.4984457533445,1.,1.35032489087101));
#56289=CARTESIAN_POINT('Ctrl Pts',(3.49847119623846,1.,1.35036670892966));
#56290=CARTESIAN_POINT('Ctrl Pts',(3.49861894124827,1.,1.35049736560527));
#56291=CARTESIAN_POINT('Ctrl Pts',(3.49920025459723,1.,1.35080045218587));
#56292=CARTESIAN_POINT('Ctrl Pts',(3.5007660381649,1.,1.35142377279517));
#56293=CARTESIAN_POINT('Ctrl Pts',(3.50408168106261,1.,1.35257032843486));
#56294=CARTESIAN_POINT('Ctrl Pts',(3.50913227059999,1.,1.35419113575956));
#56295=CARTESIAN_POINT('Ctrl Pts',(3.51542230699556,1.,1.35611275237152));
#56296=CARTESIAN_POINT('Ctrl Pts',(3.52261776116748,1.,1.35821701528836));
#56297=CARTESIAN_POINT('Ctrl Pts',(3.530344649616,1.,1.36037259643734));
#56298=CARTESIAN_POINT('Ctrl Pts',(3.53824396424961,1.,1.36245507339307));
#56299=CARTESIAN_POINT('Ctrl Pts',(3.54602591832973,1.,1.36436666257598));
#56300=CARTESIAN_POINT('Ctrl Pts',(3.55353883995949,1.,1.3660614545677));
#56301=CARTESIAN_POINT('Ctrl Pts',(3.56077662028649,1.,1.36754771771233));
#56302=CARTESIAN_POINT('Ctrl Pts',(3.5678208030466,1.,1.36886584973389));
#56303=CARTESIAN_POINT('Ctrl Pts',(3.57479875549486,1.,1.37007229485659));
#56304=CARTESIAN_POINT('Ctrl Pts',(3.58183885982715,1.,1.37122241663062));
#56305=CARTESIAN_POINT('Ctrl Pts',(3.58901853846365,1.,1.37235053660976));
#56306=CARTESIAN_POINT('Ctrl Pts',(3.59634627869048,1.,1.37346320103157));
#56307=CARTESIAN_POINT('Ctrl Pts',(3.60379020123988,1.,1.37455051379623));
#56308=CARTESIAN_POINT('Ctrl Pts',(3.61129546591064,1.,1.37559314436634));
#56309=CARTESIAN_POINT('Ctrl Pts',(3.6188048116042,1.,1.37657053403107));
#56310=CARTESIAN_POINT('Ctrl Pts',(3.62628098665145,1.,1.37746987919881));
#56311=CARTESIAN_POINT('Ctrl Pts',(3.63371727442486,1.,1.37829035457339));
#56312=CARTESIAN_POINT('Ctrl Pts',(3.64112507791141,1.,1.37903818567359));
#56313=CARTESIAN_POINT('Ctrl Pts',(3.64852652756456,1.,1.37972372481603));
#56314=CARTESIAN_POINT('Ctrl Pts',(3.6559455440439,1.,1.38035791051213));
#56315=CARTESIAN_POINT('Ctrl Pts',(3.66339848520857,1.,1.38094856333552));
#56316=CARTESIAN_POINT('Ctrl Pts',(3.67088843112262,1.,1.38149812653868));
#56317=CARTESIAN_POINT('Ctrl Pts',(3.67841038482414,1.,1.3820057429062));
#56318=CARTESIAN_POINT('Ctrl Pts',(3.68595444983837,1.,1.38246852827182));
#56319=CARTESIAN_POINT('Ctrl Pts',(3.69350967899526,1.,1.38288311171651));
#56320=CARTESIAN_POINT('Ctrl Pts',(3.701067921679,1.,1.38324717612865));
#56321=CARTESIAN_POINT('Ctrl Pts',(3.70862680753347,1.,1.38356065402124));
#56322=CARTESIAN_POINT('Ctrl Pts',(3.7161876605181,1.,1.38382489984586));
#56323=CARTESIAN_POINT('Ctrl Pts',(3.72375409358803,1.,1.3840421342895));
#56324=CARTESIAN_POINT('Ctrl Pts',(3.73133035859282,1.,1.38421479111531));
#56325=CARTESIAN_POINT('Ctrl Pts',(3.73891976418104,1.,1.38434489156458));
#56326=CARTESIAN_POINT('Ctrl Pts',(3.74652317167876,1.,1.38443344984394));
#56327=CARTESIAN_POINT('Ctrl Pts',(3.7541397631875,1.,1.38448077997163));
#56328=CARTESIAN_POINT('Ctrl Pts',(3.76176768271367,1.,1.3844867525335));
#56329=CARTESIAN_POINT('Ctrl Pts',(3.76940473185779,1.,1.38445107339518));
#56330=CARTESIAN_POINT('Ctrl Pts',(3.77704902230418,1.,1.38437354551428));
#56331=CARTESIAN_POINT('Ctrl Pts',(3.78469969805082,1.,1.38425435883756));
#56332=CARTESIAN_POINT('Ctrl Pts',(3.79235669640841,1.,1.38409399694566));
#56333=CARTESIAN_POINT('Ctrl Pts',(3.80002044322111,1.,1.38389311766682));
#56334=CARTESIAN_POINT('Ctrl Pts',(3.80769156398411,1.,1.3836524404622));
#56335=CARTESIAN_POINT('Ctrl Pts',(3.81537060817811,1.,1.38337263902782));
#56336=CARTESIAN_POINT('Ctrl Pts',(3.82305771743829,1.,1.38305421262763));
#56337=CARTESIAN_POINT('Ctrl Pts',(3.8307526698229,1.,1.38269750245138));
#56338=CARTESIAN_POINT('Ctrl Pts',(3.83845502790746,1.,1.38230274828822));
#56339=CARTESIAN_POINT('Ctrl Pts',(3.84616425605764,1.,1.38187013346109));
#56340=CARTESIAN_POINT('Ctrl Pts',(3.85387983979481,1.,1.3813998311505));
#56341=CARTESIAN_POINT('Ctrl Pts',(3.86160143043959,1.,1.3808920599299));
#56342=CARTESIAN_POINT('Ctrl Pts',(3.86932885813068,1.,1.38034709213014));
#56343=CARTESIAN_POINT('Ctrl Pts',(3.87706205830532,1.,1.37976523097073));
#56344=CARTESIAN_POINT('Ctrl Pts',(3.88480102249277,1.,1.37914679719383));
#56345=CARTESIAN_POINT('Ctrl Pts',(3.89254574338496,1.,1.3784921128802));
#56346=CARTESIAN_POINT('Ctrl Pts',(3.90029615196727,1.,1.37780148512792));
#56347=CARTESIAN_POINT('Ctrl Pts',(3.90805209523486,1.,1.3770751963402));
#56348=CARTESIAN_POINT('Ctrl Pts',(3.91581337462644,1.,1.37631350505797));
#56349=CARTESIAN_POINT('Ctrl Pts',(3.92357976987672,1.,1.37551664448242));
#56350=CARTESIAN_POINT('Ctrl Pts',(3.93135106761844,1.,1.37468482215751));
#56351=CARTESIAN_POINT('Ctrl Pts',(3.93912709040818,1.,1.37381821967165));
#56352=CARTESIAN_POINT('Ctrl Pts',(3.94690771785133,1.,1.37291699202807));
#56353=CARTESIAN_POINT('Ctrl Pts',(3.95469287280914,1.,1.37198126432386));
#56354=CARTESIAN_POINT('Ctrl Pts',(3.96092458506535,1.,1.3712051561502));
#56355=CARTESIAN_POINT('Ctrl Pts',(3.96560037974645,1.,1.37060761745635));
#56356=CARTESIAN_POINT('Ctrl Pts',(3.9687184694131,1.,1.37020239094614));
#56357=CARTESIAN_POINT('Ctrl Pts',(3.97027773754922,1.,1.36999806084573));
#56358=CARTESIAN_POINT('Origin',(3.97027773754922,0.,1.36999806084573));
#56359=CARTESIAN_POINT('',(4.01728681790024,1.,1.22531898815164));
#56360=CARTESIAN_POINT('Origin',(0.,0.,0.));
#56361=CARTESIAN_POINT('',(3.42859860294378,1.,1.51895082866166));
#56362=CARTESIAN_POINT('Origin',(0.,1.,0.));
#56363=CARTESIAN_POINT('Ctrl Pts',(3.42859860294378,1.,1.51895082866166));
#56364=CARTESIAN_POINT('Ctrl Pts',(3.42859860294378,0.666666666666667,1.51895082866166));
#56365=CARTESIAN_POINT('Ctrl Pts',(3.42859860294378,0.333333333333333,1.51895082866166));
#56366=CARTESIAN_POINT('Ctrl Pts',(3.42859860294378,-0.333333333333333,
1.51895082866166));
#56367=CARTESIAN_POINT('Ctrl Pts',(3.42859860294378,-0.666666666666667,
1.51895082866166));
#56368=CARTESIAN_POINT('Ctrl Pts',(3.42859860294378,-1.,1.51895082866166));
#56369=CARTESIAN_POINT('Ctrl Pts',(3.77614523045147,-1.,1.83867539237861));
#56370=CARTESIAN_POINT('Ctrl Pts',(3.77614523045147,1.,1.83867539237861));
#56371=CARTESIAN_POINT('Ctrl Pts',(3.77518714458232,-1.,1.83742834010821));
#56372=CARTESIAN_POINT('Ctrl Pts',(3.77518714458232,1.,1.83742834010821));
#56373=CARTESIAN_POINT('Ctrl Pts',(3.77326886065484,-1.,1.83493697935064));
#56374=CARTESIAN_POINT('Ctrl Pts',(3.77326886065484,1.,1.83493697935064));
#56375=CARTESIAN_POINT('Ctrl Pts',(3.77038509819777,-1.,1.83120816956515));
#56376=CARTESIAN_POINT('Ctrl Pts',(3.77038509819777,1.,1.83120816956515));
#56377=CARTESIAN_POINT('Ctrl Pts',(3.76652740355856,-1.,1.82625289221933));
#56378=CARTESIAN_POINT('Ctrl Pts',(3.76652740355856,1.,1.82625289221933));
#56379=CARTESIAN_POINT('Ctrl Pts',(3.76168412709652,-1.,1.82008629694924));
#56380=CARTESIAN_POINT('Ctrl Pts',(3.76168412709652,1.,1.82008629694924));
#56381=CARTESIAN_POINT('Ctrl Pts',(3.75681965683995,-1.,1.81394729834032));
#56382=CARTESIAN_POINT('Ctrl Pts',(3.75681965683995,1.,1.81394729834032));
#56383=CARTESIAN_POINT('Ctrl Pts',(3.75193395888069,-1.,1.80783603939662));
#56384=CARTESIAN_POINT('Ctrl Pts',(3.75193395888069,1.,1.80783603939662));
#56385=CARTESIAN_POINT('Ctrl Pts',(3.74702700874954,-1.,1.80175271485519));
#56386=CARTESIAN_POINT('Ctrl Pts',(3.74702700874954,1.,1.80175271485519));
#56387=CARTESIAN_POINT('Ctrl Pts',(3.74209880351667,-1.,1.79569757859041));
#56388=CARTESIAN_POINT('Ctrl Pts',(3.74209880351667,1.,1.79569757859041));
#56389=CARTESIAN_POINT('Ctrl Pts',(3.73714934729962,-1.,1.78967092823139));
#56390=CARTESIAN_POINT('Ctrl Pts',(3.73714934729962,1.,1.78967092823139));
#56391=CARTESIAN_POINT('Ctrl Pts',(3.73217863095022,-1.,1.78367308442682));
#56392=CARTESIAN_POINT('Ctrl Pts',(3.73217863095022,1.,1.78367308442682));
#56393=CARTESIAN_POINT('Ctrl Pts',(3.72718661205504,-1.,1.77770437039606));
#56394=CARTESIAN_POINT('Ctrl Pts',(3.72718661205504,1.,1.77770437039606));
#56395=CARTESIAN_POINT('Ctrl Pts',(3.72217319911429,-1.,1.77176509401846));
#56396=CARTESIAN_POINT('Ctrl Pts',(3.72217319911429,1.,1.77176509401846));
#56397=CARTESIAN_POINT('Ctrl Pts',(3.71713822377675,-1.,1.76585552124549));
#56398=CARTESIAN_POINT('Ctrl Pts',(3.71713822377675,1.,1.76585552124549));
#56399=CARTESIAN_POINT('Ctrl Pts',(3.71208146346454,-1.,1.75997588499021));
#56400=CARTESIAN_POINT('Ctrl Pts',(3.71208146346454,1.,1.75997588499021));
#56401=CARTESIAN_POINT('Ctrl Pts',(3.70700269736876,-1.,1.75412641804148));
#56402=CARTESIAN_POINT('Ctrl Pts',(3.70700269736876,1.,1.75412641804148));
#56403=CARTESIAN_POINT('Ctrl Pts',(3.70190175673422,-1.,1.74830738046092));
#56404=CARTESIAN_POINT('Ctrl Pts',(3.70190175673422,1.,1.74830738046092));
#56405=CARTESIAN_POINT('Ctrl Pts',(3.6967785691046,-1.,1.74251908492589));
#56406=CARTESIAN_POINT('Ctrl Pts',(3.6967785691046,1.,1.74251908492589));
#56407=CARTESIAN_POINT('Ctrl Pts',(3.69163322647906,-1.,1.73676193254493));
#56408=CARTESIAN_POINT('Ctrl Pts',(3.69163322647906,1.,1.73676193254493));
#56409=CARTESIAN_POINT('Ctrl Pts',(3.68646597019188,-1.,1.73103640956647));
#56410=CARTESIAN_POINT('Ctrl Pts',(3.68646597019188,1.,1.73103640956647));
#56411=CARTESIAN_POINT('Ctrl Pts',(3.68127704936472,-1.,1.72534302437003));
#56412=CARTESIAN_POINT('Ctrl Pts',(3.68127704936472,1.,1.72534302437003));
#56413=CARTESIAN_POINT('Ctrl Pts',(3.67606660374665,-1.,1.71968225581787));
#56414=CARTESIAN_POINT('Ctrl Pts',(3.67606660374665,1.,1.71968225581787));
#56415=CARTESIAN_POINT('Ctrl Pts',(3.67083454901629,-1.,1.71405450210392));
#56416=CARTESIAN_POINT('Ctrl Pts',(3.67083454901629,1.,1.71405450210392));
#56417=CARTESIAN_POINT('Ctrl Pts',(3.6655804319893,-1.,1.70846001610983));
#56418=CARTESIAN_POINT('Ctrl Pts',(3.6655804319893,1.,1.70846001610983));
#56419=CARTESIAN_POINT('Ctrl Pts',(3.6603033877491,-1.,1.70289888566904));
#56420=CARTESIAN_POINT('Ctrl Pts',(3.6603033877491,1.,1.70289888566904));
#56421=CARTESIAN_POINT('Ctrl Pts',(3.65500246526798,-1.,1.69737117722559));
#56422=CARTESIAN_POINT('Ctrl Pts',(3.65500246526798,1.,1.69737117722559));
#56423=CARTESIAN_POINT('Ctrl Pts',(3.64967689827393,-1.,1.691877054817));
#56424=CARTESIAN_POINT('Ctrl Pts',(3.64967689827393,1.,1.691877054817));
#56425=CARTESIAN_POINT('Ctrl Pts',(3.64432638915199,-1.,1.68641690471455));
#56426=CARTESIAN_POINT('Ctrl Pts',(3.64432638915199,1.,1.68641690471455));
#56427=CARTESIAN_POINT('Ctrl Pts',(3.63895140887443,-1.,1.68099146651577));
#56428=CARTESIAN_POINT('Ctrl Pts',(3.63895140887443,1.,1.68099146651577));
#56429=CARTESIAN_POINT('Ctrl Pts',(3.63355343201211,-1.,1.67560193613145));
#56430=CARTESIAN_POINT('Ctrl Pts',(3.63355343201211,1.,1.67560193613145));
#56431=CARTESIAN_POINT('Ctrl Pts',(3.62813422105257,-1.,1.67024966008037));
#56432=CARTESIAN_POINT('Ctrl Pts',(3.62813422105257,1.,1.67024966008037));
#56433=CARTESIAN_POINT('Ctrl Pts',(3.62269517989104,-1.,1.66493585923853));
#56434=CARTESIAN_POINT('Ctrl Pts',(3.62269517989104,1.,1.66493585923853));
#56435=CARTESIAN_POINT('Ctrl Pts',(3.61723666482457,-1.,1.65966133399186));
#56436=CARTESIAN_POINT('Ctrl Pts',(3.61723666482457,1.,1.65966133399186));
#56437=CARTESIAN_POINT('Ctrl Pts',(3.61175734965129,-1.,1.65442619244327));
#56438=CARTESIAN_POINT('Ctrl Pts',(3.61175734965129,1.,1.65442619244327));
#56439=CARTESIAN_POINT('Ctrl Pts',(3.60625346556992,-1.,1.64922952425833));
#56440=CARTESIAN_POINT('Ctrl Pts',(3.60625346556992,1.,1.64922952425833));
#56441=CARTESIAN_POINT('Ctrl Pts',(3.6007202851384,-1.,1.6440700438558));
#56442=CARTESIAN_POINT('Ctrl Pts',(3.6007202851384,1.,1.6440700438558));
#56443=CARTESIAN_POINT('Ctrl Pts',(3.59515368334887,-1.,1.63894676675349));
#56444=CARTESIAN_POINT('Ctrl Pts',(3.59515368334887,1.,1.63894676675349));
#56445=CARTESIAN_POINT('Ctrl Pts',(3.58955176627876,-1.,1.63385971451259));
#56446=CARTESIAN_POINT('Ctrl Pts',(3.58955176627876,1.,1.63385971451259));
#56447=CARTESIAN_POINT('Ctrl Pts',(3.5839162577435,-1.,1.62881051550748));
#56448=CARTESIAN_POINT('Ctrl Pts',(3.5839162577435,1.,1.62881051550748));
#56449=CARTESIAN_POINT('Ctrl Pts',(3.57825455954405,-1.,1.62380329464851));
#56450=CARTESIAN_POINT('Ctrl Pts',(3.57825455954405,1.,1.62380329464851));
#56451=CARTESIAN_POINT('Ctrl Pts',(3.57257679609826,-1.,1.61884340915412));
#56452=CARTESIAN_POINT('Ctrl Pts',(3.57257679609826,1.,1.61884340915412));
#56453=CARTESIAN_POINT('Ctrl Pts',(3.56689200468404,-1.,1.61393581747522));
#56454=CARTESIAN_POINT('Ctrl Pts',(3.56689200468404,1.,1.61393581747522));
#56455=CARTESIAN_POINT('Ctrl Pts',(3.56120432482986,-1.,1.60908344685459));
#56456=CARTESIAN_POINT('Ctrl Pts',(3.56120432482986,1.,1.60908344685459));
#56457=CARTESIAN_POINT('Ctrl Pts',(3.55550985096117,-1.,1.60428584699848));
#56458=CARTESIAN_POINT('Ctrl Pts',(3.55550985096117,1.,1.60428584699848));
#56459=CARTESIAN_POINT('Ctrl Pts',(3.54979148634426,-1.,1.59953698113444));
#56460=CARTESIAN_POINT('Ctrl Pts',(3.54979148634426,1.,1.59953698113444));
#56461=CARTESIAN_POINT('Ctrl Pts',(3.544024581823,-1.,1.5948276694975));
#56462=CARTESIAN_POINT('Ctrl Pts',(3.544024581823,1.,1.5948276694975));
#56463=CARTESIAN_POINT('Ctrl Pts',(3.53818616861045,-1.,1.59014958368725));
#56464=CARTESIAN_POINT('Ctrl Pts',(3.53818616861045,1.,1.59014958368725));
#56465=CARTESIAN_POINT('Ctrl Pts',(3.53226378147068,-1.,1.58549906268083));
#56466=CARTESIAN_POINT('Ctrl Pts',(3.53226378147068,1.,1.58549906268083));
#56467=CARTESIAN_POINT('Ctrl Pts',(3.52626275334899,-1.,1.58088027227856));
#56468=CARTESIAN_POINT('Ctrl Pts',(3.52626275334899,1.,1.58088027227856));
#56469=CARTESIAN_POINT('Ctrl Pts',(3.52021847865961,-1.,1.5763104998818));
#56470=CARTESIAN_POINT('Ctrl Pts',(3.52021847865961,1.,1.5763104998818));
#56471=CARTESIAN_POINT('Ctrl Pts',(3.51418598431733,-1.,1.57181569799774));
#56472=CARTESIAN_POINT('Ctrl Pts',(3.51418598431733,1.,1.57181569799774));
#56473=CARTESIAN_POINT('Ctrl Pts',(3.50821771695427,-1.,1.56742097575041));
#56474=CARTESIAN_POINT('Ctrl Pts',(3.50821771695427,1.,1.56742097575041));
#56475=CARTESIAN_POINT('Ctrl Pts',(3.50234321621607,-1.,1.56314187758689));
#56476=CARTESIAN_POINT('Ctrl Pts',(3.50234321621607,1.,1.56314187758689));
#56477=CARTESIAN_POINT('Ctrl Pts',(3.49655185179623,-1.,1.55897703097859));
#56478=CARTESIAN_POINT('Ctrl Pts',(3.49655185179623,1.,1.55897703097859));
#56479=CARTESIAN_POINT('Ctrl Pts',(3.49076460877317,-1.,1.5548959590107));
#56480=CARTESIAN_POINT('Ctrl Pts',(3.49076460877317,1.,1.5548959590107));
#56481=CARTESIAN_POINT('Ctrl Pts',(3.48485155928414,-1.,1.55084702970382));
#56482=CARTESIAN_POINT('Ctrl Pts',(3.48485155928414,1.,1.55084702970382));
#56483=CARTESIAN_POINT('Ctrl Pts',(3.47868272898599,-1.,1.54678009290207));
#56484=CARTESIAN_POINT('Ctrl Pts',(3.47868272898599,1.,1.54678009290207));
#56485=CARTESIAN_POINT('Ctrl Pts',(3.47217189224576,-1.,1.54266605398152));
#56486=CARTESIAN_POINT('Ctrl Pts',(3.47217189224576,1.,1.54266605398152));
#56487=CARTESIAN_POINT('Ctrl Pts',(3.46531752207222,-1.,1.53851507915533));
#56488=CARTESIAN_POINT('Ctrl Pts',(3.46531752207222,1.,1.53851507915533));
#56489=CARTESIAN_POINT('Ctrl Pts',(3.45825932955273,-1.,1.53440195378902));
#56490=CARTESIAN_POINT('Ctrl Pts',(3.45825932955273,1.,1.53440195378902));
#56491=CARTESIAN_POINT('Ctrl Pts',(3.45127136828667,-1.,1.530462444618));
#56492=CARTESIAN_POINT('Ctrl Pts',(3.45127136828667,1.,1.530462444618));
#56493=CARTESIAN_POINT('Ctrl Pts',(3.44469547527,-1.,1.52686242875717));
#56494=CARTESIAN_POINT('Ctrl Pts',(3.44469547527,1.,1.52686242875717));
#56495=CARTESIAN_POINT('Ctrl Pts',(3.43888895974182,-1.,1.52377348950429));
#56496=CARTESIAN_POINT('Ctrl Pts',(3.43888895974182,1.,1.52377348950429));
#56497=CARTESIAN_POINT('Ctrl Pts',(3.43417156977749,-1.,1.52134826724227));
#56498=CARTESIAN_POINT('Ctrl Pts',(3.43417156977749,1.,1.52134826724227));
#56499=CARTESIAN_POINT('Ctrl Pts',(3.43076036253384,-1.,1.51969006980792));
#56500=CARTESIAN_POINT('Ctrl Pts',(3.43076036253384,1.,1.51969006980792));
#56501=CARTESIAN_POINT('Ctrl Pts',(3.42915787669388,-1.,1.51901585838879));
#56502=CARTESIAN_POINT('Ctrl Pts',(3.42915787669388,1.,1.51901585838879));
#56503=CARTESIAN_POINT('Ctrl Pts',(3.42860527148835,-1.,1.51888450659497));
#56504=CARTESIAN_POINT('Ctrl Pts',(3.42860527148835,1.,1.51888450659497));
#56505=CARTESIAN_POINT('Ctrl Pts',(3.42852521763648,-1.,1.51896318668306));
#56506=CARTESIAN_POINT('Ctrl Pts',(3.42852521763648,1.,1.51896318668306));
#56507=CARTESIAN_POINT('Ctrl Pts',(3.42855728381368,-1.,1.519044091397));
#56508=CARTESIAN_POINT('Ctrl Pts',(3.42855728381368,1.,1.519044091397));
#56509=CARTESIAN_POINT('',(3.77614523045147,1.,1.83867539237861));
#56510=CARTESIAN_POINT('Ctrl Pts',(3.77614523045147,1.,1.83867539237861));
#56511=CARTESIAN_POINT('Ctrl Pts',(3.77518714458232,1.,1.83742834010821));
#56512=CARTESIAN_POINT('Ctrl Pts',(3.77326886065484,1.,1.83493697935064));
#56513=CARTESIAN_POINT('Ctrl Pts',(3.77038509819777,1.,1.83120816956515));
#56514=CARTESIAN_POINT('Ctrl Pts',(3.76652740355856,1.,1.82625289221933));
#56515=CARTESIAN_POINT('Ctrl Pts',(3.76168412709652,1.,1.82008629694924));
#56516=CARTESIAN_POINT('Ctrl Pts',(3.75681965683995,1.,1.81394729834032));
#56517=CARTESIAN_POINT('Ctrl Pts',(3.75193395888069,1.,1.80783603939662));
#56518=CARTESIAN_POINT('Ctrl Pts',(3.74702700874954,1.,1.80175271485519));
#56519=CARTESIAN_POINT('Ctrl Pts',(3.74209880351667,1.,1.79569757859041));
#56520=CARTESIAN_POINT('Ctrl Pts',(3.73714934729962,1.,1.78967092823139));
#56521=CARTESIAN_POINT('Ctrl Pts',(3.73217863095022,1.,1.78367308442682));
#56522=CARTESIAN_POINT('Ctrl Pts',(3.72718661205504,1.,1.77770437039606));
#56523=CARTESIAN_POINT('Ctrl Pts',(3.72217319911429,1.,1.77176509401846));
#56524=CARTESIAN_POINT('Ctrl Pts',(3.71713822377675,1.,1.76585552124549));
#56525=CARTESIAN_POINT('Ctrl Pts',(3.71208146346454,1.,1.75997588499021));
#56526=CARTESIAN_POINT('Ctrl Pts',(3.70700269736876,1.,1.75412641804148));
#56527=CARTESIAN_POINT('Ctrl Pts',(3.70190175673422,1.,1.74830738046092));
#56528=CARTESIAN_POINT('Ctrl Pts',(3.6967785691046,1.,1.74251908492589));
#56529=CARTESIAN_POINT('Ctrl Pts',(3.69163322647906,1.,1.73676193254493));
#56530=CARTESIAN_POINT('Ctrl Pts',(3.68646597019188,1.,1.73103640956647));
#56531=CARTESIAN_POINT('Ctrl Pts',(3.68127704936472,1.,1.72534302437003));
#56532=CARTESIAN_POINT('Ctrl Pts',(3.67606660374665,1.,1.71968225581787));
#56533=CARTESIAN_POINT('Ctrl Pts',(3.67083454901629,1.,1.71405450210392));
#56534=CARTESIAN_POINT('Ctrl Pts',(3.6655804319893,1.,1.70846001610983));
#56535=CARTESIAN_POINT('Ctrl Pts',(3.6603033877491,1.,1.70289888566904));
#56536=CARTESIAN_POINT('Ctrl Pts',(3.65500246526798,1.,1.69737117722559));
#56537=CARTESIAN_POINT('Ctrl Pts',(3.64967689827393,1.,1.691877054817));
#56538=CARTESIAN_POINT('Ctrl Pts',(3.64432638915199,1.,1.68641690471455));
#56539=CARTESIAN_POINT('Ctrl Pts',(3.63895140887443,1.,1.68099146651577));
#56540=CARTESIAN_POINT('Ctrl Pts',(3.63355343201211,1.,1.67560193613145));
#56541=CARTESIAN_POINT('Ctrl Pts',(3.62813422105257,1.,1.67024966008037));
#56542=CARTESIAN_POINT('Ctrl Pts',(3.62269517989104,1.,1.66493585923853));
#56543=CARTESIAN_POINT('Ctrl Pts',(3.61723666482457,1.,1.65966133399186));
#56544=CARTESIAN_POINT('Ctrl Pts',(3.61175734965129,1.,1.65442619244327));
#56545=CARTESIAN_POINT('Ctrl Pts',(3.60625346556992,1.,1.64922952425833));
#56546=CARTESIAN_POINT('Ctrl Pts',(3.6007202851384,1.,1.6440700438558));
#56547=CARTESIAN_POINT('Ctrl Pts',(3.59515368334887,1.,1.63894676675349));
#56548=CARTESIAN_POINT('Ctrl Pts',(3.58955176627876,1.,1.63385971451259));
#56549=CARTESIAN_POINT('Ctrl Pts',(3.5839162577435,1.,1.62881051550748));
#56550=CARTESIAN_POINT('Ctrl Pts',(3.57825455954405,1.,1.62380329464851));
#56551=CARTESIAN_POINT('Ctrl Pts',(3.57257679609826,1.,1.61884340915412));
#56552=CARTESIAN_POINT('Ctrl Pts',(3.56689200468404,1.,1.61393581747522));
#56553=CARTESIAN_POINT('Ctrl Pts',(3.56120432482986,1.,1.60908344685459));
#56554=CARTESIAN_POINT('Ctrl Pts',(3.55550985096117,1.,1.60428584699848));
#56555=CARTESIAN_POINT('Ctrl Pts',(3.54979148634426,1.,1.59953698113444));
#56556=CARTESIAN_POINT('Ctrl Pts',(3.544024581823,1.,1.5948276694975));
#56557=CARTESIAN_POINT('Ctrl Pts',(3.53818616861045,1.,1.59014958368725));
#56558=CARTESIAN_POINT('Ctrl Pts',(3.53226378147068,1.,1.58549906268083));
#56559=CARTESIAN_POINT('Ctrl Pts',(3.52626275334899,1.,1.58088027227856));
#56560=CARTESIAN_POINT('Ctrl Pts',(3.52021847865961,1.,1.5763104998818));
#56561=CARTESIAN_POINT('Ctrl Pts',(3.51418598431733,1.,1.57181569799774));
#56562=CARTESIAN_POINT('Ctrl Pts',(3.50821771695427,1.,1.56742097575041));
#56563=CARTESIAN_POINT('Ctrl Pts',(3.50234321621607,1.,1.56314187758689));
#56564=CARTESIAN_POINT('Ctrl Pts',(3.49655185179623,1.,1.55897703097859));
#56565=CARTESIAN_POINT('Ctrl Pts',(3.49076460877317,1.,1.5548959590107));
#56566=CARTESIAN_POINT('Ctrl Pts',(3.48485155928414,1.,1.55084702970382));
#56567=CARTESIAN_POINT('Ctrl Pts',(3.47868272898599,1.,1.54678009290207));
#56568=CARTESIAN_POINT('Ctrl Pts',(3.47217189224576,1.,1.54266605398152));
#56569=CARTESIAN_POINT('Ctrl Pts',(3.46531752207222,1.,1.53851507915533));
#56570=CARTESIAN_POINT('Ctrl Pts',(3.45825932955273,1.,1.53440195378902));
#56571=CARTESIAN_POINT('Ctrl Pts',(3.45127136828667,1.,1.530462444618));
#56572=CARTESIAN_POINT('Ctrl Pts',(3.44469547527,1.,1.52686242875717));
#56573=CARTESIAN_POINT('Ctrl Pts',(3.43888895974182,1.,1.52377348950429));
#56574=CARTESIAN_POINT('Ctrl Pts',(3.43417156977749,1.,1.52134826724227));
#56575=CARTESIAN_POINT('Ctrl Pts',(3.4310163189349,1.,1.5198144909343));
#56576=CARTESIAN_POINT('Ctrl Pts',(3.42946838852728,1.,1.51914806898539));
#56577=CARTESIAN_POINT('Ctrl Pts',(3.42884302333978,1.,1.51895133295017));
#56578=CARTESIAN_POINT('Ctrl Pts',(3.42864616361967,1.,1.51893924967231));
#56579=CARTESIAN_POINT('Ctrl Pts',(3.42859860294378,1.,1.51895082866166));
#56580=CARTESIAN_POINT('',(3.77614523045147,0.,1.83867539237861));
#56581=CARTESIAN_POINT('Ctrl Pts',(3.24418789321065,-1.,1.88088939428811));
#56582=CARTESIAN_POINT('Ctrl Pts',(3.24418789321065,1.,1.88088939428811));
#56583=CARTESIAN_POINT('Ctrl Pts',(3.24410359189733,-1.,1.8809110068042));
#56584=CARTESIAN_POINT('Ctrl Pts',(3.24410359189733,1.,1.8809110068042));
#56585=CARTESIAN_POINT('Ctrl Pts',(3.24408699284449,-1.,1.8810220187274));
#56586=CARTESIAN_POINT('Ctrl Pts',(3.24408699284449,1.,1.8810220187274));
#56587=CARTESIAN_POINT('Ctrl Pts',(3.24451807186964,-1.,1.88139187908347));
#56588=CARTESIAN_POINT('Ctrl Pts',(3.24451807186964,1.,1.88139187908347));
#56589=CARTESIAN_POINT('Ctrl Pts',(3.24600543790876,-1.,1.88229202583187));
#56590=CARTESIAN_POINT('Ctrl Pts',(3.24600543790876,1.,1.88229202583187));
#56591=CARTESIAN_POINT('Ctrl Pts',(3.24935200512055,-1.,1.88407708646435));
#56592=CARTESIAN_POINT('Ctrl Pts',(3.24935200512055,1.,1.88407708646435));
#56593=CARTESIAN_POINT('Ctrl Pts',(3.25408686339298,-1.,1.88646802523372));
#56594=CARTESIAN_POINT('Ctrl Pts',(3.25408686339298,1.,1.88646802523372));
#56595=CARTESIAN_POINT('Ctrl Pts',(3.2599988519361,-1.,1.88934996203508));
#56596=CARTESIAN_POINT('Ctrl Pts',(3.2599988519361,1.,1.88934996203508));
#56597=CARTESIAN_POINT('Ctrl Pts',(3.2667765388833,-1.,1.89255393500769));
#56598=CARTESIAN_POINT('Ctrl Pts',(3.2667765388833,1.,1.89255393500769));
#56599=CARTESIAN_POINT('Ctrl Pts',(3.27407108932908,-1.,1.89589172903662));
#56600=CARTESIAN_POINT('Ctrl Pts',(3.27407108932908,1.,1.89589172903662));
#56601=CARTESIAN_POINT('Ctrl Pts',(3.28154737912287,-1.,1.89918429230425));
#56602=CARTESIAN_POINT('Ctrl Pts',(3.28154737912287,1.,1.89918429230425));
#56603=CARTESIAN_POINT('Ctrl Pts',(3.28893448600364,-1.,1.9022897124757));
#56604=CARTESIAN_POINT('Ctrl Pts',(3.28893448600364,1.,1.9022897124757));
#56605=CARTESIAN_POINT('Ctrl Pts',(3.29608978722258,-1.,1.9051389186417));
#56606=CARTESIAN_POINT('Ctrl Pts',(3.29608978722258,1.,1.9051389186417));
#56607=CARTESIAN_POINT('Ctrl Pts',(3.30300595568341,-1.,1.90773912171424));
#56608=CARTESIAN_POINT('Ctrl Pts',(3.30300595568341,1.,1.90773912171424));
#56609=CARTESIAN_POINT('Ctrl Pts',(3.30975721158694,-1.,1.91014297830502));
#56610=CARTESIAN_POINT('Ctrl Pts',(3.30975721158694,1.,1.91014297830502));
#56611=CARTESIAN_POINT('Ctrl Pts',(3.31646052426395,-1.,1.91242616234459));
#56612=CARTESIAN_POINT('Ctrl Pts',(3.31646052426395,1.,1.91242616234459));
#56613=CARTESIAN_POINT('Ctrl Pts',(3.32323403454507,-1.,1.91466343916612));
#56614=CARTESIAN_POINT('Ctrl Pts',(3.32323403454507,1.,1.91466343916612));
#56615=CARTESIAN_POINT('Ctrl Pts',(3.33014884257812,-1.,1.91690081930297));
#56616=CARTESIAN_POINT('Ctrl Pts',(3.33014884257812,1.,1.91690081930297));
#56617=CARTESIAN_POINT('Ctrl Pts',(3.33721230709948,-1.,1.91914609610173));
#56618=CARTESIAN_POINT('Ctrl Pts',(3.33721230709948,1.,1.91914609610173));
#56619=CARTESIAN_POINT('Ctrl Pts',(3.34439448941915,-1.,1.92138450828378));
#56620=CARTESIAN_POINT('Ctrl Pts',(3.34439448941915,1.,1.92138450828378));
#56621=CARTESIAN_POINT('Ctrl Pts',(3.35164424847206,-1.,1.92358838440518));
#56622=CARTESIAN_POINT('Ctrl Pts',(3.35164424847206,1.,1.92358838440518));
#56623=CARTESIAN_POINT('Ctrl Pts',(3.35890824422976,-1.,1.92572846125763));
#56624=CARTESIAN_POINT('Ctrl Pts',(3.35890824422976,1.,1.92572846125763));
#56625=CARTESIAN_POINT('Ctrl Pts',(3.36615168657597,-1.,1.92778626543803));
#56626=CARTESIAN_POINT('Ctrl Pts',(3.36615168657597,1.,1.92778626543803));
#56627=CARTESIAN_POINT('Ctrl Pts',(3.37336807068078,-1.,1.92975993109897));
#56628=CARTESIAN_POINT('Ctrl Pts',(3.37336807068078,1.,1.92975993109897));
#56629=CARTESIAN_POINT('Ctrl Pts',(3.38056768525577,-1.,1.93165739093292));
#56630=CARTESIAN_POINT('Ctrl Pts',(3.38056768525577,1.,1.93165739093292));
#56631=CARTESIAN_POINT('Ctrl Pts',(3.38777076883267,-1.,1.93349233176794));
#56632=CARTESIAN_POINT('Ctrl Pts',(3.38777076883267,1.,1.93349233176794));
#56633=CARTESIAN_POINT('Ctrl Pts',(3.39499923640789,-1.,1.93527929945982));
#56634=CARTESIAN_POINT('Ctrl Pts',(3.39499923640789,1.,1.93527929945982));
#56635=CARTESIAN_POINT('Ctrl Pts',(3.40226802104093,-1.,1.93702857723089));
#56636=CARTESIAN_POINT('Ctrl Pts',(3.40226802104093,1.,1.93702857723089));
#56637=CARTESIAN_POINT('Ctrl Pts',(3.40957978266622,-1.,1.93874306008132));
#56638=CARTESIAN_POINT('Ctrl Pts',(3.40957978266622,1.,1.93874306008132));
#56639=CARTESIAN_POINT('Ctrl Pts',(3.41692971994082,-1.,1.94042111965237));
#56640=CARTESIAN_POINT('Ctrl Pts',(3.41692971994082,1.,1.94042111965237));
#56641=CARTESIAN_POINT('Ctrl Pts',(3.42430850941497,-1.,1.94205835913692));
#56642=CARTESIAN_POINT('Ctrl Pts',(3.42430850941497,1.,1.94205835913692));
#56643=CARTESIAN_POINT('Ctrl Pts',(3.43170586602436,-1.,1.94364973660285));
#56644=CARTESIAN_POINT('Ctrl Pts',(3.43170586602436,1.,1.94364973660285));
#56645=CARTESIAN_POINT('Ctrl Pts',(3.43911410197693,-1.,1.94519168842883));
#56646=CARTESIAN_POINT('Ctrl Pts',(3.43911410197693,1.,1.94519168842883));
#56647=CARTESIAN_POINT('Ctrl Pts',(3.44653088665685,-1.,1.94668377715332));
#56648=CARTESIAN_POINT('Ctrl Pts',(3.44653088665685,1.,1.94668377715332));
#56649=CARTESIAN_POINT('Ctrl Pts',(3.45395731584051,-1.,1.94812754766524));
#56650=CARTESIAN_POINT('Ctrl Pts',(3.45395731584051,1.,1.94812754766524));
#56651=CARTESIAN_POINT('Ctrl Pts',(3.46139661060959,-1.,1.94952575850196));
#56652=CARTESIAN_POINT('Ctrl Pts',(3.46139661060959,1.,1.94952575850196));
#56653=CARTESIAN_POINT('Ctrl Pts',(3.4688525897419,-1.,1.95088147859876));
#56654=CARTESIAN_POINT('Ctrl Pts',(3.4688525897419,1.,1.95088147859876));
#56655=CARTESIAN_POINT('Ctrl Pts',(3.47632820495926,-1.,1.95219722189878));
#56656=CARTESIAN_POINT('Ctrl Pts',(3.47632820495926,1.,1.95219722189878));
#56657=CARTESIAN_POINT('Ctrl Pts',(3.48382414832648,-1.,1.95347412486316));
#56658=CARTESIAN_POINT('Ctrl Pts',(3.48382414832648,1.,1.95347412486316));
#56659=CARTESIAN_POINT('Ctrl Pts',(3.49133956289154,-1.,1.95471236969653));
#56660=CARTESIAN_POINT('Ctrl Pts',(3.49133956289154,1.,1.95471236969653));
#56661=CARTESIAN_POINT('Ctrl Pts',(3.49887263575602,-1.,1.9559115382367));
#56662=CARTESIAN_POINT('Ctrl Pts',(3.49887263575602,1.,1.9559115382367));
#56663=CARTESIAN_POINT('Ctrl Pts',(3.50642124159913,-1.,1.95707099606514));
#56664=CARTESIAN_POINT('Ctrl Pts',(3.50642124159913,1.,1.95707099606514));
#56665=CARTESIAN_POINT('Ctrl Pts',(3.51398354617772,-1.,1.95819025316768));
#56666=CARTESIAN_POINT('Ctrl Pts',(3.51398354617772,1.,1.95819025316768));
#56667=CARTESIAN_POINT('Ctrl Pts',(3.52155867431438,-1.,1.95926936324436));
#56668=CARTESIAN_POINT('Ctrl Pts',(3.52155867431438,1.,1.95926936324436));
#56669=CARTESIAN_POINT('Ctrl Pts',(3.52914648844289,-1.,1.96030879411534));
#56670=CARTESIAN_POINT('Ctrl Pts',(3.52914648844289,1.,1.96030879411534));
#56671=CARTESIAN_POINT('Ctrl Pts',(3.53674730625759,-1.,1.96130926212661));
#56672=CARTESIAN_POINT('Ctrl Pts',(3.53674730625759,1.,1.96130926212661));
#56673=CARTESIAN_POINT('Ctrl Pts',(3.54436163300425,-1.,1.96227157573058));
#56674=CARTESIAN_POINT('Ctrl Pts',(3.54436163300425,1.,1.96227157573058));
#56675=CARTESIAN_POINT('Ctrl Pts',(3.55198990600929,-1.,1.96319648628667));
#56676=CARTESIAN_POINT('Ctrl Pts',(3.55198990600929,1.,1.96319648628667));
#56677=CARTESIAN_POINT('Ctrl Pts',(3.55963218706201,-1.,1.96408450906868));
#56678=CARTESIAN_POINT('Ctrl Pts',(3.55963218706201,1.,1.96408450906868));
#56679=CARTESIAN_POINT('Ctrl Pts',(3.56728820357933,-1.,1.96493594634643));
#56680=CARTESIAN_POINT('Ctrl Pts',(3.56728820357933,1.,1.96493594634643));
#56681=CARTESIAN_POINT('Ctrl Pts',(3.57495748601088,-1.,1.96575096652857));
#56682=CARTESIAN_POINT('Ctrl Pts',(3.57495748601088,1.,1.96575096652857));
#56683=CARTESIAN_POINT('Ctrl Pts',(3.58263947663884,-1.,1.9665296668894));
#56684=CARTESIAN_POINT('Ctrl Pts',(3.58263947663884,1.,1.9665296668894));
#56685=CARTESIAN_POINT('Ctrl Pts',(3.5903336402273,-1.,1.96727213799507));
#56686=CARTESIAN_POINT('Ctrl Pts',(3.5903336402273,1.,1.96727213799507));
#56687=CARTESIAN_POINT('Ctrl Pts',(3.59803959819725,-1.,1.96797854118257));
#56688=CARTESIAN_POINT('Ctrl Pts',(3.59803959819725,1.,1.96797854118257));
#56689=CARTESIAN_POINT('Ctrl Pts',(3.60575714017676,-1.,1.96864911885775));
#56690=CARTESIAN_POINT('Ctrl Pts',(3.60575714017676,1.,1.96864911885775));
#56691=CARTESIAN_POINT('Ctrl Pts',(3.61348615496393,-1.,1.96928416040712));
#56692=CARTESIAN_POINT('Ctrl Pts',(3.61348615496393,1.,1.96928416040712));
#56693=CARTESIAN_POINT('Ctrl Pts',(3.62122658401722,-1.,1.96988398129888));
#56694=CARTESIAN_POINT('Ctrl Pts',(3.62122658401722,1.,1.96988398129888));
#56695=CARTESIAN_POINT('Ctrl Pts',(3.62897836973397,-1.,1.97044889850518));
#56696=CARTESIAN_POINT('Ctrl Pts',(3.62897836973397,1.,1.97044889850518));
#56697=CARTESIAN_POINT('Ctrl Pts',(3.63674139590853,-1.,1.97097920454698));
#56698=CARTESIAN_POINT('Ctrl Pts',(3.63674139590853,1.,1.97097920454698));
#56699=CARTESIAN_POINT('Ctrl Pts',(3.64451546724221,-1.,1.97147515441539));
#56700=CARTESIAN_POINT('Ctrl Pts',(3.64451546724221,1.,1.97147515441539));
#56701=CARTESIAN_POINT('Ctrl Pts',(3.65230034717364,-1.,1.97193697240645));
#56702=CARTESIAN_POINT('Ctrl Pts',(3.65230034717364,1.,1.97193697240645));
#56703=CARTESIAN_POINT('Ctrl Pts',(3.66009578166865,-1.,1.97236485439317));
#56704=CARTESIAN_POINT('Ctrl Pts',(3.66009578166865,1.,1.97236485439317));
#56705=CARTESIAN_POINT('Ctrl Pts',(3.66790152751984,-1.,1.9727589719863));
#56706=CARTESIAN_POINT('Ctrl Pts',(3.66790152751984,1.,1.9727589719863));
#56707=CARTESIAN_POINT('Ctrl Pts',(3.67571738106175,-1.,1.97311947678035));
#56708=CARTESIAN_POINT('Ctrl Pts',(3.67571738106175,1.,1.97311947678035));
#56709=CARTESIAN_POINT('Ctrl Pts',(3.68354319913416,-1.,1.97344650303631));
#56710=CARTESIAN_POINT('Ctrl Pts',(3.68354319913416,1.,1.97344650303631));
#56711=CARTESIAN_POINT('Ctrl Pts',(3.69137888597855,-1.,1.97374016224397));
#56712=CARTESIAN_POINT('Ctrl Pts',(3.69137888597855,1.,1.97374016224397));
#56713=CARTESIAN_POINT('Ctrl Pts',(3.69765528558292,-1.,1.97394846382289));
#56714=CARTESIAN_POINT('Ctrl Pts',(3.69765528558292,1.,1.97394846382289));
#56715=CARTESIAN_POINT('Ctrl Pts',(3.70236698911837,-1.,1.97408973726149));
#56716=CARTESIAN_POINT('Ctrl Pts',(3.70236698911837,1.,1.97408973726149));
#56717=CARTESIAN_POINT('Ctrl Pts',(3.7055100813194,-1.,1.974177276451));
#56718=CARTESIAN_POINT('Ctrl Pts',(3.7055100813194,1.,1.974177276451));
#56719=CARTESIAN_POINT('Ctrl Pts',(3.70708211654725,-1.,1.97421938526992));
#56720=CARTESIAN_POINT('Ctrl Pts',(3.70708211654725,1.,1.97421938526992));
#56721=CARTESIAN_POINT('',(3.24413672884902,1.,1.88097764062542));
#56722=CARTESIAN_POINT('Ctrl Pts',(3.24413672884902,-1.,1.88097764062542));
#56723=CARTESIAN_POINT('Ctrl Pts',(3.24413672884902,-0.666666666666667,
1.88097764062542));
#56724=CARTESIAN_POINT('Ctrl Pts',(3.24413672884902,-0.333333333333333,
1.88097764062542));
#56725=CARTESIAN_POINT('Ctrl Pts',(3.24413672884902,0.333333333333333,1.88097764062542));
#56726=CARTESIAN_POINT('Ctrl Pts',(3.24413672884902,0.666666666666667,1.88097764062541));
#56727=CARTESIAN_POINT('Ctrl Pts',(3.24413672884902,1.,1.88097764062541));
#56728=CARTESIAN_POINT('',(3.70708211654725,1.,1.97421938526992));
#56729=CARTESIAN_POINT('',(3.70708211654725,0.,1.97421938526992));
#56730=CARTESIAN_POINT('Ctrl Pts',(3.24413672884902,1.,1.88097764062542));
#56731=CARTESIAN_POINT('Ctrl Pts',(3.24415531671311,1.,1.88102292397987));
#56732=CARTESIAN_POINT('Ctrl Pts',(3.24428080352952,1.,1.88117508446657));
#56733=CARTESIAN_POINT('Ctrl Pts',(3.24480754675942,1.,1.88156537699118));
#56734=CARTESIAN_POINT('Ctrl Pts',(3.24625654410705,1.,1.88242596600422));
#56735=CARTESIAN_POINT('Ctrl Pts',(3.24935200512055,1.,1.88407708646435));
#56736=CARTESIAN_POINT('Ctrl Pts',(3.25408686339298,1.,1.88646802523372));
#56737=CARTESIAN_POINT('Ctrl Pts',(3.2599988519361,1.,1.88934996203508));
#56738=CARTESIAN_POINT('Ctrl Pts',(3.2667765388833,1.,1.89255393500769));
#56739=CARTESIAN_POINT('Ctrl Pts',(3.27407108932908,1.,1.89589172903662));
#56740=CARTESIAN_POINT('Ctrl Pts',(3.28154737912287,1.,1.89918429230425));
#56741=CARTESIAN_POINT('Ctrl Pts',(3.28893448600364,1.,1.9022897124757));
#56742=CARTESIAN_POINT('Ctrl Pts',(3.29608978722258,1.,1.9051389186417));
#56743=CARTESIAN_POINT('Ctrl Pts',(3.30300595568341,1.,1.90773912171424));
#56744=CARTESIAN_POINT('Ctrl Pts',(3.30975721158694,1.,1.91014297830502));
#56745=CARTESIAN_POINT('Ctrl Pts',(3.31646052426395,1.,1.91242616234459));
#56746=CARTESIAN_POINT('Ctrl Pts',(3.32323403454507,1.,1.91466343916612));
#56747=CARTESIAN_POINT('Ctrl Pts',(3.33014884257812,1.,1.91690081930297));
#56748=CARTESIAN_POINT('Ctrl Pts',(3.33721230709948,1.,1.91914609610173));
#56749=CARTESIAN_POINT('Ctrl Pts',(3.34439448941915,1.,1.92138450828378));
#56750=CARTESIAN_POINT('Ctrl Pts',(3.35164424847206,1.,1.92358838440518));
#56751=CARTESIAN_POINT('Ctrl Pts',(3.35890824422976,1.,1.92572846125763));
#56752=CARTESIAN_POINT('Ctrl Pts',(3.36615168657597,1.,1.92778626543803));
#56753=CARTESIAN_POINT('Ctrl Pts',(3.37336807068078,1.,1.92975993109897));
#56754=CARTESIAN_POINT('Ctrl Pts',(3.38056768525577,1.,1.93165739093292));
#56755=CARTESIAN_POINT('Ctrl Pts',(3.38777076883267,1.,1.93349233176794));
#56756=CARTESIAN_POINT('Ctrl Pts',(3.39499923640789,1.,1.93527929945982));
#56757=CARTESIAN_POINT('Ctrl Pts',(3.40226802104093,1.,1.93702857723089));
#56758=CARTESIAN_POINT('Ctrl Pts',(3.40957978266622,1.,1.93874306008132));
#56759=CARTESIAN_POINT('Ctrl Pts',(3.41692971994082,1.,1.94042111965237));
#56760=CARTESIAN_POINT('Ctrl Pts',(3.42430850941497,1.,1.94205835913692));
#56761=CARTESIAN_POINT('Ctrl Pts',(3.43170586602436,1.,1.94364973660285));
#56762=CARTESIAN_POINT('Ctrl Pts',(3.43911410197693,1.,1.94519168842883));
#56763=CARTESIAN_POINT('Ctrl Pts',(3.44653088665685,1.,1.94668377715332));
#56764=CARTESIAN_POINT('Ctrl Pts',(3.45395731584051,1.,1.94812754766524));
#56765=CARTESIAN_POINT('Ctrl Pts',(3.46139661060959,1.,1.94952575850196));
#56766=CARTESIAN_POINT('Ctrl Pts',(3.4688525897419,1.,1.95088147859876));
#56767=CARTESIAN_POINT('Ctrl Pts',(3.47632820495926,1.,1.95219722189878));
#56768=CARTESIAN_POINT('Ctrl Pts',(3.48382414832648,1.,1.95347412486316));
#56769=CARTESIAN_POINT('Ctrl Pts',(3.49133956289154,1.,1.95471236969653));
#56770=CARTESIAN_POINT('Ctrl Pts',(3.49887263575602,1.,1.9559115382367));
#56771=CARTESIAN_POINT('Ctrl Pts',(3.50642124159913,1.,1.95707099606514));
#56772=CARTESIAN_POINT('Ctrl Pts',(3.51398354617772,1.,1.95819025316768));
#56773=CARTESIAN_POINT('Ctrl Pts',(3.52155867431438,1.,1.95926936324436));
#56774=CARTESIAN_POINT('Ctrl Pts',(3.52914648844289,1.,1.96030879411534));
#56775=CARTESIAN_POINT('Ctrl Pts',(3.53674730625759,1.,1.96130926212661));
#56776=CARTESIAN_POINT('Ctrl Pts',(3.54436163300425,1.,1.96227157573058));
#56777=CARTESIAN_POINT('Ctrl Pts',(3.55198990600929,1.,1.96319648628667));
#56778=CARTESIAN_POINT('Ctrl Pts',(3.55963218706201,1.,1.96408450906868));
#56779=CARTESIAN_POINT('Ctrl Pts',(3.56728820357933,1.,1.96493594634643));
#56780=CARTESIAN_POINT('Ctrl Pts',(3.57495748601088,1.,1.96575096652857));
#56781=CARTESIAN_POINT('Ctrl Pts',(3.58263947663884,1.,1.9665296668894));
#56782=CARTESIAN_POINT('Ctrl Pts',(3.5903336402273,1.,1.96727213799507));
#56783=CARTESIAN_POINT('Ctrl Pts',(3.59803959819725,1.,1.96797854118257));
#56784=CARTESIAN_POINT('Ctrl Pts',(3.60575714017676,1.,1.96864911885775));
#56785=CARTESIAN_POINT('Ctrl Pts',(3.61348615496393,1.,1.96928416040712));
#56786=CARTESIAN_POINT('Ctrl Pts',(3.62122658401722,1.,1.96988398129888));
#56787=CARTESIAN_POINT('Ctrl Pts',(3.62897836973397,1.,1.97044889850518));
#56788=CARTESIAN_POINT('Ctrl Pts',(3.63674139590853,1.,1.97097920454698));
#56789=CARTESIAN_POINT('Ctrl Pts',(3.64451546724221,1.,1.97147515441539));
#56790=CARTESIAN_POINT('Ctrl Pts',(3.65230034717364,1.,1.97193697240645));
#56791=CARTESIAN_POINT('Ctrl Pts',(3.66009578166865,1.,1.97236485439317));
#56792=CARTESIAN_POINT('Ctrl Pts',(3.66790152751984,1.,1.9727589719863));
#56793=CARTESIAN_POINT('Ctrl Pts',(3.67571738106175,1.,1.97311947678035));
#56794=CARTESIAN_POINT('Ctrl Pts',(3.68354319913416,1.,1.97344650303631));
#56795=CARTESIAN_POINT('Ctrl Pts',(3.69137888597855,1.,1.97374016224397));
#56796=CARTESIAN_POINT('Ctrl Pts',(3.69765528558292,1.,1.97394846382289));
#56797=CARTESIAN_POINT('Ctrl Pts',(3.70236698911837,1.,1.97408973726149));
#56798=CARTESIAN_POINT('Ctrl Pts',(3.7055100813194,1.,1.974177276451));
#56799=CARTESIAN_POINT('Ctrl Pts',(3.70708211654725,1.,1.97421938526992));
#56800=CARTESIAN_POINT('Origin',(3.70708211654725,0.,1.97421938526992));
#56801=CARTESIAN_POINT('',(3.77614523045147,1.,1.83867539237861));
#56802=CARTESIAN_POINT('Origin',(0.,0.,0.));
#56803=CARTESIAN_POINT('',(3.14877060440425,1.,2.03660101169564));
#56804=CARTESIAN_POINT('Origin',(0.,1.,0.));
#56805=CARTESIAN_POINT('Ctrl Pts',(3.14877060440425,1.,2.03660101169564));
#56806=CARTESIAN_POINT('Ctrl Pts',(3.14877060440425,0.666666666666667,2.03660101169564));
#56807=CARTESIAN_POINT('Ctrl Pts',(3.14877060440425,0.333333333333333,2.03660101169564));
#56808=CARTESIAN_POINT('Ctrl Pts',(3.14877060440425,-0.333333333333333,
2.03660101169564));
#56809=CARTESIAN_POINT('Ctrl Pts',(3.14877060440425,-0.666666666666667,
2.03660101169564));
#56810=CARTESIAN_POINT('Ctrl Pts',(3.14877060440425,-1.,2.03660101169564));
#56811=CARTESIAN_POINT('Ctrl Pts',(3.44202241512147,-1.,2.40675750623143));
#56812=CARTESIAN_POINT('Ctrl Pts',(3.44202241512147,1.,2.40675750623143));
#56813=CARTESIAN_POINT('Ctrl Pts',(3.44127120683402,-1.,2.40537592959345));
#56814=CARTESIAN_POINT('Ctrl Pts',(3.44127120683402,1.,2.40537592959345));
#56815=CARTESIAN_POINT('Ctrl Pts',(3.43976627485223,-1.,2.40261515590099));
#56816=CARTESIAN_POINT('Ctrl Pts',(3.43976627485223,1.,2.40261515590099));
#56817=CARTESIAN_POINT('Ctrl Pts',(3.43750133066036,-1.,2.39848113411429));
#56818=CARTESIAN_POINT('Ctrl Pts',(3.43750133066036,1.,2.39848113411429));
#56819=CARTESIAN_POINT('Ctrl Pts',(3.43446630680436,-1.,2.39298338805823));
#56820=CARTESIAN_POINT('Ctrl Pts',(3.43446630680436,1.,2.39298338805823));
#56821=CARTESIAN_POINT('Ctrl Pts',(3.43064732714472,-1.,2.38613505844641));
#56822=CARTESIAN_POINT('Ctrl Pts',(3.43064732714472,1.,2.38613505844641));
#56823=CARTESIAN_POINT('Ctrl Pts',(3.42680309755241,-1.,2.37931067029517));
#56824=CARTESIAN_POINT('Ctrl Pts',(3.42680309755241,1.,2.37931067029517));
#56825=CARTESIAN_POINT('Ctrl Pts',(3.42293356216595,-1.,2.37251035954351));
#56826=CARTESIAN_POINT('Ctrl Pts',(3.42293356216595,1.,2.37251035954351));
#56827=CARTESIAN_POINT('Ctrl Pts',(3.41903866635384,-1.,2.36573431470314));
#56828=CARTESIAN_POINT('Ctrl Pts',(3.41903866635384,1.,2.36573431470314));
#56829=CARTESIAN_POINT('Ctrl Pts',(3.4151183675076,-1.,2.35898278606449));
#56830=CARTESIAN_POINT('Ctrl Pts',(3.4151183675076,1.,2.35898278606449));
#56831=CARTESIAN_POINT('Ctrl Pts',(3.41117262313464,-1.,2.35225606823649));
#56832=CARTESIAN_POINT('Ctrl Pts',(3.41117262313464,1.,2.35225606823649));
#56833=CARTESIAN_POINT('Ctrl Pts',(3.40720137403888,-1.,2.34555447648901));
#56834=CARTESIAN_POINT('Ctrl Pts',(3.40720137403888,1.,2.34555447648901));
#56835=CARTESIAN_POINT('Ctrl Pts',(3.40320452776646,-1.,2.33887832342715));
#56836=CARTESIAN_POINT('Ctrl Pts',(3.40320452776646,1.,2.33887832342715));
#56837=CARTESIAN_POINT('Ctrl Pts',(3.39918194578115,-1.,2.33222789882601));
#56838=CARTESIAN_POINT('Ctrl Pts',(3.39918194578115,1.,2.33222789882601));
#56839=CARTESIAN_POINT('Ctrl Pts',(3.39513342020045,-1.,2.32560343902683));
#56840=CARTESIAN_POINT('Ctrl Pts',(3.39513342020045,1.,2.32560343902683));
#56841=CARTESIAN_POINT('Ctrl Pts',(3.39105869475112,-1.,2.31900513925627));
#56842=CARTESIAN_POINT('Ctrl Pts',(3.39105869475112,1.,2.31900513925627));
#56843=CARTESIAN_POINT('Ctrl Pts',(3.38695751492659,-1.,2.31243319489505));
#56844=CARTESIAN_POINT('Ctrl Pts',(3.38695751492659,1.,2.31243319489505));
#56845=CARTESIAN_POINT('Ctrl Pts',(3.38282967336676,-1.,2.30588783640389));
#56846=CARTESIAN_POINT('Ctrl Pts',(3.38282967336676,1.,2.30588783640389));
#56847=CARTESIAN_POINT('Ctrl Pts',(3.37867504959382,-1.,2.29936936127588));
#56848=CARTESIAN_POINT('Ctrl Pts',(3.37867504959382,1.,2.29936936127588));
#56849=CARTESIAN_POINT('Ctrl Pts',(3.37449367172707,-1.,2.2928781800731));
#56850=CARTESIAN_POINT('Ctrl Pts',(3.37449367172707,1.,2.2928781800731));
#56851=CARTESIAN_POINT('Ctrl Pts',(3.37028570206357,-1.,2.28641481081045));
#56852=CARTESIAN_POINT('Ctrl Pts',(3.37028570206357,1.,2.28641481081045));
#56853=CARTESIAN_POINT('Ctrl Pts',(3.36605130712978,-1.,2.27997979457968));
#56854=CARTESIAN_POINT('Ctrl Pts',(3.36605130712978,1.,2.27997979457968));
#56855=CARTESIAN_POINT('Ctrl Pts',(3.36179055004369,-1.,2.27357362620902));
#56856=CARTESIAN_POINT('Ctrl Pts',(3.36179055004369,1.,2.27357362620902));
#56857=CARTESIAN_POINT('Ctrl Pts',(3.35750328523077,-1.,2.26719668579921));
#56858=CARTESIAN_POINT('Ctrl Pts',(3.35750328523077,1.,2.26719668579921));
#56859=CARTESIAN_POINT('Ctrl Pts',(3.35318902552676,-1.,2.26084915222484));
#56860=CARTESIAN_POINT('Ctrl Pts',(3.35318902552676,1.,2.26084915222484));
#56861=CARTESIAN_POINT('Ctrl Pts',(3.34884690292342,-1.,2.25453097693524));
#56862=CARTESIAN_POINT('Ctrl Pts',(3.34884690292342,1.,2.25453097693524));
#56863=CARTESIAN_POINT('Ctrl Pts',(3.34447596770768,-1.,2.24824207678288));
#56864=CARTESIAN_POINT('Ctrl Pts',(3.34447596770768,1.,2.24824207678288));
#56865=CARTESIAN_POINT('Ctrl Pts',(3.34007543738044,-1.,2.24198249391437));
#56866=CARTESIAN_POINT('Ctrl Pts',(3.34007543738044,1.,2.24198249391437));
#56867=CARTESIAN_POINT('Ctrl Pts',(3.33564495756478,-1.,2.2357525632881));
#56868=CARTESIAN_POINT('Ctrl Pts',(3.33564495756478,1.,2.2357525632881));
#56869=CARTESIAN_POINT('Ctrl Pts',(3.33118487773593,-1.,2.22955308907221));
#56870=CARTESIAN_POINT('Ctrl Pts',(3.33118487773593,1.,2.22955308907221));
#56871=CARTESIAN_POINT('Ctrl Pts',(3.32669646722871,-1.,2.22338548312759));
#56872=CARTESIAN_POINT('Ctrl Pts',(3.32669646722871,1.,2.22338548312759));
#56873=CARTESIAN_POINT('Ctrl Pts',(3.32218125618955,-1.,2.21725135110889));
#56874=CARTESIAN_POINT('Ctrl Pts',(3.32218125618955,1.,2.21725135110889));
#56875=CARTESIAN_POINT('Ctrl Pts',(3.31764044024231,-1.,2.21115211847872));
#56876=CARTESIAN_POINT('Ctrl Pts',(3.31764044024231,1.,2.21115211847872));
#56877=CARTESIAN_POINT('Ctrl Pts',(3.3130742460895,-1.,2.20508863150608));
#56878=CARTESIAN_POINT('Ctrl Pts',(3.3130742460895,1.,2.20508863150608));
#56879=CARTESIAN_POINT('Ctrl Pts',(3.30848134694596,-1.,2.19906078949925));
#56880=CARTESIAN_POINT('Ctrl Pts',(3.30848134694596,1.,2.19906078949925));
#56881=CARTESIAN_POINT('Ctrl Pts',(3.30385816281831,-1.,2.19306710376112));
#56882=CARTESIAN_POINT('Ctrl Pts',(3.30385816281831,1.,2.19306710376112));
#56883=CARTESIAN_POINT('Ctrl Pts',(3.29920022557635,-1.,2.18710556500325));
#56884=CARTESIAN_POINT('Ctrl Pts',(3.29920022557635,1.,2.18710556500325));
#56885=CARTESIAN_POINT('Ctrl Pts',(3.29450361500484,-1.,2.18117455557062));
#56886=CARTESIAN_POINT('Ctrl Pts',(3.29450361500484,1.,2.18117455557062));
#56887=CARTESIAN_POINT('Ctrl Pts',(3.28976645712566,-1.,2.17527380048422));
#56888=CARTESIAN_POINT('Ctrl Pts',(3.28976645712566,1.,2.17527380048422));
#56889=CARTESIAN_POINT('Ctrl Pts',(3.2849901997973,-1.,2.16940517773459));
#56890=CARTESIAN_POINT('Ctrl Pts',(3.2849901997973,1.,2.16940517773459));
#56891=CARTESIAN_POINT('Ctrl Pts',(3.28018150841414,-1.,2.16357391934434));
#56892=CARTESIAN_POINT('Ctrl Pts',(3.28018150841414,1.,2.16357391934434));
#56893=CARTESIAN_POINT('Ctrl Pts',(3.27534954469206,-1.,2.15778690038359));
#56894=CARTESIAN_POINT('Ctrl Pts',(3.27534954469206,1.,2.15778690038359));
#56895=CARTESIAN_POINT('Ctrl Pts',(3.27050245897244,-1.,2.15205043199818));
#56896=CARTESIAN_POINT('Ctrl Pts',(3.27050245897244,1.,2.15205043199818));
#56897=CARTESIAN_POINT('Ctrl Pts',(3.26564388189764,-1.,2.14636805295663));
#56898=CARTESIAN_POINT('Ctrl Pts',(3.26564388189764,1.,2.14636805295663));
#56899=CARTESIAN_POINT('Ctrl Pts',(3.26077002641868,-1.,2.14073870754258));
#56900=CARTESIAN_POINT('Ctrl Pts',(3.26077002641868,1.,2.14073870754258));
#56901=CARTESIAN_POINT('Ctrl Pts',(3.25586495065027,-1.,2.13515375878786));
#56902=CARTESIAN_POINT('Ctrl Pts',(3.25586495065027,1.,2.13515375878786));
#56903=CARTESIAN_POINT('Ctrl Pts',(3.25090574493994,-1.,2.1296002839681));
#56904=CARTESIAN_POINT('Ctrl Pts',(3.25090574493994,1.,2.1296002839681));
#56905=CARTESIAN_POINT('Ctrl Pts',(3.24587102613347,-1.,2.12406646410943));
#56906=CARTESIAN_POINT('Ctrl Pts',(3.24587102613347,1.,2.12406646410943));
#56907=CARTESIAN_POINT('Ctrl Pts',(3.24074905517282,-1.,2.11854673326972));
#56908=CARTESIAN_POINT('Ctrl Pts',(3.24074905517282,1.,2.11854673326972));
#56909=CARTESIAN_POINT('Ctrl Pts',(3.23554444767115,-1.,2.11304604021784));
#56910=CARTESIAN_POINT('Ctrl Pts',(3.23554444767115,1.,2.11304604021784));
#56911=CARTESIAN_POINT('Ctrl Pts',(3.23028945793334,-1.,2.1075869964248));
#56912=CARTESIAN_POINT('Ctrl Pts',(3.23028945793334,1.,2.1075869964248));
#56913=CARTESIAN_POINT('Ctrl Pts',(3.22503437553496,-1.,2.10220384298534));
#56914=CARTESIAN_POINT('Ctrl Pts',(3.22503437553496,1.,2.10220384298534));
#56915=CARTESIAN_POINT('Ctrl Pts',(3.21982707347067,-1.,2.09692958434933));
#56916=CARTESIAN_POINT('Ctrl Pts',(3.21982707347067,1.,2.09692958434933));
#56917=CARTESIAN_POINT('Ctrl Pts',(3.2146942960168,-1.,2.0917841946046));
#56918=CARTESIAN_POINT('Ctrl Pts',(3.2146942960168,1.,2.0917841946046));
#56919=CARTESIAN_POINT('Ctrl Pts',(3.20962575845433,-1.,2.08676465517435));
#56920=CARTESIAN_POINT('Ctrl Pts',(3.20962575845433,1.,2.08676465517435));
#56921=CARTESIAN_POINT('Ctrl Pts',(3.20454818630635,-1.,2.08182850370816));
#56922=CARTESIAN_POINT('Ctrl Pts',(3.20454818630635,1.,2.08182850370816));
#56923=CARTESIAN_POINT('Ctrl Pts',(3.19934132835879,-1.,2.0769044187063));
#56924=CARTESIAN_POINT('Ctrl Pts',(3.19934132835879,1.,2.0769044187063));
#56925=CARTESIAN_POINT('Ctrl Pts',(3.19388465568113,-1.,2.07192253497765));
#56926=CARTESIAN_POINT('Ctrl Pts',(3.19388465568113,1.,2.07192253497765));
#56927=CARTESIAN_POINT('Ctrl Pts',(3.18809755562297,-1.,2.06684062744065));
#56928=CARTESIAN_POINT('Ctrl Pts',(3.18809755562297,1.,2.06684062744065));
#56929=CARTESIAN_POINT('Ctrl Pts',(3.18197692964677,-1.,2.06166849827143));
#56930=CARTESIAN_POINT('Ctrl Pts',(3.18197692964677,1.,2.06166849827143));
#56931=CARTESIAN_POINT('Ctrl Pts',(3.17564906975592,-1.,2.05650186773279));
#56932=CARTESIAN_POINT('Ctrl Pts',(3.17564906975592,1.,2.05650186773279));
#56933=CARTESIAN_POINT('Ctrl Pts',(3.16936341689859,-1.,2.05151770247452));
#56934=CARTESIAN_POINT('Ctrl Pts',(3.16936341689859,1.,2.05151770247452));
#56935=CARTESIAN_POINT('Ctrl Pts',(3.16343165059235,-1.,2.0469333124766));
#56936=CARTESIAN_POINT('Ctrl Pts',(3.16343165059235,1.,2.0469333124766));
#56937=CARTESIAN_POINT('Ctrl Pts',(3.15817983946525,-1.,2.04297406404132));
#56938=CARTESIAN_POINT('Ctrl Pts',(3.15817983946525,1.,2.04297406404132));
#56939=CARTESIAN_POINT('Ctrl Pts',(3.1538999167466,-1.,2.03984073791432));
#56940=CARTESIAN_POINT('Ctrl Pts',(3.1538999167466,1.,2.03984073791432));
#56941=CARTESIAN_POINT('Ctrl Pts',(3.15079010635326,-1.,2.03766932526171));
#56942=CARTESIAN_POINT('Ctrl Pts',(3.15079010635326,1.,2.03766932526171));
#56943=CARTESIAN_POINT('Ctrl Pts',(3.14931281967585,-1.,2.03675273048882));
#56944=CARTESIAN_POINT('Ctrl Pts',(3.14931281967585,1.,2.03675273048882));
#56945=CARTESIAN_POINT('Ctrl Pts',(3.14878756590499,-1.,2.03653654935384));
#56946=CARTESIAN_POINT('Ctrl Pts',(3.14878756590499,1.,2.03653654935384));
#56947=CARTESIAN_POINT('Ctrl Pts',(3.14869618937138,-1.,2.036601737578));
#56948=CARTESIAN_POINT('Ctrl Pts',(3.14869618937138,1.,2.036601737578));
#56949=CARTESIAN_POINT('Ctrl Pts',(3.1487152044751,-1.,2.03668666247593));
#56950=CARTESIAN_POINT('Ctrl Pts',(3.1487152044751,1.,2.03668666247593));
#56951=CARTESIAN_POINT('',(3.44202241512147,1.,2.40675750623143));
#56952=CARTESIAN_POINT('Ctrl Pts',(3.44202241512147,1.,2.40675750623143));
#56953=CARTESIAN_POINT('Ctrl Pts',(3.44127120683402,1.,2.40537592959345));
#56954=CARTESIAN_POINT('Ctrl Pts',(3.43976627485223,1.,2.40261515590099));
#56955=CARTESIAN_POINT('Ctrl Pts',(3.43750133066036,1.,2.39848113411429));
#56956=CARTESIAN_POINT('Ctrl Pts',(3.43446630680436,1.,2.39298338805823));
#56957=CARTESIAN_POINT('Ctrl Pts',(3.43064732714472,1.,2.38613505844641));
#56958=CARTESIAN_POINT('Ctrl Pts',(3.42680309755241,1.,2.37931067029517));
#56959=CARTESIAN_POINT('Ctrl Pts',(3.42293356216595,1.,2.37251035954351));
#56960=CARTESIAN_POINT('Ctrl Pts',(3.41903866635384,1.,2.36573431470314));
#56961=CARTESIAN_POINT('Ctrl Pts',(3.4151183675076,1.,2.35898278606449));
#56962=CARTESIAN_POINT('Ctrl Pts',(3.41117262313464,1.,2.35225606823649));
#56963=CARTESIAN_POINT('Ctrl Pts',(3.40720137403888,1.,2.34555447648901));
#56964=CARTESIAN_POINT('Ctrl Pts',(3.40320452776646,1.,2.33887832342715));
#56965=CARTESIAN_POINT('Ctrl Pts',(3.39918194578115,1.,2.33222789882601));
#56966=CARTESIAN_POINT('Ctrl Pts',(3.39513342020045,1.,2.32560343902683));
#56967=CARTESIAN_POINT('Ctrl Pts',(3.39105869475112,1.,2.31900513925627));
#56968=CARTESIAN_POINT('Ctrl Pts',(3.38695751492659,1.,2.31243319489505));
#56969=CARTESIAN_POINT('Ctrl Pts',(3.38282967336676,1.,2.30588783640389));
#56970=CARTESIAN_POINT('Ctrl Pts',(3.37867504959382,1.,2.29936936127588));
#56971=CARTESIAN_POINT('Ctrl Pts',(3.37449367172707,1.,2.2928781800731));
#56972=CARTESIAN_POINT('Ctrl Pts',(3.37028570206357,1.,2.28641481081045));
#56973=CARTESIAN_POINT('Ctrl Pts',(3.36605130712978,1.,2.27997979457968));
#56974=CARTESIAN_POINT('Ctrl Pts',(3.36179055004369,1.,2.27357362620902));
#56975=CARTESIAN_POINT('Ctrl Pts',(3.35750328523077,1.,2.26719668579921));
#56976=CARTESIAN_POINT('Ctrl Pts',(3.35318902552676,1.,2.26084915222484));
#56977=CARTESIAN_POINT('Ctrl Pts',(3.34884690292342,1.,2.25453097693524));
#56978=CARTESIAN_POINT('Ctrl Pts',(3.34447596770768,1.,2.24824207678288));
#56979=CARTESIAN_POINT('Ctrl Pts',(3.34007543738044,1.,2.24198249391437));
#56980=CARTESIAN_POINT('Ctrl Pts',(3.33564495756478,1.,2.2357525632881));
#56981=CARTESIAN_POINT('Ctrl Pts',(3.33118487773593,1.,2.22955308907221));
#56982=CARTESIAN_POINT('Ctrl Pts',(3.32669646722871,1.,2.22338548312759));
#56983=CARTESIAN_POINT('Ctrl Pts',(3.32218125618955,1.,2.21725135110889));
#56984=CARTESIAN_POINT('Ctrl Pts',(3.31764044024231,1.,2.21115211847872));
#56985=CARTESIAN_POINT('Ctrl Pts',(3.3130742460895,1.,2.20508863150608));
#56986=CARTESIAN_POINT('Ctrl Pts',(3.30848134694596,1.,2.19906078949925));
#56987=CARTESIAN_POINT('Ctrl Pts',(3.30385816281831,1.,2.19306710376112));
#56988=CARTESIAN_POINT('Ctrl Pts',(3.29920022557635,1.,2.18710556500325));
#56989=CARTESIAN_POINT('Ctrl Pts',(3.29450361500484,1.,2.18117455557062));
#56990=CARTESIAN_POINT('Ctrl Pts',(3.28976645712566,1.,2.17527380048422));
#56991=CARTESIAN_POINT('Ctrl Pts',(3.2849901997973,1.,2.16940517773459));
#56992=CARTESIAN_POINT('Ctrl Pts',(3.28018150841414,1.,2.16357391934434));
#56993=CARTESIAN_POINT('Ctrl Pts',(3.27534954469206,1.,2.15778690038359));
#56994=CARTESIAN_POINT('Ctrl Pts',(3.27050245897244,1.,2.15205043199818));
#56995=CARTESIAN_POINT('Ctrl Pts',(3.26564388189764,1.,2.14636805295663));
#56996=CARTESIAN_POINT('Ctrl Pts',(3.26077002641868,1.,2.14073870754258));
#56997=CARTESIAN_POINT('Ctrl Pts',(3.25586495065027,1.,2.13515375878786));
#56998=CARTESIAN_POINT('Ctrl Pts',(3.25090574493994,1.,2.1296002839681));
#56999=CARTESIAN_POINT('Ctrl Pts',(3.24587102613347,1.,2.12406646410943));
#57000=CARTESIAN_POINT('Ctrl Pts',(3.24074905517282,1.,2.11854673326972));
#57001=CARTESIAN_POINT('Ctrl Pts',(3.23554444767115,1.,2.11304604021784));
#57002=CARTESIAN_POINT('Ctrl Pts',(3.23028945793334,1.,2.1075869964248));
#57003=CARTESIAN_POINT('Ctrl Pts',(3.22503437553496,1.,2.10220384298534));
#57004=CARTESIAN_POINT('Ctrl Pts',(3.21982707347067,1.,2.09692958434933));
#57005=CARTESIAN_POINT('Ctrl Pts',(3.2146942960168,1.,2.0917841946046));
#57006=CARTESIAN_POINT('Ctrl Pts',(3.20962575845433,1.,2.08676465517435));
#57007=CARTESIAN_POINT('Ctrl Pts',(3.20454818630635,1.,2.08182850370816));
#57008=CARTESIAN_POINT('Ctrl Pts',(3.19934132835879,1.,2.0769044187063));
#57009=CARTESIAN_POINT('Ctrl Pts',(3.19388465568113,1.,2.07192253497765));
#57010=CARTESIAN_POINT('Ctrl Pts',(3.18809755562297,1.,2.06684062744065));
#57011=CARTESIAN_POINT('Ctrl Pts',(3.18197692964677,1.,2.06166849827143));
#57012=CARTESIAN_POINT('Ctrl Pts',(3.17564906975592,1.,2.05650186773279));
#57013=CARTESIAN_POINT('Ctrl Pts',(3.16936341689859,1.,2.05151770247452));
#57014=CARTESIAN_POINT('Ctrl Pts',(3.16343165059235,1.,2.0469333124766));
#57015=CARTESIAN_POINT('Ctrl Pts',(3.15817983946525,1.,2.04297406404132));
#57016=CARTESIAN_POINT('Ctrl Pts',(3.1538999167466,1.,2.03984073791432));
#57017=CARTESIAN_POINT('Ctrl Pts',(3.15102344775396,1.,2.03783225496023));
#57018=CARTESIAN_POINT('Ctrl Pts',(3.14959882629936,1.,2.03693188810614));
#57019=CARTESIAN_POINT('Ctrl Pts',(3.14901193669147,1.,2.03663974554941));
#57020=CARTESIAN_POINT('Ctrl Pts',(3.1488193908823,1.,2.03659701539175));
#57021=CARTESIAN_POINT('Ctrl Pts',(3.14877060440425,1.,2.03660101169564));
#57022=CARTESIAN_POINT('',(3.44202241512147,0.,2.40675750623143));
#57023=CARTESIAN_POINT('Ctrl Pts',(2.91001063062876,-1.,2.36523532225181));
#57024=CARTESIAN_POINT('Ctrl Pts',(2.91001063062876,1.,2.36523532225181));
#57025=CARTESIAN_POINT('Ctrl Pts',(2.90992398626211,-1.,2.36524348105112));
#57026=CARTESIAN_POINT('Ctrl Pts',(2.90992398626211,1.,2.36524348105112));
#57027=CARTESIAN_POINT('Ctrl Pts',(2.90989022548032,-1.,2.36535052956938));
#57028=CARTESIAN_POINT('Ctrl Pts',(2.90989022548032,1.,2.36535052956938));
#57029=CARTESIAN_POINT('Ctrl Pts',(2.91025813830041,-1.,2.36578327194741));
#57030=CARTESIAN_POINT('Ctrl Pts',(2.91025813830041,1.,2.36578327194741));
#57031=CARTESIAN_POINT('Ctrl Pts',(2.9115863784204,-1.,2.36690501170627));
#57032=CARTESIAN_POINT('Ctrl Pts',(2.9115863784204,1.,2.36690501170627));
#57033=CARTESIAN_POINT('Ctrl Pts',(2.9146124988314,-1.,2.36919161373173));
#57034=CARTESIAN_POINT('Ctrl Pts',(2.9146124988314,1.,2.36919161373173));
#57035=CARTESIAN_POINT('Ctrl Pts',(2.91891503791411,-1.,2.37229381109821));
#57036=CARTESIAN_POINT('Ctrl Pts',(2.91891503791411,1.,2.37229381109821));
#57037=CARTESIAN_POINT('Ctrl Pts',(2.92430340582608,-1.,2.3760651052403));
#57038=CARTESIAN_POINT('Ctrl Pts',(2.92430340582608,1.,2.3760651052403));
#57039=CARTESIAN_POINT('Ctrl Pts',(2.93049643640206,-1.,2.38028989582073));
#57040=CARTESIAN_POINT('Ctrl Pts',(2.93049643640206,1.,2.38028989582073));
#57041=CARTESIAN_POINT('Ctrl Pts',(2.93717903280391,-1.,2.38472771516311));
#57042=CARTESIAN_POINT('Ctrl Pts',(2.93717903280391,1.,2.38472771516311));
#57043=CARTESIAN_POINT('Ctrl Pts',(2.94404820669076,-1.,2.38914929090759));
#57044=CARTESIAN_POINT('Ctrl Pts',(2.94404820669076,1.,2.38914929090759));
#57045=CARTESIAN_POINT('Ctrl Pts',(2.95085857128439,-1.,2.39337207631667));
#57046=CARTESIAN_POINT('Ctrl Pts',(2.95085857128439,1.,2.39337207631667));
#57047=CARTESIAN_POINT('Ctrl Pts',(2.95748006482942,-1.,2.39730553974517));
#57048=CARTESIAN_POINT('Ctrl Pts',(2.95748006482942,1.,2.39730553974517));
#57049=CARTESIAN_POINT('Ctrl Pts',(2.96390432240312,-1.,2.4009556571164));
#57050=CARTESIAN_POINT('Ctrl Pts',(2.96390432240312,1.,2.4009556571164));
#57051=CARTESIAN_POINT('Ctrl Pts',(2.9701964131236,-1.,2.40438604734919));
#57052=CARTESIAN_POINT('Ctrl Pts',(2.9701964131236,1.,2.40438604734919));
#57053=CARTESIAN_POINT('Ctrl Pts',(2.97646002822422,-1.,2.40768975073713));
#57054=CARTESIAN_POINT('Ctrl Pts',(2.97646002822422,1.,2.40768975073713));
#57055=CARTESIAN_POINT('Ctrl Pts',(2.98280015815107,-1.,2.41095909342571));
#57056=CARTESIAN_POINT('Ctrl Pts',(2.98280015815107,1.,2.41095909342571));
#57057=CARTESIAN_POINT('Ctrl Pts',(2.98927983005796,-1.,2.41425064199586));
#57058=CARTESIAN_POINT('Ctrl Pts',(2.98927983005796,1.,2.41425064199586));
#57059=CARTESIAN_POINT('Ctrl Pts',(2.99590509293503,-1.,2.41757324500514));
#57060=CARTESIAN_POINT('Ctrl Pts',(2.99590509293503,1.,2.41757324500514));
#57061=CARTESIAN_POINT('Ctrl Pts',(3.00264868585996,-1.,2.42090763946779));
#57062=CARTESIAN_POINT('Ctrl Pts',(3.00264868585996,1.,2.42090763946779));
#57063=CARTESIAN_POINT('Ctrl Pts',(3.00946442616658,-1.,2.42421849439613));
#57064=CARTESIAN_POINT('Ctrl Pts',(3.00946442616658,1.,2.42421849439613));
#57065=CARTESIAN_POINT('Ctrl Pts',(3.01630420830504,-1.,2.42746856264168));
#57066=CARTESIAN_POINT('Ctrl Pts',(3.01630420830504,1.,2.42746856264168));
#57067=CARTESIAN_POINT('Ctrl Pts',(3.02313656036004,-1.,2.43063415586637));
#57068=CARTESIAN_POINT('Ctrl Pts',(3.02313656036004,1.,2.43063415586637));
#57069=CARTESIAN_POINT('Ctrl Pts',(3.02995534946978,-1.,2.43371241361488));
#57070=CARTESIAN_POINT('Ctrl Pts',(3.02995534946978,1.,2.43371241361488));
#57071=CARTESIAN_POINT('Ctrl Pts',(3.03676949672821,-1.,2.43671278042414));
#57072=CARTESIAN_POINT('Ctrl Pts',(3.03676949672821,1.,2.43671278042414));
#57073=CARTESIAN_POINT('Ctrl Pts',(3.04359685040555,-1.,2.43965194061857));
#57074=CARTESIAN_POINT('Ctrl Pts',(3.04359685040555,1.,2.43965194061857));
#57075=CARTESIAN_POINT('Ctrl Pts',(3.05045678021504,-1.,2.44254768923105));
#57076=CARTESIAN_POINT('Ctrl Pts',(3.05045678021504,1.,2.44254768923105));
#57077=CARTESIAN_POINT('Ctrl Pts',(3.05736242671506,-1.,2.44541251892556));
#57078=CARTESIAN_POINT('Ctrl Pts',(3.05736242671506,1.,2.44541251892556));
#57079=CARTESIAN_POINT('Ctrl Pts',(3.06431596421405,-1.,2.44824970516544));
#57080=CARTESIAN_POINT('Ctrl Pts',(3.06431596421405,1.,2.44824970516544));
#57081=CARTESIAN_POINT('Ctrl Pts',(3.07131290521297,-1.,2.45105688854422));
#57082=CARTESIAN_POINT('Ctrl Pts',(3.07131290521297,1.,2.45105688854422));
#57083=CARTESIAN_POINT('Ctrl Pts',(3.07834472886139,-1.,2.4538282678779));
#57084=CARTESIAN_POINT('Ctrl Pts',(3.07834472886139,1.,2.4538282678779));
#57085=CARTESIAN_POINT('Ctrl Pts',(3.08540206545315,-1.,2.45655725437039));
#57086=CARTESIAN_POINT('Ctrl Pts',(3.08540206545315,1.,2.45655725437039));
#57087=CARTESIAN_POINT('Ctrl Pts',(3.09247787931887,-1.,2.4592391256388));
#57088=CARTESIAN_POINT('Ctrl Pts',(3.09247787931887,1.,2.4592391256388));
#57089=CARTESIAN_POINT('Ctrl Pts',(3.09956993697052,-1.,2.46187308501884));
#57090=CARTESIAN_POINT('Ctrl Pts',(3.09956993697052,1.,2.46187308501884));
#57091=CARTESIAN_POINT('Ctrl Pts',(3.1066790790198,-1.,2.46446082979646));
#57092=CARTESIAN_POINT('Ctrl Pts',(3.1066790790198,1.,2.46446082979646));
#57093=CARTESIAN_POINT('Ctrl Pts',(3.11380805536122,-1.,2.46700558843506));
#57094=CARTESIAN_POINT('Ctrl Pts',(3.11380805536122,1.,2.46700558843506));
#57095=CARTESIAN_POINT('Ctrl Pts',(3.12096015766983,-1.,2.46951098947469));
#57096=CARTESIAN_POINT('Ctrl Pts',(3.12096015766983,1.,2.46951098947469));
#57097=CARTESIAN_POINT('Ctrl Pts',(3.12813790805952,-1.,2.47197997765871));
#57098=CARTESIAN_POINT('Ctrl Pts',(3.12813790805952,1.,2.47197997765871));
#57099=CARTESIAN_POINT('Ctrl Pts',(3.13534181229295,-1.,2.47441378371932));
#57100=CARTESIAN_POINT('Ctrl Pts',(3.13534181229295,1.,2.47441378371932));
#57101=CARTESIAN_POINT('Ctrl Pts',(3.1425709954655,-1.,2.47681245356109));
#57102=CARTESIAN_POINT('Ctrl Pts',(3.1425709954655,1.,2.47681245356109));
#57103=CARTESIAN_POINT('Ctrl Pts',(3.14982373241352,-1.,2.47917529057029));
#57104=CARTESIAN_POINT('Ctrl Pts',(3.14982373241352,1.,2.47917529057029));
#57105=CARTESIAN_POINT('Ctrl Pts',(3.15709802322739,-1.,2.48150133566571));
#57106=CARTESIAN_POINT('Ctrl Pts',(3.15709802322739,1.,2.48150133566571));
#57107=CARTESIAN_POINT('Ctrl Pts',(3.16439213290161,-1.,2.48378981792725));
#57108=CARTESIAN_POINT('Ctrl Pts',(3.16439213290161,1.,2.48378981792725));
#57109=CARTESIAN_POINT('Ctrl Pts',(3.17170518863313,-1.,2.48604065348587));
#57110=CARTESIAN_POINT('Ctrl Pts',(3.17170518863313,1.,2.48604065348587));
#57111=CARTESIAN_POINT('Ctrl Pts',(3.17903698136622,-1.,2.48825428288201));
#57112=CARTESIAN_POINT('Ctrl Pts',(3.17903698136622,1.,2.48825428288201));
#57113=CARTESIAN_POINT('Ctrl Pts',(3.18638771282266,-1.,2.49043146334059));
#57114=CARTESIAN_POINT('Ctrl Pts',(3.18638771282266,1.,2.49043146334059));
#57115=CARTESIAN_POINT('Ctrl Pts',(3.19375775555798,-1.,2.49257307239848));
#57116=CARTESIAN_POINT('Ctrl Pts',(3.19375775555798,1.,2.49257307239848));
#57117=CARTESIAN_POINT('Ctrl Pts',(3.20114742397588,-1.,2.49467992057755));
#57118=CARTESIAN_POINT('Ctrl Pts',(3.20114742397588,1.,2.49467992057755));
#57119=CARTESIAN_POINT('Ctrl Pts',(3.20855669849836,-1.,2.4967525264737));
#57120=CARTESIAN_POINT('Ctrl Pts',(3.20855669849836,1.,2.4967525264737));
#57121=CARTESIAN_POINT('Ctrl Pts',(3.21598526261286,-1.,2.4987911459939));
#57122=CARTESIAN_POINT('Ctrl Pts',(3.21598526261286,1.,2.4987911459939));
#57123=CARTESIAN_POINT('Ctrl Pts',(3.22343262620503,-1.,2.50079587201958));
#57124=CARTESIAN_POINT('Ctrl Pts',(3.22343262620503,1.,2.50079587201958));
#57125=CARTESIAN_POINT('Ctrl Pts',(3.23089822320646,-1.,2.50276671338111));
#57126=CARTESIAN_POINT('Ctrl Pts',(3.23089822320646,1.,2.50276671338111));
#57127=CARTESIAN_POINT('Ctrl Pts',(3.23838151080319,-1.,2.5047036758003));
#57128=CARTESIAN_POINT('Ctrl Pts',(3.23838151080319,1.,2.5047036758003));
#57129=CARTESIAN_POINT('Ctrl Pts',(3.24588208983849,-1.,2.506606859405));
#57130=CARTESIAN_POINT('Ctrl Pts',(3.24588208983849,1.,2.506606859405));
#57131=CARTESIAN_POINT('Ctrl Pts',(3.25339971460982,-1.,2.50847647070723));
#57132=CARTESIAN_POINT('Ctrl Pts',(3.25339971460982,1.,2.50847647070723));
#57133=CARTESIAN_POINT('Ctrl Pts',(3.26093423001434,-1.,2.51031277813486));
#57134=CARTESIAN_POINT('Ctrl Pts',(3.26093423001434,1.,2.51031277813486));
#57135=CARTESIAN_POINT('Ctrl Pts',(3.26848552888115,-1.,2.51211608411423));
#57136=CARTESIAN_POINT('Ctrl Pts',(3.26848552888115,1.,2.51211608411423));
#57137=CARTESIAN_POINT('Ctrl Pts',(3.27605350473142,-1.,2.513886692704));
#57138=CARTESIAN_POINT('Ctrl Pts',(3.27605350473142,1.,2.513886692704));
#57139=CARTESIAN_POINT('Ctrl Pts',(3.28363799702982,-1.,2.51562487464514));
#57140=CARTESIAN_POINT('Ctrl Pts',(3.28363799702982,1.,2.51562487464514));
#57141=CARTESIAN_POINT('Ctrl Pts',(3.2912387729927,-1.,2.51733085123797));
#57142=CARTESIAN_POINT('Ctrl Pts',(3.2912387729927,1.,2.51733085123797));
#57143=CARTESIAN_POINT('Ctrl Pts',(3.29885556388352,-1.,2.51900480701069));
#57144=CARTESIAN_POINT('Ctrl Pts',(3.29885556388352,1.,2.51900480701069));
#57145=CARTESIAN_POINT('Ctrl Pts',(3.30648808815442,-1.,2.52064689568511));
#57146=CARTESIAN_POINT('Ctrl Pts',(3.30648808815442,1.,2.52064689568511));
#57147=CARTESIAN_POINT('Ctrl Pts',(3.31413607874645,-1.,2.52225724871313));
#57148=CARTESIAN_POINT('Ctrl Pts',(3.31413607874645,1.,2.52225724871313));
#57149=CARTESIAN_POINT('Ctrl Pts',(3.32179931078699,-1.,2.5238359839626));
#57150=CARTESIAN_POINT('Ctrl Pts',(3.32179931078699,1.,2.5238359839626));
#57151=CARTESIAN_POINT('Ctrl Pts',(3.32947762187533,-1.,2.52538321164634));
#57152=CARTESIAN_POINT('Ctrl Pts',(3.32947762187533,1.,2.52538321164634));
#57153=CARTESIAN_POINT('Ctrl Pts',(3.33717089999103,-1.,2.52689902690158));
#57154=CARTESIAN_POINT('Ctrl Pts',(3.33717089999103,1.,2.52689902690158));
#57155=CARTESIAN_POINT('Ctrl Pts',(3.34333744115511,-1.,2.52808660915689));
#57156=CARTESIAN_POINT('Ctrl Pts',(3.34333744115511,1.,2.52808660915689));
#57157=CARTESIAN_POINT('Ctrl Pts',(3.34796903576663,-1.,2.52896321610703));
#57158=CARTESIAN_POINT('Ctrl Pts',(3.34796903576663,1.,2.52896321610703));
#57159=CARTESIAN_POINT('Ctrl Pts',(3.35105973714071,-1.,2.5295413654909));
#57160=CARTESIAN_POINT('Ctrl Pts',(3.35105973714071,1.,2.5295413654909));
#57161=CARTESIAN_POINT('Ctrl Pts',(3.35260583073571,-1.,2.52982887637028));
#57162=CARTESIAN_POINT('Ctrl Pts',(3.35260583073571,1.,2.52982887637028));
#57163=CARTESIAN_POINT('',(2.90994629141676,1.,2.36531447826073));
#57164=CARTESIAN_POINT('Ctrl Pts',(2.90994629141676,-1.,2.36531447826073));
#57165=CARTESIAN_POINT('Ctrl Pts',(2.90994629141676,-0.666666666666667,
2.36531447826073));
#57166=CARTESIAN_POINT('Ctrl Pts',(2.90994629141676,-0.333333333333333,
2.36531447826073));
#57167=CARTESIAN_POINT('Ctrl Pts',(2.90994629141676,0.333333333333333,2.36531447826073));
#57168=CARTESIAN_POINT('Ctrl Pts',(2.90994629141676,0.666666666666667,2.36531447826073));
#57169=CARTESIAN_POINT('Ctrl Pts',(2.90994629141676,1.,2.36531447826073));
#57170=CARTESIAN_POINT('',(3.35260583073571,1.,2.52982887637028));
#57171=CARTESIAN_POINT('',(3.35260583073571,0.,2.52982887637028));
#57172=CARTESIAN_POINT('Ctrl Pts',(2.90994629141676,1.,2.36531447826073));
#57173=CARTESIAN_POINT('Ctrl Pts',(2.90995756655606,1.,2.36536211188453));
#57174=CARTESIAN_POINT('Ctrl Pts',(2.91005770527719,1.,2.36553202948613));
#57175=CARTESIAN_POINT('Ctrl Pts',(2.91051690822156,1.,2.36599991765749));
#57176=CARTESIAN_POINT('Ctrl Pts',(2.91181344022548,1.,2.36707658451664));
#57177=CARTESIAN_POINT('Ctrl Pts',(2.9146124988314,1.,2.36919161373173));
#57178=CARTESIAN_POINT('Ctrl Pts',(2.91891503791411,1.,2.37229381109821));
#57179=CARTESIAN_POINT('Ctrl Pts',(2.92430340582608,1.,2.3760651052403));
#57180=CARTESIAN_POINT('Ctrl Pts',(2.93049643640206,1.,2.38028989582073));
#57181=CARTESIAN_POINT('Ctrl Pts',(2.93717903280391,1.,2.38472771516311));
#57182=CARTESIAN_POINT('Ctrl Pts',(2.94404820669076,1.,2.38914929090759));
#57183=CARTESIAN_POINT('Ctrl Pts',(2.95085857128439,1.,2.39337207631667));
#57184=CARTESIAN_POINT('Ctrl Pts',(2.95748006482942,1.,2.39730553974517));
#57185=CARTESIAN_POINT('Ctrl Pts',(2.96390432240312,1.,2.4009556571164));
#57186=CARTESIAN_POINT('Ctrl Pts',(2.9701964131236,1.,2.40438604734919));
#57187=CARTESIAN_POINT('Ctrl Pts',(2.97646002822422,1.,2.40768975073713));
#57188=CARTESIAN_POINT('Ctrl Pts',(2.98280015815107,1.,2.41095909342571));
#57189=CARTESIAN_POINT('Ctrl Pts',(2.98927983005796,1.,2.41425064199586));
#57190=CARTESIAN_POINT('Ctrl Pts',(2.99590509293503,1.,2.41757324500514));
#57191=CARTESIAN_POINT('Ctrl Pts',(3.00264868585996,1.,2.42090763946779));
#57192=CARTESIAN_POINT('Ctrl Pts',(3.00946442616658,1.,2.42421849439613));
#57193=CARTESIAN_POINT('Ctrl Pts',(3.01630420830504,1.,2.42746856264168));
#57194=CARTESIAN_POINT('Ctrl Pts',(3.02313656036004,1.,2.43063415586637));
#57195=CARTESIAN_POINT('Ctrl Pts',(3.02995534946978,1.,2.43371241361488));
#57196=CARTESIAN_POINT('Ctrl Pts',(3.03676949672821,1.,2.43671278042414));
#57197=CARTESIAN_POINT('Ctrl Pts',(3.04359685040555,1.,2.43965194061857));
#57198=CARTESIAN_POINT('Ctrl Pts',(3.05045678021504,1.,2.44254768923105));
#57199=CARTESIAN_POINT('Ctrl Pts',(3.05736242671506,1.,2.44541251892556));
#57200=CARTESIAN_POINT('Ctrl Pts',(3.06431596421405,1.,2.44824970516544));
#57201=CARTESIAN_POINT('Ctrl Pts',(3.07131290521297,1.,2.45105688854422));
#57202=CARTESIAN_POINT('Ctrl Pts',(3.07834472886139,1.,2.4538282678779));
#57203=CARTESIAN_POINT('Ctrl Pts',(3.08540206545315,1.,2.45655725437039));
#57204=CARTESIAN_POINT('Ctrl Pts',(3.09247787931887,1.,2.4592391256388));
#57205=CARTESIAN_POINT('Ctrl Pts',(3.09956993697052,1.,2.46187308501884));
#57206=CARTESIAN_POINT('Ctrl Pts',(3.1066790790198,1.,2.46446082979646));
#57207=CARTESIAN_POINT('Ctrl Pts',(3.11380805536122,1.,2.46700558843506));
#57208=CARTESIAN_POINT('Ctrl Pts',(3.12096015766983,1.,2.46951098947469));
#57209=CARTESIAN_POINT('Ctrl Pts',(3.12813790805952,1.,2.47197997765871));
#57210=CARTESIAN_POINT('Ctrl Pts',(3.13534181229295,1.,2.47441378371932));
#57211=CARTESIAN_POINT('Ctrl Pts',(3.1425709954655,1.,2.47681245356109));
#57212=CARTESIAN_POINT('Ctrl Pts',(3.14982373241352,1.,2.47917529057029));
#57213=CARTESIAN_POINT('Ctrl Pts',(3.15709802322739,1.,2.48150133566571));
#57214=CARTESIAN_POINT('Ctrl Pts',(3.16439213290161,1.,2.48378981792725));
#57215=CARTESIAN_POINT('Ctrl Pts',(3.17170518863313,1.,2.48604065348587));
#57216=CARTESIAN_POINT('Ctrl Pts',(3.17903698136622,1.,2.48825428288201));
#57217=CARTESIAN_POINT('Ctrl Pts',(3.18638771282266,1.,2.49043146334059));
#57218=CARTESIAN_POINT('Ctrl Pts',(3.19375775555798,1.,2.49257307239848));
#57219=CARTESIAN_POINT('Ctrl Pts',(3.20114742397588,1.,2.49467992057755));
#57220=CARTESIAN_POINT('Ctrl Pts',(3.20855669849836,1.,2.4967525264737));
#57221=CARTESIAN_POINT('Ctrl Pts',(3.21598526261286,1.,2.4987911459939));
#57222=CARTESIAN_POINT('Ctrl Pts',(3.22343262620503,1.,2.50079587201958));
#57223=CARTESIAN_POINT('Ctrl Pts',(3.23089822320646,1.,2.50276671338111));
#57224=CARTESIAN_POINT('Ctrl Pts',(3.23838151080319,1.,2.5047036758003));
#57225=CARTESIAN_POINT('Ctrl Pts',(3.24588208983849,1.,2.506606859405));
#57226=CARTESIAN_POINT('Ctrl Pts',(3.25339971460982,1.,2.50847647070723));
#57227=CARTESIAN_POINT('Ctrl Pts',(3.26093423001434,1.,2.51031277813486));
#57228=CARTESIAN_POINT('Ctrl Pts',(3.26848552888115,1.,2.51211608411423));
#57229=CARTESIAN_POINT('Ctrl Pts',(3.27605350473142,1.,2.513886692704));
#57230=CARTESIAN_POINT('Ctrl Pts',(3.28363799702982,1.,2.51562487464514));
#57231=CARTESIAN_POINT('Ctrl Pts',(3.2912387729927,1.,2.51733085123797));
#57232=CARTESIAN_POINT('Ctrl Pts',(3.29885556388352,1.,2.51900480701069));
#57233=CARTESIAN_POINT('Ctrl Pts',(3.30648808815442,1.,2.52064689568511));
#57234=CARTESIAN_POINT('Ctrl Pts',(3.31413607874645,1.,2.52225724871313));
#57235=CARTESIAN_POINT('Ctrl Pts',(3.32179931078699,1.,2.5238359839626));
#57236=CARTESIAN_POINT('Ctrl Pts',(3.32947762187533,1.,2.52538321164634));
#57237=CARTESIAN_POINT('Ctrl Pts',(3.33717089999103,1.,2.52689902690158));
#57238=CARTESIAN_POINT('Ctrl Pts',(3.34333744115511,1.,2.52808660915689));
#57239=CARTESIAN_POINT('Ctrl Pts',(3.34796903576663,1.,2.52896321610703));
#57240=CARTESIAN_POINT('Ctrl Pts',(3.35105973714071,1.,2.5295413654909));
#57241=CARTESIAN_POINT('Ctrl Pts',(3.35260583073571,1.,2.52982887637028));
#57242=CARTESIAN_POINT('Origin',(3.35260583073571,0.,2.52982887637028));
#57243=CARTESIAN_POINT('',(3.44202241512147,1.,2.40675750623143));
#57244=CARTESIAN_POINT('Origin',(0.,0.,0.));
#57245=CARTESIAN_POINT('',(2.79140942341378,1.,2.50410331873042));
#57246=CARTESIAN_POINT('Origin',(0.,1.,0.));
#57247=CARTESIAN_POINT('Ctrl Pts',(2.79140942341378,1.,2.50410331873043));
#57248=CARTESIAN_POINT('Ctrl Pts',(2.79140942341378,0.666666666666667,2.50410331873043));
#57249=CARTESIAN_POINT('Ctrl Pts',(2.79140942341378,0.333333333333333,2.50410331873042));
#57250=CARTESIAN_POINT('Ctrl Pts',(2.79140942341378,-0.333333333333333,
2.50410331873042));
#57251=CARTESIAN_POINT('Ctrl Pts',(2.79140942341378,-0.666666666666667,
2.50410331873042));
#57252=CARTESIAN_POINT('Ctrl Pts',(2.79140942341378,-1.,2.50410331873042));
#57253=CARTESIAN_POINT('Ctrl Pts',(3.02314558451372,-1.,2.91557726271063));
#57254=CARTESIAN_POINT('Ctrl Pts',(3.02314558451372,1.,2.91557726271063));
#57255=CARTESIAN_POINT('Ctrl Pts',(3.02261975104912,-1.,2.91409518070707));
#57256=CARTESIAN_POINT('Ctrl Pts',(3.02261975104912,1.,2.91409518070707));
#57257=CARTESIAN_POINT('Ctrl Pts',(3.02156522743299,-1.,2.91113297349052));
#57258=CARTESIAN_POINT('Ctrl Pts',(3.02156522743299,1.,2.91113297349052));
#57259=CARTESIAN_POINT('Ctrl Pts',(3.01997487194926,-1.,2.90669553303902));
#57260=CARTESIAN_POINT('Ctrl Pts',(3.01997487194926,1.,2.90669553303902));
#57261=CARTESIAN_POINT('Ctrl Pts',(3.01783725123646,-1.,2.90079069102661));
#57262=CARTESIAN_POINT('Ctrl Pts',(3.01783725123646,1.,2.90079069102661));
#57263=CARTESIAN_POINT('Ctrl Pts',(3.01513660433291,-1.,2.8934292556764));
#57264=CARTESIAN_POINT('Ctrl Pts',(3.01513660433291,1.,2.8934292556764));
#57265=CARTESIAN_POINT('Ctrl Pts',(3.01240727309568,-1.,2.88608751706796));
#57266=CARTESIAN_POINT('Ctrl Pts',(3.01240727309568,1.,2.88608751706796));
#57267=CARTESIAN_POINT('Ctrl Pts',(3.0096491810855,-1.,2.87876560072799));
#57268=CARTESIAN_POINT('Ctrl Pts',(3.0096491810855,1.,2.87876560072799));
#57269=CARTESIAN_POINT('Ctrl Pts',(3.00686224485374,-1.,2.87146368430104));
#57270=CARTESIAN_POINT('Ctrl Pts',(3.00686224485374,1.,2.87146368430104));
#57271=CARTESIAN_POINT('Ctrl Pts',(3.00404638316245,-1.,2.86418200833065));
#57272=CARTESIAN_POINT('Ctrl Pts',(3.00404638316245,1.,2.86418200833065));
#57273=CARTESIAN_POINT('Ctrl Pts',(3.0012015079552,-1.,2.85692085715129));
#57274=CARTESIAN_POINT('Ctrl Pts',(3.0012015079552,1.,2.85692085715129));
#57275=CARTESIAN_POINT('Ctrl Pts',(2.99832751144566,-1.,2.84968053289104));
#57276=CARTESIAN_POINT('Ctrl Pts',(2.99832751144566,1.,2.84968053289104));
#57277=CARTESIAN_POINT('Ctrl Pts',(2.995424253416,-1.,2.84246132984334));
#57278=CARTESIAN_POINT('Ctrl Pts',(2.995424253416,1.,2.84246132984334));
#57279=CARTESIAN_POINT('Ctrl Pts',(2.99249155170479,-1.,2.83526351254383));
#57280=CARTESIAN_POINT('Ctrl Pts',(2.99249155170479,1.,2.83526351254383));
#57281=CARTESIAN_POINT('Ctrl Pts',(2.98952916401699,-1.,2.82808728190402));
#57282=CARTESIAN_POINT('Ctrl Pts',(2.98952916401699,1.,2.82808728190402));
#57283=CARTESIAN_POINT('Ctrl Pts',(2.98653680669434,-1.,2.82093279065704));
#57284=CARTESIAN_POINT('Ctrl Pts',(2.98653680669434,1.,2.82093279065704));
#57285=CARTESIAN_POINT('Ctrl Pts',(2.9835141977994,-1.,2.81380019196454));
#57286=CARTESIAN_POINT('Ctrl Pts',(2.9835141977994,1.,2.81380019196454));
#57287=CARTESIAN_POINT('Ctrl Pts',(2.98046109647299,-1.,2.80668968101162));
#57288=CARTESIAN_POINT('Ctrl Pts',(2.98046109647299,1.,2.80668968101162));
#57289=CARTESIAN_POINT('Ctrl Pts',(2.97737733718242,-1.,2.79960153278186));
#57290=CARTESIAN_POINT('Ctrl Pts',(2.97737733718242,1.,2.79960153278186));
#57291=CARTESIAN_POINT('Ctrl Pts',(2.97426288347475,-1.,2.79253615718147));
#57292=CARTESIAN_POINT('Ctrl Pts',(2.97426288347475,1.,2.79253615718147));
#57293=CARTESIAN_POINT('Ctrl Pts',(2.97111781461349,-1.,2.78549409123657));
#57294=CARTESIAN_POINT('Ctrl Pts',(2.97111781461349,1.,2.78549409123657));
#57295=CARTESIAN_POINT('Ctrl Pts',(2.9679422104295,-1.,2.77847589542767));
#57296=CARTESIAN_POINT('Ctrl Pts',(2.9679422104295,1.,2.77847589542767));
#57297=CARTESIAN_POINT('Ctrl Pts',(2.96473605585548,-1.,2.77148206836464));
#57298=CARTESIAN_POINT('Ctrl Pts',(2.96473605585548,1.,2.77148206836464));
#57299=CARTESIAN_POINT('Ctrl Pts',(2.96149914764832,-1.,2.76451296269571));
#57300=CARTESIAN_POINT('Ctrl Pts',(2.96149914764832,1.,2.76451296269571));
#57301=CARTESIAN_POINT('Ctrl Pts',(2.9582309766594,-1.,2.75756867888393));
#57302=CARTESIAN_POINT('Ctrl Pts',(2.9582309766594,1.,2.75756867888393));
#57303=CARTESIAN_POINT('Ctrl Pts',(2.95493069316211,-1.,2.75064903318996));
#57304=CARTESIAN_POINT('Ctrl Pts',(2.95493069316211,1.,2.75064903318996));
#57305=CARTESIAN_POINT('Ctrl Pts',(2.95159737214304,-1.,2.7437537949221));
#57306=CARTESIAN_POINT('Ctrl Pts',(2.95159737214304,1.,2.7437537949221));
#57307=CARTESIAN_POINT('Ctrl Pts',(2.94823023414381,-1.,2.73688288329825));
#57308=CARTESIAN_POINT('Ctrl Pts',(2.94823023414381,1.,2.73688288329825));
#57309=CARTESIAN_POINT('Ctrl Pts',(2.94482887675139,-1.,2.73003657371613));
#57310=CARTESIAN_POINT('Ctrl Pts',(2.94482887675139,1.,2.73003657371613));
#57311=CARTESIAN_POINT('Ctrl Pts',(2.94139351933882,-1.,2.72321571511322));
#57312=CARTESIAN_POINT('Ctrl Pts',(2.94139351933882,1.,2.72321571511322));
#57313=CARTESIAN_POINT('Ctrl Pts',(2.93792519474955,-1.,2.71642190053575));
#57314=CARTESIAN_POINT('Ctrl Pts',(2.93792519474955,1.,2.71642190053575));
#57315=CARTESIAN_POINT('Ctrl Pts',(2.93442516311167,-1.,2.70965695523776));
#57316=CARTESIAN_POINT('Ctrl Pts',(2.93442516311167,1.,2.70965695523776));
#57317=CARTESIAN_POINT('Ctrl Pts',(2.93089438233746,-1.,2.70292247416881));
#57318=CARTESIAN_POINT('Ctrl Pts',(2.93089438233746,1.,2.70292247416881));
#57319=CARTESIAN_POINT('Ctrl Pts',(2.92733294395268,-1.,2.69621932864302));
#57320=CARTESIAN_POINT('Ctrl Pts',(2.92733294395268,1.,2.69621932864302));
#57321=CARTESIAN_POINT('Ctrl Pts',(2.92373955325876,-1.,2.68954721165342));
#57322=CARTESIAN_POINT('Ctrl Pts',(2.92373955325876,1.,2.68954721165342));
#57323=CARTESIAN_POINT('Ctrl Pts',(2.92011090722152,-1.,2.68290409279689));
#57324=CARTESIAN_POINT('Ctrl Pts',(2.92011090722152,1.,2.68290409279689));
#57325=CARTESIAN_POINT('Ctrl Pts',(2.91644290704281,-1.,2.67628728855309));
#57326=CARTESIAN_POINT('Ctrl Pts',(2.91644290704281,1.,2.67628728855309));
#57327=CARTESIAN_POINT('Ctrl Pts',(2.91273193382876,-1.,2.66969458792627));
#57328=CARTESIAN_POINT('Ctrl Pts',(2.91273193382876,1.,2.66969458792627));
#57329=CARTESIAN_POINT('Ctrl Pts',(2.90897617968921,-1.,2.66312542616809));
#57330=CARTESIAN_POINT('Ctrl Pts',(2.90897617968921,1.,2.66312542616809));
#57331=CARTESIAN_POINT('Ctrl Pts',(2.90517678087467,-1.,2.65658188464287));
#57332=CARTESIAN_POINT('Ctrl Pts',(2.90517678087467,1.,2.65658188464287));
#57333=CARTESIAN_POINT('Ctrl Pts',(2.90133950224879,-1.,2.65007017365576));
#57334=CARTESIAN_POINT('Ctrl Pts',(2.90133950224879,1.,2.65007017365576));
#57335=CARTESIAN_POINT('Ctrl Pts',(2.89747231723361,-1.,2.64359851684146));
#57336=CARTESIAN_POINT('Ctrl Pts',(2.89747231723361,1.,2.64359851684146));
#57337=CARTESIAN_POINT('Ctrl Pts',(2.89358228854557,-1.,2.63717442263944));
#57338=CARTESIAN_POINT('Ctrl Pts',(2.89358228854557,1.,2.63717442263944));
#57339=CARTESIAN_POINT('Ctrl Pts',(2.88967244854243,-1.,2.63080195420771));
#57340=CARTESIAN_POINT('Ctrl Pts',(2.88967244854243,1.,2.63080195420771));
#57341=CARTESIAN_POINT('Ctrl Pts',(2.88573922195049,-1.,2.62447947640253));
#57342=CARTESIAN_POINT('Ctrl Pts',(2.88573922195049,1.,2.62447947640253));
#57343=CARTESIAN_POINT('Ctrl Pts',(2.88176821427502,-1.,2.61819596473087));
#57344=CARTESIAN_POINT('Ctrl Pts',(2.88176821427502,1.,2.61819596473087));
#57345=CARTESIAN_POINT('Ctrl Pts',(2.87773881947885,-1.,2.61193507170928));
#57346=CARTESIAN_POINT('Ctrl Pts',(2.87773881947885,1.,2.61193507170928));
#57347=CARTESIAN_POINT('Ctrl Pts',(2.87363176656475,-1.,2.6056817788128));
#57348=CARTESIAN_POINT('Ctrl Pts',(2.87363176656475,1.,2.6056817788128));
#57349=CARTESIAN_POINT('Ctrl Pts',(2.86943633170712,-1.,2.59942875223202));
#57350=CARTESIAN_POINT('Ctrl Pts',(2.86943633170712,1.,2.59942875223202));
#57351=CARTESIAN_POINT('Ctrl Pts',(2.86515629953528,-1.,2.59318160184921));
#57352=CARTESIAN_POINT('Ctrl Pts',(2.86515629953528,1.,2.59318160184921));
#57353=CARTESIAN_POINT('Ctrl Pts',(2.86081999003668,-1.,2.5869677064356));
#57354=CARTESIAN_POINT('Ctrl Pts',(2.86081999003668,1.,2.5869677064356));
#57355=CARTESIAN_POINT('Ctrl Pts',(2.85647171715147,-1.,2.58082875254407));
#57356=CARTESIAN_POINT('Ctrl Pts',(2.85647171715147,1.,2.58082875254407));
#57357=CARTESIAN_POINT('Ctrl Pts',(2.85215360144482,-1.,2.57480482727128));
#57358=CARTESIAN_POINT('Ctrl Pts',(2.85215360144482,1.,2.57480482727128));
#57359=CARTESIAN_POINT('Ctrl Pts',(2.84788893329091,-1.,2.56891984251743));
#57360=CARTESIAN_POINT('Ctrl Pts',(2.84788893329091,1.,2.56891984251743));
#57361=CARTESIAN_POINT('Ctrl Pts',(2.84366802680211,-1.,2.56316920798489));
#57362=CARTESIAN_POINT('Ctrl Pts',(2.84366802680211,1.,2.56316920798489));
#57363=CARTESIAN_POINT('Ctrl Pts',(2.83942515220699,-1.,2.55749952145165));
#57364=CARTESIAN_POINT('Ctrl Pts',(2.83942515220699,1.,2.55749952145165));
#57365=CARTESIAN_POINT('Ctrl Pts',(2.83505269592412,-1.,2.55182152806964));
#57366=CARTESIAN_POINT('Ctrl Pts',(2.83505269592412,1.,2.55182152806964));
#57367=CARTESIAN_POINT('Ctrl Pts',(2.83044254225794,-1.,2.54604736792542));
#57368=CARTESIAN_POINT('Ctrl Pts',(2.83044254225794,1.,2.54604736792542));
#57369=CARTESIAN_POINT('Ctrl Pts',(2.82552167649157,-1.,2.54012272520141));
#57370=CARTESIAN_POINT('Ctrl Pts',(2.82552167649157,1.,2.54012272520141));
#57371=CARTESIAN_POINT('Ctrl Pts',(2.82028550483744,-1.,2.53405679667463));
#57372=CARTESIAN_POINT('Ctrl Pts',(2.82028550483744,1.,2.53405679667463));
#57373=CARTESIAN_POINT('Ctrl Pts',(2.8148437904867,-1.,2.52796388055457));
#57374=CARTESIAN_POINT('Ctrl Pts',(2.8148437904867,1.,2.52796388055457));
#57375=CARTESIAN_POINT('Ctrl Pts',(2.80941521967234,-1.,2.52205778589922));
#57376=CARTESIAN_POINT('Ctrl Pts',(2.80941521967234,1.,2.52205778589922));
#57377=CARTESIAN_POINT('Ctrl Pts',(2.80427363984939,-1.,2.51660190466067));
#57378=CARTESIAN_POINT('Ctrl Pts',(2.80427363984939,1.,2.51660190466067));
#57379=CARTESIAN_POINT('Ctrl Pts',(2.79970585014308,-1.,2.51186983687947));
#57380=CARTESIAN_POINT('Ctrl Pts',(2.79970585014308,1.,2.51186983687947));
#57381=CARTESIAN_POINT('Ctrl Pts',(2.7959687805717,-1.,2.50810555977564));
#57382=CARTESIAN_POINT('Ctrl Pts',(2.7959687805717,1.,2.50810555977564));
#57383=CARTESIAN_POINT('Ctrl Pts',(2.79323694088143,-1.,2.50547439929077));
#57384=CARTESIAN_POINT('Ctrl Pts',(2.79323694088143,1.,2.50547439929077));
#57385=CARTESIAN_POINT('Ctrl Pts',(2.79192122906739,-1.,2.50433799076945));
#57386=CARTESIAN_POINT('Ctrl Pts',(2.79192122906739,1.,2.50433799076945));
#57387=CARTESIAN_POINT('Ctrl Pts',(2.79143626022225,-1.,2.50404230339032));
#57388=CARTESIAN_POINT('Ctrl Pts',(2.79143626022225,1.,2.50404230339032));
#57389=CARTESIAN_POINT('Ctrl Pts',(2.79133581100044,-1.,2.50409239460011));
#57390=CARTESIAN_POINT('Ctrl Pts',(2.79133581100044,1.,2.50409239460011));
#57391=CARTESIAN_POINT('Ctrl Pts',(2.79134130681569,-1.,2.50417924854921));
#57392=CARTESIAN_POINT('Ctrl Pts',(2.79134130681569,1.,2.50417924854921));
#57393=CARTESIAN_POINT('',(3.02314558451372,1.,2.91557726271063));
#57394=CARTESIAN_POINT('Ctrl Pts',(3.02314558451372,1.,2.91557726271063));
#57395=CARTESIAN_POINT('Ctrl Pts',(3.02261975104912,1.,2.91409518070707));
#57396=CARTESIAN_POINT('Ctrl Pts',(3.02156522743299,1.,2.91113297349052));
#57397=CARTESIAN_POINT('Ctrl Pts',(3.01997487194926,1.,2.90669553303902));
#57398=CARTESIAN_POINT('Ctrl Pts',(3.01783725123646,1.,2.90079069102661));
#57399=CARTESIAN_POINT('Ctrl Pts',(3.01513660433291,1.,2.8934292556764));
#57400=CARTESIAN_POINT('Ctrl Pts',(3.01240727309568,1.,2.88608751706796));
#57401=CARTESIAN_POINT('Ctrl Pts',(3.0096491810855,1.,2.87876560072799));
#57402=CARTESIAN_POINT('Ctrl Pts',(3.00686224485374,1.,2.87146368430104));
#57403=CARTESIAN_POINT('Ctrl Pts',(3.00404638316245,1.,2.86418200833065));
#57404=CARTESIAN_POINT('Ctrl Pts',(3.0012015079552,1.,2.85692085715129));
#57405=CARTESIAN_POINT('Ctrl Pts',(2.99832751144566,1.,2.84968053289104));
#57406=CARTESIAN_POINT('Ctrl Pts',(2.995424253416,1.,2.84246132984334));
#57407=CARTESIAN_POINT('Ctrl Pts',(2.99249155170479,1.,2.83526351254383));
#57408=CARTESIAN_POINT('Ctrl Pts',(2.98952916401699,1.,2.82808728190402));
#57409=CARTESIAN_POINT('Ctrl Pts',(2.98653680669434,1.,2.82093279065704));
#57410=CARTESIAN_POINT('Ctrl Pts',(2.9835141977994,1.,2.81380019196454));
#57411=CARTESIAN_POINT('Ctrl Pts',(2.98046109647299,1.,2.80668968101162));
#57412=CARTESIAN_POINT('Ctrl Pts',(2.97737733718242,1.,2.79960153278186));
#57413=CARTESIAN_POINT('Ctrl Pts',(2.97426288347475,1.,2.79253615718147));
#57414=CARTESIAN_POINT('Ctrl Pts',(2.97111781461349,1.,2.78549409123657));
#57415=CARTESIAN_POINT('Ctrl Pts',(2.9679422104295,1.,2.77847589542767));
#57416=CARTESIAN_POINT('Ctrl Pts',(2.96473605585548,1.,2.77148206836464));
#57417=CARTESIAN_POINT('Ctrl Pts',(2.96149914764832,1.,2.76451296269571));
#57418=CARTESIAN_POINT('Ctrl Pts',(2.9582309766594,1.,2.75756867888393));
#57419=CARTESIAN_POINT('Ctrl Pts',(2.95493069316211,1.,2.75064903318996));
#57420=CARTESIAN_POINT('Ctrl Pts',(2.95159737214304,1.,2.7437537949221));
#57421=CARTESIAN_POINT('Ctrl Pts',(2.94823023414381,1.,2.73688288329825));
#57422=CARTESIAN_POINT('Ctrl Pts',(2.94482887675139,1.,2.73003657371613));
#57423=CARTESIAN_POINT('Ctrl Pts',(2.94139351933882,1.,2.72321571511322));
#57424=CARTESIAN_POINT('Ctrl Pts',(2.93792519474955,1.,2.71642190053575));
#57425=CARTESIAN_POINT('Ctrl Pts',(2.93442516311167,1.,2.70965695523776));
#57426=CARTESIAN_POINT('Ctrl Pts',(2.93089438233746,1.,2.70292247416881));
#57427=CARTESIAN_POINT('Ctrl Pts',(2.92733294395268,1.,2.69621932864302));
#57428=CARTESIAN_POINT('Ctrl Pts',(2.92373955325876,1.,2.68954721165342));
#57429=CARTESIAN_POINT('Ctrl Pts',(2.92011090722152,1.,2.68290409279689));
#57430=CARTESIAN_POINT('Ctrl Pts',(2.91644290704281,1.,2.67628728855309));
#57431=CARTESIAN_POINT('Ctrl Pts',(2.91273193382876,1.,2.66969458792627));
#57432=CARTESIAN_POINT('Ctrl Pts',(2.90897617968921,1.,2.66312542616809));
#57433=CARTESIAN_POINT('Ctrl Pts',(2.90517678087467,1.,2.65658188464287));
#57434=CARTESIAN_POINT('Ctrl Pts',(2.90133950224879,1.,2.65007017365576));
#57435=CARTESIAN_POINT('Ctrl Pts',(2.89747231723361,1.,2.64359851684146));
#57436=CARTESIAN_POINT('Ctrl Pts',(2.89358228854557,1.,2.63717442263944));
#57437=CARTESIAN_POINT('Ctrl Pts',(2.88967244854243,1.,2.63080195420771));
#57438=CARTESIAN_POINT('Ctrl Pts',(2.88573922195049,1.,2.62447947640253));
#57439=CARTESIAN_POINT('Ctrl Pts',(2.88176821427502,1.,2.61819596473087));
#57440=CARTESIAN_POINT('Ctrl Pts',(2.87773881947885,1.,2.61193507170928));
#57441=CARTESIAN_POINT('Ctrl Pts',(2.87363176656475,1.,2.6056817788128));
#57442=CARTESIAN_POINT('Ctrl Pts',(2.86943633170712,1.,2.59942875223202));
#57443=CARTESIAN_POINT('Ctrl Pts',(2.86515629953528,1.,2.59318160184921));
#57444=CARTESIAN_POINT('Ctrl Pts',(2.86081999003668,1.,2.5869677064356));
#57445=CARTESIAN_POINT('Ctrl Pts',(2.85647171715147,1.,2.58082875254407));
#57446=CARTESIAN_POINT('Ctrl Pts',(2.85215360144482,1.,2.57480482727128));
#57447=CARTESIAN_POINT('Ctrl Pts',(2.84788893329091,1.,2.56891984251743));
#57448=CARTESIAN_POINT('Ctrl Pts',(2.84366802680211,1.,2.56316920798489));
#57449=CARTESIAN_POINT('Ctrl Pts',(2.83942515220699,1.,2.55749952145165));
#57450=CARTESIAN_POINT('Ctrl Pts',(2.83505269592412,1.,2.55182152806964));
#57451=CARTESIAN_POINT('Ctrl Pts',(2.83044254225794,1.,2.54604736792542));
#57452=CARTESIAN_POINT('Ctrl Pts',(2.82552167649157,1.,2.54012272520141));
#57453=CARTESIAN_POINT('Ctrl Pts',(2.82028550483744,1.,2.53405679667463));
#57454=CARTESIAN_POINT('Ctrl Pts',(2.8148437904867,1.,2.52796388055457));
#57455=CARTESIAN_POINT('Ctrl Pts',(2.80941521967234,1.,2.52205778589922));
#57456=CARTESIAN_POINT('Ctrl Pts',(2.80427363984939,1.,2.51660190466067));
#57457=CARTESIAN_POINT('Ctrl Pts',(2.79970585014308,1.,2.51186983687947));
#57458=CARTESIAN_POINT('Ctrl Pts',(2.7959687805717,1.,2.50810555977564));
#57459=CARTESIAN_POINT('Ctrl Pts',(2.79344192164204,1.,2.50567182569153));
#57460=CARTESIAN_POINT('Ctrl Pts',(2.79217568804874,1.,2.50455968395235));
#57461=CARTESIAN_POINT('Ctrl Pts',(2.79164172519039,1.,2.50417932839344));
#57462=CARTESIAN_POINT('Ctrl Pts',(2.79145823440899,1.,2.50410700351426));
#57463=CARTESIAN_POINT('Ctrl Pts',(2.79140942341378,1.,2.50410331873042));
#57464=CARTESIAN_POINT('',(3.02314558451372,0.,2.91557726271063));
#57465=CARTESIAN_POINT('Ctrl Pts',(2.5041792485492,-1.,2.79134130681569));
#57466=CARTESIAN_POINT('Ctrl Pts',(2.5041792485492,1.,2.79134130681569));
#57467=CARTESIAN_POINT('Ctrl Pts',(2.50409239460108,-1.,2.7913358110015));
#57468=CARTESIAN_POINT('Ctrl Pts',(2.50409239460108,1.,2.7913358110015));
#57469=CARTESIAN_POINT('Ctrl Pts',(2.50404230339286,-1.,2.79143626022503));
#57470=CARTESIAN_POINT('Ctrl Pts',(2.50404230339286,1.,2.79143626022503));
#57471=CARTESIAN_POINT('Ctrl Pts',(2.5043379907732,-1.,2.79192122907148));
#57472=CARTESIAN_POINT('Ctrl Pts',(2.5043379907732,1.,2.79192122907148));
#57473=CARTESIAN_POINT('Ctrl Pts',(2.50547439929414,-1.,2.7932369408851));
#57474=CARTESIAN_POINT('Ctrl Pts',(2.50547439929414,1.,2.7932369408851));
#57475=CARTESIAN_POINT('Ctrl Pts',(2.5081055597767,-1.,2.79596878057287));
#57476=CARTESIAN_POINT('Ctrl Pts',(2.5081055597767,1.,2.79596878057287));
#57477=CARTESIAN_POINT('Ctrl Pts',(2.51186983687818,-1.,2.79970585014168));
#57478=CARTESIAN_POINT('Ctrl Pts',(2.51186983687818,1.,2.79970585014168));
#57479=CARTESIAN_POINT('Ctrl Pts',(2.51660190465805,-1.,2.80427363984653));
#57480=CARTESIAN_POINT('Ctrl Pts',(2.51660190465805,1.,2.80427363984653));
#57481=CARTESIAN_POINT('Ctrl Pts',(2.52205778589653,-1.,2.80941521966941));
#57482=CARTESIAN_POINT('Ctrl Pts',(2.52205778589653,1.,2.80941521966941));
#57483=CARTESIAN_POINT('Ctrl Pts',(2.52796388055278,-1.,2.81484379048475));
#57484=CARTESIAN_POINT('Ctrl Pts',(2.52796388055278,1.,2.81484379048475));
#57485=CARTESIAN_POINT('Ctrl Pts',(2.53405679667412,-1.,2.82028550483689));
#57486=CARTESIAN_POINT('Ctrl Pts',(2.53405679667412,1.,2.82028550483689));
#57487=CARTESIAN_POINT('Ctrl Pts',(2.54012272520199,-1.,2.8255216764922));
#57488=CARTESIAN_POINT('Ctrl Pts',(2.54012272520199,1.,2.8255216764922));
#57489=CARTESIAN_POINT('Ctrl Pts',(2.54604736792655,-1.,2.83044254225917));
#57490=CARTESIAN_POINT('Ctrl Pts',(2.54604736792655,1.,2.83044254225917));
#57491=CARTESIAN_POINT('Ctrl Pts',(2.55182152807077,-1.,2.83505269592536));
#57492=CARTESIAN_POINT('Ctrl Pts',(2.55182152807077,1.,2.83505269592536));
#57493=CARTESIAN_POINT('Ctrl Pts',(2.55749952145241,-1.,2.83942515220782));
#57494=CARTESIAN_POINT('Ctrl Pts',(2.55749952145241,1.,2.83942515220782));
#57495=CARTESIAN_POINT('Ctrl Pts',(2.56316920798513,-1.,2.84366802680237));
#57496=CARTESIAN_POINT('Ctrl Pts',(2.56316920798513,1.,2.84366802680237));
#57497=CARTESIAN_POINT('Ctrl Pts',(2.56891984251721,-1.,2.84788893329067));
#57498=CARTESIAN_POINT('Ctrl Pts',(2.56891984251721,1.,2.84788893329067));
#57499=CARTESIAN_POINT('Ctrl Pts',(2.57480482727081,-1.,2.85215360144431));
#57500=CARTESIAN_POINT('Ctrl Pts',(2.57480482727081,1.,2.85215360144431));
#57501=CARTESIAN_POINT('Ctrl Pts',(2.58082875254357,-1.,2.85647171715092));
#57502=CARTESIAN_POINT('Ctrl Pts',(2.58082875254357,1.,2.85647171715092));
#57503=CARTESIAN_POINT('Ctrl Pts',(2.58696770643524,-1.,2.86081999003629));
#57504=CARTESIAN_POINT('Ctrl Pts',(2.58696770643524,1.,2.86081999003629));
#57505=CARTESIAN_POINT('Ctrl Pts',(2.59318160184908,-1.,2.86515629953513));
#57506=CARTESIAN_POINT('Ctrl Pts',(2.59318160184908,1.,2.86515629953513));
#57507=CARTESIAN_POINT('Ctrl Pts',(2.5994287522321,-1.,2.86943633170722));
#57508=CARTESIAN_POINT('Ctrl Pts',(2.5994287522321,1.,2.86943633170722));
#57509=CARTESIAN_POINT('Ctrl Pts',(2.60568177881303,-1.,2.87363176656501));
#57510=CARTESIAN_POINT('Ctrl Pts',(2.60568177881303,1.,2.87363176656501));
#57511=CARTESIAN_POINT('Ctrl Pts',(2.61193507170955,-1.,2.87773881947916));
#57512=CARTESIAN_POINT('Ctrl Pts',(2.61193507170955,1.,2.87773881947916));
#57513=CARTESIAN_POINT('Ctrl Pts',(2.61819596473108,-1.,2.88176821427525));
#57514=CARTESIAN_POINT('Ctrl Pts',(2.61819596473108,1.,2.88176821427525));
#57515=CARTESIAN_POINT('Ctrl Pts',(2.62447947640262,-1.,2.88573922195059));
#57516=CARTESIAN_POINT('Ctrl Pts',(2.62447947640262,1.,2.88573922195059));
#57517=CARTESIAN_POINT('Ctrl Pts',(2.63080195420767,-1.,2.88967244854239));
#57518=CARTESIAN_POINT('Ctrl Pts',(2.63080195420767,1.,2.88967244854239));
#57519=CARTESIAN_POINT('Ctrl Pts',(2.63717442263932,-1.,2.89358228854544));
#57520=CARTESIAN_POINT('Ctrl Pts',(2.63717442263932,1.,2.89358228854544));
#57521=CARTESIAN_POINT('Ctrl Pts',(2.64359851684131,-1.,2.89747231723345));
#57522=CARTESIAN_POINT('Ctrl Pts',(2.64359851684131,1.,2.89747231723345));
#57523=CARTESIAN_POINT('Ctrl Pts',(2.65007017365564,-1.,2.90133950224867));
#57524=CARTESIAN_POINT('Ctrl Pts',(2.65007017365564,1.,2.90133950224867));
#57525=CARTESIAN_POINT('Ctrl Pts',(2.65658188464282,-1.,2.90517678087461));
#57526=CARTESIAN_POINT('Ctrl Pts',(2.65658188464282,1.,2.90517678087461));
#57527=CARTESIAN_POINT('Ctrl Pts',(2.6631254261681,-1.,2.90897617968923));
#57528=CARTESIAN_POINT('Ctrl Pts',(2.6631254261681,1.,2.90897617968923));
#57529=CARTESIAN_POINT('Ctrl Pts',(2.66969458792631,-1.,2.91273193382882));
#57530=CARTESIAN_POINT('Ctrl Pts',(2.66969458792631,1.,2.91273193382882));
#57531=CARTESIAN_POINT('Ctrl Pts',(2.67628728855312,-1.,2.91644290704285));
#57532=CARTESIAN_POINT('Ctrl Pts',(2.67628728855312,1.,2.91644290704285));
#57533=CARTESIAN_POINT('Ctrl Pts',(2.68290409279688,-1.,2.92011090722152));
#57534=CARTESIAN_POINT('Ctrl Pts',(2.68290409279688,1.,2.92011090722152));
#57535=CARTESIAN_POINT('Ctrl Pts',(2.68954721165339,-1.,2.92373955325875));
#57536=CARTESIAN_POINT('Ctrl Pts',(2.68954721165339,1.,2.92373955325875));
#57537=CARTESIAN_POINT('Ctrl Pts',(2.69621932864301,-1.,2.92733294395267));
#57538=CARTESIAN_POINT('Ctrl Pts',(2.69621932864301,1.,2.92733294395267));
#57539=CARTESIAN_POINT('Ctrl Pts',(2.70292247416885,-1.,2.9308943823375));
#57540=CARTESIAN_POINT('Ctrl Pts',(2.70292247416885,1.,2.9308943823375));
#57541=CARTESIAN_POINT('Ctrl Pts',(2.70965695523787,-1.,2.93442516311179));
#57542=CARTESIAN_POINT('Ctrl Pts',(2.70965695523787,1.,2.93442516311179));
#57543=CARTESIAN_POINT('Ctrl Pts',(2.71642190053592,-1.,2.93792519474972));
#57544=CARTESIAN_POINT('Ctrl Pts',(2.71642190053592,1.,2.93792519474972));
#57545=CARTESIAN_POINT('Ctrl Pts',(2.72321571511337,-1.,2.94139351933897));
#57546=CARTESIAN_POINT('Ctrl Pts',(2.72321571511337,1.,2.94139351933897));
#57547=CARTESIAN_POINT('Ctrl Pts',(2.73003657371616,-1.,2.94482887675143));
#57548=CARTESIAN_POINT('Ctrl Pts',(2.73003657371616,1.,2.94482887675143));
#57549=CARTESIAN_POINT('Ctrl Pts',(2.73688288329808,-1.,2.94823023414364));
#57550=CARTESIAN_POINT('Ctrl Pts',(2.73688288329808,1.,2.94823023414364));
#57551=CARTESIAN_POINT('Ctrl Pts',(2.74375379492172,-1.,2.95159737214266));
#57552=CARTESIAN_POINT('Ctrl Pts',(2.74375379492172,1.,2.95159737214266));
#57553=CARTESIAN_POINT('Ctrl Pts',(2.75064903318947,-1.,2.95493069316161));
#57554=CARTESIAN_POINT('Ctrl Pts',(2.75064903318947,1.,2.95493069316161));
#57555=CARTESIAN_POINT('Ctrl Pts',(2.7575686788835,-1.,2.95823097665896));
#57556=CARTESIAN_POINT('Ctrl Pts',(2.7575686788835,1.,2.95823097665896));
#57557=CARTESIAN_POINT('Ctrl Pts',(2.76451296269557,-1.,2.96149914764818));
#57558=CARTESIAN_POINT('Ctrl Pts',(2.76451296269557,1.,2.96149914764818));
#57559=CARTESIAN_POINT('Ctrl Pts',(2.77148206836498,-1.,2.96473605585583));
#57560=CARTESIAN_POINT('Ctrl Pts',(2.77148206836498,1.,2.96473605585583));
#57561=CARTESIAN_POINT('Ctrl Pts',(2.7784758954285,-1.,2.96794221043036));
#57562=CARTESIAN_POINT('Ctrl Pts',(2.7784758954285,1.,2.96794221043036));
#57563=CARTESIAN_POINT('Ctrl Pts',(2.78549409123769,-1.,2.97111781461465));
#57564=CARTESIAN_POINT('Ctrl Pts',(2.78549409123769,1.,2.97111781461465));
#57565=CARTESIAN_POINT('Ctrl Pts',(2.79253615718248,-1.,2.9742628834758));
#57566=CARTESIAN_POINT('Ctrl Pts',(2.79253615718248,1.,2.9742628834758));
#57567=CARTESIAN_POINT('Ctrl Pts',(2.7996015327823,-1.,2.97737733718287));
#57568=CARTESIAN_POINT('Ctrl Pts',(2.7996015327823,1.,2.97737733718287));
#57569=CARTESIAN_POINT('Ctrl Pts',(2.80668968101106,-1.,2.98046109647241));
#57570=CARTESIAN_POINT('Ctrl Pts',(2.80668968101106,1.,2.98046109647241));
#57571=CARTESIAN_POINT('Ctrl Pts',(2.81380019196286,-1.,2.98351419779767));
#57572=CARTESIAN_POINT('Ctrl Pts',(2.81380019196286,1.,2.98351419779767));
#57573=CARTESIAN_POINT('Ctrl Pts',(2.82093279065457,-1.,2.9865368066918));
#57574=CARTESIAN_POINT('Ctrl Pts',(2.82093279065457,1.,2.9865368066918));
#57575=CARTESIAN_POINT('Ctrl Pts',(2.82808728190157,-1.,2.98952916401446));
#57576=CARTESIAN_POINT('Ctrl Pts',(2.82808728190157,1.,2.98952916401446));
#57577=CARTESIAN_POINT('Ctrl Pts',(2.83526351254248,-1.,2.9924915517034));
#57578=CARTESIAN_POINT('Ctrl Pts',(2.83526351254248,1.,2.9924915517034));
#57579=CARTESIAN_POINT('Ctrl Pts',(2.84246132984415,-1.,2.99542425341685));
#57580=CARTESIAN_POINT('Ctrl Pts',(2.84246132984415,1.,2.99542425341685));
#57581=CARTESIAN_POINT('Ctrl Pts',(2.84968053289451,-1.,2.99832751144925));
#57582=CARTESIAN_POINT('Ctrl Pts',(2.84968053289451,1.,2.99832751144925));
#57583=CARTESIAN_POINT('Ctrl Pts',(2.85692085715685,-1.,3.00120150796095));
#57584=CARTESIAN_POINT('Ctrl Pts',(2.85692085715685,1.,3.00120150796095));
#57585=CARTESIAN_POINT('Ctrl Pts',(2.86418200833667,-1.,3.00404638316867));
#57586=CARTESIAN_POINT('Ctrl Pts',(2.86418200833667,1.,3.00404638316867));
#57587=CARTESIAN_POINT('Ctrl Pts',(2.87146368430501,-1.,3.00686224485784));
#57588=CARTESIAN_POINT('Ctrl Pts',(2.87146368430501,1.,3.00686224485784));
#57589=CARTESIAN_POINT('Ctrl Pts',(2.87876560072727,-1.,3.00964918108476));
#57590=CARTESIAN_POINT('Ctrl Pts',(2.87876560072727,1.,3.00964918108476));
#57591=CARTESIAN_POINT('Ctrl Pts',(2.8860875170608,-1.,3.01240727308829));
#57592=CARTESIAN_POINT('Ctrl Pts',(2.8860875170608,1.,3.01240727308829));
#57593=CARTESIAN_POINT('Ctrl Pts',(2.89342925566321,-1.,3.01513660431928));
#57594=CARTESIAN_POINT('Ctrl Pts',(2.89342925566321,1.,3.01513660431928));
#57595=CARTESIAN_POINT('Ctrl Pts',(2.9007906910105,-1.,3.01783725121981));
#57596=CARTESIAN_POINT('Ctrl Pts',(2.9007906910105,1.,3.01783725121981));
#57597=CARTESIAN_POINT('Ctrl Pts',(2.90669553302526,-1.,3.01997487193503));
#57598=CARTESIAN_POINT('Ctrl Pts',(2.90669553302526,1.,3.01997487193503));
#57599=CARTESIAN_POINT('Ctrl Pts',(2.91113297348212,-1.,3.02156522742431));
#57600=CARTESIAN_POINT('Ctrl Pts',(2.91113297348212,1.,3.02156522742431));
#57601=CARTESIAN_POINT('Ctrl Pts',(2.91409518070399,-1.,3.02261975104593));
#57602=CARTESIAN_POINT('Ctrl Pts',(2.91409518070399,1.,3.02261975104593));
#57603=CARTESIAN_POINT('Ctrl Pts',(2.91557726271063,-1.,3.02314558451372));
#57604=CARTESIAN_POINT('Ctrl Pts',(2.91557726271063,1.,3.02314558451372));
#57605=CARTESIAN_POINT('',(2.50410331873176,1.,2.79140942341258));
#57606=CARTESIAN_POINT('Ctrl Pts',(2.50410331873176,-1.,2.79140942341258));
#57607=CARTESIAN_POINT('Ctrl Pts',(2.50410331873176,-0.666666666666667,
2.79140942341258));
#57608=CARTESIAN_POINT('Ctrl Pts',(2.50410331873176,-0.333333333333333,
2.79140942341258));
#57609=CARTESIAN_POINT('Ctrl Pts',(2.50410331873176,0.333333333333333,2.79140942341258));
#57610=CARTESIAN_POINT('Ctrl Pts',(2.50410331873176,0.666666666666667,2.79140942341258));
#57611=CARTESIAN_POINT('Ctrl Pts',(2.50410331873176,1.,2.79140942341258));
#57612=CARTESIAN_POINT('',(2.91557726271063,1.,3.02314558451372));
#57613=CARTESIAN_POINT('',(2.91557726271063,0.,3.02314558451372));
#57614=CARTESIAN_POINT('Ctrl Pts',(2.50410331873176,1.,2.79140942341258));
#57615=CARTESIAN_POINT('Ctrl Pts',(2.50410700351493,1.,2.79145823440781));
#57616=CARTESIAN_POINT('Ctrl Pts',(2.50417932839313,1.,2.79164172518905));
#57617=CARTESIAN_POINT('Ctrl Pts',(2.50455968395146,1.,2.79217568804755));
#57618=CARTESIAN_POINT('Ctrl Pts',(2.50567182569081,1.,2.79344192164147));
#57619=CARTESIAN_POINT('Ctrl Pts',(2.5081055597767,1.,2.79596878057287));
#57620=CARTESIAN_POINT('Ctrl Pts',(2.51186983687818,1.,2.79970585014168));
#57621=CARTESIAN_POINT('Ctrl Pts',(2.51660190465805,1.,2.80427363984653));
#57622=CARTESIAN_POINT('Ctrl Pts',(2.52205778589653,1.,2.80941521966941));
#57623=CARTESIAN_POINT('Ctrl Pts',(2.52796388055278,1.,2.81484379048475));
#57624=CARTESIAN_POINT('Ctrl Pts',(2.53405679667412,1.,2.82028550483689));
#57625=CARTESIAN_POINT('Ctrl Pts',(2.54012272520199,1.,2.8255216764922));
#57626=CARTESIAN_POINT('Ctrl Pts',(2.54604736792655,1.,2.83044254225917));
#57627=CARTESIAN_POINT('Ctrl Pts',(2.55182152807077,1.,2.83505269592536));
#57628=CARTESIAN_POINT('Ctrl Pts',(2.55749952145241,1.,2.83942515220782));
#57629=CARTESIAN_POINT('Ctrl Pts',(2.56316920798513,1.,2.84366802680237));
#57630=CARTESIAN_POINT('Ctrl Pts',(2.56891984251721,1.,2.84788893329067));
#57631=CARTESIAN_POINT('Ctrl Pts',(2.57480482727081,1.,2.85215360144431));
#57632=CARTESIAN_POINT('Ctrl Pts',(2.58082875254357,1.,2.85647171715092));
#57633=CARTESIAN_POINT('Ctrl Pts',(2.58696770643524,1.,2.86081999003629));
#57634=CARTESIAN_POINT('Ctrl Pts',(2.59318160184908,1.,2.86515629953513));
#57635=CARTESIAN_POINT('Ctrl Pts',(2.5994287522321,1.,2.86943633170722));
#57636=CARTESIAN_POINT('Ctrl Pts',(2.60568177881303,1.,2.87363176656501));
#57637=CARTESIAN_POINT('Ctrl Pts',(2.61193507170955,1.,2.87773881947916));
#57638=CARTESIAN_POINT('Ctrl Pts',(2.61819596473108,1.,2.88176821427525));
#57639=CARTESIAN_POINT('Ctrl Pts',(2.62447947640262,1.,2.88573922195059));
#57640=CARTESIAN_POINT('Ctrl Pts',(2.63080195420767,1.,2.88967244854239));
#57641=CARTESIAN_POINT('Ctrl Pts',(2.63717442263932,1.,2.89358228854544));
#57642=CARTESIAN_POINT('Ctrl Pts',(2.64359851684131,1.,2.89747231723345));
#57643=CARTESIAN_POINT('Ctrl Pts',(2.65007017365564,1.,2.90133950224867));
#57644=CARTESIAN_POINT('Ctrl Pts',(2.65658188464282,1.,2.90517678087461));
#57645=CARTESIAN_POINT('Ctrl Pts',(2.6631254261681,1.,2.90897617968923));
#57646=CARTESIAN_POINT('Ctrl Pts',(2.66969458792631,1.,2.91273193382882));
#57647=CARTESIAN_POINT('Ctrl Pts',(2.67628728855312,1.,2.91644290704285));
#57648=CARTESIAN_POINT('Ctrl Pts',(2.68290409279688,1.,2.92011090722152));
#57649=CARTESIAN_POINT('Ctrl Pts',(2.68954721165339,1.,2.92373955325875));
#57650=CARTESIAN_POINT('Ctrl Pts',(2.69621932864301,1.,2.92733294395267));
#57651=CARTESIAN_POINT('Ctrl Pts',(2.70292247416885,1.,2.9308943823375));
#57652=CARTESIAN_POINT('Ctrl Pts',(2.70965695523787,1.,2.93442516311179));
#57653=CARTESIAN_POINT('Ctrl Pts',(2.71642190053592,1.,2.93792519474972));
#57654=CARTESIAN_POINT('Ctrl Pts',(2.72321571511337,1.,2.94139351933897));
#57655=CARTESIAN_POINT('Ctrl Pts',(2.73003657371616,1.,2.94482887675143));
#57656=CARTESIAN_POINT('Ctrl Pts',(2.73688288329808,1.,2.94823023414364));
#57657=CARTESIAN_POINT('Ctrl Pts',(2.74375379492172,1.,2.95159737214266));
#57658=CARTESIAN_POINT('Ctrl Pts',(2.75064903318947,1.,2.95493069316161));
#57659=CARTESIAN_POINT('Ctrl Pts',(2.7575686788835,1.,2.95823097665896));
#57660=CARTESIAN_POINT('Ctrl Pts',(2.76451296269557,1.,2.96149914764818));
#57661=CARTESIAN_POINT('Ctrl Pts',(2.77148206836498,1.,2.96473605585583));
#57662=CARTESIAN_POINT('Ctrl Pts',(2.7784758954285,1.,2.96794221043036));
#57663=CARTESIAN_POINT('Ctrl Pts',(2.78549409123769,1.,2.97111781461465));
#57664=CARTESIAN_POINT('Ctrl Pts',(2.79253615718248,1.,2.9742628834758));
#57665=CARTESIAN_POINT('Ctrl Pts',(2.7996015327823,1.,2.97737733718287));
#57666=CARTESIAN_POINT('Ctrl Pts',(2.80668968101106,1.,2.98046109647241));
#57667=CARTESIAN_POINT('Ctrl Pts',(2.81380019196286,1.,2.98351419779767));
#57668=CARTESIAN_POINT('Ctrl Pts',(2.82093279065457,1.,2.9865368066918));
#57669=CARTESIAN_POINT('Ctrl Pts',(2.82808728190157,1.,2.98952916401446));
#57670=CARTESIAN_POINT('Ctrl Pts',(2.83526351254248,1.,2.9924915517034));
#57671=CARTESIAN_POINT('Ctrl Pts',(2.84246132984415,1.,2.99542425341685));
#57672=CARTESIAN_POINT('Ctrl Pts',(2.84968053289451,1.,2.99832751144925));
#57673=CARTESIAN_POINT('Ctrl Pts',(2.85692085715685,1.,3.00120150796095));
#57674=CARTESIAN_POINT('Ctrl Pts',(2.86418200833667,1.,3.00404638316867));
#57675=CARTESIAN_POINT('Ctrl Pts',(2.87146368430501,1.,3.00686224485784));
#57676=CARTESIAN_POINT('Ctrl Pts',(2.87876560072727,1.,3.00964918108476));
#57677=CARTESIAN_POINT('Ctrl Pts',(2.8860875170608,1.,3.01240727308829));
#57678=CARTESIAN_POINT('Ctrl Pts',(2.89342925566321,1.,3.01513660431928));
#57679=CARTESIAN_POINT('Ctrl Pts',(2.9007906910105,1.,3.01783725121981));
#57680=CARTESIAN_POINT('Ctrl Pts',(2.90669553302526,1.,3.01997487193503));
#57681=CARTESIAN_POINT('Ctrl Pts',(2.91113297348212,1.,3.02156522742431));
#57682=CARTESIAN_POINT('Ctrl Pts',(2.91409518070399,1.,3.02261975104593));
#57683=CARTESIAN_POINT('Ctrl Pts',(2.91557726271063,1.,3.02314558451372));
#57684=CARTESIAN_POINT('Origin',(2.91557726271063,0.,3.02314558451372));
#57685=CARTESIAN_POINT('',(3.02314558451372,1.,2.91557726271063));
#57686=CARTESIAN_POINT('Origin',(0.,0.,0.));
#57687=CARTESIAN_POINT('',(2.36531447826213,1.,2.90994629141562));
#57688=CARTESIAN_POINT('Origin',(0.,1.,0.));
#57689=CARTESIAN_POINT('Ctrl Pts',(2.36531447826213,1.,2.90994629141563));
#57690=CARTESIAN_POINT('Ctrl Pts',(2.36531447826213,0.666666666666667,2.90994629141563));
#57691=CARTESIAN_POINT('Ctrl Pts',(2.36531447826213,0.333333333333333,2.90994629141563));
#57692=CARTESIAN_POINT('Ctrl Pts',(2.36531447826213,-0.333333333333333,
2.90994629141563));
#57693=CARTESIAN_POINT('Ctrl Pts',(2.36531447826213,-0.666666666666667,
2.90994629141563));
#57694=CARTESIAN_POINT('Ctrl Pts',(2.36531447826213,-1.,2.90994629141563));
#57695=CARTESIAN_POINT('Ctrl Pts',(2.52982887637028,-1.,3.35260583073571));
#57696=CARTESIAN_POINT('Ctrl Pts',(2.52982887637028,1.,3.35260583073571));
#57697=CARTESIAN_POINT('Ctrl Pts',(2.52954136549357,-1.,3.35105973714426));
#57698=CARTESIAN_POINT('Ctrl Pts',(2.52954136549357,1.,3.35105973714426));
#57699=CARTESIAN_POINT('Ctrl Pts',(2.5289632161143,-1.,3.34796903577628));
#57700=CARTESIAN_POINT('Ctrl Pts',(2.5289632161143,1.,3.34796903577628));
#57701=CARTESIAN_POINT('Ctrl Pts',(2.52808660916879,-1.,3.34333744117093));
#57702=CARTESIAN_POINT('Ctrl Pts',(2.52808660916879,1.,3.34333744117093));
#57703=CARTESIAN_POINT('Ctrl Pts',(2.52689902691551,-1.,3.33717090000955));
#57704=CARTESIAN_POINT('Ctrl Pts',(2.52689902691551,1.,3.33717090000955));
#57705=CARTESIAN_POINT('Ctrl Pts',(2.52538321165774,-1.,3.32947762189049));
#57706=CARTESIAN_POINT('Ctrl Pts',(2.52538321165774,1.,3.32947762189049));
#57707=CARTESIAN_POINT('Ctrl Pts',(2.52383598396878,-1.,3.32179931079521));
#57708=CARTESIAN_POINT('Ctrl Pts',(2.52383598396878,1.,3.32179931079521));
#57709=CARTESIAN_POINT('Ctrl Pts',(2.52225724871375,-1.,3.31413607874727));
#57710=CARTESIAN_POINT('Ctrl Pts',(2.52225724871375,1.,3.31413607874727));
#57711=CARTESIAN_POINT('Ctrl Pts',(2.52064689568167,-1.,3.30648808814986));
#57712=CARTESIAN_POINT('Ctrl Pts',(2.52064689568167,1.,3.30648808814986));
#57713=CARTESIAN_POINT('Ctrl Pts',(2.51900480700548,-1.,3.29885556387661));
#57714=CARTESIAN_POINT('Ctrl Pts',(2.51900480700548,1.,3.29885556387661));
#57715=CARTESIAN_POINT('Ctrl Pts',(2.51733085123316,-1.,3.2912387729863));
#57716=CARTESIAN_POINT('Ctrl Pts',(2.51733085123316,1.,3.2912387729863));
#57717=CARTESIAN_POINT('Ctrl Pts',(2.51562487464214,-1.,3.28363799702583));
#57718=CARTESIAN_POINT('Ctrl Pts',(2.51562487464214,1.,3.28363799702583));
#57719=CARTESIAN_POINT('Ctrl Pts',(2.51388669270329,-1.,3.27605350473048));
#57720=CARTESIAN_POINT('Ctrl Pts',(2.51388669270329,1.,3.27605350473048));
#57721=CARTESIAN_POINT('Ctrl Pts',(2.51211608411539,-1.,3.26848552888271));
#57722=CARTESIAN_POINT('Ctrl Pts',(2.51211608411539,1.,3.26848552888271));
#57723=CARTESIAN_POINT('Ctrl Pts',(2.51031277813697,-1.,3.26093423001716));
#57724=CARTESIAN_POINT('Ctrl Pts',(2.51031277813697,1.,3.26093423001716));
#57725=CARTESIAN_POINT('Ctrl Pts',(2.50847647070936,-1.,3.25339971461265));
#57726=CARTESIAN_POINT('Ctrl Pts',(2.50847647070936,1.,3.25339971461265));
#57727=CARTESIAN_POINT('Ctrl Pts',(2.50660685940645,-1.,3.24588208984042));
#57728=CARTESIAN_POINT('Ctrl Pts',(2.50660685940645,1.,3.24588208984042));
#57729=CARTESIAN_POINT('Ctrl Pts',(2.50470367580078,-1.,3.23838151080383));
#57730=CARTESIAN_POINT('Ctrl Pts',(2.50470367580078,1.,3.23838151080383));
#57731=CARTESIAN_POINT('Ctrl Pts',(2.50276671338074,-1.,3.23089822320596));
#57732=CARTESIAN_POINT('Ctrl Pts',(2.50276671338074,1.,3.23089822320596));
#57733=CARTESIAN_POINT('Ctrl Pts',(2.5007958720187,-1.,3.22343262620387));
#57734=CARTESIAN_POINT('Ctrl Pts',(2.5007958720187,1.,3.22343262620387));
#57735=CARTESIAN_POINT('Ctrl Pts',(2.49879114599293,-1.,3.21598526261157));
#57736=CARTESIAN_POINT('Ctrl Pts',(2.49879114599293,1.,3.21598526261157));
#57737=CARTESIAN_POINT('Ctrl Pts',(2.49675252647298,-1.,3.2085566984974));
#57738=CARTESIAN_POINT('Ctrl Pts',(2.49675252647298,1.,3.2085566984974));
#57739=CARTESIAN_POINT('Ctrl Pts',(2.49467992057726,-1.,3.20114742397549));
#57740=CARTESIAN_POINT('Ctrl Pts',(2.49467992057726,1.,3.20114742397549));
#57741=CARTESIAN_POINT('Ctrl Pts',(2.4925730723986,-1.,3.19375775555814));
#57742=CARTESIAN_POINT('Ctrl Pts',(2.4925730723986,1.,3.19375775555814));
#57743=CARTESIAN_POINT('Ctrl Pts',(2.49043146334095,-1.,3.18638771282315));
#57744=CARTESIAN_POINT('Ctrl Pts',(2.49043146334095,1.,3.18638771282315));
#57745=CARTESIAN_POINT('Ctrl Pts',(2.48825428288242,-1.,3.17903698136679));
#57746=CARTESIAN_POINT('Ctrl Pts',(2.48825428288242,1.,3.17903698136679));
#57747=CARTESIAN_POINT('Ctrl Pts',(2.48604065348619,-1.,3.17170518863357));
#57748=CARTESIAN_POINT('Ctrl Pts',(2.48604065348619,1.,3.17170518863357));
#57749=CARTESIAN_POINT('Ctrl Pts',(2.48378981792739,-1.,3.16439213290181));
#57750=CARTESIAN_POINT('Ctrl Pts',(2.48378981792739,1.,3.16439213290181));
#57751=CARTESIAN_POINT('Ctrl Pts',(2.48150133566568,-1.,3.15709802322735));
#57752=CARTESIAN_POINT('Ctrl Pts',(2.48150133566568,1.,3.15709802322735));
#57753=CARTESIAN_POINT('Ctrl Pts',(2.47917529057016,-1.,3.14982373241335));
#57754=CARTESIAN_POINT('Ctrl Pts',(2.47917529057016,1.,3.14982373241335));
#57755=CARTESIAN_POINT('Ctrl Pts',(2.47681245356095,-1.,3.14257099546531));
#57756=CARTESIAN_POINT('Ctrl Pts',(2.47681245356095,1.,3.14257099546531));
#57757=CARTESIAN_POINT('Ctrl Pts',(2.47441378371923,-1.,3.13534181229282));
#57758=CARTESIAN_POINT('Ctrl Pts',(2.47441378371923,1.,3.13534181229282));
#57759=CARTESIAN_POINT('Ctrl Pts',(2.47197997765868,-1.,3.12813790805948));
#57760=CARTESIAN_POINT('Ctrl Pts',(2.47197997765868,1.,3.12813790805948));
#57761=CARTESIAN_POINT('Ctrl Pts',(2.4695109894747,-1.,3.12096015766984));
#57762=CARTESIAN_POINT('Ctrl Pts',(2.4695109894747,1.,3.12096015766984));
#57763=CARTESIAN_POINT('Ctrl Pts',(2.46700558843507,-1.,3.11380805536124));
#57764=CARTESIAN_POINT('Ctrl Pts',(2.46700558843507,1.,3.11380805536124));
#57765=CARTESIAN_POINT('Ctrl Pts',(2.46446082979645,-1.,3.10667907901981));
#57766=CARTESIAN_POINT('Ctrl Pts',(2.46446082979645,1.,3.10667907901981));
#57767=CARTESIAN_POINT('Ctrl Pts',(2.4618730850188,-1.,3.09956993697048));
#57768=CARTESIAN_POINT('Ctrl Pts',(2.4618730850188,1.,3.09956993697048));
#57769=CARTESIAN_POINT('Ctrl Pts',(2.45923912563875,-1.,3.09247787931881));
#57770=CARTESIAN_POINT('Ctrl Pts',(2.45923912563875,1.,3.09247787931881));
#57771=CARTESIAN_POINT('Ctrl Pts',(2.45655725437037,-1.,3.08540206545313));
#57772=CARTESIAN_POINT('Ctrl Pts',(2.45655725437037,1.,3.08540206545313));
#57773=CARTESIAN_POINT('Ctrl Pts',(2.45382826787795,-1.,3.07834472886145));
#57774=CARTESIAN_POINT('Ctrl Pts',(2.45382826787795,1.,3.07834472886145));
#57775=CARTESIAN_POINT('Ctrl Pts',(2.45105688854432,-1.,3.0713129052131));
#57776=CARTESIAN_POINT('Ctrl Pts',(2.45105688854432,1.,3.0713129052131));
#57777=CARTESIAN_POINT('Ctrl Pts',(2.44824970516557,-1.,3.06431596421422));
#57778=CARTESIAN_POINT('Ctrl Pts',(2.44824970516557,1.,3.06431596421422));
#57779=CARTESIAN_POINT('Ctrl Pts',(2.44541251892568,-1.,3.05736242671521));
#57780=CARTESIAN_POINT('Ctrl Pts',(2.44541251892568,1.,3.05736242671521));
#57781=CARTESIAN_POINT('Ctrl Pts',(2.44254768923109,-1.,3.05045678021509));
#57782=CARTESIAN_POINT('Ctrl Pts',(2.44254768923109,1.,3.05045678021509));
#57783=CARTESIAN_POINT('Ctrl Pts',(2.43965194061849,-1.,3.04359685040545));
#57784=CARTESIAN_POINT('Ctrl Pts',(2.43965194061849,1.,3.04359685040545));
#57785=CARTESIAN_POINT('Ctrl Pts',(2.43671278042394,-1.,3.03676949672797));
#57786=CARTESIAN_POINT('Ctrl Pts',(2.43671278042394,1.,3.03676949672797));
#57787=CARTESIAN_POINT('Ctrl Pts',(2.43371241361462,-1.,3.02995534946946));
#57788=CARTESIAN_POINT('Ctrl Pts',(2.43371241361462,1.,3.02995534946946));
#57789=CARTESIAN_POINT('Ctrl Pts',(2.43063415586615,-1.,3.02313656035977));
#57790=CARTESIAN_POINT('Ctrl Pts',(2.43063415586615,1.,3.02313656035977));
#57791=CARTESIAN_POINT('Ctrl Pts',(2.4274685626416,-1.,3.01630420830494));
#57792=CARTESIAN_POINT('Ctrl Pts',(2.4274685626416,1.,3.01630420830494));
#57793=CARTESIAN_POINT('Ctrl Pts',(2.42421849439625,-1.,3.00946442616674));
#57794=CARTESIAN_POINT('Ctrl Pts',(2.42421849439625,1.,3.00946442616674));
#57795=CARTESIAN_POINT('Ctrl Pts',(2.42090763946812,-1.,3.00264868586038));
#57796=CARTESIAN_POINT('Ctrl Pts',(2.42090763946812,1.,3.00264868586038));
#57797=CARTESIAN_POINT('Ctrl Pts',(2.4175732450056,-1.,2.99590509293561));
#57798=CARTESIAN_POINT('Ctrl Pts',(2.4175732450056,1.,2.99590509293561));
#57799=CARTESIAN_POINT('Ctrl Pts',(2.4142506419963,-1.,2.98927983005851));
#57800=CARTESIAN_POINT('Ctrl Pts',(2.4142506419963,1.,2.98927983005851));
#57801=CARTESIAN_POINT('Ctrl Pts',(2.41095909342591,-1.,2.98280015815132));
#57802=CARTESIAN_POINT('Ctrl Pts',(2.41095909342591,1.,2.98280015815132));
#57803=CARTESIAN_POINT('Ctrl Pts',(2.40768975073691,-1.,2.97646002822395));
#57804=CARTESIAN_POINT('Ctrl Pts',(2.40768975073691,1.,2.97646002822395));
#57805=CARTESIAN_POINT('Ctrl Pts',(2.40438604734848,-1.,2.97019641312272));
#57806=CARTESIAN_POINT('Ctrl Pts',(2.40438604734848,1.,2.97019641312272));
#57807=CARTESIAN_POINT('Ctrl Pts',(2.40095565711535,-1.,2.96390432240181));
#57808=CARTESIAN_POINT('Ctrl Pts',(2.40095565711535,1.,2.96390432240181));
#57809=CARTESIAN_POINT('Ctrl Pts',(2.39730553974412,-1.,2.95748006482811));
#57810=CARTESIAN_POINT('Ctrl Pts',(2.39730553974412,1.,2.95748006482811));
#57811=CARTESIAN_POINT('Ctrl Pts',(2.39337207631613,-1.,2.95085857128372));
#57812=CARTESIAN_POINT('Ctrl Pts',(2.39337207631613,1.,2.95085857128372));
#57813=CARTESIAN_POINT('Ctrl Pts',(2.38914929090806,-1.,2.94404820669135));
#57814=CARTESIAN_POINT('Ctrl Pts',(2.38914929090806,1.,2.94404820669135));
#57815=CARTESIAN_POINT('Ctrl Pts',(2.38472771516476,-1.,2.93717903280599));
#57816=CARTESIAN_POINT('Ctrl Pts',(2.38472771516476,1.,2.93717903280599));
#57817=CARTESIAN_POINT('Ctrl Pts',(2.3802898958232,-1.,2.93049643640517));
#57818=CARTESIAN_POINT('Ctrl Pts',(2.3802898958232,1.,2.93049643640517));
#57819=CARTESIAN_POINT('Ctrl Pts',(2.37606510524271,-1.,2.92430340582912));
#57820=CARTESIAN_POINT('Ctrl Pts',(2.37606510524271,1.,2.92430340582912));
#57821=CARTESIAN_POINT('Ctrl Pts',(2.37229381109939,-1.,2.9189150379156));
#57822=CARTESIAN_POINT('Ctrl Pts',(2.37229381109939,1.,2.9189150379156));
#57823=CARTESIAN_POINT('Ctrl Pts',(2.36919161373074,-1.,2.91461249883016));
#57824=CARTESIAN_POINT('Ctrl Pts',(2.36919161373074,1.,2.91461249883016));
#57825=CARTESIAN_POINT('Ctrl Pts',(2.36690501170317,-1.,2.9115863784165));
#57826=CARTESIAN_POINT('Ctrl Pts',(2.36690501170317,1.,2.9115863784165));
#57827=CARTESIAN_POINT('Ctrl Pts',(2.36578327194396,-1.,2.91025813829606));
#57828=CARTESIAN_POINT('Ctrl Pts',(2.36578327194396,1.,2.91025813829606));
#57829=CARTESIAN_POINT('Ctrl Pts',(2.36535052956704,-1.,2.90989022547738));
#57830=CARTESIAN_POINT('Ctrl Pts',(2.36535052956704,1.,2.90989022547738));
#57831=CARTESIAN_POINT('Ctrl Pts',(2.36524348105023,-1.,2.90992398626098));
#57832=CARTESIAN_POINT('Ctrl Pts',(2.36524348105023,1.,2.90992398626098));
#57833=CARTESIAN_POINT('Ctrl Pts',(2.36523532225181,-1.,2.91001063062876));
#57834=CARTESIAN_POINT('Ctrl Pts',(2.36523532225181,1.,2.91001063062876));
#57835=CARTESIAN_POINT('',(2.52982887637028,1.,3.35260583073571));
#57836=CARTESIAN_POINT('Ctrl Pts',(2.52982887637028,1.,3.35260583073571));
#57837=CARTESIAN_POINT('Ctrl Pts',(2.52954136549357,1.,3.35105973714426));
#57838=CARTESIAN_POINT('Ctrl Pts',(2.5289632161143,1.,3.34796903577628));
#57839=CARTESIAN_POINT('Ctrl Pts',(2.52808660916879,1.,3.34333744117093));
#57840=CARTESIAN_POINT('Ctrl Pts',(2.52689902691551,1.,3.33717090000955));
#57841=CARTESIAN_POINT('Ctrl Pts',(2.52538321165774,1.,3.32947762189049));
#57842=CARTESIAN_POINT('Ctrl Pts',(2.52383598396878,1.,3.32179931079521));
#57843=CARTESIAN_POINT('Ctrl Pts',(2.52225724871375,1.,3.31413607874727));
#57844=CARTESIAN_POINT('Ctrl Pts',(2.52064689568167,1.,3.30648808814986));
#57845=CARTESIAN_POINT('Ctrl Pts',(2.51900480700548,1.,3.29885556387661));
#57846=CARTESIAN_POINT('Ctrl Pts',(2.51733085123316,1.,3.2912387729863));
#57847=CARTESIAN_POINT('Ctrl Pts',(2.51562487464214,1.,3.28363799702583));
#57848=CARTESIAN_POINT('Ctrl Pts',(2.51388669270329,1.,3.27605350473048));
#57849=CARTESIAN_POINT('Ctrl Pts',(2.51211608411539,1.,3.26848552888271));
#57850=CARTESIAN_POINT('Ctrl Pts',(2.51031277813697,1.,3.26093423001716));
#57851=CARTESIAN_POINT('Ctrl Pts',(2.50847647070936,1.,3.25339971461265));
#57852=CARTESIAN_POINT('Ctrl Pts',(2.50660685940645,1.,3.24588208984042));
#57853=CARTESIAN_POINT('Ctrl Pts',(2.50470367580078,1.,3.23838151080383));
#57854=CARTESIAN_POINT('Ctrl Pts',(2.50276671338074,1.,3.23089822320596));
#57855=CARTESIAN_POINT('Ctrl Pts',(2.5007958720187,1.,3.22343262620387));
#57856=CARTESIAN_POINT('Ctrl Pts',(2.49879114599293,1.,3.21598526261157));
#57857=CARTESIAN_POINT('Ctrl Pts',(2.49675252647298,1.,3.2085566984974));
#57858=CARTESIAN_POINT('Ctrl Pts',(2.49467992057726,1.,3.20114742397549));
#57859=CARTESIAN_POINT('Ctrl Pts',(2.4925730723986,1.,3.19375775555814));
#57860=CARTESIAN_POINT('Ctrl Pts',(2.49043146334095,1.,3.18638771282315));
#57861=CARTESIAN_POINT('Ctrl Pts',(2.48825428288242,1.,3.17903698136679));
#57862=CARTESIAN_POINT('Ctrl Pts',(2.48604065348619,1.,3.17170518863357));
#57863=CARTESIAN_POINT('Ctrl Pts',(2.48378981792739,1.,3.16439213290181));
#57864=CARTESIAN_POINT('Ctrl Pts',(2.48150133566568,1.,3.15709802322735));
#57865=CARTESIAN_POINT('Ctrl Pts',(2.47917529057016,1.,3.14982373241335));
#57866=CARTESIAN_POINT('Ctrl Pts',(2.47681245356095,1.,3.14257099546531));
#57867=CARTESIAN_POINT('Ctrl Pts',(2.47441378371923,1.,3.13534181229282));
#57868=CARTESIAN_POINT('Ctrl Pts',(2.47197997765868,1.,3.12813790805948));
#57869=CARTESIAN_POINT('Ctrl Pts',(2.4695109894747,1.,3.12096015766984));
#57870=CARTESIAN_POINT('Ctrl Pts',(2.46700558843507,1.,3.11380805536124));
#57871=CARTESIAN_POINT('Ctrl Pts',(2.46446082979645,1.,3.10667907901981));
#57872=CARTESIAN_POINT('Ctrl Pts',(2.4618730850188,1.,3.09956993697048));
#57873=CARTESIAN_POINT('Ctrl Pts',(2.45923912563875,1.,3.09247787931881));
#57874=CARTESIAN_POINT('Ctrl Pts',(2.45655725437037,1.,3.08540206545313));
#57875=CARTESIAN_POINT('Ctrl Pts',(2.45382826787795,1.,3.07834472886145));
#57876=CARTESIAN_POINT('Ctrl Pts',(2.45105688854432,1.,3.0713129052131));
#57877=CARTESIAN_POINT('Ctrl Pts',(2.44824970516557,1.,3.06431596421422));
#57878=CARTESIAN_POINT('Ctrl Pts',(2.44541251892568,1.,3.05736242671521));
#57879=CARTESIAN_POINT('Ctrl Pts',(2.44254768923109,1.,3.05045678021509));
#57880=CARTESIAN_POINT('Ctrl Pts',(2.43965194061849,1.,3.04359685040545));
#57881=CARTESIAN_POINT('Ctrl Pts',(2.43671278042394,1.,3.03676949672797));
#57882=CARTESIAN_POINT('Ctrl Pts',(2.43371241361462,1.,3.02995534946946));
#57883=CARTESIAN_POINT('Ctrl Pts',(2.43063415586615,1.,3.02313656035977));
#57884=CARTESIAN_POINT('Ctrl Pts',(2.4274685626416,1.,3.01630420830494));
#57885=CARTESIAN_POINT('Ctrl Pts',(2.42421849439625,1.,3.00946442616674));
#57886=CARTESIAN_POINT('Ctrl Pts',(2.42090763946812,1.,3.00264868586038));
#57887=CARTESIAN_POINT('Ctrl Pts',(2.4175732450056,1.,2.99590509293561));
#57888=CARTESIAN_POINT('Ctrl Pts',(2.4142506419963,1.,2.98927983005851));
#57889=CARTESIAN_POINT('Ctrl Pts',(2.41095909342591,1.,2.98280015815132));
#57890=CARTESIAN_POINT('Ctrl Pts',(2.40768975073691,1.,2.97646002822395));
#57891=CARTESIAN_POINT('Ctrl Pts',(2.40438604734848,1.,2.97019641312272));
#57892=CARTESIAN_POINT('Ctrl Pts',(2.40095565711535,1.,2.96390432240181));
#57893=CARTESIAN_POINT('Ctrl Pts',(2.39730553974412,1.,2.95748006482811));
#57894=CARTESIAN_POINT('Ctrl Pts',(2.39337207631613,1.,2.95085857128372));
#57895=CARTESIAN_POINT('Ctrl Pts',(2.38914929090806,1.,2.94404820669135));
#57896=CARTESIAN_POINT('Ctrl Pts',(2.38472771516476,1.,2.93717903280599));
#57897=CARTESIAN_POINT('Ctrl Pts',(2.3802898958232,1.,2.93049643640517));
#57898=CARTESIAN_POINT('Ctrl Pts',(2.37606510524271,1.,2.92430340582912));
#57899=CARTESIAN_POINT('Ctrl Pts',(2.37229381109939,1.,2.9189150379156));
#57900=CARTESIAN_POINT('Ctrl Pts',(2.36919161373074,1.,2.91461249883016));
#57901=CARTESIAN_POINT('Ctrl Pts',(2.36707658451709,1.,2.91181344022628));
#57902=CARTESIAN_POINT('Ctrl Pts',(2.36599991765853,1.,2.91051690822262));
#57903=CARTESIAN_POINT('Ctrl Pts',(2.36553202948741,1.,2.91005770527771));
#57904=CARTESIAN_POINT('Ctrl Pts',(2.3653621118858,1.,2.90995756655559));
#57905=CARTESIAN_POINT('Ctrl Pts',(2.36531447826213,1.,2.90994629141563));
#57906=CARTESIAN_POINT('',(2.52982887637028,0.,3.35260583073571));
#57907=CARTESIAN_POINT('Ctrl Pts',(2.03668666247593,-1.,3.1487152044751));
#57908=CARTESIAN_POINT('Ctrl Pts',(2.03668666247593,1.,3.1487152044751));
#57909=CARTESIAN_POINT('Ctrl Pts',(2.03660173757879,-1.,3.14869618937258));
#57910=CARTESIAN_POINT('Ctrl Pts',(2.03660173757879,1.,3.14869618937258));
#57911=CARTESIAN_POINT('Ctrl Pts',(2.03653654935591,-1.,3.14878756590812));
#57912=CARTESIAN_POINT('Ctrl Pts',(2.03653654935591,1.,3.14878756590812));
#57913=CARTESIAN_POINT('Ctrl Pts',(2.03675273049189,-1.,3.14931281968048));
#57914=CARTESIAN_POINT('Ctrl Pts',(2.03675273049189,1.,3.14931281968048));
#57915=CARTESIAN_POINT('Ctrl Pts',(2.03766932526445,-1.,3.15079010635742));
#57916=CARTESIAN_POINT('Ctrl Pts',(2.03766932526445,1.,3.15079010635742));
#57917=CARTESIAN_POINT('Ctrl Pts',(2.03984073791519,-1.,3.15389991674792));
#57918=CARTESIAN_POINT('Ctrl Pts',(2.03984073791519,1.,3.15389991674792));
#57919=CARTESIAN_POINT('Ctrl Pts',(2.04297406404027,-1.,3.15817983946367));
#57920=CARTESIAN_POINT('Ctrl Pts',(2.04297406404027,1.,3.15817983946367));
#57921=CARTESIAN_POINT('Ctrl Pts',(2.04693331247446,-1.,3.16343165058912));
#57922=CARTESIAN_POINT('Ctrl Pts',(2.04693331247446,1.,3.16343165058912));
#57923=CARTESIAN_POINT('Ctrl Pts',(2.05151770247233,-1.,3.16936341689527));
#57924=CARTESIAN_POINT('Ctrl Pts',(2.05151770247233,1.,3.16936341689527));
#57925=CARTESIAN_POINT('Ctrl Pts',(2.05650186773132,-1.,3.17564906975371));
#57926=CARTESIAN_POINT('Ctrl Pts',(2.05650186773132,1.,3.17564906975371));
#57927=CARTESIAN_POINT('Ctrl Pts',(2.06166849827101,-1.,3.18197692964614));
#57928=CARTESIAN_POINT('Ctrl Pts',(2.06166849827101,1.,3.18197692964614));
#57929=CARTESIAN_POINT('Ctrl Pts',(2.06684062744112,-1.,3.18809755562368));
#57930=CARTESIAN_POINT('Ctrl Pts',(2.06684062744112,1.,3.18809755562368));
#57931=CARTESIAN_POINT('Ctrl Pts',(2.07192253497857,-1.,3.19388465568252));
#57932=CARTESIAN_POINT('Ctrl Pts',(2.07192253497857,1.,3.19388465568252));
#57933=CARTESIAN_POINT('Ctrl Pts',(2.07690441870722,-1.,3.19934132836019));
#57934=CARTESIAN_POINT('Ctrl Pts',(2.07690441870722,1.,3.19934132836019));
#57935=CARTESIAN_POINT('Ctrl Pts',(2.08182850370878,-1.,3.2045481863073));
#57936=CARTESIAN_POINT('Ctrl Pts',(2.08182850370878,1.,3.2045481863073));
#57937=CARTESIAN_POINT('Ctrl Pts',(2.08676465517455,-1.,3.20962575845463));
#57938=CARTESIAN_POINT('Ctrl Pts',(2.08676465517455,1.,3.20962575845463));
#57939=CARTESIAN_POINT('Ctrl Pts',(2.09178419460443,-1.,3.21469429601654));
#57940=CARTESIAN_POINT('Ctrl Pts',(2.09178419460443,1.,3.21469429601654));
#57941=CARTESIAN_POINT('Ctrl Pts',(2.09692958434895,-1.,3.21982707347009));
#57942=CARTESIAN_POINT('Ctrl Pts',(2.09692958434895,1.,3.21982707347009));
#57943=CARTESIAN_POINT('Ctrl Pts',(2.10220384298492,-1.,3.22503437553434));
#57944=CARTESIAN_POINT('Ctrl Pts',(2.10220384298492,1.,3.22503437553434));
#57945=CARTESIAN_POINT('Ctrl Pts',(2.10758699642451,-1.,3.23028945793289));
#57946=CARTESIAN_POINT('Ctrl Pts',(2.10758699642451,1.,3.23028945793289));
#57947=CARTESIAN_POINT('Ctrl Pts',(2.11304604021773,-1.,3.23554444767099));
#57948=CARTESIAN_POINT('Ctrl Pts',(2.11304604021773,1.,3.23554444767099));
#57949=CARTESIAN_POINT('Ctrl Pts',(2.11854673326979,-1.,3.24074905517293));
#57950=CARTESIAN_POINT('Ctrl Pts',(2.11854673326979,1.,3.24074905517293));
#57951=CARTESIAN_POINT('Ctrl Pts',(2.12406646410962,-1.,3.24587102613376));
#57952=CARTESIAN_POINT('Ctrl Pts',(2.12406646410962,1.,3.24587102613376));
#57953=CARTESIAN_POINT('Ctrl Pts',(2.12960028396832,-1.,3.25090574494028));
#57954=CARTESIAN_POINT('Ctrl Pts',(2.12960028396832,1.,3.25090574494028));
#57955=CARTESIAN_POINT('Ctrl Pts',(2.13515375878803,-1.,3.25586495065054));
#57956=CARTESIAN_POINT('Ctrl Pts',(2.13515375878803,1.,3.25586495065054));
#57957=CARTESIAN_POINT('Ctrl Pts',(2.14073870754264,-1.,3.26077002641879));
#57958=CARTESIAN_POINT('Ctrl Pts',(2.14073870754264,1.,3.26077002641879));
#57959=CARTESIAN_POINT('Ctrl Pts',(2.1463680529566,-1.,3.26564388189759));
#57960=CARTESIAN_POINT('Ctrl Pts',(2.1463680529566,1.,3.26564388189759));
#57961=CARTESIAN_POINT('Ctrl Pts',(2.15205043199808,-1.,3.27050245897228));
#57962=CARTESIAN_POINT('Ctrl Pts',(2.15205043199808,1.,3.27050245897228));
#57963=CARTESIAN_POINT('Ctrl Pts',(2.15778690038347,-1.,3.27534954469187));
#57964=CARTESIAN_POINT('Ctrl Pts',(2.15778690038347,1.,3.27534954469187));
#57965=CARTESIAN_POINT('Ctrl Pts',(2.16357391934425,-1.,3.280181508414));
#57966=CARTESIAN_POINT('Ctrl Pts',(2.16357391934425,1.,3.280181508414));
#57967=CARTESIAN_POINT('Ctrl Pts',(2.16940517773455,-1.,3.28499019979724));
#57968=CARTESIAN_POINT('Ctrl Pts',(2.16940517773455,1.,3.28499019979724));
#57969=CARTESIAN_POINT('Ctrl Pts',(2.17527380048423,-1.,3.28976645712568));
#57970=CARTESIAN_POINT('Ctrl Pts',(2.17527380048423,1.,3.28976645712568));
#57971=CARTESIAN_POINT('Ctrl Pts',(2.18117455557065,-1.,3.2945036150049));
#57972=CARTESIAN_POINT('Ctrl Pts',(2.18117455557065,1.,3.2945036150049));
#57973=CARTESIAN_POINT('Ctrl Pts',(2.18710556500327,-1.,3.29920022557639));
#57974=CARTESIAN_POINT('Ctrl Pts',(2.18710556500327,1.,3.29920022557639));
#57975=CARTESIAN_POINT('Ctrl Pts',(2.19306710376111,-1.,3.30385816281831));
#57976=CARTESIAN_POINT('Ctrl Pts',(2.19306710376111,1.,3.30385816281831));
#57977=CARTESIAN_POINT('Ctrl Pts',(2.19906078949922,-1.,3.30848134694595));
#57978=CARTESIAN_POINT('Ctrl Pts',(2.19906078949922,1.,3.30848134694595));
#57979=CARTESIAN_POINT('Ctrl Pts',(2.20508863150607,-1.,3.31307424608949));
#57980=CARTESIAN_POINT('Ctrl Pts',(2.20508863150607,1.,3.31307424608949));
#57981=CARTESIAN_POINT('Ctrl Pts',(2.21115211847875,-1.,3.31764044024235));
#57982=CARTESIAN_POINT('Ctrl Pts',(2.21115211847875,1.,3.31764044024235));
#57983=CARTESIAN_POINT('Ctrl Pts',(2.21725135110898,-1.,3.32218125618968));
#57984=CARTESIAN_POINT('Ctrl Pts',(2.21725135110898,1.,3.32218125618968));
#57985=CARTESIAN_POINT('Ctrl Pts',(2.22338548312772,-1.,3.3266964672289));
#57986=CARTESIAN_POINT('Ctrl Pts',(2.22338548312772,1.,3.3266964672289));
#57987=CARTESIAN_POINT('Ctrl Pts',(2.22955308907233,-1.,3.33118487773611));
#57988=CARTESIAN_POINT('Ctrl Pts',(2.22955308907233,1.,3.33118487773611));
#57989=CARTESIAN_POINT('Ctrl Pts',(2.23575256328812,-1.,3.33564495756482));
#57990=CARTESIAN_POINT('Ctrl Pts',(2.23575256328812,1.,3.33564495756482));
#57991=CARTESIAN_POINT('Ctrl Pts',(2.24198249391422,-1.,3.34007543738025));
#57992=CARTESIAN_POINT('Ctrl Pts',(2.24198249391422,1.,3.34007543738025));
#57993=CARTESIAN_POINT('Ctrl Pts',(2.24824207678256,-1.,3.34447596770723));
#57994=CARTESIAN_POINT('Ctrl Pts',(2.24824207678256,1.,3.34447596770723));
#57995=CARTESIAN_POINT('Ctrl Pts',(2.25453097693483,-1.,3.34884690292285));
#57996=CARTESIAN_POINT('Ctrl Pts',(2.25453097693483,1.,3.34884690292285));
#57997=CARTESIAN_POINT('Ctrl Pts',(2.26084915222449,-1.,3.35318902552626));
#57998=CARTESIAN_POINT('Ctrl Pts',(2.26084915222449,1.,3.35318902552626));
#57999=CARTESIAN_POINT('Ctrl Pts',(2.26719668579909,-1.,3.35750328523061));
#58000=CARTESIAN_POINT('Ctrl Pts',(2.26719668579909,1.,3.35750328523061));
#58001=CARTESIAN_POINT('Ctrl Pts',(2.2735736262093,-1.,3.36179055004409));
#58002=CARTESIAN_POINT('Ctrl Pts',(2.2735736262093,1.,3.36179055004409));
#58003=CARTESIAN_POINT('Ctrl Pts',(2.27997979458037,-1.,3.36605130713076));
#58004=CARTESIAN_POINT('Ctrl Pts',(2.27997979458037,1.,3.36605130713076));
#58005=CARTESIAN_POINT('Ctrl Pts',(2.28641481081137,-1.,3.37028570206488));
#58006=CARTESIAN_POINT('Ctrl Pts',(2.28641481081137,1.,3.37028570206488));
#58007=CARTESIAN_POINT('Ctrl Pts',(2.29287818007393,-1.,3.37449367172826));
#58008=CARTESIAN_POINT('Ctrl Pts',(2.29287818007393,1.,3.37449367172826));
#58009=CARTESIAN_POINT('Ctrl Pts',(2.29936936127624,-1.,3.37867504959433));
#58010=CARTESIAN_POINT('Ctrl Pts',(2.29936936127624,1.,3.37867504959433));
#58011=CARTESIAN_POINT('Ctrl Pts',(2.30588783640343,-1.,3.3828296733661));
#58012=CARTESIAN_POINT('Ctrl Pts',(2.30588783640343,1.,3.3828296733661));
#58013=CARTESIAN_POINT('Ctrl Pts',(2.31243319489367,-1.,3.38695751492462));
#58014=CARTESIAN_POINT('Ctrl Pts',(2.31243319489367,1.,3.38695751492462));
#58015=CARTESIAN_POINT('Ctrl Pts',(2.31900513925424,-1.,3.39105869474822));
#58016=CARTESIAN_POINT('Ctrl Pts',(2.31900513925424,1.,3.39105869474822));
#58017=CARTESIAN_POINT('Ctrl Pts',(2.3256034390248,-1.,3.39513342019756));
#58018=CARTESIAN_POINT('Ctrl Pts',(2.3256034390248,1.,3.39513342019756));
#58019=CARTESIAN_POINT('Ctrl Pts',(2.33222789882489,-1.,3.39918194577956));
#58020=CARTESIAN_POINT('Ctrl Pts',(2.33222789882489,1.,3.39918194577956));
#58021=CARTESIAN_POINT('Ctrl Pts',(2.33887832342782,-1.,3.40320452776743));
#58022=CARTESIAN_POINT('Ctrl Pts',(2.33887832342782,1.,3.40320452776743));
#58023=CARTESIAN_POINT('Ctrl Pts',(2.34555447649188,-1.,3.40720137404297));
#58024=CARTESIAN_POINT('Ctrl Pts',(2.34555447649188,1.,3.40720137404297));
#58025=CARTESIAN_POINT('Ctrl Pts',(2.35225606824109,-1.,3.41117262314119));
#58026=CARTESIAN_POINT('Ctrl Pts',(2.35225606824109,1.,3.41117262314119));
#58027=CARTESIAN_POINT('Ctrl Pts',(2.35898278606946,-1.,3.41511836751469));
#58028=CARTESIAN_POINT('Ctrl Pts',(2.35898278606946,1.,3.41511836751469));
#58029=CARTESIAN_POINT('Ctrl Pts',(2.36573431470642,-1.,3.41903866635852));
#58030=CARTESIAN_POINT('Ctrl Pts',(2.36573431470642,1.,3.41903866635852));
#58031=CARTESIAN_POINT('Ctrl Pts',(2.37251035954292,-1.,3.42293356216511));
#58032=CARTESIAN_POINT('Ctrl Pts',(2.37251035954292,1.,3.42293356216511));
#58033=CARTESIAN_POINT('Ctrl Pts',(2.37931067028926,-1.,3.42680309754399));
#58034=CARTESIAN_POINT('Ctrl Pts',(2.37931067028926,1.,3.42680309754399));
#58035=CARTESIAN_POINT('Ctrl Pts',(2.38613505843552,-1.,3.4306473271292));
#58036=CARTESIAN_POINT('Ctrl Pts',(2.38613505843552,1.,3.4306473271292));
#58037=CARTESIAN_POINT('Ctrl Pts',(2.39298338804493,-1.,3.4344663067854));
#58038=CARTESIAN_POINT('Ctrl Pts',(2.39298338804493,1.,3.4344663067854));
#58039=CARTESIAN_POINT('Ctrl Pts',(2.39848113410292,-1.,3.43750133064416));
#58040=CARTESIAN_POINT('Ctrl Pts',(2.39848113410292,1.,3.43750133064416));
#58041=CARTESIAN_POINT('Ctrl Pts',(2.40261515589405,-1.,3.43976627484234));
#58042=CARTESIAN_POINT('Ctrl Pts',(2.40261515589405,1.,3.43976627484234));
#58043=CARTESIAN_POINT('Ctrl Pts',(2.4053759295909,-1.,3.44127120683039));
#58044=CARTESIAN_POINT('Ctrl Pts',(2.4053759295909,1.,3.44127120683039));
#58045=CARTESIAN_POINT('Ctrl Pts',(2.40675750623143,-1.,3.44202241512147));
#58046=CARTESIAN_POINT('Ctrl Pts',(2.40675750623143,1.,3.44202241512147));
#58047=CARTESIAN_POINT('',(2.03660101169714,1.,3.14877060440328));
#58048=CARTESIAN_POINT('Ctrl Pts',(2.03660101169714,-1.,3.14877060440327));
#58049=CARTESIAN_POINT('Ctrl Pts',(2.03660101169714,-0.666666666666667,
3.14877060440327));
#58050=CARTESIAN_POINT('Ctrl Pts',(2.03660101169714,-0.333333333333333,
3.14877060440327));
#58051=CARTESIAN_POINT('Ctrl Pts',(2.03660101169714,0.333333333333333,3.14877060440327));
#58052=CARTESIAN_POINT('Ctrl Pts',(2.03660101169714,0.666666666666667,3.14877060440327));
#58053=CARTESIAN_POINT('Ctrl Pts',(2.03660101169714,1.,3.14877060440327));
#58054=CARTESIAN_POINT('',(2.40675750623143,1.,3.44202241512147));
#58055=CARTESIAN_POINT('',(2.40675750623143,0.,3.44202241512147));
#58056=CARTESIAN_POINT('Ctrl Pts',(2.03660101169714,1.,3.14877060440328));
#58057=CARTESIAN_POINT('Ctrl Pts',(2.03659701539259,1.,3.14881939088124));
#58058=CARTESIAN_POINT('Ctrl Pts',(2.03663974554932,1.,3.1490119366901));
#58059=CARTESIAN_POINT('Ctrl Pts',(2.03693188810545,1.,3.14959882629805));
#58060=CARTESIAN_POINT('Ctrl Pts',(2.03783225495961,1.,3.15102344775328));
#58061=CARTESIAN_POINT('Ctrl Pts',(2.03984073791519,1.,3.15389991674792));
#58062=CARTESIAN_POINT('Ctrl Pts',(2.04297406404027,1.,3.15817983946367));
#58063=CARTESIAN_POINT('Ctrl Pts',(2.04693331247446,1.,3.16343165058912));
#58064=CARTESIAN_POINT('Ctrl Pts',(2.05151770247233,1.,3.16936341689527));
#58065=CARTESIAN_POINT('Ctrl Pts',(2.05650186773132,1.,3.17564906975371));
#58066=CARTESIAN_POINT('Ctrl Pts',(2.06166849827101,1.,3.18197692964614));
#58067=CARTESIAN_POINT('Ctrl Pts',(2.06684062744112,1.,3.18809755562368));
#58068=CARTESIAN_POINT('Ctrl Pts',(2.07192253497857,1.,3.19388465568252));
#58069=CARTESIAN_POINT('Ctrl Pts',(2.07690441870722,1.,3.19934132836019));
#58070=CARTESIAN_POINT('Ctrl Pts',(2.08182850370878,1.,3.2045481863073));
#58071=CARTESIAN_POINT('Ctrl Pts',(2.08676465517455,1.,3.20962575845463));
#58072=CARTESIAN_POINT('Ctrl Pts',(2.09178419460443,1.,3.21469429601654));
#58073=CARTESIAN_POINT('Ctrl Pts',(2.09692958434895,1.,3.21982707347009));
#58074=CARTESIAN_POINT('Ctrl Pts',(2.10220384298492,1.,3.22503437553434));
#58075=CARTESIAN_POINT('Ctrl Pts',(2.10758699642451,1.,3.23028945793289));
#58076=CARTESIAN_POINT('Ctrl Pts',(2.11304604021773,1.,3.23554444767099));
#58077=CARTESIAN_POINT('Ctrl Pts',(2.11854673326979,1.,3.24074905517293));
#58078=CARTESIAN_POINT('Ctrl Pts',(2.12406646410962,1.,3.24587102613376));
#58079=CARTESIAN_POINT('Ctrl Pts',(2.12960028396832,1.,3.25090574494028));
#58080=CARTESIAN_POINT('Ctrl Pts',(2.13515375878803,1.,3.25586495065054));
#58081=CARTESIAN_POINT('Ctrl Pts',(2.14073870754264,1.,3.26077002641879));
#58082=CARTESIAN_POINT('Ctrl Pts',(2.1463680529566,1.,3.26564388189759));
#58083=CARTESIAN_POINT('Ctrl Pts',(2.15205043199808,1.,3.27050245897228));
#58084=CARTESIAN_POINT('Ctrl Pts',(2.15778690038347,1.,3.27534954469187));
#58085=CARTESIAN_POINT('Ctrl Pts',(2.16357391934425,1.,3.280181508414));
#58086=CARTESIAN_POINT('Ctrl Pts',(2.16940517773455,1.,3.28499019979724));
#58087=CARTESIAN_POINT('Ctrl Pts',(2.17527380048423,1.,3.28976645712568));
#58088=CARTESIAN_POINT('Ctrl Pts',(2.18117455557065,1.,3.2945036150049));
#58089=CARTESIAN_POINT('Ctrl Pts',(2.18710556500327,1.,3.29920022557639));
#58090=CARTESIAN_POINT('Ctrl Pts',(2.19306710376111,1.,3.30385816281831));
#58091=CARTESIAN_POINT('Ctrl Pts',(2.19906078949922,1.,3.30848134694595));
#58092=CARTESIAN_POINT('Ctrl Pts',(2.20508863150607,1.,3.31307424608949));
#58093=CARTESIAN_POINT('Ctrl Pts',(2.21115211847875,1.,3.31764044024235));
#58094=CARTESIAN_POINT('Ctrl Pts',(2.21725135110898,1.,3.32218125618968));
#58095=CARTESIAN_POINT('Ctrl Pts',(2.22338548312772,1.,3.3266964672289));
#58096=CARTESIAN_POINT('Ctrl Pts',(2.22955308907233,1.,3.33118487773611));
#58097=CARTESIAN_POINT('Ctrl Pts',(2.23575256328812,1.,3.33564495756482));
#58098=CARTESIAN_POINT('Ctrl Pts',(2.24198249391422,1.,3.34007543738025));
#58099=CARTESIAN_POINT('Ctrl Pts',(2.24824207678256,1.,3.34447596770723));
#58100=CARTESIAN_POINT('Ctrl Pts',(2.25453097693483,1.,3.34884690292285));
#58101=CARTESIAN_POINT('Ctrl Pts',(2.26084915222449,1.,3.35318902552626));
#58102=CARTESIAN_POINT('Ctrl Pts',(2.26719668579909,1.,3.35750328523061));
#58103=CARTESIAN_POINT('Ctrl Pts',(2.2735736262093,1.,3.36179055004409));
#58104=CARTESIAN_POINT('Ctrl Pts',(2.27997979458037,1.,3.36605130713076));
#58105=CARTESIAN_POINT('Ctrl Pts',(2.28641481081137,1.,3.37028570206488));
#58106=CARTESIAN_POINT('Ctrl Pts',(2.29287818007393,1.,3.37449367172826));
#58107=CARTESIAN_POINT('Ctrl Pts',(2.29936936127624,1.,3.37867504959433));
#58108=CARTESIAN_POINT('Ctrl Pts',(2.30588783640343,1.,3.3828296733661));
#58109=CARTESIAN_POINT('Ctrl Pts',(2.31243319489367,1.,3.38695751492462));
#58110=CARTESIAN_POINT('Ctrl Pts',(2.31900513925424,1.,3.39105869474822));
#58111=CARTESIAN_POINT('Ctrl Pts',(2.3256034390248,1.,3.39513342019756));
#58112=CARTESIAN_POINT('Ctrl Pts',(2.33222789882489,1.,3.39918194577956));
#58113=CARTESIAN_POINT('Ctrl Pts',(2.33887832342782,1.,3.40320452776743));
#58114=CARTESIAN_POINT('Ctrl Pts',(2.34555447649188,1.,3.40720137404297));
#58115=CARTESIAN_POINT('Ctrl Pts',(2.35225606824109,1.,3.41117262314119));
#58116=CARTESIAN_POINT('Ctrl Pts',(2.35898278606946,1.,3.41511836751469));
#58117=CARTESIAN_POINT('Ctrl Pts',(2.36573431470642,1.,3.41903866635852));
#58118=CARTESIAN_POINT('Ctrl Pts',(2.37251035954292,1.,3.42293356216511));
#58119=CARTESIAN_POINT('Ctrl Pts',(2.37931067028926,1.,3.42680309754399));
#58120=CARTESIAN_POINT('Ctrl Pts',(2.38613505843552,1.,3.4306473271292));
#58121=CARTESIAN_POINT('Ctrl Pts',(2.39298338804493,1.,3.4344663067854));
#58122=CARTESIAN_POINT('Ctrl Pts',(2.39848113410292,1.,3.43750133064416));
#58123=CARTESIAN_POINT('Ctrl Pts',(2.40261515589405,1.,3.43976627484234));
#58124=CARTESIAN_POINT('Ctrl Pts',(2.4053759295909,1.,3.44127120683039));
#58125=CARTESIAN_POINT('Ctrl Pts',(2.40675750623143,1.,3.44202241512147));
#58126=CARTESIAN_POINT('Origin',(2.40675750623143,0.,3.44202241512147));
#58127=CARTESIAN_POINT('',(2.52982887637028,1.,3.35260583073571));
#58128=CARTESIAN_POINT('Origin',(0.,0.,0.));
#58129=CARTESIAN_POINT('',(1.88097764062697,1.,3.24413672884812));
#58130=CARTESIAN_POINT('Origin',(0.,1.,0.));
#58131=CARTESIAN_POINT('Ctrl Pts',(1.88097764062697,1.,3.24413672884812));
#58132=CARTESIAN_POINT('Ctrl Pts',(1.88097764062697,0.666666666666667,3.24413672884812));
#58133=CARTESIAN_POINT('Ctrl Pts',(1.88097764062697,0.333333333333333,3.24413672884812));
#58134=CARTESIAN_POINT('Ctrl Pts',(1.88097764062697,-0.333333333333333,
3.24413672884812));
#58135=CARTESIAN_POINT('Ctrl Pts',(1.88097764062697,-0.666666666666667,
3.24413672884812));
#58136=CARTESIAN_POINT('Ctrl Pts',(1.88097764062697,-1.,3.24413672884812));
#58137=CARTESIAN_POINT('Ctrl Pts',(1.97421938526992,-1.,3.70708211654725));
#58138=CARTESIAN_POINT('Ctrl Pts',(1.97421938526992,1.,3.70708211654725));
#58139=CARTESIAN_POINT('Ctrl Pts',(1.97417727645308,-1.,3.70551008132332));
#58140=CARTESIAN_POINT('Ctrl Pts',(1.97417727645308,1.,3.70551008132332));
#58141=CARTESIAN_POINT('Ctrl Pts',(1.97408973726715,-1.,3.70236698912904));
#58142=CARTESIAN_POINT('Ctrl Pts',(1.97408973726715,1.,3.70236698912904));
#58143=CARTESIAN_POINT('Ctrl Pts',(1.97394846383216,-1.,3.6976552856004));
#58144=CARTESIAN_POINT('Ctrl Pts',(1.97394846383216,1.,3.6976552856004));
#58145=CARTESIAN_POINT('Ctrl Pts',(1.97374016225483,-1.,3.69137888599902));
#58146=CARTESIAN_POINT('Ctrl Pts',(1.97374016225483,1.,3.69137888599902));
#58147=CARTESIAN_POINT('Ctrl Pts',(1.97344650304519,-1.,3.68354319915092));
#58148=CARTESIAN_POINT('Ctrl Pts',(1.97344650304519,1.,3.68354319915092));
#58149=CARTESIAN_POINT('Ctrl Pts',(1.97311947678516,-1.,3.67571738107084));
#58150=CARTESIAN_POINT('Ctrl Pts',(1.97311947678516,1.,3.67571738107084));
#58151=CARTESIAN_POINT('Ctrl Pts',(1.97275897198678,-1.,3.66790152752075));
#58152=CARTESIAN_POINT('Ctrl Pts',(1.97275897198678,1.,3.66790152752075));
#58153=CARTESIAN_POINT('Ctrl Pts',(1.9723648543905,-1.,3.6600957816636));
#58154=CARTESIAN_POINT('Ctrl Pts',(1.9723648543905,1.,3.6600957816636));
#58155=CARTESIAN_POINT('Ctrl Pts',(1.97193697240239,-1.,3.652300347166));
#58156=CARTESIAN_POINT('Ctrl Pts',(1.97193697240239,1.,3.652300347166));
#58157=CARTESIAN_POINT('Ctrl Pts',(1.97147515441164,-1.,3.64451546723514));
#58158=CARTESIAN_POINT('Ctrl Pts',(1.97147515441164,1.,3.64451546723514));
#58159=CARTESIAN_POINT('Ctrl Pts',(1.97097920454464,-1.,3.63674139590412));
#58160=CARTESIAN_POINT('Ctrl Pts',(1.97097920454464,1.,3.63674139590412));
#58161=CARTESIAN_POINT('Ctrl Pts',(1.97044889850463,-1.,3.62897836973293));
#58162=CARTESIAN_POINT('Ctrl Pts',(1.97044889850463,1.,3.62897836973293));
#58163=CARTESIAN_POINT('Ctrl Pts',(1.96988398129978,-1.,3.62122658401893));
#58164=CARTESIAN_POINT('Ctrl Pts',(1.96988398129978,1.,3.62122658401893));
#58165=CARTESIAN_POINT('Ctrl Pts',(1.96928416040877,-1.,3.61348615496704));
#58166=CARTESIAN_POINT('Ctrl Pts',(1.96928416040877,1.,3.61348615496704));
#58167=CARTESIAN_POINT('Ctrl Pts',(1.9686491188594,-1.,3.60575714017989));
#58168=CARTESIAN_POINT('Ctrl Pts',(1.9686491188594,1.,3.60575714017989));
#58169=CARTESIAN_POINT('Ctrl Pts',(1.96797854118369,-1.,3.59803959819938));
#58170=CARTESIAN_POINT('Ctrl Pts',(1.96797854118369,1.,3.59803959819938));
#58171=CARTESIAN_POINT('Ctrl Pts',(1.96727213799544,-1.,3.59033364022801));
#58172=CARTESIAN_POINT('Ctrl Pts',(1.96727213799544,1.,3.59033364022801));
#58173=CARTESIAN_POINT('Ctrl Pts',(1.96652966688911,-1.,3.58263947663829));
#58174=CARTESIAN_POINT('Ctrl Pts',(1.96652966688911,1.,3.58263947663829));
#58175=CARTESIAN_POINT('Ctrl Pts',(1.96575096652789,-1.,3.57495748600959));
#58176=CARTESIAN_POINT('Ctrl Pts',(1.96575096652789,1.,3.57495748600959));
#58177=CARTESIAN_POINT('Ctrl Pts',(1.96493594634567,-1.,3.56728820357791));
#58178=CARTESIAN_POINT('Ctrl Pts',(1.96493594634567,1.,3.56728820357791));
#58179=CARTESIAN_POINT('Ctrl Pts',(1.96408450906812,-1.,3.55963218706096));
#58180=CARTESIAN_POINT('Ctrl Pts',(1.96408450906812,1.,3.55963218706096));
#58181=CARTESIAN_POINT('Ctrl Pts',(1.96319648628644,-1.,3.55198990600886));
#58182=CARTESIAN_POINT('Ctrl Pts',(1.96319648628644,1.,3.55198990600886));
#58183=CARTESIAN_POINT('Ctrl Pts',(1.96227157573067,-1.,3.54436163300443));
#58184=CARTESIAN_POINT('Ctrl Pts',(1.96227157573067,1.,3.54436163300443));
#58185=CARTESIAN_POINT('Ctrl Pts',(1.96130926212689,-1.,3.53674730625813));
#58186=CARTESIAN_POINT('Ctrl Pts',(1.96130926212689,1.,3.53674730625813));
#58187=CARTESIAN_POINT('Ctrl Pts',(1.96030879411566,-1.,3.52914648844351));
#58188=CARTESIAN_POINT('Ctrl Pts',(1.96030879411566,1.,3.52914648844351));
#58189=CARTESIAN_POINT('Ctrl Pts',(1.95926936324461,-1.,3.52155867431486));
#58190=CARTESIAN_POINT('Ctrl Pts',(1.95926936324461,1.,3.52155867431486));
#58191=CARTESIAN_POINT('Ctrl Pts',(1.95819025316779,-1.,3.51398354617794));
#58192=CARTESIAN_POINT('Ctrl Pts',(1.95819025316779,1.,3.51398354617794));
#58193=CARTESIAN_POINT('Ctrl Pts',(1.95707099606511,-1.,3.50642124159909));
#58194=CARTESIAN_POINT('Ctrl Pts',(1.95707099606511,1.,3.50642124159909));
#58195=CARTESIAN_POINT('Ctrl Pts',(1.95591153823661,-1.,3.49887263575583));
#58196=CARTESIAN_POINT('Ctrl Pts',(1.95591153823661,1.,3.49887263575583));
#58197=CARTESIAN_POINT('Ctrl Pts',(1.95471236969643,-1.,3.49133956289133));
#58198=CARTESIAN_POINT('Ctrl Pts',(1.95471236969643,1.,3.49133956289133));
#58199=CARTESIAN_POINT('Ctrl Pts',(1.95347412486308,-1.,3.48382414832634));
#58200=CARTESIAN_POINT('Ctrl Pts',(1.95347412486308,1.,3.48382414832634));
#58201=CARTESIAN_POINT('Ctrl Pts',(1.95219722189876,-1.,3.47632820495921));
#58202=CARTESIAN_POINT('Ctrl Pts',(1.95219722189876,1.,3.47632820495921));
#58203=CARTESIAN_POINT('Ctrl Pts',(1.95088147859876,-1.,3.46885258974191));
#58204=CARTESIAN_POINT('Ctrl Pts',(1.95088147859876,1.,3.46885258974191));
#58205=CARTESIAN_POINT('Ctrl Pts',(1.94952575850197,-1.,3.46139661060962));
#58206=CARTESIAN_POINT('Ctrl Pts',(1.94952575850197,1.,3.46139661060962));
#58207=CARTESIAN_POINT('Ctrl Pts',(1.94812754766524,-1.,3.45395731584051));
#58208=CARTESIAN_POINT('Ctrl Pts',(1.94812754766524,1.,3.45395731584051));
#58209=CARTESIAN_POINT('Ctrl Pts',(1.94668377715329,-1.,3.44653088665681));
#58210=CARTESIAN_POINT('Ctrl Pts',(1.94668377715329,1.,3.44653088665681));
#58211=CARTESIAN_POINT('Ctrl Pts',(1.94519168842879,-1.,3.43911410197687));
#58212=CARTESIAN_POINT('Ctrl Pts',(1.94519168842879,1.,3.43911410197687));
#58213=CARTESIAN_POINT('Ctrl Pts',(1.94364973660284,-1.,3.43170586602434));
#58214=CARTESIAN_POINT('Ctrl Pts',(1.94364973660284,1.,3.43170586602434));
#58215=CARTESIAN_POINT('Ctrl Pts',(1.94205835913696,-1.,3.42430850941503));
#58216=CARTESIAN_POINT('Ctrl Pts',(1.94205835913696,1.,3.42430850941503));
#58217=CARTESIAN_POINT('Ctrl Pts',(1.94042111965246,-1.,3.41692971994096));
#58218=CARTESIAN_POINT('Ctrl Pts',(1.94042111965246,1.,3.41692971994096));
#58219=CARTESIAN_POINT('Ctrl Pts',(1.93874306008143,-1.,3.40957978266642));
#58220=CARTESIAN_POINT('Ctrl Pts',(1.93874306008143,1.,3.40957978266642));
#58221=CARTESIAN_POINT('Ctrl Pts',(1.93702857723098,-1.,3.40226802104109));
#58222=CARTESIAN_POINT('Ctrl Pts',(1.93702857723098,1.,3.40226802104109));
#58223=CARTESIAN_POINT('Ctrl Pts',(1.93527929945985,-1.,3.39499923640795));
#58224=CARTESIAN_POINT('Ctrl Pts',(1.93527929945985,1.,3.39499923640795));
#58225=CARTESIAN_POINT('Ctrl Pts',(1.93349233176788,-1.,3.38777076883256));
#58226=CARTESIAN_POINT('Ctrl Pts',(1.93349233176788,1.,3.38777076883256));
#58227=CARTESIAN_POINT('Ctrl Pts',(1.93165739093276,-1.,3.3805676852555));
#58228=CARTESIAN_POINT('Ctrl Pts',(1.93165739093276,1.,3.3805676852555));
#58229=CARTESIAN_POINT('Ctrl Pts',(1.92975993109877,-1.,3.37336807068043));
#58230=CARTESIAN_POINT('Ctrl Pts',(1.92975993109877,1.,3.37336807068043));
#58231=CARTESIAN_POINT('Ctrl Pts',(1.92778626543786,-1.,3.36615168657567));
#58232=CARTESIAN_POINT('Ctrl Pts',(1.92778626543786,1.,3.36615168657567));
#58233=CARTESIAN_POINT('Ctrl Pts',(1.92572846125756,-1.,3.35890824422965));
#58234=CARTESIAN_POINT('Ctrl Pts',(1.92572846125756,1.,3.35890824422965));
#58235=CARTESIAN_POINT('Ctrl Pts',(1.92358838440528,-1.,3.35164424847223));
#58236=CARTESIAN_POINT('Ctrl Pts',(1.92358838440528,1.,3.35164424847223));
#58237=CARTESIAN_POINT('Ctrl Pts',(1.92138450828404,-1.,3.34439448941961));
#58238=CARTESIAN_POINT('Ctrl Pts',(1.92138450828404,1.,3.34439448941961));
#58239=CARTESIAN_POINT('Ctrl Pts',(1.9191460961021,-1.,3.33721230710012));
#58240=CARTESIAN_POINT('Ctrl Pts',(1.9191460961021,1.,3.33721230710012));
#58241=CARTESIAN_POINT('Ctrl Pts',(1.91690081930331,-1.,3.33014884257873));
#58242=CARTESIAN_POINT('Ctrl Pts',(1.91690081930331,1.,3.33014884257873));
#58243=CARTESIAN_POINT('Ctrl Pts',(1.91466343916627,-1.,3.32323403454535));
#58244=CARTESIAN_POINT('Ctrl Pts',(1.91466343916627,1.,3.32323403454535));
#58245=CARTESIAN_POINT('Ctrl Pts',(1.91242616234442,-1.,3.31646052426364));
#58246=CARTESIAN_POINT('Ctrl Pts',(1.91242616234442,1.,3.31646052426364));
#58247=CARTESIAN_POINT('Ctrl Pts',(1.91014297830446,-1.,3.30975721158596));
#58248=CARTESIAN_POINT('Ctrl Pts',(1.91014297830446,1.,3.30975721158596));
#58249=CARTESIAN_POINT('Ctrl Pts',(1.90773912171341,-1.,3.30300595568195));
#58250=CARTESIAN_POINT('Ctrl Pts',(1.90773912171341,1.,3.30300595568195));
#58251=CARTESIAN_POINT('Ctrl Pts',(1.90513891864087,-1.,3.29608978722113));
#58252=CARTESIAN_POINT('Ctrl Pts',(1.90513891864087,1.,3.29608978722113));
#58253=CARTESIAN_POINT('Ctrl Pts',(1.90228971247527,-1.,3.2889344860029));
#58254=CARTESIAN_POINT('Ctrl Pts',(1.90228971247527,1.,3.2889344860029));
#58255=CARTESIAN_POINT('Ctrl Pts',(1.89918429230462,-1.,3.28154737912352));
#58256=CARTESIAN_POINT('Ctrl Pts',(1.89918429230462,1.,3.28154737912352));
#58257=CARTESIAN_POINT('Ctrl Pts',(1.89589172903793,-1.,3.27407108933139));
#58258=CARTESIAN_POINT('Ctrl Pts',(1.89589172903793,1.,3.27407108933139));
#58259=CARTESIAN_POINT('Ctrl Pts',(1.89255393500965,-1.,3.26677653888676));
#58260=CARTESIAN_POINT('Ctrl Pts',(1.89255393500965,1.,3.26677653888676));
#58261=CARTESIAN_POINT('Ctrl Pts',(1.88934996203698,-1.,3.25999885193947));
#58262=CARTESIAN_POINT('Ctrl Pts',(1.88934996203698,1.,3.25999885193947));
#58263=CARTESIAN_POINT('Ctrl Pts',(1.88646802523466,-1.,3.25408686339463));
#58264=CARTESIAN_POINT('Ctrl Pts',(1.88646802523466,1.,3.25408686339463));
#58265=CARTESIAN_POINT('Ctrl Pts',(1.88407708646357,-1.,3.24935200511918));
#58266=CARTESIAN_POINT('Ctrl Pts',(1.88407708646357,1.,3.24935200511918));
#58267=CARTESIAN_POINT('Ctrl Pts',(1.88229202582941,-1.,3.24600543790443));
#58268=CARTESIAN_POINT('Ctrl Pts',(1.88229202582941,1.,3.24600543790443));
#58269=CARTESIAN_POINT('Ctrl Pts',(1.88139187908074,-1.,3.24451807186481));
#58270=CARTESIAN_POINT('Ctrl Pts',(1.88139187908074,1.,3.24451807186481));
#58271=CARTESIAN_POINT('Ctrl Pts',(1.88102201872555,-1.,3.24408699284121));
#58272=CARTESIAN_POINT('Ctrl Pts',(1.88102201872555,1.,3.24408699284121));
#58273=CARTESIAN_POINT('Ctrl Pts',(1.88091100680349,-1.,3.24410359189609));
#58274=CARTESIAN_POINT('Ctrl Pts',(1.88091100680349,1.,3.24410359189609));
#58275=CARTESIAN_POINT('Ctrl Pts',(1.8808893942881,-1.,3.24418789321065));
#58276=CARTESIAN_POINT('Ctrl Pts',(1.8808893942881,1.,3.24418789321065));
#58277=CARTESIAN_POINT('',(1.97421938526992,1.,3.70708211654725));
#58278=CARTESIAN_POINT('Ctrl Pts',(1.97421938526992,1.,3.70708211654725));
#58279=CARTESIAN_POINT('Ctrl Pts',(1.97417727645308,1.,3.70551008132332));
#58280=CARTESIAN_POINT('Ctrl Pts',(1.97408973726715,1.,3.70236698912904));
#58281=CARTESIAN_POINT('Ctrl Pts',(1.97394846383216,1.,3.6976552856004));
#58282=CARTESIAN_POINT('Ctrl Pts',(1.97374016225483,1.,3.69137888599902));
#58283=CARTESIAN_POINT('Ctrl Pts',(1.97344650304519,1.,3.68354319915092));
#58284=CARTESIAN_POINT('Ctrl Pts',(1.97311947678516,1.,3.67571738107084));
#58285=CARTESIAN_POINT('Ctrl Pts',(1.97275897198678,1.,3.66790152752075));
#58286=CARTESIAN_POINT('Ctrl Pts',(1.9723648543905,1.,3.6600957816636));
#58287=CARTESIAN_POINT('Ctrl Pts',(1.97193697240239,1.,3.652300347166));
#58288=CARTESIAN_POINT('Ctrl Pts',(1.97147515441164,1.,3.64451546723514));
#58289=CARTESIAN_POINT('Ctrl Pts',(1.97097920454464,1.,3.63674139590412));
#58290=CARTESIAN_POINT('Ctrl Pts',(1.97044889850463,1.,3.62897836973293));
#58291=CARTESIAN_POINT('Ctrl Pts',(1.96988398129978,1.,3.62122658401893));
#58292=CARTESIAN_POINT('Ctrl Pts',(1.96928416040877,1.,3.61348615496704));
#58293=CARTESIAN_POINT('Ctrl Pts',(1.9686491188594,1.,3.60575714017989));
#58294=CARTESIAN_POINT('Ctrl Pts',(1.96797854118369,1.,3.59803959819938));
#58295=CARTESIAN_POINT('Ctrl Pts',(1.96727213799544,1.,3.59033364022801));
#58296=CARTESIAN_POINT('Ctrl Pts',(1.96652966688911,1.,3.58263947663829));
#58297=CARTESIAN_POINT('Ctrl Pts',(1.96575096652789,1.,3.57495748600959));
#58298=CARTESIAN_POINT('Ctrl Pts',(1.96493594634567,1.,3.56728820357791));
#58299=CARTESIAN_POINT('Ctrl Pts',(1.96408450906812,1.,3.55963218706096));
#58300=CARTESIAN_POINT('Ctrl Pts',(1.96319648628644,1.,3.55198990600886));
#58301=CARTESIAN_POINT('Ctrl Pts',(1.96227157573067,1.,3.54436163300443));
#58302=CARTESIAN_POINT('Ctrl Pts',(1.96130926212689,1.,3.53674730625813));
#58303=CARTESIAN_POINT('Ctrl Pts',(1.96030879411566,1.,3.52914648844351));
#58304=CARTESIAN_POINT('Ctrl Pts',(1.95926936324461,1.,3.52155867431486));
#58305=CARTESIAN_POINT('Ctrl Pts',(1.95819025316779,1.,3.51398354617794));
#58306=CARTESIAN_POINT('Ctrl Pts',(1.95707099606511,1.,3.50642124159909));
#58307=CARTESIAN_POINT('Ctrl Pts',(1.95591153823661,1.,3.49887263575583));
#58308=CARTESIAN_POINT('Ctrl Pts',(1.95471236969643,1.,3.49133956289133));
#58309=CARTESIAN_POINT('Ctrl Pts',(1.95347412486308,1.,3.48382414832634));
#58310=CARTESIAN_POINT('Ctrl Pts',(1.95219722189876,1.,3.47632820495921));
#58311=CARTESIAN_POINT('Ctrl Pts',(1.95088147859876,1.,3.46885258974191));
#58312=CARTESIAN_POINT('Ctrl Pts',(1.94952575850197,1.,3.46139661060962));
#58313=CARTESIAN_POINT('Ctrl Pts',(1.94812754766524,1.,3.45395731584051));
#58314=CARTESIAN_POINT('Ctrl Pts',(1.94668377715329,1.,3.44653088665681));
#58315=CARTESIAN_POINT('Ctrl Pts',(1.94519168842879,1.,3.43911410197687));
#58316=CARTESIAN_POINT('Ctrl Pts',(1.94364973660284,1.,3.43170586602434));
#58317=CARTESIAN_POINT('Ctrl Pts',(1.94205835913696,1.,3.42430850941503));
#58318=CARTESIAN_POINT('Ctrl Pts',(1.94042111965246,1.,3.41692971994096));
#58319=CARTESIAN_POINT('Ctrl Pts',(1.93874306008143,1.,3.40957978266642));
#58320=CARTESIAN_POINT('Ctrl Pts',(1.93702857723098,1.,3.40226802104109));
#58321=CARTESIAN_POINT('Ctrl Pts',(1.93527929945985,1.,3.39499923640795));
#58322=CARTESIAN_POINT('Ctrl Pts',(1.93349233176788,1.,3.38777076883256));
#58323=CARTESIAN_POINT('Ctrl Pts',(1.93165739093276,1.,3.3805676852555));
#58324=CARTESIAN_POINT('Ctrl Pts',(1.92975993109877,1.,3.37336807068043));
#58325=CARTESIAN_POINT('Ctrl Pts',(1.92778626543786,1.,3.36615168657567));
#58326=CARTESIAN_POINT('Ctrl Pts',(1.92572846125756,1.,3.35890824422965));
#58327=CARTESIAN_POINT('Ctrl Pts',(1.92358838440528,1.,3.35164424847223));
#58328=CARTESIAN_POINT('Ctrl Pts',(1.92138450828404,1.,3.34439448941961));
#58329=CARTESIAN_POINT('Ctrl Pts',(1.9191460961021,1.,3.33721230710012));
#58330=CARTESIAN_POINT('Ctrl Pts',(1.91690081930331,1.,3.33014884257873));
#58331=CARTESIAN_POINT('Ctrl Pts',(1.91466343916627,1.,3.32323403454535));
#58332=CARTESIAN_POINT('Ctrl Pts',(1.91242616234442,1.,3.31646052426364));
#58333=CARTESIAN_POINT('Ctrl Pts',(1.91014297830446,1.,3.30975721158596));
#58334=CARTESIAN_POINT('Ctrl Pts',(1.90773912171341,1.,3.30300595568195));
#58335=CARTESIAN_POINT('Ctrl Pts',(1.90513891864087,1.,3.29608978722113));
#58336=CARTESIAN_POINT('Ctrl Pts',(1.90228971247527,1.,3.2889344860029));
#58337=CARTESIAN_POINT('Ctrl Pts',(1.89918429230462,1.,3.28154737912352));
#58338=CARTESIAN_POINT('Ctrl Pts',(1.89589172903793,1.,3.27407108933139));
#58339=CARTESIAN_POINT('Ctrl Pts',(1.89255393500965,1.,3.26677653888676));
#58340=CARTESIAN_POINT('Ctrl Pts',(1.88934996203698,1.,3.25999885193947));
#58341=CARTESIAN_POINT('Ctrl Pts',(1.88646802523466,1.,3.25408686339463));
#58342=CARTESIAN_POINT('Ctrl Pts',(1.88407708646357,1.,3.24935200511918));
#58343=CARTESIAN_POINT('Ctrl Pts',(1.88242596600454,1.,3.2462565441079));
#58344=CARTESIAN_POINT('Ctrl Pts',(1.88156537699203,1.,3.24480754676064));
#58345=CARTESIAN_POINT('Ctrl Pts',(1.88117508446775,1.,3.24428080353022));
#58346=CARTESIAN_POINT('Ctrl Pts',(1.8810229239812,1.,3.24415531671284));
#58347=CARTESIAN_POINT('Ctrl Pts',(1.88097764062697,1.,3.24413672884812));
#58348=CARTESIAN_POINT('',(1.97421938526992,0.,3.70708211654725));
#58349=CARTESIAN_POINT('Ctrl Pts',(1.519044091397,-1.,3.42855728381368));
#58350=CARTESIAN_POINT('Ctrl Pts',(1.519044091397,1.,3.42855728381368));
#58351=CARTESIAN_POINT('Ctrl Pts',(1.51896318668366,-1.,3.42852521763778));
#58352=CARTESIAN_POINT('Ctrl Pts',(1.51896318668366,1.,3.42852521763778));
#58353=CARTESIAN_POINT('Ctrl Pts',(1.51888450659652,-1.,3.42860527149177));
#58354=CARTESIAN_POINT('Ctrl Pts',(1.51888450659652,1.,3.42860527149177));
#58355=CARTESIAN_POINT('Ctrl Pts',(1.51901585839109,-1.,3.42915787669893));
#58356=CARTESIAN_POINT('Ctrl Pts',(1.51901585839109,1.,3.42915787669893));
#58357=CARTESIAN_POINT('Ctrl Pts',(1.51969006980999,-1.,3.43076036253837));
#58358=CARTESIAN_POINT('Ctrl Pts',(1.51969006980999,1.,3.43076036253837));
#58359=CARTESIAN_POINT('Ctrl Pts',(1.52134826724292,-1.,3.43417156977893));
#58360=CARTESIAN_POINT('Ctrl Pts',(1.52134826724292,1.,3.43417156977893));
#58361=CARTESIAN_POINT('Ctrl Pts',(1.5237734895035,-1.,3.4388889597401));
#58362=CARTESIAN_POINT('Ctrl Pts',(1.5237734895035,1.,3.4388889597401));
#58363=CARTESIAN_POINT('Ctrl Pts',(1.52686242875556,-1.,3.44469547526647));
#58364=CARTESIAN_POINT('Ctrl Pts',(1.52686242875556,1.,3.44469547526647));
#58365=CARTESIAN_POINT('Ctrl Pts',(1.53046244461635,-1.,3.45127136828305));
#58366=CARTESIAN_POINT('Ctrl Pts',(1.53046244461635,1.,3.45127136828305));
#58367=CARTESIAN_POINT('Ctrl Pts',(1.53440195378792,-1.,3.45825932955032));
#58368=CARTESIAN_POINT('Ctrl Pts',(1.53440195378792,1.,3.45825932955032));
#58369=CARTESIAN_POINT('Ctrl Pts',(1.53851507915502,-1.,3.46531752207153));
#58370=CARTESIAN_POINT('Ctrl Pts',(1.53851507915502,1.,3.46531752207153));
#58371=CARTESIAN_POINT('Ctrl Pts',(1.54266605398187,-1.,3.47217189224653));
#58372=CARTESIAN_POINT('Ctrl Pts',(1.54266605398187,1.,3.47217189224653));
#58373=CARTESIAN_POINT('Ctrl Pts',(1.54678009290276,-1.,3.47868272898751));
#58374=CARTESIAN_POINT('Ctrl Pts',(1.54678009290276,1.,3.47868272898751));
#58375=CARTESIAN_POINT('Ctrl Pts',(1.55084702970452,-1.,3.48485155928567));
#58376=CARTESIAN_POINT('Ctrl Pts',(1.55084702970452,1.,3.48485155928567));
#58377=CARTESIAN_POINT('Ctrl Pts',(1.55489595901116,-1.,3.4907646087742));
#58378=CARTESIAN_POINT('Ctrl Pts',(1.55489595901116,1.,3.4907646087742));
#58379=CARTESIAN_POINT('Ctrl Pts',(1.55897703097874,-1.,3.49655185179655));
#58380=CARTESIAN_POINT('Ctrl Pts',(1.55897703097874,1.,3.49655185179655));
#58381=CARTESIAN_POINT('Ctrl Pts',(1.56314187758675,-1.,3.50234321621578));
#58382=CARTESIAN_POINT('Ctrl Pts',(1.56314187758675,1.,3.50234321621578));
#58383=CARTESIAN_POINT('Ctrl Pts',(1.56742097575012,-1.,3.50821771695363));
#58384=CARTESIAN_POINT('Ctrl Pts',(1.56742097575012,1.,3.50821771695363));
#58385=CARTESIAN_POINT('Ctrl Pts',(1.57181569799743,-1.,3.51418598431665));
#58386=CARTESIAN_POINT('Ctrl Pts',(1.57181569799743,1.,3.51418598431665));
#58387=CARTESIAN_POINT('Ctrl Pts',(1.57631049988158,-1.,3.52021847865912));
#58388=CARTESIAN_POINT('Ctrl Pts',(1.57631049988158,1.,3.52021847865912));
#58389=CARTESIAN_POINT('Ctrl Pts',(1.58088027227848,-1.,3.52626275334881));
#58390=CARTESIAN_POINT('Ctrl Pts',(1.58088027227848,1.,3.52626275334881));
#58391=CARTESIAN_POINT('Ctrl Pts',(1.58549906268088,-1.,3.5322637814708));
#58392=CARTESIAN_POINT('Ctrl Pts',(1.58549906268088,1.,3.5322637814708));
#58393=CARTESIAN_POINT('Ctrl Pts',(1.59014958368739,-1.,3.53818616861077));
#58394=CARTESIAN_POINT('Ctrl Pts',(1.59014958368739,1.,3.53818616861077));
#58395=CARTESIAN_POINT('Ctrl Pts',(1.59482766949766,-1.,3.54402458182337));
#58396=CARTESIAN_POINT('Ctrl Pts',(1.59482766949766,1.,3.54402458182337));
#58397=CARTESIAN_POINT('Ctrl Pts',(1.59953698113457,-1.,3.54979148634454));
#58398=CARTESIAN_POINT('Ctrl Pts',(1.59953698113457,1.,3.54979148634454));
#58399=CARTESIAN_POINT('Ctrl Pts',(1.60428584699853,-1.,3.55550985096129));
#58400=CARTESIAN_POINT('Ctrl Pts',(1.60428584699853,1.,3.55550985096129));
#58401=CARTESIAN_POINT('Ctrl Pts',(1.60908344685457,-1.,3.5612043248298));
#58402=CARTESIAN_POINT('Ctrl Pts',(1.60908344685457,1.,3.5612043248298));
#58403=CARTESIAN_POINT('Ctrl Pts',(1.61393581747514,-1.,3.56689200468387));
#58404=CARTESIAN_POINT('Ctrl Pts',(1.61393581747514,1.,3.56689200468387));
#58405=CARTESIAN_POINT('Ctrl Pts',(1.61884340915404,-1.,3.57257679609806));
#58406=CARTESIAN_POINT('Ctrl Pts',(1.61884340915404,1.,3.57257679609806));
#58407=CARTESIAN_POINT('Ctrl Pts',(1.62380329464844,-1.,3.5782545595439));
#58408=CARTESIAN_POINT('Ctrl Pts',(1.62380329464844,1.,3.5782545595439));
#58409=CARTESIAN_POINT('Ctrl Pts',(1.62881051550745,-1.,3.58391625774343));
#58410=CARTESIAN_POINT('Ctrl Pts',(1.62881051550745,1.,3.58391625774343));
#58411=CARTESIAN_POINT('Ctrl Pts',(1.6338597145126,-1.,3.58955176627879));
#58412=CARTESIAN_POINT('Ctrl Pts',(1.6338597145126,1.,3.58955176627879));
#58413=CARTESIAN_POINT('Ctrl Pts',(1.63894676675352,-1.,3.59515368334893));
#58414=CARTESIAN_POINT('Ctrl Pts',(1.63894676675352,1.,3.59515368334893));
#58415=CARTESIAN_POINT('Ctrl Pts',(1.64407004385582,-1.,3.60072028513845));
#58416=CARTESIAN_POINT('Ctrl Pts',(1.64407004385582,1.,3.60072028513845));
#58417=CARTESIAN_POINT('Ctrl Pts',(1.64922952425832,-1.,3.60625346556992));
#58418=CARTESIAN_POINT('Ctrl Pts',(1.64922952425832,1.,3.60625346556992));
#58419=CARTESIAN_POINT('Ctrl Pts',(1.65442619244325,-1.,3.61175734965127));
#58420=CARTESIAN_POINT('Ctrl Pts',(1.65442619244325,1.,3.61175734965127));
#58421=CARTESIAN_POINT('Ctrl Pts',(1.65966133399186,-1.,3.61723666482456));
#58422=CARTESIAN_POINT('Ctrl Pts',(1.65966133399186,1.,3.61723666482456));
#58423=CARTESIAN_POINT('Ctrl Pts',(1.66493585923855,-1.,3.62269517989109));
#58424=CARTESIAN_POINT('Ctrl Pts',(1.66493585923855,1.,3.62269517989109));
#58425=CARTESIAN_POINT('Ctrl Pts',(1.67024966008044,-1.,3.62813422105271));
#58426=CARTESIAN_POINT('Ctrl Pts',(1.67024966008044,1.,3.62813422105271));
#58427=CARTESIAN_POINT('Ctrl Pts',(1.67560193613156,-1.,3.63355343201232));
#58428=CARTESIAN_POINT('Ctrl Pts',(1.67560193613156,1.,3.63355343201232));
#58429=CARTESIAN_POINT('Ctrl Pts',(1.68099146651586,-1.,3.63895140887462));
#58430=CARTESIAN_POINT('Ctrl Pts',(1.68099146651586,1.,3.63895140887462));
#58431=CARTESIAN_POINT('Ctrl Pts',(1.68641690471457,-1.,3.64432638915203));
#58432=CARTESIAN_POINT('Ctrl Pts',(1.68641690471457,1.,3.64432638915203));
#58433=CARTESIAN_POINT('Ctrl Pts',(1.69187705481689,-1.,3.64967689827371));
#58434=CARTESIAN_POINT('Ctrl Pts',(1.69187705481689,1.,3.64967689827371));
#58435=CARTESIAN_POINT('Ctrl Pts',(1.69737117722534,-1.,3.65500246526749));
#58436=CARTESIAN_POINT('Ctrl Pts',(1.69737117722534,1.,3.65500246526749));
#58437=CARTESIAN_POINT('Ctrl Pts',(1.70289888566873,-1.,3.66030338774847));
#58438=CARTESIAN_POINT('Ctrl Pts',(1.70289888566873,1.,3.66030338774847));
#58439=CARTESIAN_POINT('Ctrl Pts',(1.70846001610956,-1.,3.66558043198876));
#58440=CARTESIAN_POINT('Ctrl Pts',(1.70846001610956,1.,3.66558043198876));
#58441=CARTESIAN_POINT('Ctrl Pts',(1.71405450210383,-1.,3.67083454901611));
#58442=CARTESIAN_POINT('Ctrl Pts',(1.71405450210383,1.,3.67083454901611));
#58443=CARTESIAN_POINT('Ctrl Pts',(1.71968225581808,-1.,3.67606660374709));
#58444=CARTESIAN_POINT('Ctrl Pts',(1.71968225581808,1.,3.67606660374709));
#58445=CARTESIAN_POINT('Ctrl Pts',(1.72534302437056,-1.,3.68127704936579));
#58446=CARTESIAN_POINT('Ctrl Pts',(1.72534302437056,1.,3.68127704936579));
#58447=CARTESIAN_POINT('Ctrl Pts',(1.73103640956717,-1.,3.68646597019332));
#58448=CARTESIAN_POINT('Ctrl Pts',(1.73103640956717,1.,3.68646597019332));
#58449=CARTESIAN_POINT('Ctrl Pts',(1.73676193254557,-1.,3.69163322648036));
#58450=CARTESIAN_POINT('Ctrl Pts',(1.73676193254557,1.,3.69163322648036));
#58451=CARTESIAN_POINT('Ctrl Pts',(1.74251908492617,-1.,3.69677856910517));
#58452=CARTESIAN_POINT('Ctrl Pts',(1.74251908492617,1.,3.69677856910517));
#58453=CARTESIAN_POINT('Ctrl Pts',(1.74830738046057,-1.,3.7019017567335));
#58454=CARTESIAN_POINT('Ctrl Pts',(1.74830738046057,1.,3.7019017567335));
#58455=CARTESIAN_POINT('Ctrl Pts',(1.75412641804042,-1.,3.70700269736659));
#58456=CARTESIAN_POINT('Ctrl Pts',(1.75412641804042,1.,3.70700269736659));
#58457=CARTESIAN_POINT('Ctrl Pts',(1.75997588498865,-1.,3.71208146346136));
#58458=CARTESIAN_POINT('Ctrl Pts',(1.75997588498865,1.,3.71208146346136));
#58459=CARTESIAN_POINT('Ctrl Pts',(1.76585552124394,-1.,3.71713822377359));
#58460=CARTESIAN_POINT('Ctrl Pts',(1.76585552124394,1.,3.71713822377359));
#58461=CARTESIAN_POINT('Ctrl Pts',(1.77176509401761,-1.,3.72217319911254));
#58462=CARTESIAN_POINT('Ctrl Pts',(1.77176509401761,1.,3.72217319911254));
#58463=CARTESIAN_POINT('Ctrl Pts',(1.77770437039658,-1.,3.72718661205609));
#58464=CARTESIAN_POINT('Ctrl Pts',(1.77770437039658,1.,3.72718661205609));
#58465=CARTESIAN_POINT('Ctrl Pts',(1.78367308442901,-1.,3.7321786309547));
#58466=CARTESIAN_POINT('Ctrl Pts',(1.78367308442901,1.,3.7321786309547));
#58467=CARTESIAN_POINT('Ctrl Pts',(1.78967092823491,-1.,3.73714934730681));
#58468=CARTESIAN_POINT('Ctrl Pts',(1.78967092823491,1.,3.73714934730681));
#58469=CARTESIAN_POINT('Ctrl Pts',(1.79569757859422,-1.,3.74209880352445));
#58470=CARTESIAN_POINT('Ctrl Pts',(1.79569757859422,1.,3.74209880352445));
#58471=CARTESIAN_POINT('Ctrl Pts',(1.8017527148577,-1.,3.74702700875467));
#58472=CARTESIAN_POINT('Ctrl Pts',(1.8017527148577,1.,3.74702700875467));
#58473=CARTESIAN_POINT('Ctrl Pts',(1.80783603939617,-1.,3.75193395887977));
#58474=CARTESIAN_POINT('Ctrl Pts',(1.80783603939617,1.,3.75193395887977));
#58475=CARTESIAN_POINT('Ctrl Pts',(1.8139472983358,-1.,3.75681965683071));
#58476=CARTESIAN_POINT('Ctrl Pts',(1.8139472983358,1.,3.75681965683071));
#58477=CARTESIAN_POINT('Ctrl Pts',(1.82008629694091,-1.,3.76168412707948));
#58478=CARTESIAN_POINT('Ctrl Pts',(1.82008629694091,1.,3.76168412707948));
#58479=CARTESIAN_POINT('Ctrl Pts',(1.82625289220915,-1.,3.76652740353775));
#58480=CARTESIAN_POINT('Ctrl Pts',(1.82625289220915,1.,3.76652740353775));
#58481=CARTESIAN_POINT('Ctrl Pts',(1.83120816955645,-1.,3.77038509817999));
#58482=CARTESIAN_POINT('Ctrl Pts',(1.83120816955645,1.,3.77038509817999));
#58483=CARTESIAN_POINT('Ctrl Pts',(1.83493697934534,-1.,3.77326886064398));
#58484=CARTESIAN_POINT('Ctrl Pts',(1.83493697934534,1.,3.77326886064398));
#58485=CARTESIAN_POINT('Ctrl Pts',(1.83742834010626,-1.,3.77518714457833));
#58486=CARTESIAN_POINT('Ctrl Pts',(1.83742834010626,1.,3.77518714457833));
#58487=CARTESIAN_POINT('Ctrl Pts',(1.8386753923786,-1.,3.77614523045147));
#58488=CARTESIAN_POINT('Ctrl Pts',(1.8386753923786,1.,3.77614523045147));
#58489=CARTESIAN_POINT('',(1.5189508286633,1.,3.42859860294306));
#58490=CARTESIAN_POINT('Ctrl Pts',(1.5189508286633,-1.,3.42859860294306));
#58491=CARTESIAN_POINT('Ctrl Pts',(1.5189508286633,-0.666666666666667,3.42859860294306));
#58492=CARTESIAN_POINT('Ctrl Pts',(1.5189508286633,-0.333333333333333,3.42859860294306));
#58493=CARTESIAN_POINT('Ctrl Pts',(1.5189508286633,0.333333333333333,3.42859860294306));
#58494=CARTESIAN_POINT('Ctrl Pts',(1.5189508286633,0.666666666666667,3.42859860294306));
#58495=CARTESIAN_POINT('Ctrl Pts',(1.5189508286633,1.,3.42859860294306));
#58496=CARTESIAN_POINT('',(1.8386753923786,1.,3.77614523045147));
#58497=CARTESIAN_POINT('',(1.8386753923786,0.,3.77614523045147));
#58498=CARTESIAN_POINT('Ctrl Pts',(1.5189508286633,1.,3.42859860294306));
#58499=CARTESIAN_POINT('Ctrl Pts',(1.51893924967331,1.,3.42864616361875));
#58500=CARTESIAN_POINT('Ctrl Pts',(1.5189513329503,1.,3.42884302333841));
#58501=CARTESIAN_POINT('Ctrl Pts',(1.51914806898491,1.,3.42946838852587));
#58502=CARTESIAN_POINT('Ctrl Pts',(1.5198144909338,1.,3.43101631893414));
#58503=CARTESIAN_POINT('Ctrl Pts',(1.52134826724292,1.,3.43417156977893));
#58504=CARTESIAN_POINT('Ctrl Pts',(1.5237734895035,1.,3.4388889597401));
#58505=CARTESIAN_POINT('Ctrl Pts',(1.52686242875556,1.,3.44469547526647));
#58506=CARTESIAN_POINT('Ctrl Pts',(1.53046244461635,1.,3.45127136828305));
#58507=CARTESIAN_POINT('Ctrl Pts',(1.53440195378792,1.,3.45825932955032));
#58508=CARTESIAN_POINT('Ctrl Pts',(1.53851507915502,1.,3.46531752207153));
#58509=CARTESIAN_POINT('Ctrl Pts',(1.54266605398187,1.,3.47217189224653));
#58510=CARTESIAN_POINT('Ctrl Pts',(1.54678009290276,1.,3.47868272898751));
#58511=CARTESIAN_POINT('Ctrl Pts',(1.55084702970452,1.,3.48485155928567));
#58512=CARTESIAN_POINT('Ctrl Pts',(1.55489595901116,1.,3.4907646087742));
#58513=CARTESIAN_POINT('Ctrl Pts',(1.55897703097874,1.,3.49655185179655));
#58514=CARTESIAN_POINT('Ctrl Pts',(1.56314187758675,1.,3.50234321621578));
#58515=CARTESIAN_POINT('Ctrl Pts',(1.56742097575012,1.,3.50821771695363));
#58516=CARTESIAN_POINT('Ctrl Pts',(1.57181569799743,1.,3.51418598431665));
#58517=CARTESIAN_POINT('Ctrl Pts',(1.57631049988158,1.,3.52021847865912));
#58518=CARTESIAN_POINT('Ctrl Pts',(1.58088027227848,1.,3.52626275334881));
#58519=CARTESIAN_POINT('Ctrl Pts',(1.58549906268088,1.,3.5322637814708));
#58520=CARTESIAN_POINT('Ctrl Pts',(1.59014958368739,1.,3.53818616861077));
#58521=CARTESIAN_POINT('Ctrl Pts',(1.59482766949766,1.,3.54402458182337));
#58522=CARTESIAN_POINT('Ctrl Pts',(1.59953698113457,1.,3.54979148634454));
#58523=CARTESIAN_POINT('Ctrl Pts',(1.60428584699853,1.,3.55550985096129));
#58524=CARTESIAN_POINT('Ctrl Pts',(1.60908344685457,1.,3.5612043248298));
#58525=CARTESIAN_POINT('Ctrl Pts',(1.61393581747514,1.,3.56689200468387));
#58526=CARTESIAN_POINT('Ctrl Pts',(1.61884340915404,1.,3.57257679609806));
#58527=CARTESIAN_POINT('Ctrl Pts',(1.62380329464844,1.,3.5782545595439));
#58528=CARTESIAN_POINT('Ctrl Pts',(1.62881051550745,1.,3.58391625774343));
#58529=CARTESIAN_POINT('Ctrl Pts',(1.6338597145126,1.,3.58955176627879));
#58530=CARTESIAN_POINT('Ctrl Pts',(1.63894676675352,1.,3.59515368334893));
#58531=CARTESIAN_POINT('Ctrl Pts',(1.64407004385582,1.,3.60072028513845));
#58532=CARTESIAN_POINT('Ctrl Pts',(1.64922952425832,1.,3.60625346556992));
#58533=CARTESIAN_POINT('Ctrl Pts',(1.65442619244325,1.,3.61175734965127));
#58534=CARTESIAN_POINT('Ctrl Pts',(1.65966133399186,1.,3.61723666482456));
#58535=CARTESIAN_POINT('Ctrl Pts',(1.66493585923855,1.,3.62269517989109));
#58536=CARTESIAN_POINT('Ctrl Pts',(1.67024966008044,1.,3.62813422105271));
#58537=CARTESIAN_POINT('Ctrl Pts',(1.67560193613156,1.,3.63355343201232));
#58538=CARTESIAN_POINT('Ctrl Pts',(1.68099146651586,1.,3.63895140887462));
#58539=CARTESIAN_POINT('Ctrl Pts',(1.68641690471457,1.,3.64432638915203));
#58540=CARTESIAN_POINT('Ctrl Pts',(1.69187705481689,1.,3.64967689827371));
#58541=CARTESIAN_POINT('Ctrl Pts',(1.69737117722534,1.,3.65500246526749));
#58542=CARTESIAN_POINT('Ctrl Pts',(1.70289888566873,1.,3.66030338774847));
#58543=CARTESIAN_POINT('Ctrl Pts',(1.70846001610956,1.,3.66558043198876));
#58544=CARTESIAN_POINT('Ctrl Pts',(1.71405450210383,1.,3.67083454901611));
#58545=CARTESIAN_POINT('Ctrl Pts',(1.71968225581808,1.,3.67606660374709));
#58546=CARTESIAN_POINT('Ctrl Pts',(1.72534302437056,1.,3.68127704936579));
#58547=CARTESIAN_POINT('Ctrl Pts',(1.73103640956717,1.,3.68646597019332));
#58548=CARTESIAN_POINT('Ctrl Pts',(1.73676193254557,1.,3.69163322648036));
#58549=CARTESIAN_POINT('Ctrl Pts',(1.74251908492617,1.,3.69677856910517));
#58550=CARTESIAN_POINT('Ctrl Pts',(1.74830738046057,1.,3.7019017567335));
#58551=CARTESIAN_POINT('Ctrl Pts',(1.75412641804042,1.,3.70700269736659));
#58552=CARTESIAN_POINT('Ctrl Pts',(1.75997588498865,1.,3.71208146346136));
#58553=CARTESIAN_POINT('Ctrl Pts',(1.76585552124394,1.,3.71713822377359));
#58554=CARTESIAN_POINT('Ctrl Pts',(1.77176509401761,1.,3.72217319911254));
#58555=CARTESIAN_POINT('Ctrl Pts',(1.77770437039658,1.,3.72718661205609));
#58556=CARTESIAN_POINT('Ctrl Pts',(1.78367308442901,1.,3.7321786309547));
#58557=CARTESIAN_POINT('Ctrl Pts',(1.78967092823491,1.,3.73714934730681));
#58558=CARTESIAN_POINT('Ctrl Pts',(1.79569757859422,1.,3.74209880352445));
#58559=CARTESIAN_POINT('Ctrl Pts',(1.8017527148577,1.,3.74702700875467));
#58560=CARTESIAN_POINT('Ctrl Pts',(1.80783603939617,1.,3.75193395887977));
#58561=CARTESIAN_POINT('Ctrl Pts',(1.8139472983358,1.,3.75681965683071));
#58562=CARTESIAN_POINT('Ctrl Pts',(1.82008629694091,1.,3.76168412707948));
#58563=CARTESIAN_POINT('Ctrl Pts',(1.82625289220915,1.,3.76652740353775));
#58564=CARTESIAN_POINT('Ctrl Pts',(1.83120816955645,1.,3.77038509817999));
#58565=CARTESIAN_POINT('Ctrl Pts',(1.83493697934534,1.,3.77326886064398));
#58566=CARTESIAN_POINT('Ctrl Pts',(1.83742834010626,1.,3.77518714457833));
#58567=CARTESIAN_POINT('Ctrl Pts',(1.8386753923786,1.,3.77614523045147));
#58568=CARTESIAN_POINT('Origin',(1.8386753923786,0.,3.77614523045147));
#58569=CARTESIAN_POINT('',(1.97421938526992,1.,3.70708211654725));
#58570=CARTESIAN_POINT('Origin',(0.,0.,0.));
#58571=CARTESIAN_POINT('',(1.35032489087269,1.,3.49844575334386));
#58572=CARTESIAN_POINT('Origin',(0.,1.,0.));
#58573=CARTESIAN_POINT('Ctrl Pts',(1.35032489087269,1.,3.49844575334386));
#58574=CARTESIAN_POINT('Ctrl Pts',(1.35032489087269,0.666666666666667,3.49844575334386));
#58575=CARTESIAN_POINT('Ctrl Pts',(1.35032489087269,0.333333333333333,3.49844575334386));
#58576=CARTESIAN_POINT('Ctrl Pts',(1.35032489087269,-0.333333333333333,
3.49844575334386));
#58577=CARTESIAN_POINT('Ctrl Pts',(1.35032489087269,-0.666666666666667,
3.49844575334386));
#58578=CARTESIAN_POINT('Ctrl Pts',(1.35032489087269,-1.,3.49844575334386));
#58579=CARTESIAN_POINT('Ctrl Pts',(1.36999806084572,-1.,3.97027773754922));
#58580=CARTESIAN_POINT('Ctrl Pts',(1.36999806084572,1.,3.97027773754922));
#58581=CARTESIAN_POINT('Ctrl Pts',(1.37020239094758,-1.,3.9687184694173));
#58582=CARTESIAN_POINT('Ctrl Pts',(1.37020239094758,1.,3.9687184694173));
#58583=CARTESIAN_POINT('Ctrl Pts',(1.37060761746027,-1.,3.96560037975788));
#58584=CARTESIAN_POINT('Ctrl Pts',(1.37060761746027,1.,3.96560037975788));
#58585=CARTESIAN_POINT('Ctrl Pts',(1.37120515615663,-1.,3.96092458508407));
#58586=CARTESIAN_POINT('Ctrl Pts',(1.37120515615663,1.,3.96092458508407));
#58587=CARTESIAN_POINT('Ctrl Pts',(1.37198126433139,-1.,3.95469287283105));
#58588=CARTESIAN_POINT('Ctrl Pts',(1.37198126433139,1.,3.95469287283105));
#58589=CARTESIAN_POINT('Ctrl Pts',(1.37291699203423,-1.,3.94690771786926));
#58590=CARTESIAN_POINT('Ctrl Pts',(1.37291699203423,1.,3.94690771786926));
#58591=CARTESIAN_POINT('Ctrl Pts',(1.37381821967499,-1.,3.93912709041791));
#58592=CARTESIAN_POINT('Ctrl Pts',(1.37381821967499,1.,3.93912709041791));
#58593=CARTESIAN_POINT('Ctrl Pts',(1.37468482215784,-1.,3.93135106761941));
#58594=CARTESIAN_POINT('Ctrl Pts',(1.37468482215784,1.,3.93135106761941));
#58595=CARTESIAN_POINT('Ctrl Pts',(1.37551664448057,-1.,3.92357976987132));
#58596=CARTESIAN_POINT('Ctrl Pts',(1.37551664448057,1.,3.92357976987132));
#58597=CARTESIAN_POINT('Ctrl Pts',(1.37631350505516,-1.,3.91581337461825));
#58598=CARTESIAN_POINT('Ctrl Pts',(1.37631350505516,1.,3.91581337461825));
#58599=CARTESIAN_POINT('Ctrl Pts',(1.3770751963376,-1.,3.90805209522729));
#58600=CARTESIAN_POINT('Ctrl Pts',(1.3770751963376,1.,3.90805209522729));
#58601=CARTESIAN_POINT('Ctrl Pts',(1.3778014851263,-1.,3.90029615196255));
#58602=CARTESIAN_POINT('Ctrl Pts',(1.3778014851263,1.,3.90029615196255));
#58603=CARTESIAN_POINT('Ctrl Pts',(1.37849211287981,-1.,3.89254574338385));
#58604=CARTESIAN_POINT('Ctrl Pts',(1.37849211287981,1.,3.89254574338385));
#58605=CARTESIAN_POINT('Ctrl Pts',(1.37914679719446,-1.,3.88480102249461));
#58606=CARTESIAN_POINT('Ctrl Pts',(1.37914679719446,1.,3.88480102249461));
#58607=CARTESIAN_POINT('Ctrl Pts',(1.37976523097187,-1.,3.87706205830865));
#58608=CARTESIAN_POINT('Ctrl Pts',(1.37976523097187,1.,3.87706205830865));
#58609=CARTESIAN_POINT('Ctrl Pts',(1.38034709213129,-1.,3.86932885813403));
#58610=CARTESIAN_POINT('Ctrl Pts',(1.38034709213129,1.,3.86932885813403));
#58611=CARTESIAN_POINT('Ctrl Pts',(1.38089205993067,-1.,3.86160143044187));
#58612=CARTESIAN_POINT('Ctrl Pts',(1.38089205993067,1.,3.86160143044187));
#58613=CARTESIAN_POINT('Ctrl Pts',(1.38139983115075,-1.,3.85387983979557));
#58614=CARTESIAN_POINT('Ctrl Pts',(1.38139983115075,1.,3.85387983979557));
#58615=CARTESIAN_POINT('Ctrl Pts',(1.38187013346089,-1.,3.84616425605705));
#58616=CARTESIAN_POINT('Ctrl Pts',(1.38187013346089,1.,3.84616425605705));
#58617=CARTESIAN_POINT('Ctrl Pts',(1.38230274828774,-1.,3.83845502790609));
#58618=CARTESIAN_POINT('Ctrl Pts',(1.38230274828774,1.,3.83845502790609));
#58619=CARTESIAN_POINT('Ctrl Pts',(1.38269750245086,-1.,3.83075266982138));
#58620=CARTESIAN_POINT('Ctrl Pts',(1.38269750245086,1.,3.83075266982138));
#58621=CARTESIAN_POINT('Ctrl Pts',(1.38305421262724,-1.,3.82305771743715));
#58622=CARTESIAN_POINT('Ctrl Pts',(1.38305421262724,1.,3.82305771743715));
#58623=CARTESIAN_POINT('Ctrl Pts',(1.38337263902766,-1.,3.81537060817765));
#58624=CARTESIAN_POINT('Ctrl Pts',(1.38337263902766,1.,3.81537060817765));
#58625=CARTESIAN_POINT('Ctrl Pts',(1.38365244046226,-1.,3.80769156398429));
#58626=CARTESIAN_POINT('Ctrl Pts',(1.38365244046226,1.,3.80769156398429));
#58627=CARTESIAN_POINT('Ctrl Pts',(1.38389311766701,-1.,3.80002044322169));
#58628=CARTESIAN_POINT('Ctrl Pts',(1.38389311766701,1.,3.80002044322169));
#58629=CARTESIAN_POINT('Ctrl Pts',(1.38409399694588,-1.,3.79235669640907));
#58630=CARTESIAN_POINT('Ctrl Pts',(1.38409399694588,1.,3.79235669640907));
#58631=CARTESIAN_POINT('Ctrl Pts',(1.38425435883773,-1.,3.78469969805134));
#58632=CARTESIAN_POINT('Ctrl Pts',(1.38425435883773,1.,3.78469969805134));
#58633=CARTESIAN_POINT('Ctrl Pts',(1.38437354551435,-1.,3.77704902230441));
#58634=CARTESIAN_POINT('Ctrl Pts',(1.38437354551435,1.,3.77704902230441));
#58635=CARTESIAN_POINT('Ctrl Pts',(1.38445107339517,-1.,3.76940473185775));
#58636=CARTESIAN_POINT('Ctrl Pts',(1.38445107339517,1.,3.76940473185775));
#58637=CARTESIAN_POINT('Ctrl Pts',(1.38448675253343,-1.,3.76176768271347));
#58638=CARTESIAN_POINT('Ctrl Pts',(1.38448675253343,1.,3.76176768271347));
#58639=CARTESIAN_POINT('Ctrl Pts',(1.38448077997155,-1.,3.75413976318727));
#58640=CARTESIAN_POINT('Ctrl Pts',(1.38448077997155,1.,3.75413976318727));
#58641=CARTESIAN_POINT('Ctrl Pts',(1.38443344984389,-1.,3.7465231716786));
#58642=CARTESIAN_POINT('Ctrl Pts',(1.38443344984389,1.,3.7465231716786));
#58643=CARTESIAN_POINT('Ctrl Pts',(1.38434489156456,-1.,3.73891976418099));
#58644=CARTESIAN_POINT('Ctrl Pts',(1.38434489156456,1.,3.73891976418099));
#58645=CARTESIAN_POINT('Ctrl Pts',(1.38421479111531,-1.,3.73133035859283));
#58646=CARTESIAN_POINT('Ctrl Pts',(1.38421479111531,1.,3.73133035859283));
#58647=CARTESIAN_POINT('Ctrl Pts',(1.3840421342895,-1.,3.72375409358805));
#58648=CARTESIAN_POINT('Ctrl Pts',(1.3840421342895,1.,3.72375409358805));
#58649=CARTESIAN_POINT('Ctrl Pts',(1.38382489984585,-1.,3.7161876605181));
#58650=CARTESIAN_POINT('Ctrl Pts',(1.38382489984585,1.,3.7161876605181));
#58651=CARTESIAN_POINT('Ctrl Pts',(1.38356065402122,-1.,3.70862680753343));
#58652=CARTESIAN_POINT('Ctrl Pts',(1.38356065402122,1.,3.70862680753343));
#58653=CARTESIAN_POINT('Ctrl Pts',(1.38324717612862,-1.,3.70106792167894));
#58654=CARTESIAN_POINT('Ctrl Pts',(1.38324717612862,1.,3.70106792167894));
#58655=CARTESIAN_POINT('Ctrl Pts',(1.38288311171649,-1.,3.69350967899523));
#58656=CARTESIAN_POINT('Ctrl Pts',(1.38288311171649,1.,3.69350967899523));
#58657=CARTESIAN_POINT('Ctrl Pts',(1.38246852827185,-1.,3.68595444983844));
#58658=CARTESIAN_POINT('Ctrl Pts',(1.38246852827185,1.,3.68595444983844));
#58659=CARTESIAN_POINT('Ctrl Pts',(1.38200574290626,-1.,3.6784103848243));
#58660=CARTESIAN_POINT('Ctrl Pts',(1.38200574290626,1.,3.6784103848243));
#58661=CARTESIAN_POINT('Ctrl Pts',(1.38149812653876,-1.,3.67088843112282));
#58662=CARTESIAN_POINT('Ctrl Pts',(1.38149812653876,1.,3.67088843112282));
#58663=CARTESIAN_POINT('Ctrl Pts',(1.38094856333558,-1.,3.66339848520874));
#58664=CARTESIAN_POINT('Ctrl Pts',(1.38094856333558,1.,3.66339848520874));
#58665=CARTESIAN_POINT('Ctrl Pts',(1.38035791051215,-1.,3.65594554404396));
#58666=CARTESIAN_POINT('Ctrl Pts',(1.38035791051215,1.,3.65594554404396));
#58667=CARTESIAN_POINT('Ctrl Pts',(1.37972372481598,-1.,3.64852652756444));
#58668=CARTESIAN_POINT('Ctrl Pts',(1.37972372481598,1.,3.64852652756444));
#58669=CARTESIAN_POINT('Ctrl Pts',(1.37903818567347,-1.,3.64112507791112));
#58670=CARTESIAN_POINT('Ctrl Pts',(1.37903818567347,1.,3.64112507791112));
#58671=CARTESIAN_POINT('Ctrl Pts',(1.37829035457324,-1.,3.63371727442448));
#58672=CARTESIAN_POINT('Ctrl Pts',(1.37829035457324,1.,3.63371727442448));
#58673=CARTESIAN_POINT('Ctrl Pts',(1.37746987919868,-1.,3.62628098665112));
#58674=CARTESIAN_POINT('Ctrl Pts',(1.37746987919868,1.,3.62628098665112));
#58675=CARTESIAN_POINT('Ctrl Pts',(1.37657053403102,-1.,3.61880481160408));
#58676=CARTESIAN_POINT('Ctrl Pts',(1.37657053403102,1.,3.61880481160408));
#58677=CARTESIAN_POINT('Ctrl Pts',(1.37559314436641,-1.,3.61129546591082));
#58678=CARTESIAN_POINT('Ctrl Pts',(1.37559314436641,1.,3.61129546591082));
#58679=CARTESIAN_POINT('Ctrl Pts',(1.37455051379642,-1.,3.60379020124038));
#58680=CARTESIAN_POINT('Ctrl Pts',(1.37455051379642,1.,3.60379020124038));
#58681=CARTESIAN_POINT('Ctrl Pts',(1.37346320103184,-1.,3.59634627869117));
#58682=CARTESIAN_POINT('Ctrl Pts',(1.37346320103184,1.,3.59634627869117));
#58683=CARTESIAN_POINT('Ctrl Pts',(1.37235053661,-1.,3.5890185384643));
#58684=CARTESIAN_POINT('Ctrl Pts',(1.37235053661,1.,3.5890185384643));
#58685=CARTESIAN_POINT('Ctrl Pts',(1.37122241663073,-1.,3.58183885982745));
#58686=CARTESIAN_POINT('Ctrl Pts',(1.37122241663073,1.,3.58183885982745));
#58687=CARTESIAN_POINT('Ctrl Pts',(1.37007229485646,-1.,3.57479875549453));
#58688=CARTESIAN_POINT('Ctrl Pts',(1.37007229485646,1.,3.57479875549453));
#58689=CARTESIAN_POINT('Ctrl Pts',(1.36886584973349,-1.,3.56782080304554));
#58690=CARTESIAN_POINT('Ctrl Pts',(1.36886584973349,1.,3.56782080304554));
#58691=CARTESIAN_POINT('Ctrl Pts',(1.36754771771174,-1.,3.56077662028492));
#58692=CARTESIAN_POINT('Ctrl Pts',(1.36754771771174,1.,3.56077662028492));
#58693=CARTESIAN_POINT('Ctrl Pts',(1.36606145456711,-1.,3.55353883995793));
#58694=CARTESIAN_POINT('Ctrl Pts',(1.36606145456711,1.,3.55353883995793));
#58695=CARTESIAN_POINT('Ctrl Pts',(1.36436666257567,-1.,3.54602591832893));
#58696=CARTESIAN_POINT('Ctrl Pts',(1.36436666257567,1.,3.54602591832893));
#58697=CARTESIAN_POINT('Ctrl Pts',(1.36245507339334,-1.,3.53824396425032));
#58698=CARTESIAN_POINT('Ctrl Pts',(1.36245507339334,1.,3.53824396425032));
#58699=CARTESIAN_POINT('Ctrl Pts',(1.36037259643827,-1.,3.53034464961849));
#58700=CARTESIAN_POINT('Ctrl Pts',(1.36037259643827,1.,3.53034464961849));
#58701=CARTESIAN_POINT('Ctrl Pts',(1.35821701528975,-1.,3.52261776117121));
#58702=CARTESIAN_POINT('Ctrl Pts',(1.35821701528975,1.,3.52261776117121));
#58703=CARTESIAN_POINT('Ctrl Pts',(1.35611275237288,-1.,3.51542230699919));
#58704=CARTESIAN_POINT('Ctrl Pts',(1.35611275237288,1.,3.51542230699919));
#58705=CARTESIAN_POINT('Ctrl Pts',(1.35419113576022,-1.,3.50913227060177));
#58706=CARTESIAN_POINT('Ctrl Pts',(1.35419113576022,1.,3.50913227060177));
#58707=CARTESIAN_POINT('Ctrl Pts',(1.3525703284343,-1.,3.50408168106113));
#58708=CARTESIAN_POINT('Ctrl Pts',(1.3525703284343,1.,3.50408168106113));
#58709=CARTESIAN_POINT('Ctrl Pts',(1.35133076331065,-1.,3.50049707063673));
#58710=CARTESIAN_POINT('Ctrl Pts',(1.35133076331065,1.,3.50049707063673));
#58711=CARTESIAN_POINT('Ctrl Pts',(1.35067437417289,-1.,3.49888720256612));
#58712=CARTESIAN_POINT('Ctrl Pts',(1.35067437417289,1.,3.49888720256612));
#58713=CARTESIAN_POINT('Ctrl Pts',(1.35037650302887,-1.,3.49840357193384));
#58714=CARTESIAN_POINT('Ctrl Pts',(1.35037650302887,1.,3.49840357193384));
#58715=CARTESIAN_POINT('Ctrl Pts',(1.35026426118351,-1.,3.49840260053616));
#58716=CARTESIAN_POINT('Ctrl Pts',(1.35026426118351,1.,3.49840260053616));
#58717=CARTESIAN_POINT('Ctrl Pts',(1.35022972712301,-1.,3.49848248301936));
#58718=CARTESIAN_POINT('Ctrl Pts',(1.35022972712301,1.,3.49848248301936));
#58719=CARTESIAN_POINT('',(1.36999806084572,1.,3.97027773754922));
#58720=CARTESIAN_POINT('Ctrl Pts',(1.36999806084572,1.,3.97027773754922));
#58721=CARTESIAN_POINT('Ctrl Pts',(1.37020239094758,1.,3.9687184694173));
#58722=CARTESIAN_POINT('Ctrl Pts',(1.37060761746027,1.,3.96560037975788));
#58723=CARTESIAN_POINT('Ctrl Pts',(1.37120515615663,1.,3.96092458508407));
#58724=CARTESIAN_POINT('Ctrl Pts',(1.37198126433139,1.,3.95469287283105));
#58725=CARTESIAN_POINT('Ctrl Pts',(1.37291699203423,1.,3.94690771786926));
#58726=CARTESIAN_POINT('Ctrl Pts',(1.37381821967499,1.,3.93912709041791));
#58727=CARTESIAN_POINT('Ctrl Pts',(1.37468482215784,1.,3.93135106761941));
#58728=CARTESIAN_POINT('Ctrl Pts',(1.37551664448057,1.,3.92357976987132));
#58729=CARTESIAN_POINT('Ctrl Pts',(1.37631350505516,1.,3.91581337461825));
#58730=CARTESIAN_POINT('Ctrl Pts',(1.3770751963376,1.,3.90805209522729));
#58731=CARTESIAN_POINT('Ctrl Pts',(1.3778014851263,1.,3.90029615196255));
#58732=CARTESIAN_POINT('Ctrl Pts',(1.37849211287981,1.,3.89254574338385));
#58733=CARTESIAN_POINT('Ctrl Pts',(1.37914679719446,1.,3.88480102249461));
#58734=CARTESIAN_POINT('Ctrl Pts',(1.37976523097187,1.,3.87706205830865));
#58735=CARTESIAN_POINT('Ctrl Pts',(1.38034709213129,1.,3.86932885813403));
#58736=CARTESIAN_POINT('Ctrl Pts',(1.38089205993067,1.,3.86160143044187));
#58737=CARTESIAN_POINT('Ctrl Pts',(1.38139983115075,1.,3.85387983979557));
#58738=CARTESIAN_POINT('Ctrl Pts',(1.38187013346089,1.,3.84616425605705));
#58739=CARTESIAN_POINT('Ctrl Pts',(1.38230274828774,1.,3.83845502790609));
#58740=CARTESIAN_POINT('Ctrl Pts',(1.38269750245086,1.,3.83075266982138));
#58741=CARTESIAN_POINT('Ctrl Pts',(1.38305421262724,1.,3.82305771743715));
#58742=CARTESIAN_POINT('Ctrl Pts',(1.38337263902766,1.,3.81537060817765));
#58743=CARTESIAN_POINT('Ctrl Pts',(1.38365244046226,1.,3.80769156398429));
#58744=CARTESIAN_POINT('Ctrl Pts',(1.38389311766701,1.,3.80002044322169));
#58745=CARTESIAN_POINT('Ctrl Pts',(1.38409399694588,1.,3.79235669640907));
#58746=CARTESIAN_POINT('Ctrl Pts',(1.38425435883773,1.,3.78469969805134));
#58747=CARTESIAN_POINT('Ctrl Pts',(1.38437354551435,1.,3.77704902230441));
#58748=CARTESIAN_POINT('Ctrl Pts',(1.38445107339517,1.,3.76940473185775));
#58749=CARTESIAN_POINT('Ctrl Pts',(1.38448675253343,1.,3.76176768271347));
#58750=CARTESIAN_POINT('Ctrl Pts',(1.38448077997155,1.,3.75413976318727));
#58751=CARTESIAN_POINT('Ctrl Pts',(1.38443344984389,1.,3.7465231716786));
#58752=CARTESIAN_POINT('Ctrl Pts',(1.38434489156456,1.,3.73891976418099));
#58753=CARTESIAN_POINT('Ctrl Pts',(1.38421479111531,1.,3.73133035859283));
#58754=CARTESIAN_POINT('Ctrl Pts',(1.3840421342895,1.,3.72375409358805));
#58755=CARTESIAN_POINT('Ctrl Pts',(1.38382489984585,1.,3.7161876605181));
#58756=CARTESIAN_POINT('Ctrl Pts',(1.38356065402122,1.,3.70862680753343));
#58757=CARTESIAN_POINT('Ctrl Pts',(1.38324717612862,1.,3.70106792167894));
#58758=CARTESIAN_POINT('Ctrl Pts',(1.38288311171649,1.,3.69350967899523));
#58759=CARTESIAN_POINT('Ctrl Pts',(1.38246852827185,1.,3.68595444983844));
#58760=CARTESIAN_POINT('Ctrl Pts',(1.38200574290626,1.,3.6784103848243));
#58761=CARTESIAN_POINT('Ctrl Pts',(1.38149812653876,1.,3.67088843112282));
#58762=CARTESIAN_POINT('Ctrl Pts',(1.38094856333558,1.,3.66339848520874));
#58763=CARTESIAN_POINT('Ctrl Pts',(1.38035791051215,1.,3.65594554404396));
#58764=CARTESIAN_POINT('Ctrl Pts',(1.37972372481598,1.,3.64852652756444));
#58765=CARTESIAN_POINT('Ctrl Pts',(1.37903818567347,1.,3.64112507791112));
#58766=CARTESIAN_POINT('Ctrl Pts',(1.37829035457324,1.,3.63371727442448));
#58767=CARTESIAN_POINT('Ctrl Pts',(1.37746987919868,1.,3.62628098665112));
#58768=CARTESIAN_POINT('Ctrl Pts',(1.37657053403102,1.,3.61880481160408));
#58769=CARTESIAN_POINT('Ctrl Pts',(1.37559314436641,1.,3.61129546591082));
#58770=CARTESIAN_POINT('Ctrl Pts',(1.37455051379642,1.,3.60379020124038));
#58771=CARTESIAN_POINT('Ctrl Pts',(1.37346320103184,1.,3.59634627869117));
#58772=CARTESIAN_POINT('Ctrl Pts',(1.37235053661,1.,3.5890185384643));
#58773=CARTESIAN_POINT('Ctrl Pts',(1.37122241663073,1.,3.58183885982745));
#58774=CARTESIAN_POINT('Ctrl Pts',(1.37007229485646,1.,3.57479875549453));
#58775=CARTESIAN_POINT('Ctrl Pts',(1.36886584973349,1.,3.56782080304554));
#58776=CARTESIAN_POINT('Ctrl Pts',(1.36754771771174,1.,3.56077662028492));
#58777=CARTESIAN_POINT('Ctrl Pts',(1.36606145456711,1.,3.55353883995793));
#58778=CARTESIAN_POINT('Ctrl Pts',(1.36436666257567,1.,3.54602591832893));
#58779=CARTESIAN_POINT('Ctrl Pts',(1.36245507339334,1.,3.53824396425032));
#58780=CARTESIAN_POINT('Ctrl Pts',(1.36037259643827,1.,3.53034464961849));
#58781=CARTESIAN_POINT('Ctrl Pts',(1.35821701528975,1.,3.52261776117121));
#58782=CARTESIAN_POINT('Ctrl Pts',(1.35611275237288,1.,3.51542230699919));
#58783=CARTESIAN_POINT('Ctrl Pts',(1.35419113576022,1.,3.50913227060177));
#58784=CARTESIAN_POINT('Ctrl Pts',(1.3525703284343,1.,3.50408168106113));
#58785=CARTESIAN_POINT('Ctrl Pts',(1.35142377279535,1.,3.5007660381658));
#58786=CARTESIAN_POINT('Ctrl Pts',(1.35080045218652,1.,3.49920025459856));
#58787=CARTESIAN_POINT('Ctrl Pts',(1.35049736560633,1.,3.49861894124915));
#58788=CARTESIAN_POINT('Ctrl Pts',(1.35036670893102,1.,3.49847119623841));
#58789=CARTESIAN_POINT('Ctrl Pts',(1.35032489087269,1.,3.49844575334386));
#58790=CARTESIAN_POINT('',(1.36999806084572,0.,3.97027773754922));
#58791=CARTESIAN_POINT('Ctrl Pts',(0.96399761336957,-1.,3.62397690409552));
#58792=CARTESIAN_POINT('Ctrl Pts',(0.96399761336957,1.,3.62397690409552));
#58793=CARTESIAN_POINT('Ctrl Pts',(0.963922720982576,-1.,3.62393257642191));
#58794=CARTESIAN_POINT('Ctrl Pts',(0.963922720982576,1.,3.62393257642191));
#58795=CARTESIAN_POINT('Ctrl Pts',(0.963832486396055,-1.,3.62399933640277));
#58796=CARTESIAN_POINT('Ctrl Pts',(0.963832486396055,1.,3.62399933640277));
#58797=CARTESIAN_POINT('Ctrl Pts',(0.963875774532102,-1.,3.62456568607055));
#58798=CARTESIAN_POINT('Ctrl Pts',(0.963875774532102,1.,3.62456568607055));
#58799=CARTESIAN_POINT('Ctrl Pts',(0.964291001274618,-1.,3.62625391255277));
#58800=CARTESIAN_POINT('Ctrl Pts',(0.964291001274618,1.,3.62625391255277));
#58801=CARTESIAN_POINT('Ctrl Pts',(0.965395153165715,-1.,3.62988252139998));
#58802=CARTESIAN_POINT('Ctrl Pts',(0.965395153165715,1.,3.62988252139998));
#58803=CARTESIAN_POINT('Ctrl Pts',(0.967052554540877,-1.,3.6349212208096));
#58804=CARTESIAN_POINT('Ctrl Pts',(0.967052554540877,1.,3.6349212208096));
#58805=CARTESIAN_POINT('Ctrl Pts',(0.969195124674828,-1.,3.64113946505393));
#58806=CARTESIAN_POINT('Ctrl Pts',(0.969195124674828,1.,3.64113946505393));
#58807=CARTESIAN_POINT('Ctrl Pts',(0.971722122060277,-1.,3.64819756447072));
#58808=CARTESIAN_POINT('Ctrl Pts',(0.971722122060277,1.,3.64819756447072));
#58809=CARTESIAN_POINT('Ctrl Pts',(0.974519971354138,-1.,3.6557157673487));
#58810=CARTESIAN_POINT('Ctrl Pts',(0.974519971354138,1.,3.6557157673487));
#58811=CARTESIAN_POINT('Ctrl Pts',(0.977478312751416,-1.,3.66333049637403));
#58812=CARTESIAN_POINT('Ctrl Pts',(0.977478312751416,1.,3.66333049637403));
#58813=CARTESIAN_POINT('Ctrl Pts',(0.980505922458494,-1.,3.67074983340444));
#58814=CARTESIAN_POINT('Ctrl Pts',(0.980505922458494,1.,3.67074983340444));
#58815=CARTESIAN_POINT('Ctrl Pts',(0.983550791470864,-1.,3.67782408841876));
#58816=CARTESIAN_POINT('Ctrl Pts',(0.983550791470864,1.,3.67782408841876));
#58817=CARTESIAN_POINT('Ctrl Pts',(0.986602639864285,-1.,3.6845531792623));
#58818=CARTESIAN_POINT('Ctrl Pts',(0.986602639864285,1.,3.6845531792623));
#58819=CARTESIAN_POINT('Ctrl Pts',(0.989676715398858,-1.,3.69102682138955));
#58820=CARTESIAN_POINT('Ctrl Pts',(0.989676715398858,1.,3.69102682138955));
#58821=CARTESIAN_POINT('Ctrl Pts',(0.992802218332103,-1.,3.69738123415696));
#58822=CARTESIAN_POINT('Ctrl Pts',(0.992802218332103,1.,3.69738123415696));
#58823=CARTESIAN_POINT('Ctrl Pts',(0.996009819772431,-1.,3.70375282282107));
#58824=CARTESIAN_POINT('Ctrl Pts',(0.996009819772431,1.,3.70375282282107));
#58825=CARTESIAN_POINT('Ctrl Pts',(0.999317260756344,-1.,3.7102243971387));
#58826=CARTESIAN_POINT('Ctrl Pts',(0.999317260756344,1.,3.7102243971387));
#58827=CARTESIAN_POINT('Ctrl Pts',(1.00272423396802,-1.,3.71680667125047));
#58828=CARTESIAN_POINT('Ctrl Pts',(1.00272423396802,1.,3.71680667125047));
#58829=CARTESIAN_POINT('Ctrl Pts',(1.00622000735696,-1.,3.72346803750544));
#58830=CARTESIAN_POINT('Ctrl Pts',(1.00622000735696,1.,3.72346803750544));
#58831=CARTESIAN_POINT('Ctrl Pts',(1.00978798539491,-1.,3.73015276704407));
#58832=CARTESIAN_POINT('Ctrl Pts',(1.00978798539491,1.,3.73015276704407));
#58833=CARTESIAN_POINT('Ctrl Pts',(1.01341114319906,-1.,3.73680245055747));
#58834=CARTESIAN_POINT('Ctrl Pts',(1.01341114319906,1.,3.73680245055747));
#58835=CARTESIAN_POINT('Ctrl Pts',(1.01707794311088,-1.,3.74337942504993));
#58836=CARTESIAN_POINT('Ctrl Pts',(1.01707794311088,1.,3.74337942504993));
#58837=CARTESIAN_POINT('Ctrl Pts',(1.02078510487439,-1.,3.74987777155873));
#58838=CARTESIAN_POINT('Ctrl Pts',(1.02078510487439,1.,3.74987777155873));
#58839=CARTESIAN_POINT('Ctrl Pts',(1.02453429444668,-1.,3.75631037456224));
#58840=CARTESIAN_POINT('Ctrl Pts',(1.02453429444668,1.,3.75631037456224));
#58841=CARTESIAN_POINT('Ctrl Pts',(1.02833014458184,-1.,3.76270122291245));
#58842=CARTESIAN_POINT('Ctrl Pts',(1.02833014458184,1.,3.76270122291245));
#58843=CARTESIAN_POINT('Ctrl Pts',(1.03217786604919,-1.,3.76907609832516));
#58844=CARTESIAN_POINT('Ctrl Pts',(1.03217786604919,1.,3.76907609832516));
#58845=CARTESIAN_POINT('Ctrl Pts',(1.03608074678008,-1.,3.77545283140427));
#58846=CARTESIAN_POINT('Ctrl Pts',(1.03608074678008,1.,3.77545283140427));
#58847=CARTESIAN_POINT('Ctrl Pts',(1.04003862055798,-1.,3.7818353500817));
#58848=CARTESIAN_POINT('Ctrl Pts',(1.04003862055798,1.,3.7818353500817));
#58849=CARTESIAN_POINT('Ctrl Pts',(1.04404924374422,-1.,3.78821910787179));
#58850=CARTESIAN_POINT('Ctrl Pts',(1.04404924374422,1.,3.78821910787179));
#58851=CARTESIAN_POINT('Ctrl Pts',(1.04810913267639,-1.,3.79459440308786));
#58852=CARTESIAN_POINT('Ctrl Pts',(1.04810913267639,1.,3.79459440308786));
#58853=CARTESIAN_POINT('Ctrl Pts',(1.05221457990016,-1.,3.80095039790681));
#58854=CARTESIAN_POINT('Ctrl Pts',(1.05221457990016,1.,3.80095039790681));
#58855=CARTESIAN_POINT('Ctrl Pts',(1.05636266918644,-1.,3.80727913637791));
#58856=CARTESIAN_POINT('Ctrl Pts',(1.05636266918644,1.,3.80727913637791));
#58857=CARTESIAN_POINT('Ctrl Pts',(1.06055206187299,-1.,3.8135786611749));
#58858=CARTESIAN_POINT('Ctrl Pts',(1.06055206187299,1.,3.8135786611749));
#58859=CARTESIAN_POINT('Ctrl Pts',(1.0647824403893,-1.,3.81985083953012));
#58860=CARTESIAN_POINT('Ctrl Pts',(1.0647824403893,1.,3.81985083953012));
#58861=CARTESIAN_POINT('Ctrl Pts',(1.06905413180359,-1.,3.82609989967276));
#58862=CARTESIAN_POINT('Ctrl Pts',(1.06905413180359,1.,3.82609989967276));
#58863=CARTESIAN_POINT('Ctrl Pts',(1.07336766633459,-1.,3.83233071195144));
#58864=CARTESIAN_POINT('Ctrl Pts',(1.07336766633459,1.,3.83233071195144));
#58865=CARTESIAN_POINT('Ctrl Pts',(1.07772335353858,-1.,3.83854714117491));
#58866=CARTESIAN_POINT('Ctrl Pts',(1.07772335353858,1.,3.83854714117491));
#58867=CARTESIAN_POINT('Ctrl Pts',(1.08212087917991,-1.,3.8447504803063));
#58868=CARTESIAN_POINT('Ctrl Pts',(1.08212087917991,1.,3.8447504803063));
#58869=CARTESIAN_POINT('Ctrl Pts',(1.08655950846384,-1.,3.85094025222713));
#58870=CARTESIAN_POINT('Ctrl Pts',(1.08655950846384,1.,3.85094025222713));
#58871=CARTESIAN_POINT('Ctrl Pts',(1.09103825516294,-1.,3.85711487933931));
#58872=CARTESIAN_POINT('Ctrl Pts',(1.09103825516294,1.,3.85711487933931));
#58873=CARTESIAN_POINT('Ctrl Pts',(1.09555606505013,-1.,3.86327241021247));
#58874=CARTESIAN_POINT('Ctrl Pts',(1.09555606505013,1.,3.86327241021247));
#58875=CARTESIAN_POINT('Ctrl Pts',(1.10011198761195,-1.,3.86941120134849));
#58876=CARTESIAN_POINT('Ctrl Pts',(1.10011198761195,1.,3.86941120134849));
#58877=CARTESIAN_POINT('Ctrl Pts',(1.10470536603287,-1.,3.87553067187514));
#58878=CARTESIAN_POINT('Ctrl Pts',(1.10470536603287,1.,3.87553067187514));
#58879=CARTESIAN_POINT('Ctrl Pts',(1.10933577224008,-1.,3.88163105531724));
#58880=CARTESIAN_POINT('Ctrl Pts',(1.10933577224008,1.,3.88163105531724));
#58881=CARTESIAN_POINT('Ctrl Pts',(1.11400292434429,-1.,3.88771308285171));
#58882=CARTESIAN_POINT('Ctrl Pts',(1.11400292434429,1.,3.88771308285171));
#58883=CARTESIAN_POINT('Ctrl Pts',(1.11870660794603,-1.,3.89377768340344));
#58884=CARTESIAN_POINT('Ctrl Pts',(1.11870660794603,1.,3.89377768340344));
#58885=CARTESIAN_POINT('Ctrl Pts',(1.12344660099043,-1.,3.89982569750025));
#58886=CARTESIAN_POINT('Ctrl Pts',(1.12344660099043,1.,3.89982569750025));
#58887=CARTESIAN_POINT('Ctrl Pts',(1.12822258281553,-1.,3.90585753318737));
#58888=CARTESIAN_POINT('Ctrl Pts',(1.12822258281553,1.,3.90585753318737));
#58889=CARTESIAN_POINT('Ctrl Pts',(1.13303414693896,-1.,3.91187321145649));
#58890=CARTESIAN_POINT('Ctrl Pts',(1.13303414693896,1.,3.91187321145649));
#58891=CARTESIAN_POINT('Ctrl Pts',(1.13788084225554,-1.,3.91787251936827));
#58892=CARTESIAN_POINT('Ctrl Pts',(1.13788084225554,1.,3.91787251936827));
#58893=CARTESIAN_POINT('Ctrl Pts',(1.14276220561593,-1.,3.92385513133997));
#58894=CARTESIAN_POINT('Ctrl Pts',(1.14276220561593,1.,3.92385513133997));
#58895=CARTESIAN_POINT('Ctrl Pts',(1.14767779451123,-1.,3.92982073294257));
#58896=CARTESIAN_POINT('Ctrl Pts',(1.14767779451123,1.,3.92982073294257));
#58897=CARTESIAN_POINT('Ctrl Pts',(1.1526272271632,-1.,3.9357691705628));
#58898=CARTESIAN_POINT('Ctrl Pts',(1.1526272271632,1.,3.9357691705628));
#58899=CARTESIAN_POINT('Ctrl Pts',(1.15761018340956,-1.,3.94170046685203));
#58900=CARTESIAN_POINT('Ctrl Pts',(1.15761018340956,1.,3.94170046685203));
#58901=CARTESIAN_POINT('Ctrl Pts',(1.16262637999157,-1.,3.94761474780583));
#58902=CARTESIAN_POINT('Ctrl Pts',(1.16262637999157,1.,3.94761474780583));
#58903=CARTESIAN_POINT('Ctrl Pts',(1.16767555244438,-1.,3.95351219509876));
#58904=CARTESIAN_POINT('Ctrl Pts',(1.16767555244438,1.,3.95351219509876));
#58905=CARTESIAN_POINT('Ctrl Pts',(1.17275743590361,-1.,3.95939299213276));
#58906=CARTESIAN_POINT('Ctrl Pts',(1.17275743590361,1.,3.95939299213276));
#58907=CARTESIAN_POINT('Ctrl Pts',(1.17787174135592,-1.,3.96525726358159));
#58908=CARTESIAN_POINT('Ctrl Pts',(1.17787174135592,1.,3.96525726358159));
#58909=CARTESIAN_POINT('Ctrl Pts',(1.18301815039831,-1.,3.97110505165415));
#58910=CARTESIAN_POINT('Ctrl Pts',(1.18301815039831,1.,3.97110505165415));
#58911=CARTESIAN_POINT('Ctrl Pts',(1.18819633715539,-1.,3.97693634767754));
#58912=CARTESIAN_POINT('Ctrl Pts',(1.18819633715539,1.,3.97693634767754));
#58913=CARTESIAN_POINT('Ctrl Pts',(1.19340598349475,-1.,3.98275111052561));
#58914=CARTESIAN_POINT('Ctrl Pts',(1.19340598349475,1.,3.98275111052561));
#58915=CARTESIAN_POINT('Ctrl Pts',(1.19864679609566,-1.,3.98854928957189));
#58916=CARTESIAN_POINT('Ctrl Pts',(1.19864679609566,1.,3.98854928957189));
#58917=CARTESIAN_POINT('Ctrl Pts',(1.20391852375138,-1.,3.99433084799666));
#58918=CARTESIAN_POINT('Ctrl Pts',(1.20391852375138,1.,3.99433084799666));
#58919=CARTESIAN_POINT('Ctrl Pts',(1.20922097029551,-1.,4.00009577950721));
#58920=CARTESIAN_POINT('Ctrl Pts',(1.20922097029551,1.,4.00009577950721));
#58921=CARTESIAN_POINT('Ctrl Pts',(1.21455398918133,-1.,4.00584409522722));
#58922=CARTESIAN_POINT('Ctrl Pts',(1.21455398918133,1.,4.00584409522722));
#58923=CARTESIAN_POINT('Ctrl Pts',(1.21884478244403,-1.,4.01042947140789));
#58924=CARTESIAN_POINT('Ctrl Pts',(1.21884478244403,1.,4.01042947140789));
#58925=CARTESIAN_POINT('Ctrl Pts',(1.22207656455845,-1.,4.01386104433519));
#58926=CARTESIAN_POINT('Ctrl Pts',(1.22207656455845,1.,4.01386104433519));
#58927=CARTESIAN_POINT('Ctrl Pts',(1.22423716681317,-1.,4.01614544569895));
#58928=CARTESIAN_POINT('Ctrl Pts',(1.22423716681317,1.,4.01614544569895));
#58929=CARTESIAN_POINT('Ctrl Pts',(1.22531898815164,-1.,4.01728681790024));
#58930=CARTESIAN_POINT('Ctrl Pts',(1.22531898815164,1.,4.01728681790024));
#58931=CARTESIAN_POINT('',(0.963899035118985,1.,3.62400312501199));
#58932=CARTESIAN_POINT('Ctrl Pts',(0.963899035118985,-1.,3.62400312501199));
#58933=CARTESIAN_POINT('Ctrl Pts',(0.963899035118985,-0.666666666666667,
3.62400312501199));
#58934=CARTESIAN_POINT('Ctrl Pts',(0.963899035118985,-0.333333333333333,
3.62400312501199));
#58935=CARTESIAN_POINT('Ctrl Pts',(0.963899035118985,0.333333333333333,
3.62400312501199));
#58936=CARTESIAN_POINT('Ctrl Pts',(0.963899035118985,0.666666666666667,
3.62400312501199));
#58937=CARTESIAN_POINT('Ctrl Pts',(0.963899035118985,1.,3.62400312501199));
#58938=CARTESIAN_POINT('',(1.22531898815164,1.,4.01728681790024));
#58939=CARTESIAN_POINT('',(1.22531898815164,0.,4.01728681790024));
#58940=CARTESIAN_POINT('Ctrl Pts',(0.963899035118985,1.,3.62400312501199));
#58941=CARTESIAN_POINT('Ctrl Pts',(0.963880158556712,1.,3.62404828878375));
#58942=CARTESIAN_POINT('Ctrl Pts',(0.963861297423578,1.,3.62424461507455));
#58943=CARTESIAN_POINT('Ctrl Pts',(0.963957782642589,1.,3.62489305727516));
#58944=CARTESIAN_POINT('Ctrl Pts',(0.964373850166081,1.,3.62652618145252));
#58945=CARTESIAN_POINT('Ctrl Pts',(0.965395153165715,1.,3.62988252139998));
#58946=CARTESIAN_POINT('Ctrl Pts',(0.967052554540877,1.,3.6349212208096));
#58947=CARTESIAN_POINT('Ctrl Pts',(0.969195124674828,1.,3.64113946505393));
#58948=CARTESIAN_POINT('Ctrl Pts',(0.971722122060277,1.,3.64819756447072));
#58949=CARTESIAN_POINT('Ctrl Pts',(0.974519971354138,1.,3.6557157673487));
#58950=CARTESIAN_POINT('Ctrl Pts',(0.977478312751416,1.,3.66333049637403));
#58951=CARTESIAN_POINT('Ctrl Pts',(0.980505922458494,1.,3.67074983340444));
#58952=CARTESIAN_POINT('Ctrl Pts',(0.983550791470864,1.,3.67782408841876));
#58953=CARTESIAN_POINT('Ctrl Pts',(0.986602639864285,1.,3.6845531792623));
#58954=CARTESIAN_POINT('Ctrl Pts',(0.989676715398858,1.,3.69102682138955));
#58955=CARTESIAN_POINT('Ctrl Pts',(0.992802218332103,1.,3.69738123415696));
#58956=CARTESIAN_POINT('Ctrl Pts',(0.996009819772431,1.,3.70375282282107));
#58957=CARTESIAN_POINT('Ctrl Pts',(0.999317260756344,1.,3.7102243971387));
#58958=CARTESIAN_POINT('Ctrl Pts',(1.00272423396802,1.,3.71680667125047));
#58959=CARTESIAN_POINT('Ctrl Pts',(1.00622000735696,1.,3.72346803750544));
#58960=CARTESIAN_POINT('Ctrl Pts',(1.00978798539491,1.,3.73015276704407));
#58961=CARTESIAN_POINT('Ctrl Pts',(1.01341114319906,1.,3.73680245055747));
#58962=CARTESIAN_POINT('Ctrl Pts',(1.01707794311088,1.,3.74337942504993));
#58963=CARTESIAN_POINT('Ctrl Pts',(1.02078510487439,1.,3.74987777155873));
#58964=CARTESIAN_POINT('Ctrl Pts',(1.02453429444668,1.,3.75631037456224));
#58965=CARTESIAN_POINT('Ctrl Pts',(1.02833014458184,1.,3.76270122291245));
#58966=CARTESIAN_POINT('Ctrl Pts',(1.03217786604919,1.,3.76907609832516));
#58967=CARTESIAN_POINT('Ctrl Pts',(1.03608074678008,1.,3.77545283140427));
#58968=CARTESIAN_POINT('Ctrl Pts',(1.04003862055798,1.,3.7818353500817));
#58969=CARTESIAN_POINT('Ctrl Pts',(1.04404924374422,1.,3.78821910787179));
#58970=CARTESIAN_POINT('Ctrl Pts',(1.04810913267639,1.,3.79459440308786));
#58971=CARTESIAN_POINT('Ctrl Pts',(1.05221457990016,1.,3.80095039790681));
#58972=CARTESIAN_POINT('Ctrl Pts',(1.05636266918644,1.,3.80727913637791));
#58973=CARTESIAN_POINT('Ctrl Pts',(1.06055206187299,1.,3.8135786611749));
#58974=CARTESIAN_POINT('Ctrl Pts',(1.0647824403893,1.,3.81985083953012));
#58975=CARTESIAN_POINT('Ctrl Pts',(1.06905413180359,1.,3.82609989967276));
#58976=CARTESIAN_POINT('Ctrl Pts',(1.07336766633459,1.,3.83233071195144));
#58977=CARTESIAN_POINT('Ctrl Pts',(1.07772335353858,1.,3.83854714117491));
#58978=CARTESIAN_POINT('Ctrl Pts',(1.08212087917991,1.,3.8447504803063));
#58979=CARTESIAN_POINT('Ctrl Pts',(1.08655950846384,1.,3.85094025222713));
#58980=CARTESIAN_POINT('Ctrl Pts',(1.09103825516294,1.,3.85711487933931));
#58981=CARTESIAN_POINT('Ctrl Pts',(1.09555606505013,1.,3.86327241021247));
#58982=CARTESIAN_POINT('Ctrl Pts',(1.10011198761195,1.,3.86941120134849));
#58983=CARTESIAN_POINT('Ctrl Pts',(1.10470536603287,1.,3.87553067187514));
#58984=CARTESIAN_POINT('Ctrl Pts',(1.10933577224008,1.,3.88163105531724));
#58985=CARTESIAN_POINT('Ctrl Pts',(1.11400292434429,1.,3.88771308285171));
#58986=CARTESIAN_POINT('Ctrl Pts',(1.11870660794603,1.,3.89377768340344));
#58987=CARTESIAN_POINT('Ctrl Pts',(1.12344660099043,1.,3.89982569750025));
#58988=CARTESIAN_POINT('Ctrl Pts',(1.12822258281553,1.,3.90585753318737));
#58989=CARTESIAN_POINT('Ctrl Pts',(1.13303414693896,1.,3.91187321145649));
#58990=CARTESIAN_POINT('Ctrl Pts',(1.13788084225554,1.,3.91787251936827));
#58991=CARTESIAN_POINT('Ctrl Pts',(1.14276220561593,1.,3.92385513133997));
#58992=CARTESIAN_POINT('Ctrl Pts',(1.14767779451123,1.,3.92982073294257));
#58993=CARTESIAN_POINT('Ctrl Pts',(1.1526272271632,1.,3.9357691705628));
#58994=CARTESIAN_POINT('Ctrl Pts',(1.15761018340956,1.,3.94170046685203));
#58995=CARTESIAN_POINT('Ctrl Pts',(1.16262637999157,1.,3.94761474780583));
#58996=CARTESIAN_POINT('Ctrl Pts',(1.16767555244438,1.,3.95351219509876));
#58997=CARTESIAN_POINT('Ctrl Pts',(1.17275743590361,1.,3.95939299213276));
#58998=CARTESIAN_POINT('Ctrl Pts',(1.17787174135592,1.,3.96525726358159));
#58999=CARTESIAN_POINT('Ctrl Pts',(1.18301815039831,1.,3.97110505165415));
#59000=CARTESIAN_POINT('Ctrl Pts',(1.18819633715539,1.,3.97693634767754));
#59001=CARTESIAN_POINT('Ctrl Pts',(1.19340598349475,1.,3.98275111052561));
#59002=CARTESIAN_POINT('Ctrl Pts',(1.19864679609566,1.,3.98854928957189));
#59003=CARTESIAN_POINT('Ctrl Pts',(1.20391852375138,1.,3.99433084799666));
#59004=CARTESIAN_POINT('Ctrl Pts',(1.20922097029551,1.,4.00009577950721));
#59005=CARTESIAN_POINT('Ctrl Pts',(1.21455398918133,1.,4.00584409522722));
#59006=CARTESIAN_POINT('Ctrl Pts',(1.21884478244403,1.,4.01042947140789));
#59007=CARTESIAN_POINT('Ctrl Pts',(1.22207656455845,1.,4.01386104433519));
#59008=CARTESIAN_POINT('Ctrl Pts',(1.22423716681317,1.,4.01614544569895));
#59009=CARTESIAN_POINT('Ctrl Pts',(1.22531898815164,1.,4.01728681790024));
#59010=CARTESIAN_POINT('Origin',(1.22531898815164,0.,4.01728681790024));
#59011=CARTESIAN_POINT('',(1.36999806084572,1.,3.97027773754922));
#59012=CARTESIAN_POINT('Origin',(0.,0.,0.));
#59013=CARTESIAN_POINT('',(0.786422660833742,1.,3.66661143271648));
#59014=CARTESIAN_POINT('Origin',(0.,1.,0.));
#59015=CARTESIAN_POINT('Ctrl Pts',(0.786422660833742,1.,3.66661143271648));
#59016=CARTESIAN_POINT('Ctrl Pts',(0.786422660833742,0.666666666666667,
3.66661143271648));
#59017=CARTESIAN_POINT('Ctrl Pts',(0.786422660833742,0.333333333333333,
3.66661143271648));
#59018=CARTESIAN_POINT('Ctrl Pts',(0.786422660833742,-0.333333333333333,
3.66661143271648));
#59019=CARTESIAN_POINT('Ctrl Pts',(0.786422660833742,-0.666666666666667,
3.66661143271648));
#59020=CARTESIAN_POINT('Ctrl Pts',(0.786422660833742,-1.,3.66661143271648));
#59021=CARTESIAN_POINT('Ctrl Pts',(0.732042837400619,-1.,4.13571194405636));
#59022=CARTESIAN_POINT('Ctrl Pts',(0.732042837400619,1.,4.13571194405636));
#59023=CARTESIAN_POINT('Ctrl Pts',(0.732488575135925,-1.,4.13420383737278));
#59024=CARTESIAN_POINT('Ctrl Pts',(0.732488575135925,1.,4.13420383737278));
#59025=CARTESIAN_POINT('Ctrl Pts',(0.733376589325634,-1.,4.13118752796397));
#59026=CARTESIAN_POINT('Ctrl Pts',(0.733376589325634,1.,4.13118752796397));
#59027=CARTESIAN_POINT('Ctrl Pts',(0.734698226767512,-1.,4.12666277572794));
#59028=CARTESIAN_POINT('Ctrl Pts',(0.734698226767512,1.,4.12666277572794));
#59029=CARTESIAN_POINT('Ctrl Pts',(0.736439634335347,-1.,4.12062919626082));
#59030=CARTESIAN_POINT('Ctrl Pts',(0.736439634335347,1.,4.12062919626082));
#59031=CARTESIAN_POINT('Ctrl Pts',(0.738581708229118,-1.,4.11308626953795));
#59032=CARTESIAN_POINT('Ctrl Pts',(0.738581708229118,1.,4.11308626953795));
#59033=CARTESIAN_POINT('Ctrl Pts',(0.740688998555151,-1.,4.1055424175856));
#59034=CARTESIAN_POINT('Ctrl Pts',(0.740688998555151,1.,4.1055424175856));
#59035=CARTESIAN_POINT('Ctrl Pts',(0.742761369690017,-1.,4.09799769702712));
#59036=CARTESIAN_POINT('Ctrl Pts',(0.742761369690017,1.,4.09799769702712));
#59037=CARTESIAN_POINT('Ctrl Pts',(0.744798649705513,-1.,4.09045220253011));
#59038=CARTESIAN_POINT('Ctrl Pts',(0.744798649705513,1.,4.09045220253011));
#59039=CARTESIAN_POINT('Ctrl Pts',(0.746800631490821,-1.,4.08290608094789));
#59040=CARTESIAN_POINT('Ctrl Pts',(0.746800631490821,1.,4.08290608094789));
#59041=CARTESIAN_POINT('Ctrl Pts',(0.748767076679176,-1.,4.07535951055363));
#59042=CARTESIAN_POINT('Ctrl Pts',(0.748767076679176,1.,4.07535951055363));
#59043=CARTESIAN_POINT('Ctrl Pts',(0.750697720483175,-1.,4.06781267241886));
#59044=CARTESIAN_POINT('Ctrl Pts',(0.750697720483175,1.,4.06781267241886));
#59045=CARTESIAN_POINT('Ctrl Pts',(0.752592276482868,-1.,4.06026572221399));
#59046=CARTESIAN_POINT('Ctrl Pts',(0.752592276482868,1.,4.06026572221399));
#59047=CARTESIAN_POINT('Ctrl Pts',(0.754450441816411,-1.,4.05271876688106));
#59048=CARTESIAN_POINT('Ctrl Pts',(0.754450441816411,1.,4.05271876688106));
#59049=CARTESIAN_POINT('Ctrl Pts',(0.756271902370186,-1.,4.04517182654344));
#59050=CARTESIAN_POINT('Ctrl Pts',(0.756271902370186,1.,4.04517182654344));
#59051=CARTESIAN_POINT('Ctrl Pts',(0.758056338885553,-1.,4.03762485803468));
#59052=CARTESIAN_POINT('Ctrl Pts',(0.758056338885553,1.,4.03762485803468));
#59053=CARTESIAN_POINT('Ctrl Pts',(0.759803433244165,-1.,4.0300778195465));
#59054=CARTESIAN_POINT('Ctrl Pts',(0.759803433244165,1.,4.0300778195465));
#59055=CARTESIAN_POINT('Ctrl Pts',(0.761512875859941,-1.,4.02253072741347));
#59056=CARTESIAN_POINT('Ctrl Pts',(0.761512875859941,1.,4.02253072741347));
#59057=CARTESIAN_POINT('Ctrl Pts',(0.763184371182826,-1.,4.01498370680434));
#59058=CARTESIAN_POINT('Ctrl Pts',(0.763184371182826,1.,4.01498370680434));
#59059=CARTESIAN_POINT('Ctrl Pts',(0.764817648784946,-1.,4.00743706791366));
#59060=CARTESIAN_POINT('Ctrl Pts',(0.764817648784946,1.,4.00743706791366));
#59061=CARTESIAN_POINT('Ctrl Pts',(0.766412457135785,-1.,3.99989129179464));
#59062=CARTESIAN_POINT('Ctrl Pts',(0.766412457135785,1.,3.99989129179464));
#59063=CARTESIAN_POINT('Ctrl Pts',(0.767968531377707,-1.,3.99234687880892));
#59064=CARTESIAN_POINT('Ctrl Pts',(0.767968531377707,1.,3.99234687880892));
#59065=CARTESIAN_POINT('Ctrl Pts',(0.769485566245459,-1.,3.98480422348403));
#59066=CARTESIAN_POINT('Ctrl Pts',(0.769485566245459,1.,3.98480422348403));
#59067=CARTESIAN_POINT('Ctrl Pts',(0.770963190030503,-1.,3.97726349165507));
#59068=CARTESIAN_POINT('Ctrl Pts',(0.770963190030503,1.,3.97726349165507));
#59069=CARTESIAN_POINT('Ctrl Pts',(0.772400931772238,-1.,3.96972446532832));
#59070=CARTESIAN_POINT('Ctrl Pts',(0.772400931772238,1.,3.96972446532832));
#59071=CARTESIAN_POINT('Ctrl Pts',(0.773798212026682,-1.,3.96218649639876));
#59072=CARTESIAN_POINT('Ctrl Pts',(0.773798212026682,1.,3.96218649639876));
#59073=CARTESIAN_POINT('Ctrl Pts',(0.775154418039441,-1.,3.95464885452364));
#59074=CARTESIAN_POINT('Ctrl Pts',(0.775154418039441,1.,3.95464885452364));
#59075=CARTESIAN_POINT('Ctrl Pts',(0.776468966697959,-1.,3.94711101619471));
#59076=CARTESIAN_POINT('Ctrl Pts',(0.776468966697959,1.,3.94711101619471));
#59077=CARTESIAN_POINT('Ctrl Pts',(0.777741370568549,-1.,3.93957296768098));
#59078=CARTESIAN_POINT('Ctrl Pts',(0.777741370568549,1.,3.93957296768098));
#59079=CARTESIAN_POINT('Ctrl Pts',(0.778971308134786,-1.,3.93203552473153));
#59080=CARTESIAN_POINT('Ctrl Pts',(0.778971308134786,1.,3.93203552473153));
#59081=CARTESIAN_POINT('Ctrl Pts',(0.780158678615506,-1.,3.92450058323799));
#59082=CARTESIAN_POINT('Ctrl Pts',(0.780158678615506,1.,3.92450058323799));
#59083=CARTESIAN_POINT('Ctrl Pts',(0.781303428618343,-1.,3.9169703605466));
#59084=CARTESIAN_POINT('Ctrl Pts',(0.781303428618343,1.,3.9169703605466));
#59085=CARTESIAN_POINT('Ctrl Pts',(0.782405395622758,-1.,3.90944671004536));
#59086=CARTESIAN_POINT('Ctrl Pts',(0.782405395622758,1.,3.90944671004536));
#59087=CARTESIAN_POINT('Ctrl Pts',(0.783464141529082,-1.,3.90193039043971));
#59088=CARTESIAN_POINT('Ctrl Pts',(0.783464141529082,1.,3.90193039043971));
#59089=CARTESIAN_POINT('Ctrl Pts',(0.784478799358335,-1.,3.89442039235105));
#59090=CARTESIAN_POINT('Ctrl Pts',(0.784478799358335,1.,3.89442039235105));
#59091=CARTESIAN_POINT('Ctrl Pts',(0.785447890340723,-1.,3.88691313167399));
#59092=CARTESIAN_POINT('Ctrl Pts',(0.785447890340723,1.,3.88691313167399));
#59093=CARTESIAN_POINT('Ctrl Pts',(0.786369675812591,-1.,3.87940402818186));
#59094=CARTESIAN_POINT('Ctrl Pts',(0.786369675812591,1.,3.87940402818186));
#59095=CARTESIAN_POINT('Ctrl Pts',(0.78724252761798,-1.,3.87188916600905));
#59096=CARTESIAN_POINT('Ctrl Pts',(0.78724252761798,1.,3.87188916600905));
#59097=CARTESIAN_POINT('Ctrl Pts',(0.78806531509377,-1.,3.86436702561342));
#59098=CARTESIAN_POINT('Ctrl Pts',(0.78806531509377,1.,3.86436702561342));
#59099=CARTESIAN_POINT('Ctrl Pts',(0.788837734090688,-1.,3.85683995872536));
#59100=CARTESIAN_POINT('Ctrl Pts',(0.788837734090688,1.,3.85683995872536));
#59101=CARTESIAN_POINT('Ctrl Pts',(0.789560798155618,-1.,3.8493163780891));
#59102=CARTESIAN_POINT('Ctrl Pts',(0.789560798155618,1.,3.8493163780891));
#59103=CARTESIAN_POINT('Ctrl Pts',(0.790236124191289,-1.,3.84180762342476));
#59104=CARTESIAN_POINT('Ctrl Pts',(0.790236124191289,1.,3.84180762342476));
#59105=CARTESIAN_POINT('Ctrl Pts',(0.790865012705339,-1.,3.83432392054804));
#59106=CARTESIAN_POINT('Ctrl Pts',(0.790865012705339,1.,3.83432392054804));
#59107=CARTESIAN_POINT('Ctrl Pts',(0.791447528662381,-1.,3.82687033899799));
#59108=CARTESIAN_POINT('Ctrl Pts',(0.791447528662381,1.,3.82687033899799));
#59109=CARTESIAN_POINT('Ctrl Pts',(0.791981740718606,-1.,3.81944345442237));
#59110=CARTESIAN_POINT('Ctrl Pts',(0.791981740718606,1.,3.81944345442237));
#59111=CARTESIAN_POINT('Ctrl Pts',(0.792462483517568,-1.,3.81202588694726));
#59112=CARTESIAN_POINT('Ctrl Pts',(0.792462483517568,1.,3.81202588694726));
#59113=CARTESIAN_POINT('Ctrl Pts',(0.792882695234692,-1.,3.80459229925598));
#59114=CARTESIAN_POINT('Ctrl Pts',(0.792882695234692,1.,3.80459229925598));
#59115=CARTESIAN_POINT('Ctrl Pts',(0.7932356129732,-1.,3.79711921389862));
#59116=CARTESIAN_POINT('Ctrl Pts',(0.7932356129732,1.,3.79711921389862));
#59117=CARTESIAN_POINT('Ctrl Pts',(0.793516871680965,-1.,3.78959439439222));
#59118=CARTESIAN_POINT('Ctrl Pts',(0.793516871680965,1.,3.78959439439222));
#59119=CARTESIAN_POINT('Ctrl Pts',(0.793726235781339,-1.,3.78202460377617));
#59120=CARTESIAN_POINT('Ctrl Pts',(0.793726235781339,1.,3.78202460377617));
#59121=CARTESIAN_POINT('Ctrl Pts',(0.793870523787515,-1.,3.77444863801264));
#59122=CARTESIAN_POINT('Ctrl Pts',(0.793870523787515,1.,3.77444863801264));
#59123=CARTESIAN_POINT('Ctrl Pts',(0.793961083689141,-1.,3.76692626931184));
#59124=CARTESIAN_POINT('Ctrl Pts',(0.793961083689141,1.,3.76692626931184));
#59125=CARTESIAN_POINT('Ctrl Pts',(0.794008429135046,-1.,3.75951468666325));
#59126=CARTESIAN_POINT('Ctrl Pts',(0.794008429135046,1.,3.75951468666325));
#59127=CARTESIAN_POINT('Ctrl Pts',(0.79401734737144,-1.,3.75224692493895));
#59128=CARTESIAN_POINT('Ctrl Pts',(0.79401734737144,1.,3.75224692493895));
#59129=CARTESIAN_POINT('Ctrl Pts',(0.79398270045988,-1.,3.74511357728827));
#59130=CARTESIAN_POINT('Ctrl Pts',(0.79398270045988,1.,3.74511357728827));
#59131=CARTESIAN_POINT('Ctrl Pts',(0.79388270093679,-1.,3.73803280541576));
#59132=CARTESIAN_POINT('Ctrl Pts',(0.79388270093679,1.,3.73803280541576));
#59133=CARTESIAN_POINT('Ctrl Pts',(0.793682750269347,-1.,3.7308691469564));
#59134=CARTESIAN_POINT('Ctrl Pts',(0.793682750269347,1.,3.7308691469564));
#59135=CARTESIAN_POINT('Ctrl Pts',(0.79334702378387,-1.,3.7234879729357));
#59136=CARTESIAN_POINT('Ctrl Pts',(0.79334702378387,1.,3.7234879729357));
#59137=CARTESIAN_POINT('Ctrl Pts',(0.792848377370115,-1.,3.7158024239604));
#59138=CARTESIAN_POINT('Ctrl Pts',(0.792848377370115,1.,3.7158024239604));
#59139=CARTESIAN_POINT('Ctrl Pts',(0.792177688845967,-1.,3.70781724021879));
#59140=CARTESIAN_POINT('Ctrl Pts',(0.792177688845967,1.,3.70781724021879));
#59141=CARTESIAN_POINT('Ctrl Pts',(0.791356575696508,-1.,3.69968940808982));
#59142=CARTESIAN_POINT('Ctrl Pts',(0.791356575696508,1.,3.69968940808982));
#59143=CARTESIAN_POINT('Ctrl Pts',(0.790436284989579,-1.,3.69172044327754));
#59144=CARTESIAN_POINT('Ctrl Pts',(0.790436284989579,1.,3.69172044327754));
#59145=CARTESIAN_POINT('Ctrl Pts',(0.789483546065158,-1.,3.68428439784285));
#59146=CARTESIAN_POINT('Ctrl Pts',(0.789483546065158,1.,3.68428439784285));
#59147=CARTESIAN_POINT('Ctrl Pts',(0.788569566220662,-1.,3.67777119516438));
#59148=CARTESIAN_POINT('Ctrl Pts',(0.788569566220662,1.,3.67777119516438));
#59149=CARTESIAN_POINT('Ctrl Pts',(0.787758799995426,-1.,3.672529236635));
#59150=CARTESIAN_POINT('Ctrl Pts',(0.787758799995426,1.,3.672529236635));
#59151=CARTESIAN_POINT('Ctrl Pts',(0.787095252589507,-1.,3.66879484800625));
#59152=CARTESIAN_POINT('Ctrl Pts',(0.787095252589507,1.,3.66879484800625));
#59153=CARTESIAN_POINT('Ctrl Pts',(0.786698783541657,-1.,3.66710211819938));
#59154=CARTESIAN_POINT('Ctrl Pts',(0.786698783541657,1.,3.66710211819938));
#59155=CARTESIAN_POINT('Ctrl Pts',(0.786480236184947,-1.,3.66657784454965));
#59156=CARTESIAN_POINT('Ctrl Pts',(0.786480236184947,1.,3.66657784454965));
#59157=CARTESIAN_POINT('Ctrl Pts',(0.786369528183039,-1.,3.66655932661846));
#59158=CARTESIAN_POINT('Ctrl Pts',(0.786369528183039,1.,3.66655932661846));
#59159=CARTESIAN_POINT('Ctrl Pts',(0.786322922920599,-1.,3.66663282329846));
#59160=CARTESIAN_POINT('Ctrl Pts',(0.786322922920599,1.,3.66663282329846));
#59161=CARTESIAN_POINT('',(0.732042837400619,1.,4.13571194405636));
#59162=CARTESIAN_POINT('Ctrl Pts',(0.732042837400619,1.,4.13571194405636));
#59163=CARTESIAN_POINT('Ctrl Pts',(0.732488575135925,1.,4.13420383737278));
#59164=CARTESIAN_POINT('Ctrl Pts',(0.733376589325634,1.,4.13118752796397));
#59165=CARTESIAN_POINT('Ctrl Pts',(0.734698226767512,1.,4.12666277572794));
#59166=CARTESIAN_POINT('Ctrl Pts',(0.736439634335347,1.,4.12062919626082));
#59167=CARTESIAN_POINT('Ctrl Pts',(0.738581708229118,1.,4.11308626953795));
#59168=CARTESIAN_POINT('Ctrl Pts',(0.740688998555151,1.,4.1055424175856));
#59169=CARTESIAN_POINT('Ctrl Pts',(0.742761369690017,1.,4.09799769702712));
#59170=CARTESIAN_POINT('Ctrl Pts',(0.744798649705513,1.,4.09045220253011));
#59171=CARTESIAN_POINT('Ctrl Pts',(0.746800631490821,1.,4.08290608094789));
#59172=CARTESIAN_POINT('Ctrl Pts',(0.748767076679176,1.,4.07535951055363));
#59173=CARTESIAN_POINT('Ctrl Pts',(0.750697720483175,1.,4.06781267241886));
#59174=CARTESIAN_POINT('Ctrl Pts',(0.752592276482868,1.,4.06026572221399));
#59175=CARTESIAN_POINT('Ctrl Pts',(0.754450441816411,1.,4.05271876688106));
#59176=CARTESIAN_POINT('Ctrl Pts',(0.756271902370186,1.,4.04517182654344));
#59177=CARTESIAN_POINT('Ctrl Pts',(0.758056338885553,1.,4.03762485803468));
#59178=CARTESIAN_POINT('Ctrl Pts',(0.759803433244165,1.,4.0300778195465));
#59179=CARTESIAN_POINT('Ctrl Pts',(0.761512875859941,1.,4.02253072741347));
#59180=CARTESIAN_POINT('Ctrl Pts',(0.763184371182826,1.,4.01498370680434));
#59181=CARTESIAN_POINT('Ctrl Pts',(0.764817648784946,1.,4.00743706791366));
#59182=CARTESIAN_POINT('Ctrl Pts',(0.766412457135785,1.,3.99989129179464));
#59183=CARTESIAN_POINT('Ctrl Pts',(0.767968531377707,1.,3.99234687880892));
#59184=CARTESIAN_POINT('Ctrl Pts',(0.769485566245459,1.,3.98480422348403));
#59185=CARTESIAN_POINT('Ctrl Pts',(0.770963190030503,1.,3.97726349165507));
#59186=CARTESIAN_POINT('Ctrl Pts',(0.772400931772238,1.,3.96972446532832));
#59187=CARTESIAN_POINT('Ctrl Pts',(0.773798212026682,1.,3.96218649639876));
#59188=CARTESIAN_POINT('Ctrl Pts',(0.775154418039441,1.,3.95464885452364));
#59189=CARTESIAN_POINT('Ctrl Pts',(0.776468966697959,1.,3.94711101619471));
#59190=CARTESIAN_POINT('Ctrl Pts',(0.777741370568549,1.,3.93957296768098));
#59191=CARTESIAN_POINT('Ctrl Pts',(0.778971308134786,1.,3.93203552473153));
#59192=CARTESIAN_POINT('Ctrl Pts',(0.780158678615506,1.,3.92450058323799));
#59193=CARTESIAN_POINT('Ctrl Pts',(0.781303428618343,1.,3.9169703605466));
#59194=CARTESIAN_POINT('Ctrl Pts',(0.782405395622758,1.,3.90944671004536));
#59195=CARTESIAN_POINT('Ctrl Pts',(0.783464141529082,1.,3.90193039043971));
#59196=CARTESIAN_POINT('Ctrl Pts',(0.784478799358335,1.,3.89442039235105));
#59197=CARTESIAN_POINT('Ctrl Pts',(0.785447890340723,1.,3.88691313167399));
#59198=CARTESIAN_POINT('Ctrl Pts',(0.786369675812591,1.,3.87940402818186));
#59199=CARTESIAN_POINT('Ctrl Pts',(0.78724252761798,1.,3.87188916600905));
#59200=CARTESIAN_POINT('Ctrl Pts',(0.78806531509377,1.,3.86436702561342));
#59201=CARTESIAN_POINT('Ctrl Pts',(0.788837734090688,1.,3.85683995872536));
#59202=CARTESIAN_POINT('Ctrl Pts',(0.789560798155618,1.,3.8493163780891));
#59203=CARTESIAN_POINT('Ctrl Pts',(0.790236124191289,1.,3.84180762342476));
#59204=CARTESIAN_POINT('Ctrl Pts',(0.790865012705339,1.,3.83432392054804));
#59205=CARTESIAN_POINT('Ctrl Pts',(0.791447528662381,1.,3.82687033899799));
#59206=CARTESIAN_POINT('Ctrl Pts',(0.791981740718606,1.,3.81944345442237));
#59207=CARTESIAN_POINT('Ctrl Pts',(0.792462483517568,1.,3.81202588694726));
#59208=CARTESIAN_POINT('Ctrl Pts',(0.792882695234692,1.,3.80459229925598));
#59209=CARTESIAN_POINT('Ctrl Pts',(0.7932356129732,1.,3.79711921389862));
#59210=CARTESIAN_POINT('Ctrl Pts',(0.793516871680965,1.,3.78959439439222));
#59211=CARTESIAN_POINT('Ctrl Pts',(0.793726235781339,1.,3.78202460377617));
#59212=CARTESIAN_POINT('Ctrl Pts',(0.793870523787515,1.,3.77444863801264));
#59213=CARTESIAN_POINT('Ctrl Pts',(0.793961083689141,1.,3.76692626931184));
#59214=CARTESIAN_POINT('Ctrl Pts',(0.794008429135046,1.,3.75951468666325));
#59215=CARTESIAN_POINT('Ctrl Pts',(0.79401734737144,1.,3.75224692493895));
#59216=CARTESIAN_POINT('Ctrl Pts',(0.79398270045988,1.,3.74511357728827));
#59217=CARTESIAN_POINT('Ctrl Pts',(0.79388270093679,1.,3.73803280541576));
#59218=CARTESIAN_POINT('Ctrl Pts',(0.793682750269347,1.,3.7308691469564));
#59219=CARTESIAN_POINT('Ctrl Pts',(0.79334702378387,1.,3.7234879729357));
#59220=CARTESIAN_POINT('Ctrl Pts',(0.792848377370115,1.,3.7158024239604));
#59221=CARTESIAN_POINT('Ctrl Pts',(0.792177688845967,1.,3.70781724021879));
#59222=CARTESIAN_POINT('Ctrl Pts',(0.791356575696508,1.,3.69968940808982));
#59223=CARTESIAN_POINT('Ctrl Pts',(0.790436284989579,1.,3.69172044327754));
#59224=CARTESIAN_POINT('Ctrl Pts',(0.789483546065158,1.,3.68428439784285));
#59225=CARTESIAN_POINT('Ctrl Pts',(0.788569566220662,1.,3.67777119516438));
#59226=CARTESIAN_POINT('Ctrl Pts',(0.787758799995426,1.,3.672529236635));
#59227=CARTESIAN_POINT('Ctrl Pts',(0.787145041181588,1.,3.66907505398769));
#59228=CARTESIAN_POINT('Ctrl Pts',(0.786774337198499,1.,3.66743103898844));
#59229=CARTESIAN_POINT('Ctrl Pts',(0.786565919559889,1.,3.66680946938396));
#59230=CARTESIAN_POINT('Ctrl Pts',(0.786459983896781,1.,3.66664310415236));
#59231=CARTESIAN_POINT('Ctrl Pts',(0.786422660833743,1.,3.66661143271648));
#59232=CARTESIAN_POINT('',(0.732042837400619,0.,4.13571194405636));
#59233=CARTESIAN_POINT('Ctrl Pts',(0.385214314776328,-1.,3.73016218570874));
#59234=CARTESIAN_POINT('Ctrl Pts',(0.385214314776328,1.,3.73016218570874));
#59235=CARTESIAN_POINT('Ctrl Pts',(0.385147278814803,-1.,3.73010668803185));
#59236=CARTESIAN_POINT('Ctrl Pts',(0.385147278814803,1.,3.73010668803185));
#59237=CARTESIAN_POINT('Ctrl Pts',(0.385047711603887,-1.,3.73015851028729));
#59238=CARTESIAN_POINT('Ctrl Pts',(0.385047711603887,1.,3.73015851028729));
#59239=CARTESIAN_POINT('Ctrl Pts',(0.385001870183841,-1.,3.73072465900727));
#59240=CARTESIAN_POINT('Ctrl Pts',(0.385001870183841,1.,3.73072465900727));
#59241=CARTESIAN_POINT('Ctrl Pts',(0.385147887989514,-1.,3.73245705639337));
#59242=CARTESIAN_POINT('Ctrl Pts',(0.385147887989514,1.,3.73245705639337));
#59243=CARTESIAN_POINT('Ctrl Pts',(0.385670806454744,-1.,3.73621371845475));
#59244=CARTESIAN_POINT('Ctrl Pts',(0.385670806454744,1.,3.73621371845475));
#59245=CARTESIAN_POINT('Ctrl Pts',(0.386519576222035,-1.,3.74144965781088));
#59246=CARTESIAN_POINT('Ctrl Pts',(0.386519576222035,1.,3.74144965781088));
#59247=CARTESIAN_POINT('Ctrl Pts',(0.387663020050396,-1.,3.74792651696269));
#59248=CARTESIAN_POINT('Ctrl Pts',(0.387663020050396,1.,3.74792651696269));
#59249=CARTESIAN_POINT('Ctrl Pts',(0.38905477589825,-1.,3.75529302894757));
#59250=CARTESIAN_POINT('Ctrl Pts',(0.38905477589825,1.,3.75529302894757));
#59251=CARTESIAN_POINT('Ctrl Pts',(0.390642072979258,-1.,3.76315635032993));
#59252=CARTESIAN_POINT('Ctrl Pts',(0.390642072979258,1.,3.76315635032993));
#59253=CARTESIAN_POINT('Ctrl Pts',(0.392372786223346,-1.,3.77114011595892));
#59254=CARTESIAN_POINT('Ctrl Pts',(0.392372786223346,1.,3.77114011595892));
#59255=CARTESIAN_POINT('Ctrl Pts',(0.394202481011595,-1.,3.77894173114368));
#59256=CARTESIAN_POINT('Ctrl Pts',(0.394202481011595,1.,3.77894173114368));
#59257=CARTESIAN_POINT('Ctrl Pts',(0.396103205335028,-1.,3.78640521279479));
#59258=CARTESIAN_POINT('Ctrl Pts',(0.396103205335028,1.,3.78640521279479));
#59259=CARTESIAN_POINT('Ctrl Pts',(0.398064818684158,-1.,3.79352887163457));
#59260=CARTESIAN_POINT('Ctrl Pts',(0.398064818684158,1.,3.79352887163457));
#59261=CARTESIAN_POINT('Ctrl Pts',(0.400088346504726,-1.,3.80040370384659));
#59262=CARTESIAN_POINT('Ctrl Pts',(0.400088346504726,1.,3.80040370384659));
#59263=CARTESIAN_POINT('Ctrl Pts',(0.402181320148474,-1.,3.80716881962763));
#59264=CARTESIAN_POINT('Ctrl Pts',(0.402181320148474,1.,3.80716881962763));
#59265=CARTESIAN_POINT('Ctrl Pts',(0.404352694628236,-1.,3.81396374287762));
#59266=CARTESIAN_POINT('Ctrl Pts',(0.404352694628236,1.,3.81396374287762));
#59267=CARTESIAN_POINT('Ctrl Pts',(0.406607038258906,-1.,3.82087303913741));
#59268=CARTESIAN_POINT('Ctrl Pts',(0.406607038258906,1.,3.82087303913741));
#59269=CARTESIAN_POINT('Ctrl Pts',(0.408942371447376,-1.,3.82790724256397));
#59270=CARTESIAN_POINT('Ctrl Pts',(0.408942371447376,1.,3.82790724256397));
#59271=CARTESIAN_POINT('Ctrl Pts',(0.411353038798459,-1.,3.83503345578645));
#59272=CARTESIAN_POINT('Ctrl Pts',(0.411353038798459,1.,3.83503345578645));
#59273=CARTESIAN_POINT('Ctrl Pts',(0.413831367016726,-1.,3.84219403994742));
#59274=CARTESIAN_POINT('Ctrl Pts',(0.413831367016726,1.,3.84219403994742));
#59275=CARTESIAN_POINT('Ctrl Pts',(0.41636967805292,-1.,3.8493286415751));
#59276=CARTESIAN_POINT('Ctrl Pts',(0.41636967805292,1.,3.8493286415751));
#59277=CARTESIAN_POINT('Ctrl Pts',(0.418962468086809,-1.,3.85639825648031));
#59278=CARTESIAN_POINT('Ctrl Pts',(0.418962468086809,1.,3.85639825648031));
#59279=CARTESIAN_POINT('Ctrl Pts',(0.421607423177575,-1.,3.86339652542749));
#59280=CARTESIAN_POINT('Ctrl Pts',(0.421607423177575,1.,3.86339652542749));
#59281=CARTESIAN_POINT('Ctrl Pts',(0.424304173195142,-1.,3.87033643487882));
#59282=CARTESIAN_POINT('Ctrl Pts',(0.424304173195142,1.,3.87033643487882));
#59283=CARTESIAN_POINT('Ctrl Pts',(0.427053541173469,-1.,3.87724240306609));
#59284=CARTESIAN_POINT('Ctrl Pts',(0.427053541173469,1.,3.87724240306609));
#59285=CARTESIAN_POINT('Ctrl Pts',(0.429856640579733,-1.,3.88414070943334));
#59286=CARTESIAN_POINT('Ctrl Pts',(0.429856640579733,1.,3.88414070943334));
#59287=CARTESIAN_POINT('Ctrl Pts',(0.432713929544439,-1.,3.89104947940592));
#59288=CARTESIAN_POINT('Ctrl Pts',(0.432713929544439,1.,3.89104947940592));
#59289=CARTESIAN_POINT('Ctrl Pts',(0.435624629433505,-1.,3.8979725665544));
#59290=CARTESIAN_POINT('Ctrl Pts',(0.435624629433505,1.,3.8979725665544));
#59291=CARTESIAN_POINT('Ctrl Pts',(0.438587235458233,-1.,3.90490512938546));
#59292=CARTESIAN_POINT('Ctrl Pts',(0.438587235458233,1.,3.90490512938546));
#59293=CARTESIAN_POINT('Ctrl Pts',(0.441599824524047,-1.,3.91183704069146));
#59294=CARTESIAN_POINT('Ctrl Pts',(0.441599824524047,1.,3.91183704069146));
#59295=CARTESIAN_POINT('Ctrl Pts',(0.444660430230592,-1.,3.91875701610721));
#59296=CARTESIAN_POINT('Ctrl Pts',(0.444660430230592,1.,3.91875701610721));
#59297=CARTESIAN_POINT('Ctrl Pts',(0.447767416837296,-1.,3.92565674143424));
#59298=CARTESIAN_POINT('Ctrl Pts',(0.447767416837296,1.,3.92565674143424));
#59299=CARTESIAN_POINT('Ctrl Pts',(0.450919768356346,-1.,3.93253407403128));
#59300=CARTESIAN_POINT('Ctrl Pts',(0.450919768356346,1.,3.93253407403128));
#59301=CARTESIAN_POINT('Ctrl Pts',(0.454116879027575,-1.,3.93939080846298));
#59302=CARTESIAN_POINT('Ctrl Pts',(0.454116879027575,1.,3.93939080846298));
#59303=CARTESIAN_POINT('Ctrl Pts',(0.457358410451673,-1.,3.94623117206675));
#59304=CARTESIAN_POINT('Ctrl Pts',(0.457358410451673,1.,3.94623117206675));
#59305=CARTESIAN_POINT('Ctrl Pts',(0.460644124429119,-1.,3.95306005817363));
#59306=CARTESIAN_POINT('Ctrl Pts',(0.460644124429119,1.,3.95306005817363));
#59307=CARTESIAN_POINT('Ctrl Pts',(0.463973722115744,-1.,3.95988133243543));
#59308=CARTESIAN_POINT('Ctrl Pts',(0.463973722115744,1.,3.95988133243543));
#59309=CARTESIAN_POINT('Ctrl Pts',(0.467346690880671,-1.,3.96669622273946));
#59310=CARTESIAN_POINT('Ctrl Pts',(0.467346690880671,1.,3.96669622273946));
#59311=CARTESIAN_POINT('Ctrl Pts',(0.470762379613477,-1.,3.97350414289415));
#59312=CARTESIAN_POINT('Ctrl Pts',(0.470762379613477,1.,3.97350414289415));
#59313=CARTESIAN_POINT('Ctrl Pts',(0.474220061019542,-1.,3.9803033804443));
#59314=CARTESIAN_POINT('Ctrl Pts',(0.474220061019542,1.,3.9803033804443));
#59315=CARTESIAN_POINT('Ctrl Pts',(0.477718999122033,-1.,3.98709184306743));
#59316=CARTESIAN_POINT('Ctrl Pts',(0.477718999122033,1.,3.98709184306743));
#59317=CARTESIAN_POINT('Ctrl Pts',(0.481258512209637,-1.,3.99386775880655));
#59318=CARTESIAN_POINT('Ctrl Pts',(0.481258512209637,1.,3.99386775880655));
#59319=CARTESIAN_POINT('Ctrl Pts',(0.484838042421754,-1.,4.00063045119234));
#59320=CARTESIAN_POINT('Ctrl Pts',(0.484838042421754,1.,4.00063045119234));
#59321=CARTESIAN_POINT('Ctrl Pts',(0.48845713042453,-1.,4.0073800839092));
#59322=CARTESIAN_POINT('Ctrl Pts',(0.48845713042453,1.,4.0073800839092));
#59323=CARTESIAN_POINT('Ctrl Pts',(0.49211538341793,-1.,4.01411733503486));
#59324=CARTESIAN_POINT('Ctrl Pts',(0.49211538341793,1.,4.01411733503486));
#59325=CARTESIAN_POINT('Ctrl Pts',(0.495812444326222,-1.,4.02084308851813));
#59326=CARTESIAN_POINT('Ctrl Pts',(0.495812444326222,1.,4.02084308851813));
#59327=CARTESIAN_POINT('Ctrl Pts',(0.499547962340889,-1.,4.0275581398015));
#59328=CARTESIAN_POINT('Ctrl Pts',(0.499547962340889,1.,4.0275581398015));
#59329=CARTESIAN_POINT('Ctrl Pts',(0.503321556915513,-1.,4.0342628417439));
#59330=CARTESIAN_POINT('Ctrl Pts',(0.503321556915513,1.,4.0342628417439));
#59331=CARTESIAN_POINT('Ctrl Pts',(0.507132823288361,-1.,4.04095715149074));
#59332=CARTESIAN_POINT('Ctrl Pts',(0.507132823288361,1.,4.04095715149074));
#59333=CARTESIAN_POINT('Ctrl Pts',(0.510981349219173,-1.,4.04764078815591));
#59334=CARTESIAN_POINT('Ctrl Pts',(0.510981349219173,1.,4.04764078815591));
#59335=CARTESIAN_POINT('Ctrl Pts',(0.514866728193103,-1.,4.05431335771261));
#59336=CARTESIAN_POINT('Ctrl Pts',(0.514866728193103,1.,4.05431335771261));
#59337=CARTESIAN_POINT('Ctrl Pts',(0.518788572336809,-1.,4.06097448037934));
#59338=CARTESIAN_POINT('Ctrl Pts',(0.518788572336809,1.,4.06097448037934));
#59339=CARTESIAN_POINT('Ctrl Pts',(0.522746528602767,-1.,4.06762394471075));
#59340=CARTESIAN_POINT('Ctrl Pts',(0.522746528602767,1.,4.06762394471075));
#59341=CARTESIAN_POINT('Ctrl Pts',(0.526740277226999,-1.,4.07426172299496));
#59342=CARTESIAN_POINT('Ctrl Pts',(0.526740277226999,1.,4.07426172299496));
#59343=CARTESIAN_POINT('Ctrl Pts',(0.530769518728075,-1.,4.08088789536488));
#59344=CARTESIAN_POINT('Ctrl Pts',(0.530769518728075,1.,4.08088789536488));
#59345=CARTESIAN_POINT('Ctrl Pts',(0.534833963476999,-1.,4.08750259988693));
#59346=CARTESIAN_POINT('Ctrl Pts',(0.534833963476999,1.,4.08750259988693));
#59347=CARTESIAN_POINT('Ctrl Pts',(0.53893332117992,-1.,4.09410597627116));
#59348=CARTESIAN_POINT('Ctrl Pts',(0.53893332117992,1.,4.09410597627116));
#59349=CARTESIAN_POINT('Ctrl Pts',(0.543067286878457,-1.,4.10069810244473));
#59350=CARTESIAN_POINT('Ctrl Pts',(0.543067286878457,1.,4.10069810244473));
#59351=CARTESIAN_POINT('Ctrl Pts',(0.547235539486759,-1.,4.1072789702877));
#59352=CARTESIAN_POINT('Ctrl Pts',(0.547235539486759,1.,4.1072789702877));
#59353=CARTESIAN_POINT('Ctrl Pts',(0.551437758498246,-1.,4.11384852025578));
#59354=CARTESIAN_POINT('Ctrl Pts',(0.551437758498246,1.,4.11384852025578));
#59355=CARTESIAN_POINT('Ctrl Pts',(0.555673636130778,-1.,4.1204066619623));
#59356=CARTESIAN_POINT('Ctrl Pts',(0.555673636130778,1.,4.1204066619623));
#59357=CARTESIAN_POINT('Ctrl Pts',(0.559942890594628,-1.,4.12695329951859));
#59358=CARTESIAN_POINT('Ctrl Pts',(0.559942890594628,1.,4.12695329951859));
#59359=CARTESIAN_POINT('Ctrl Pts',(0.564245279535705,-1.,4.13348835726086));
#59360=CARTESIAN_POINT('Ctrl Pts',(0.564245279535705,1.,4.13348835726086));
#59361=CARTESIAN_POINT('Ctrl Pts',(0.568580610187115,-1.,4.14001179828669));
#59362=CARTESIAN_POINT('Ctrl Pts',(0.568580610187115,1.,4.14001179828669));
#59363=CARTESIAN_POINT('Ctrl Pts',(0.572948736066276,-1.,4.14652361065787));
#59364=CARTESIAN_POINT('Ctrl Pts',(0.572948736066276,1.,4.14652361065787));
#59365=CARTESIAN_POINT('Ctrl Pts',(0.576469391673916,-1.,4.1517237611974));
#59366=CARTESIAN_POINT('Ctrl Pts',(0.576469391673916,1.,4.1517237611974));
#59367=CARTESIAN_POINT('Ctrl Pts',(0.579124568912543,-1.,4.15561864787379));
#59368=CARTESIAN_POINT('Ctrl Pts',(0.579124568912543,1.,4.15561864787379));
#59369=CARTESIAN_POINT('Ctrl Pts',(0.580901211462913,-1.,4.15821291712391));
#59370=CARTESIAN_POINT('Ctrl Pts',(0.580901211462913,1.,4.15821291712391));
#59371=CARTESIAN_POINT('Ctrl Pts',(0.581791163835814,-1.,4.15950947128175));
#59372=CARTESIAN_POINT('Ctrl Pts',(0.581791163835814,1.,4.15950947128175));
#59373=CARTESIAN_POINT('',(0.385112848332548,1.,3.73017266276632));
#59374=CARTESIAN_POINT('Ctrl Pts',(0.385112848332548,-1.,3.73017266276632));
#59375=CARTESIAN_POINT('Ctrl Pts',(0.385112848332548,-0.666666666666667,
3.73017266276632));
#59376=CARTESIAN_POINT('Ctrl Pts',(0.385112848332548,-0.333333333333333,
3.73017266276632));
#59377=CARTESIAN_POINT('Ctrl Pts',(0.385112848332548,0.333333333333333,
3.73017266276632));
#59378=CARTESIAN_POINT('Ctrl Pts',(0.385112848332548,0.666666666666667,
3.73017266276632));
#59379=CARTESIAN_POINT('Ctrl Pts',(0.385112848332548,1.,3.73017266276632));
#59380=CARTESIAN_POINT('',(0.581791163835814,1.,4.15950947128175));
#59381=CARTESIAN_POINT('',(0.581791163835814,0.,4.15950947128175));
#59382=CARTESIAN_POINT('Ctrl Pts',(0.385112848332549,1.,3.73017266276632));
#59383=CARTESIAN_POINT('Ctrl Pts',(0.385087139001608,1.,3.73021431755218));
#59384=CARTESIAN_POINT('Ctrl Pts',(0.385037797882046,1.,3.73040527620929));
#59385=CARTESIAN_POINT('Ctrl Pts',(0.385031656499141,1.,3.731060828624));
#59386=CARTESIAN_POINT('Ctrl Pts',(0.385187124633964,1.,3.73273893363318));
#59387=CARTESIAN_POINT('Ctrl Pts',(0.385670806454744,1.,3.73621371845475));
#59388=CARTESIAN_POINT('Ctrl Pts',(0.386519576222035,1.,3.74144965781088));
#59389=CARTESIAN_POINT('Ctrl Pts',(0.387663020050396,1.,3.74792651696269));
#59390=CARTESIAN_POINT('Ctrl Pts',(0.38905477589825,1.,3.75529302894757));
#59391=CARTESIAN_POINT('Ctrl Pts',(0.390642072979258,1.,3.76315635032993));
#59392=CARTESIAN_POINT('Ctrl Pts',(0.392372786223346,1.,3.77114011595892));
#59393=CARTESIAN_POINT('Ctrl Pts',(0.394202481011595,1.,3.77894173114368));
#59394=CARTESIAN_POINT('Ctrl Pts',(0.396103205335028,1.,3.78640521279479));
#59395=CARTESIAN_POINT('Ctrl Pts',(0.398064818684158,1.,3.79352887163457));
#59396=CARTESIAN_POINT('Ctrl Pts',(0.400088346504726,1.,3.80040370384659));
#59397=CARTESIAN_POINT('Ctrl Pts',(0.402181320148474,1.,3.80716881962763));
#59398=CARTESIAN_POINT('Ctrl Pts',(0.404352694628236,1.,3.81396374287762));
#59399=CARTESIAN_POINT('Ctrl Pts',(0.406607038258906,1.,3.82087303913741));
#59400=CARTESIAN_POINT('Ctrl Pts',(0.408942371447376,1.,3.82790724256397));
#59401=CARTESIAN_POINT('Ctrl Pts',(0.411353038798459,1.,3.83503345578645));
#59402=CARTESIAN_POINT('Ctrl Pts',(0.413831367016726,1.,3.84219403994742));
#59403=CARTESIAN_POINT('Ctrl Pts',(0.41636967805292,1.,3.8493286415751));
#59404=CARTESIAN_POINT('Ctrl Pts',(0.418962468086809,1.,3.85639825648031));
#59405=CARTESIAN_POINT('Ctrl Pts',(0.421607423177575,1.,3.86339652542749));
#59406=CARTESIAN_POINT('Ctrl Pts',(0.424304173195142,1.,3.87033643487882));
#59407=CARTESIAN_POINT('Ctrl Pts',(0.427053541173469,1.,3.87724240306609));
#59408=CARTESIAN_POINT('Ctrl Pts',(0.429856640579733,1.,3.88414070943334));
#59409=CARTESIAN_POINT('Ctrl Pts',(0.432713929544439,1.,3.89104947940592));
#59410=CARTESIAN_POINT('Ctrl Pts',(0.435624629433505,1.,3.8979725665544));
#59411=CARTESIAN_POINT('Ctrl Pts',(0.438587235458233,1.,3.90490512938546));
#59412=CARTESIAN_POINT('Ctrl Pts',(0.441599824524047,1.,3.91183704069146));
#59413=CARTESIAN_POINT('Ctrl Pts',(0.444660430230592,1.,3.91875701610721));
#59414=CARTESIAN_POINT('Ctrl Pts',(0.447767416837296,1.,3.92565674143424));
#59415=CARTESIAN_POINT('Ctrl Pts',(0.450919768356346,1.,3.93253407403128));
#59416=CARTESIAN_POINT('Ctrl Pts',(0.454116879027575,1.,3.93939080846298));
#59417=CARTESIAN_POINT('Ctrl Pts',(0.457358410451673,1.,3.94623117206675));
#59418=CARTESIAN_POINT('Ctrl Pts',(0.460644124429119,1.,3.95306005817363));
#59419=CARTESIAN_POINT('Ctrl Pts',(0.463973722115744,1.,3.95988133243543));
#59420=CARTESIAN_POINT('Ctrl Pts',(0.467346690880671,1.,3.96669622273946));
#59421=CARTESIAN_POINT('Ctrl Pts',(0.470762379613477,1.,3.97350414289415));
#59422=CARTESIAN_POINT('Ctrl Pts',(0.474220061019542,1.,3.9803033804443));
#59423=CARTESIAN_POINT('Ctrl Pts',(0.477718999122033,1.,3.98709184306743));
#59424=CARTESIAN_POINT('Ctrl Pts',(0.481258512209637,1.,3.99386775880655));
#59425=CARTESIAN_POINT('Ctrl Pts',(0.484838042421754,1.,4.00063045119234));
#59426=CARTESIAN_POINT('Ctrl Pts',(0.48845713042453,1.,4.0073800839092));
#59427=CARTESIAN_POINT('Ctrl Pts',(0.49211538341793,1.,4.01411733503486));
#59428=CARTESIAN_POINT('Ctrl Pts',(0.495812444326222,1.,4.02084308851813));
#59429=CARTESIAN_POINT('Ctrl Pts',(0.499547962340889,1.,4.0275581398015));
#59430=CARTESIAN_POINT('Ctrl Pts',(0.503321556915513,1.,4.0342628417439));
#59431=CARTESIAN_POINT('Ctrl Pts',(0.507132823288361,1.,4.04095715149074));
#59432=CARTESIAN_POINT('Ctrl Pts',(0.510981349219173,1.,4.04764078815591));
#59433=CARTESIAN_POINT('Ctrl Pts',(0.514866728193103,1.,4.05431335771261));
#59434=CARTESIAN_POINT('Ctrl Pts',(0.518788572336809,1.,4.06097448037934));
#59435=CARTESIAN_POINT('Ctrl Pts',(0.522746528602767,1.,4.06762394471075));
#59436=CARTESIAN_POINT('Ctrl Pts',(0.526740277226999,1.,4.07426172299496));
#59437=CARTESIAN_POINT('Ctrl Pts',(0.530769518728075,1.,4.08088789536488));
#59438=CARTESIAN_POINT('Ctrl Pts',(0.534833963476999,1.,4.08750259988693));
#59439=CARTESIAN_POINT('Ctrl Pts',(0.53893332117992,1.,4.09410597627116));
#59440=CARTESIAN_POINT('Ctrl Pts',(0.543067286878457,1.,4.10069810244473));
#59441=CARTESIAN_POINT('Ctrl Pts',(0.547235539486759,1.,4.1072789702877));
#59442=CARTESIAN_POINT('Ctrl Pts',(0.551437758498246,1.,4.11384852025578));
#59443=CARTESIAN_POINT('Ctrl Pts',(0.555673636130778,1.,4.1204066619623));
#59444=CARTESIAN_POINT('Ctrl Pts',(0.559942890594628,1.,4.12695329951859));
#59445=CARTESIAN_POINT('Ctrl Pts',(0.564245279535705,1.,4.13348835726086));
#59446=CARTESIAN_POINT('Ctrl Pts',(0.568580610187115,1.,4.14001179828669));
#59447=CARTESIAN_POINT('Ctrl Pts',(0.572948736066276,1.,4.14652361065787));
#59448=CARTESIAN_POINT('Ctrl Pts',(0.576469391673916,1.,4.1517237611974));
#59449=CARTESIAN_POINT('Ctrl Pts',(0.579124568912543,1.,4.15561864787379));
#59450=CARTESIAN_POINT('Ctrl Pts',(0.580901211462913,1.,4.15821291712391));
#59451=CARTESIAN_POINT('Ctrl Pts',(0.581791163835814,1.,4.15950947128175));
#59452=CARTESIAN_POINT('Origin',(0.581791163835814,0.,4.15950947128175));
#59453=CARTESIAN_POINT('',(0.732042837400619,1.,4.13571194405636));
#59454=CARTESIAN_POINT('Origin',(0.,0.,0.));
#59455=CARTESIAN_POINT('',(0.203156094897895,1.,3.74449296982994));
#59456=CARTESIAN_POINT('Origin',(0.,1.,0.));
#59457=CARTESIAN_POINT('Ctrl Pts',(0.203156094897895,1.,3.74449296982994));
#59458=CARTESIAN_POINT('Ctrl Pts',(0.203156094897895,0.666666666666667,
3.74449296982994));
#59459=CARTESIAN_POINT('Ctrl Pts',(0.203156094897895,0.333333333333333,
3.74449296982994));
#59460=CARTESIAN_POINT('Ctrl Pts',(0.203156094897895,-0.333333333333333,
3.74449296982994));
#59461=CARTESIAN_POINT('Ctrl Pts',(0.203156094897895,-0.666666666666667,
3.74449296982994));
#59462=CARTESIAN_POINT('Ctrl Pts',(0.203156094897895,-1.,3.74449296982994));
#59463=CARTESIAN_POINT('Ctrl Pts',(0.0760622897878233,-1.,4.19931119685982));
#59464=CARTESIAN_POINT('Ctrl Pts',(0.0760622897878233,1.,4.19931119685982));
#59465=CARTESIAN_POINT('Ctrl Pts',(0.0767384596142192,-1.,4.19789138621624));
#59466=CARTESIAN_POINT('Ctrl Pts',(0.0767384596142192,1.,4.19789138621624));
#59467=CARTESIAN_POINT('Ctrl Pts',(0.0780873956244399,-1.,4.19505112860624));
#59468=CARTESIAN_POINT('Ctrl Pts',(0.0780873956244399,1.,4.19505112860624));
#59469=CARTESIAN_POINT('Ctrl Pts',(0.08010058871176,-1.,4.19078883322483));
#59470=CARTESIAN_POINT('Ctrl Pts',(0.08010058871176,1.,4.19078883322483));
#59471=CARTESIAN_POINT('Ctrl Pts',(0.0827644164389507,-1.,4.1851019532944));
#59472=CARTESIAN_POINT('Ctrl Pts',(0.0827644164389507,1.,4.1851019532944));
#59473=CARTESIAN_POINT('Ctrl Pts',(0.0860600915552512,-1.,4.17798698669991));
#59474=CARTESIAN_POINT('Ctrl Pts',(0.0860600915552512,1.,4.17798698669991));
#59475=CARTESIAN_POINT('Ctrl Pts',(0.0893215560850325,-1.,4.17086566491823));
#59476=CARTESIAN_POINT('Ctrl Pts',(0.0893215560850325,1.,4.17086566491823));
#59477=CARTESIAN_POINT('Ctrl Pts',(0.0925486672167687,-1.,4.16373802265942));
#59478=CARTESIAN_POINT('Ctrl Pts',(0.0925486672167687,1.,4.16373802265942));
#59479=CARTESIAN_POINT('Ctrl Pts',(0.0957412403297065,-1.,4.15660412653006));
#59480=CARTESIAN_POINT('Ctrl Pts',(0.0957412403297065,1.,4.15660412653006));
#59481=CARTESIAN_POINT('Ctrl Pts',(0.0988990478899809,-1.,4.1494640891762));
#59482=CARTESIAN_POINT('Ctrl Pts',(0.0988990478899809,1.,4.1494640891762));
#59483=CARTESIAN_POINT('Ctrl Pts',(0.102021826577453,-1.,4.14231804938737));
#59484=CARTESIAN_POINT('Ctrl Pts',(0.102021826577453,1.,4.14231804938737));
#59485=CARTESIAN_POINT('Ctrl Pts',(0.105109286538864,-1.,4.13516614458396));
#59486=CARTESIAN_POINT('Ctrl Pts',(0.105109286538864,1.,4.13516614458396));
#59487=CARTESIAN_POINT('Ctrl Pts',(0.10816112052835,-1.,4.12800848371386));
#59488=CARTESIAN_POINT('Ctrl Pts',(0.10816112052835,1.,4.12800848371386));
#59489=CARTESIAN_POINT('Ctrl Pts',(0.111177012683377,-1.,4.12084512502444));
#59490=CARTESIAN_POINT('Ctrl Pts',(0.111177012683377,1.,4.12084512502444));
#59491=CARTESIAN_POINT('Ctrl Pts',(0.114156649609601,-1.,4.11367603925313));
#59492=CARTESIAN_POINT('Ctrl Pts',(0.114156649609601,1.,4.11367603925313));
#59493=CARTESIAN_POINT('Ctrl Pts',(0.117099722731704,-1.,4.10650113382187));
#59494=CARTESIAN_POINT('Ctrl Pts',(0.117099722731704,1.,4.10650113382187));
#59495=CARTESIAN_POINT('Ctrl Pts',(0.120005924388162,-1.,4.09932031767243));
#59496=CARTESIAN_POINT('Ctrl Pts',(0.120005924388162,1.,4.09932031767243));
#59497=CARTESIAN_POINT('Ctrl Pts',(0.122874946249119,-1.,4.09213355850836));
#59498=CARTESIAN_POINT('Ctrl Pts',(0.122874946249119,1.,4.09213355850836));
#59499=CARTESIAN_POINT('Ctrl Pts',(0.125706476822529,-1.,4.08494093372315));
#59500=CARTESIAN_POINT('Ctrl Pts',(0.125706476822529,1.,4.08494093372315));
#59501=CARTESIAN_POINT('Ctrl Pts',(0.128500200484813,-1.,4.07774270738809));
#59502=CARTESIAN_POINT('Ctrl Pts',(0.128500200484813,1.,4.07774270738809));
#59503=CARTESIAN_POINT('Ctrl Pts',(0.131255793548914,-1.,4.07053931528579));
#59504=CARTESIAN_POINT('Ctrl Pts',(0.131255793548914,1.,4.07053931528579));
#59505=CARTESIAN_POINT('Ctrl Pts',(0.133972916144225,-1.,4.06333121018476));
#59506=CARTESIAN_POINT('Ctrl Pts',(0.133972916144225,1.,4.06333121018476));
#59507=CARTESIAN_POINT('Ctrl Pts',(0.136651205046111,-1.,4.05611873400122));
#59508=CARTESIAN_POINT('Ctrl Pts',(0.136651205046111,1.,4.05611873400122));
#59509=CARTESIAN_POINT('Ctrl Pts',(0.139290267180059,-1.,4.04890199238056));
#59510=CARTESIAN_POINT('Ctrl Pts',(0.139290267180059,1.,4.04890199238056));
#59511=CARTESIAN_POINT('Ctrl Pts',(0.141889671485507,-1.,4.04168069633842));
#59512=CARTESIAN_POINT('Ctrl Pts',(0.141889671485507,1.,4.04168069633842));
#59513=CARTESIAN_POINT('Ctrl Pts',(0.144448947038352,-1.,4.03445411510403));
#59514=CARTESIAN_POINT('Ctrl Pts',(0.144448947038352,1.,4.03445411510403));
#59515=CARTESIAN_POINT('Ctrl Pts',(0.146967602878998,-1.,4.02722143147048));
#59516=CARTESIAN_POINT('Ctrl Pts',(0.146967602878998,1.,4.02722143147048));
#59517=CARTESIAN_POINT('Ctrl Pts',(0.149445144968707,-1.,4.01998203715588));
#59518=CARTESIAN_POINT('Ctrl Pts',(0.149445144968707,1.,4.01998203715588));
#59519=CARTESIAN_POINT('Ctrl Pts',(0.151881094022909,-1.,4.01273584234684));
#59520=CARTESIAN_POINT('Ctrl Pts',(0.151881094022909,1.,4.01273584234684));
#59521=CARTESIAN_POINT('Ctrl Pts',(0.154275004872309,-1.,4.00548360245297));
#59522=CARTESIAN_POINT('Ctrl Pts',(0.154275004872309,1.,4.00548360245297));
#59523=CARTESIAN_POINT('Ctrl Pts',(0.156626481393735,-1.,3.99822717425869));
#59524=CARTESIAN_POINT('Ctrl Pts',(0.156626481393735,1.,3.99822717425869));
#59525=CARTESIAN_POINT('Ctrl Pts',(0.158935123982796,-1.,3.99096873945862));
#59526=CARTESIAN_POINT('Ctrl Pts',(0.158935123982796,1.,3.99096873945862));
#59527=CARTESIAN_POINT('Ctrl Pts',(0.161200482186087,-1.,3.98371010319866));
#59528=CARTESIAN_POINT('Ctrl Pts',(0.161200482186087,1.,3.98371010319866));
#59529=CARTESIAN_POINT('Ctrl Pts',(0.163422004609998,-1.,3.97645194630944));
#59530=CARTESIAN_POINT('Ctrl Pts',(0.163422004609998,1.,3.97645194630944));
#59531=CARTESIAN_POINT('Ctrl Pts',(0.165598992851097,-1.,3.9691931362141));
#59532=CARTESIAN_POINT('Ctrl Pts',(0.165598992851097,1.,3.9691931362141));
#59533=CARTESIAN_POINT('Ctrl Pts',(0.167730547023312,-1.,3.96192990160296));
#59534=CARTESIAN_POINT('Ctrl Pts',(0.167730547023312,1.,3.96192990160296));
#59535=CARTESIAN_POINT('Ctrl Pts',(0.16981566637413,-1.,3.95465744665263));
#59536=CARTESIAN_POINT('Ctrl Pts',(0.16981566637413,1.,3.95465744665263));
#59537=CARTESIAN_POINT('Ctrl Pts',(0.171853355369232,-1.,3.94737164900861));
#59538=CARTESIAN_POINT('Ctrl Pts',(0.171853355369232,1.,3.94737164900861));
#59539=CARTESIAN_POINT('Ctrl Pts',(0.173842734974607,-1.,3.94007083096214));
#59540=CARTESIAN_POINT('Ctrl Pts',(0.173842734974607,1.,3.94007083096214));
#59541=CARTESIAN_POINT('Ctrl Pts',(0.175783136893872,-1.,3.93275726771049));
#59542=CARTESIAN_POINT('Ctrl Pts',(0.175783136893872,1.,3.93275726771049));
#59543=CARTESIAN_POINT('Ctrl Pts',(0.177674246152328,-1.,3.92543942697672));
#59544=CARTESIAN_POINT('Ctrl Pts',(0.177674246152328,1.,3.92543942697672));
#59545=CARTESIAN_POINT('Ctrl Pts',(0.179515885822894,-1.,3.91812876180948));
#59546=CARTESIAN_POINT('Ctrl Pts',(0.179515885822894,1.,3.91812876180948));
#59547=CARTESIAN_POINT('Ctrl Pts',(0.181307740731795,-1.,3.91083557557193));
#59548=CARTESIAN_POINT('Ctrl Pts',(0.181307740731795,1.,3.91083557557193));
#59549=CARTESIAN_POINT('Ctrl Pts',(0.183049081993193,-1.,3.90356488555138));
#59550=CARTESIAN_POINT('Ctrl Pts',(0.183049081993193,1.,3.90356488555138));
#59551=CARTESIAN_POINT('Ctrl Pts',(0.184738537728034,-1.,3.89631300742633));
#59552=CARTESIAN_POINT('Ctrl Pts',(0.184738537728034,1.,3.89631300742633));
#59553=CARTESIAN_POINT('Ctrl Pts',(0.186373724985263,-1.,3.88906196725817));
#59554=CARTESIAN_POINT('Ctrl Pts',(0.186373724985263,1.,3.88906196725817));
#59555=CARTESIAN_POINT('Ctrl Pts',(0.187951632512663,-1.,3.88178563496187));
#59556=CARTESIAN_POINT('Ctrl Pts',(0.187951632512663,1.,3.88178563496187));
#59557=CARTESIAN_POINT('Ctrl Pts',(0.189469253358254,-1.,3.87445976418377));
#59558=CARTESIAN_POINT('Ctrl Pts',(0.189469253358254,1.,3.87445976418377));
#59559=CARTESIAN_POINT('Ctrl Pts',(0.190924190418612,-1.,3.8670715862477));
#59560=CARTESIAN_POINT('Ctrl Pts',(0.190924190418612,1.,3.8670715862477));
#59561=CARTESIAN_POINT('Ctrl Pts',(0.192315153044979,-1.,3.85962774407652));
#59562=CARTESIAN_POINT('Ctrl Pts',(0.192315153044979,1.,3.85962774407652));
#59563=CARTESIAN_POINT('Ctrl Pts',(0.193642806777747,-1.,3.85216762264019));
#59564=CARTESIAN_POINT('Ctrl Pts',(0.193642806777747,1.,3.85216762264019));
#59565=CARTESIAN_POINT('Ctrl Pts',(0.194909009460254,-1.,3.84475203347052));
#59566=CARTESIAN_POINT('Ctrl Pts',(0.194909009460254,1.,3.84475203347052));
#59567=CARTESIAN_POINT('Ctrl Pts',(0.196115198971889,-1.,3.83743910616265));
#59568=CARTESIAN_POINT('Ctrl Pts',(0.196115198971889,1.,3.83743910616265));
#59569=CARTESIAN_POINT('Ctrl Pts',(0.197260935827375,-1.,3.83026221776488));
#59570=CARTESIAN_POINT('Ctrl Pts',(0.197260935827375,1.,3.83026221776488));
#59571=CARTESIAN_POINT('Ctrl Pts',(0.198342616900469,-1.,3.82321127348981));
#59572=CARTESIAN_POINT('Ctrl Pts',(0.198342616900469,1.,3.82321127348981));
#59573=CARTESIAN_POINT('Ctrl Pts',(0.199351525297396,-1.,3.81620203429702));
#59574=CARTESIAN_POINT('Ctrl Pts',(0.199351525297396,1.,3.81620203429702));
#59575=CARTESIAN_POINT('Ctrl Pts',(0.200274679433289,-1.,3.80909529318501));
#59576=CARTESIAN_POINT('Ctrl Pts',(0.200274679433289,1.,3.80909529318501));
#59577=CARTESIAN_POINT('Ctrl Pts',(0.201097756307251,-1.,3.80175247447171));
#59578=CARTESIAN_POINT('Ctrl Pts',(0.201097756307251,1.,3.80175247447171));
#59579=CARTESIAN_POINT('Ctrl Pts',(0.201807533800798,-1.,3.79408354187274));
#59580=CARTESIAN_POINT('Ctrl Pts',(0.201807533800798,1.,3.79408354187274));
#59581=CARTESIAN_POINT('Ctrl Pts',(0.202394260512192,-1.,3.78609175019317));
#59582=CARTESIAN_POINT('Ctrl Pts',(0.202394260512192,1.,3.78609175019317));
#59583=CARTESIAN_POINT('Ctrl Pts',(0.202854729699196,-1.,3.77793553476879));
#59584=CARTESIAN_POINT('Ctrl Pts',(0.202854729699196,1.,3.77793553476879));
#59585=CARTESIAN_POINT('Ctrl Pts',(0.203192390045337,-1.,3.76992071595267));
#59586=CARTESIAN_POINT('Ctrl Pts',(0.203192390045337,1.,3.76992071595267));
#59587=CARTESIAN_POINT('Ctrl Pts',(0.203414634707646,-1.,3.76242717937273));
#59588=CARTESIAN_POINT('Ctrl Pts',(0.203414634707646,1.,3.76242717937273));
#59589=CARTESIAN_POINT('Ctrl Pts',(0.203530796848403,-1.,3.75585118707924));
#59590=CARTESIAN_POINT('Ctrl Pts',(0.203530796848403,1.,3.75585118707924));
#59591=CARTESIAN_POINT('Ctrl Pts',(0.203550035479096,-1.,3.75054693397716));
#59592=CARTESIAN_POINT('Ctrl Pts',(0.203550035479096,1.,3.75054693397716));
#59593=CARTESIAN_POINT('Ctrl Pts',(0.203478844530229,-1.,3.74675472018582));
#59594=CARTESIAN_POINT('Ctrl Pts',(0.203478844530229,1.,3.74675472018582));
#59595=CARTESIAN_POINT('Ctrl Pts',(0.203352057956055,-1.,3.7450208092684));
#59596=CARTESIAN_POINT('Ctrl Pts',(0.203352057956055,1.,3.7450208092684));
#59597=CARTESIAN_POINT('Ctrl Pts',(0.203218215747894,-1.,3.74446880195845));
#59598=CARTESIAN_POINT('Ctrl Pts',(0.203218215747894,1.,3.74446880195845));
#59599=CARTESIAN_POINT('Ctrl Pts',(0.20311176758786,-1.,3.74443319346666));
#59600=CARTESIAN_POINT('Ctrl Pts',(0.20311176758786,1.,3.74443319346666));
#59601=CARTESIAN_POINT('Ctrl Pts',(0.203054238699719,-1.,3.74449849461127));
#59602=CARTESIAN_POINT('Ctrl Pts',(0.203054238699719,1.,3.74449849461127));
#59603=CARTESIAN_POINT('',(0.0760622897878233,1.,4.19931119685982));
#59604=CARTESIAN_POINT('Ctrl Pts',(0.0760622897878233,1.,4.19931119685982));
#59605=CARTESIAN_POINT('Ctrl Pts',(0.0767384596142192,1.,4.19789138621624));
#59606=CARTESIAN_POINT('Ctrl Pts',(0.0780873956244399,1.,4.19505112860624));
#59607=CARTESIAN_POINT('Ctrl Pts',(0.08010058871176,1.,4.19078883322483));
#59608=CARTESIAN_POINT('Ctrl Pts',(0.0827644164389507,1.,4.1851019532944));
#59609=CARTESIAN_POINT('Ctrl Pts',(0.0860600915552512,1.,4.17798698669991));
#59610=CARTESIAN_POINT('Ctrl Pts',(0.0893215560850325,1.,4.17086566491823));
#59611=CARTESIAN_POINT('Ctrl Pts',(0.0925486672167687,1.,4.16373802265942));
#59612=CARTESIAN_POINT('Ctrl Pts',(0.0957412403297065,1.,4.15660412653006));
#59613=CARTESIAN_POINT('Ctrl Pts',(0.0988990478899809,1.,4.1494640891762));
#59614=CARTESIAN_POINT('Ctrl Pts',(0.102021826577453,1.,4.14231804938737));
#59615=CARTESIAN_POINT('Ctrl Pts',(0.105109286538864,1.,4.13516614458396));
#59616=CARTESIAN_POINT('Ctrl Pts',(0.10816112052835,1.,4.12800848371386));
#59617=CARTESIAN_POINT('Ctrl Pts',(0.111177012683377,1.,4.12084512502444));
#59618=CARTESIAN_POINT('Ctrl Pts',(0.114156649609601,1.,4.11367603925313));
#59619=CARTESIAN_POINT('Ctrl Pts',(0.117099722731704,1.,4.10650113382187));
#59620=CARTESIAN_POINT('Ctrl Pts',(0.120005924388162,1.,4.09932031767243));
#59621=CARTESIAN_POINT('Ctrl Pts',(0.122874946249119,1.,4.09213355850836));
#59622=CARTESIAN_POINT('Ctrl Pts',(0.125706476822529,1.,4.08494093372315));
#59623=CARTESIAN_POINT('Ctrl Pts',(0.128500200484813,1.,4.07774270738809));
#59624=CARTESIAN_POINT('Ctrl Pts',(0.131255793548914,1.,4.07053931528579));
#59625=CARTESIAN_POINT('Ctrl Pts',(0.133972916144225,1.,4.06333121018476));
#59626=CARTESIAN_POINT('Ctrl Pts',(0.136651205046111,1.,4.05611873400122));
#59627=CARTESIAN_POINT('Ctrl Pts',(0.139290267180059,1.,4.04890199238056));
#59628=CARTESIAN_POINT('Ctrl Pts',(0.141889671485507,1.,4.04168069633842));
#59629=CARTESIAN_POINT('Ctrl Pts',(0.144448947038352,1.,4.03445411510403));
#59630=CARTESIAN_POINT('Ctrl Pts',(0.146967602878998,1.,4.02722143147048));
#59631=CARTESIAN_POINT('Ctrl Pts',(0.149445144968707,1.,4.01998203715588));
#59632=CARTESIAN_POINT('Ctrl Pts',(0.151881094022909,1.,4.01273584234684));
#59633=CARTESIAN_POINT('Ctrl Pts',(0.154275004872309,1.,4.00548360245297));
#59634=CARTESIAN_POINT('Ctrl Pts',(0.156626481393735,1.,3.99822717425869));
#59635=CARTESIAN_POINT('Ctrl Pts',(0.158935123982796,1.,3.99096873945862));
#59636=CARTESIAN_POINT('Ctrl Pts',(0.161200482186087,1.,3.98371010319866));
#59637=CARTESIAN_POINT('Ctrl Pts',(0.163422004609998,1.,3.97645194630944));
#59638=CARTESIAN_POINT('Ctrl Pts',(0.165598992851097,1.,3.9691931362141));
#59639=CARTESIAN_POINT('Ctrl Pts',(0.167730547023312,1.,3.96192990160296));
#59640=CARTESIAN_POINT('Ctrl Pts',(0.16981566637413,1.,3.95465744665263));
#59641=CARTESIAN_POINT('Ctrl Pts',(0.171853355369232,1.,3.94737164900861));
#59642=CARTESIAN_POINT('Ctrl Pts',(0.173842734974607,1.,3.94007083096214));
#59643=CARTESIAN_POINT('Ctrl Pts',(0.175783136893872,1.,3.93275726771049));
#59644=CARTESIAN_POINT('Ctrl Pts',(0.177674246152328,1.,3.92543942697672));
#59645=CARTESIAN_POINT('Ctrl Pts',(0.179515885822894,1.,3.91812876180948));
#59646=CARTESIAN_POINT('Ctrl Pts',(0.181307740731795,1.,3.91083557557193));
#59647=CARTESIAN_POINT('Ctrl Pts',(0.183049081993193,1.,3.90356488555138));
#59648=CARTESIAN_POINT('Ctrl Pts',(0.184738537728034,1.,3.89631300742633));
#59649=CARTESIAN_POINT('Ctrl Pts',(0.186373724985263,1.,3.88906196725817));
#59650=CARTESIAN_POINT('Ctrl Pts',(0.187951632512663,1.,3.88178563496187));
#59651=CARTESIAN_POINT('Ctrl Pts',(0.189469253358254,1.,3.87445976418377));
#59652=CARTESIAN_POINT('Ctrl Pts',(0.190924190418612,1.,3.8670715862477));
#59653=CARTESIAN_POINT('Ctrl Pts',(0.192315153044979,1.,3.85962774407652));
#59654=CARTESIAN_POINT('Ctrl Pts',(0.193642806777747,1.,3.85216762264019));
#59655=CARTESIAN_POINT('Ctrl Pts',(0.194909009460254,1.,3.84475203347052));
#59656=CARTESIAN_POINT('Ctrl Pts',(0.196115198971889,1.,3.83743910616265));
#59657=CARTESIAN_POINT('Ctrl Pts',(0.197260935827375,1.,3.83026221776488));
#59658=CARTESIAN_POINT('Ctrl Pts',(0.198342616900469,1.,3.82321127348981));
#59659=CARTESIAN_POINT('Ctrl Pts',(0.199351525297396,1.,3.81620203429702));
#59660=CARTESIAN_POINT('Ctrl Pts',(0.200274679433289,1.,3.80909529318501));
#59661=CARTESIAN_POINT('Ctrl Pts',(0.201097756307251,1.,3.80175247447171));
#59662=CARTESIAN_POINT('Ctrl Pts',(0.201807533800798,1.,3.79408354187274));
#59663=CARTESIAN_POINT('Ctrl Pts',(0.202394260512192,1.,3.78609175019317));
#59664=CARTESIAN_POINT('Ctrl Pts',(0.202854729699196,1.,3.77793553476879));
#59665=CARTESIAN_POINT('Ctrl Pts',(0.203192390045337,1.,3.76992071595267));
#59666=CARTESIAN_POINT('Ctrl Pts',(0.203414634707646,1.,3.76242717937273));
#59667=CARTESIAN_POINT('Ctrl Pts',(0.203530796848403,1.,3.75585118707924));
#59668=CARTESIAN_POINT('Ctrl Pts',(0.203550035479096,1.,3.75054693397716));
#59669=CARTESIAN_POINT('Ctrl Pts',(0.203484186269314,1.,3.74703926501843));
#59670=CARTESIAN_POINT('Ctrl Pts',(0.203375226874331,1.,3.74535749969262));
#59671=CARTESIAN_POINT('Ctrl Pts',(0.203266610111263,1.,3.74471097893961));
#59672=CARTESIAN_POINT('Ctrl Pts',(0.203188003947964,1.,3.74453008995129));
#59673=CARTESIAN_POINT('Ctrl Pts',(0.203156094897895,1.,3.74449296982994));
#59674=CARTESIAN_POINT('',(0.0760622897878233,0.,4.19931119685982));
#59675=CARTESIAN_POINT('Ctrl Pts',(-0.20305423869972,-1.,3.74449849461127));
#59676=CARTESIAN_POINT('Ctrl Pts',(-0.20305423869972,1.,3.74449849461127));
#59677=CARTESIAN_POINT('Ctrl Pts',(-0.203111767587923,-1.,3.7444331934681));
#59678=CARTESIAN_POINT('Ctrl Pts',(-0.203111767587923,1.,3.7444331934681));
#59679=CARTESIAN_POINT('Ctrl Pts',(-0.203218215748059,-1.,3.7444688019622));
#59680=CARTESIAN_POINT('Ctrl Pts',(-0.203218215748059,1.,3.7444688019622));
#59681=CARTESIAN_POINT('Ctrl Pts',(-0.203352057956297,-1.,3.74502080927395));
#59682=CARTESIAN_POINT('Ctrl Pts',(-0.203352057956297,1.,3.74502080927395));
#59683=CARTESIAN_POINT('Ctrl Pts',(-0.203478844530447,-1.,3.7467547201908));
#59684=CARTESIAN_POINT('Ctrl Pts',(-0.203478844530447,1.,3.7467547201908));
#59685=CARTESIAN_POINT('Ctrl Pts',(-0.203550035479166,-1.,3.75054693397875));
#59686=CARTESIAN_POINT('Ctrl Pts',(-0.203550035479166,1.,3.75054693397875));
#59687=CARTESIAN_POINT('Ctrl Pts',(-0.203530796848322,-1.,3.75585118707734));
#59688=CARTESIAN_POINT('Ctrl Pts',(-0.203530796848322,1.,3.75585118707734));
#59689=CARTESIAN_POINT('Ctrl Pts',(-0.203414634707479,-1.,3.76242717936885));
#59690=CARTESIAN_POINT('Ctrl Pts',(-0.203414634707479,1.,3.76242717936885));
#59691=CARTESIAN_POINT('Ctrl Pts',(-0.203192390045165,-1.,3.7699207159487));
#59692=CARTESIAN_POINT('Ctrl Pts',(-0.203192390045165,1.,3.7699207159487));
#59693=CARTESIAN_POINT('Ctrl Pts',(-0.202854729699081,-1.,3.77793553476614));
#59694=CARTESIAN_POINT('Ctrl Pts',(-0.202854729699081,1.,3.77793553476614));
#59695=CARTESIAN_POINT('Ctrl Pts',(-0.20239426051216,-1.,3.78609175019242));
#59696=CARTESIAN_POINT('Ctrl Pts',(-0.20239426051216,1.,3.78609175019242));
#59697=CARTESIAN_POINT('Ctrl Pts',(-0.201807533800837,-1.,3.7940835418736));
#59698=CARTESIAN_POINT('Ctrl Pts',(-0.201807533800837,1.,3.7940835418736));
#59699=CARTESIAN_POINT('Ctrl Pts',(-0.201097756307326,-1.,3.80175247447337));
#59700=CARTESIAN_POINT('Ctrl Pts',(-0.201097756307326,1.,3.80175247447337));
#59701=CARTESIAN_POINT('Ctrl Pts',(-0.200274679433365,-1.,3.80909529318669));
#59702=CARTESIAN_POINT('Ctrl Pts',(-0.200274679433365,1.,3.80909529318669));
#59703=CARTESIAN_POINT('Ctrl Pts',(-0.199351525297447,-1.,3.81620203429815));
#59704=CARTESIAN_POINT('Ctrl Pts',(-0.199351525297447,1.,3.81620203429815));
#59705=CARTESIAN_POINT('Ctrl Pts',(-0.198342616900487,-1.,3.82321127349016));
#59706=CARTESIAN_POINT('Ctrl Pts',(-0.198342616900487,1.,3.82321127349016));
#59707=CARTESIAN_POINT('Ctrl Pts',(-0.197260935827362,-1.,3.83026221776456));
#59708=CARTESIAN_POINT('Ctrl Pts',(-0.197260935827362,1.,3.83026221776456));
#59709=CARTESIAN_POINT('Ctrl Pts',(-0.196115198971859,-1.,3.83743910616195));
#59710=CARTESIAN_POINT('Ctrl Pts',(-0.196115198971859,1.,3.83743910616195));
#59711=CARTESIAN_POINT('Ctrl Pts',(-0.194909009460221,-1.,3.84475203346977));
#59712=CARTESIAN_POINT('Ctrl Pts',(-0.194909009460221,1.,3.84475203346977));
#59713=CARTESIAN_POINT('Ctrl Pts',(-0.193642806777723,-1.,3.85216762263966));
#59714=CARTESIAN_POINT('Ctrl Pts',(-0.193642806777723,1.,3.85216762263966));
#59715=CARTESIAN_POINT('Ctrl Pts',(-0.192315153044971,-1.,3.85962774407633));
#59716=CARTESIAN_POINT('Ctrl Pts',(-0.192315153044971,1.,3.85962774407633));
#59717=CARTESIAN_POINT('Ctrl Pts',(-0.19092419041862,-1.,3.86707158624783));
#59718=CARTESIAN_POINT('Ctrl Pts',(-0.19092419041862,1.,3.86707158624783));
#59719=CARTESIAN_POINT('Ctrl Pts',(-0.189469253358273,-1.,3.87445976418412));
#59720=CARTESIAN_POINT('Ctrl Pts',(-0.189469253358273,1.,3.87445976418412));
#59721=CARTESIAN_POINT('Ctrl Pts',(-0.187951632512685,-1.,3.88178563496228));
#59722=CARTESIAN_POINT('Ctrl Pts',(-0.187951632512685,1.,3.88178563496228));
#59723=CARTESIAN_POINT('Ctrl Pts',(-0.186373724985281,-1.,3.88906196725848));
#59724=CARTESIAN_POINT('Ctrl Pts',(-0.186373724985281,1.,3.88906196725848));
#59725=CARTESIAN_POINT('Ctrl Pts',(-0.184738537728043,-1.,3.89631300742646));
#59726=CARTESIAN_POINT('Ctrl Pts',(-0.184738537728043,1.,3.89631300742646));
#59727=CARTESIAN_POINT('Ctrl Pts',(-0.183049081993191,-1.,3.90356488555132));
#59728=CARTESIAN_POINT('Ctrl Pts',(-0.183049081993191,1.,3.90356488555132));
#59729=CARTESIAN_POINT('Ctrl Pts',(-0.181307740731786,-1.,3.91083557557175));
#59730=CARTESIAN_POINT('Ctrl Pts',(-0.181307740731786,1.,3.91083557557175));
#59731=CARTESIAN_POINT('Ctrl Pts',(-0.179515885822882,-1.,3.91812876180926));
#59732=CARTESIAN_POINT('Ctrl Pts',(-0.179515885822882,1.,3.91812876180926));
#59733=CARTESIAN_POINT('Ctrl Pts',(-0.177674246152318,-1.,3.92543942697655));
#59734=CARTESIAN_POINT('Ctrl Pts',(-0.177674246152318,1.,3.92543942697655));
#59735=CARTESIAN_POINT('Ctrl Pts',(-0.175783136893868,-1.,3.93275726771042));
#59736=CARTESIAN_POINT('Ctrl Pts',(-0.175783136893868,1.,3.93275726771042));
#59737=CARTESIAN_POINT('Ctrl Pts',(-0.17384273497461,-1.,3.94007083096217));
#59738=CARTESIAN_POINT('Ctrl Pts',(-0.17384273497461,1.,3.94007083096217));
#59739=CARTESIAN_POINT('Ctrl Pts',(-0.17185335536924,-1.,3.94737164900868));
#59740=CARTESIAN_POINT('Ctrl Pts',(-0.17185335536924,1.,3.94737164900868));
#59741=CARTESIAN_POINT('Ctrl Pts',(-0.169815666374139,-1.,3.95465744665268));
#59742=CARTESIAN_POINT('Ctrl Pts',(-0.169815666374139,1.,3.95465744665268));
#59743=CARTESIAN_POINT('Ctrl Pts',(-0.16773054702332,-1.,3.96192990160296));
#59744=CARTESIAN_POINT('Ctrl Pts',(-0.16773054702332,1.,3.96192990160296));
#59745=CARTESIAN_POINT('Ctrl Pts',(-0.165598992851102,-1.,3.96919313621407));
#59746=CARTESIAN_POINT('Ctrl Pts',(-0.165598992851102,1.,3.96919313621407));
#59747=CARTESIAN_POINT('Ctrl Pts',(-0.163422004609999,-1.,3.97645194630943));
#59748=CARTESIAN_POINT('Ctrl Pts',(-0.163422004609999,1.,3.97645194630943));
#59749=CARTESIAN_POINT('Ctrl Pts',(-0.161200482186085,-1.,3.98371010319872));
#59750=CARTESIAN_POINT('Ctrl Pts',(-0.161200482186085,1.,3.98371010319872));
#59751=CARTESIAN_POINT('Ctrl Pts',(-0.158935123982793,-1.,3.99096873945878));
#59752=CARTESIAN_POINT('Ctrl Pts',(-0.158935123982793,1.,3.99096873945878));
#59753=CARTESIAN_POINT('Ctrl Pts',(-0.156626481393734,-1.,3.99822717425893));
#59754=CARTESIAN_POINT('Ctrl Pts',(-0.156626481393734,1.,3.99822717425893));
#59755=CARTESIAN_POINT('Ctrl Pts',(-0.154275004872311,-1.,4.00548360245319));
#59756=CARTESIAN_POINT('Ctrl Pts',(-0.154275004872311,1.,4.00548360245319));
#59757=CARTESIAN_POINT('Ctrl Pts',(-0.151881094022911,-1.,4.01273584234689));
#59758=CARTESIAN_POINT('Ctrl Pts',(-0.151881094022911,1.,4.01273584234689));
#59759=CARTESIAN_POINT('Ctrl Pts',(-0.149445144968707,-1.,4.01998203715564));
#59760=CARTESIAN_POINT('Ctrl Pts',(-0.149445144968707,1.,4.01998203715564));
#59761=CARTESIAN_POINT('Ctrl Pts',(-0.146967602878994,-1.,4.02722143146994));
#59762=CARTESIAN_POINT('Ctrl Pts',(-0.146967602878994,1.,4.02722143146994));
#59763=CARTESIAN_POINT('Ctrl Pts',(-0.144448947038345,-1.,4.03445411510333));
#59764=CARTESIAN_POINT('Ctrl Pts',(-0.144448947038345,1.,4.03445411510333));
#59765=CARTESIAN_POINT('Ctrl Pts',(-0.1418896714855,-1.,4.04168069633781));
#59766=CARTESIAN_POINT('Ctrl Pts',(-0.1418896714855,1.,4.04168069633781));
#59767=CARTESIAN_POINT('Ctrl Pts',(-0.139290267180057,-1.,4.04890199238036));
#59768=CARTESIAN_POINT('Ctrl Pts',(-0.139290267180057,1.,4.04890199238036));
#59769=CARTESIAN_POINT('Ctrl Pts',(-0.136651205046119,-1.,4.05611873400172));
#59770=CARTESIAN_POINT('Ctrl Pts',(-0.136651205046119,1.,4.05611873400172));
#59771=CARTESIAN_POINT('Ctrl Pts',(-0.133972916144245,-1.,4.06333121018596));
#59772=CARTESIAN_POINT('Ctrl Pts',(-0.133972916144245,1.,4.06333121018596));
#59773=CARTESIAN_POINT('Ctrl Pts',(-0.131255793548941,-1.,4.0705393152874));
#59774=CARTESIAN_POINT('Ctrl Pts',(-0.131255793548941,1.,4.0705393152874));
#59775=CARTESIAN_POINT('Ctrl Pts',(-0.128500200484838,-1.,4.07774270738954));
#59776=CARTESIAN_POINT('Ctrl Pts',(-0.128500200484838,1.,4.07774270738954));
#59777=CARTESIAN_POINT('Ctrl Pts',(-0.12570647682254,-1.,4.08494093372377));
#59778=CARTESIAN_POINT('Ctrl Pts',(-0.12570647682254,1.,4.08494093372377));
#59779=CARTESIAN_POINT('Ctrl Pts',(-0.122874946249107,-1.,4.09213355850756));
#59780=CARTESIAN_POINT('Ctrl Pts',(-0.122874946249107,1.,4.09213355850756));
#59781=CARTESIAN_POINT('Ctrl Pts',(-0.120005924388124,-1.,4.09932031767002));
#59782=CARTESIAN_POINT('Ctrl Pts',(-0.120005924388124,1.,4.09932031767002));
#59783=CARTESIAN_POINT('Ctrl Pts',(-0.117099722731648,-1.,4.10650113381833));
#59784=CARTESIAN_POINT('Ctrl Pts',(-0.117099722731648,1.,4.10650113381833));
#59785=CARTESIAN_POINT('Ctrl Pts',(-0.114156649609546,-1.,4.11367603924961));
#59786=CARTESIAN_POINT('Ctrl Pts',(-0.114156649609546,1.,4.11367603924961));
#59787=CARTESIAN_POINT('Ctrl Pts',(-0.111177012683347,-1.,4.1208451250225));
#59788=CARTESIAN_POINT('Ctrl Pts',(-0.111177012683347,1.,4.1208451250225));
#59789=CARTESIAN_POINT('Ctrl Pts',(-0.10816112052837,-1.,4.12800848371504));
#59790=CARTESIAN_POINT('Ctrl Pts',(-0.10816112052837,1.,4.12800848371504));
#59791=CARTESIAN_POINT('Ctrl Pts',(-0.105109286538945,-1.,4.13516614458895));
#59792=CARTESIAN_POINT('Ctrl Pts',(-0.105109286538945,1.,4.13516614458895));
#59793=CARTESIAN_POINT('Ctrl Pts',(-0.102021826577584,-1.,4.14231804939538));
#59794=CARTESIAN_POINT('Ctrl Pts',(-0.102021826577584,1.,4.14231804939538));
#59795=CARTESIAN_POINT('Ctrl Pts',(-0.0988990478901228,-1.,4.14946408918485));
#59796=CARTESIAN_POINT('Ctrl Pts',(-0.0988990478901228,1.,4.14946408918485));
#59797=CARTESIAN_POINT('Ctrl Pts',(-0.0957412403298009,-1.,4.15660412653577));
#59798=CARTESIAN_POINT('Ctrl Pts',(-0.0957412403298009,1.,4.15660412653577));
#59799=CARTESIAN_POINT('Ctrl Pts',(-0.0925486672167534,-1.,4.16373802265839));
#59800=CARTESIAN_POINT('Ctrl Pts',(-0.0925486672167534,1.,4.16373802265839));
#59801=CARTESIAN_POINT('Ctrl Pts',(-0.0893215560848652,-1.,4.17086566490794));
#59802=CARTESIAN_POINT('Ctrl Pts',(-0.0893215560848652,1.,4.17086566490794));
#59803=CARTESIAN_POINT('Ctrl Pts',(-0.0860600915549399,-1.,4.17798698668094));
#59804=CARTESIAN_POINT('Ctrl Pts',(-0.0860600915549399,1.,4.17798698668094));
#59805=CARTESIAN_POINT('Ctrl Pts',(-0.0827644164385681,-1.,4.18510195327123));
#59806=CARTESIAN_POINT('Ctrl Pts',(-0.0827644164385681,1.,4.18510195327123));
#59807=CARTESIAN_POINT('Ctrl Pts',(-0.0801005887114322,-1.,4.19078883320504));
#59808=CARTESIAN_POINT('Ctrl Pts',(-0.0801005887114322,1.,4.19078883320504));
#59809=CARTESIAN_POINT('Ctrl Pts',(-0.07808739562424,-1.,4.19505112859416));
#59810=CARTESIAN_POINT('Ctrl Pts',(-0.07808739562424,1.,4.19505112859416));
#59811=CARTESIAN_POINT('Ctrl Pts',(-0.0767384596141467,-1.,4.1978913862118));
#59812=CARTESIAN_POINT('Ctrl Pts',(-0.0767384596141467,1.,4.1978913862118));
#59813=CARTESIAN_POINT('Ctrl Pts',(-0.0760622897878249,-1.,4.19931119685982));
#59814=CARTESIAN_POINT('Ctrl Pts',(-0.0760622897878249,1.,4.19931119685982));
#59815=CARTESIAN_POINT('',(-0.203156094896102,1.,3.74449296983004));
#59816=CARTESIAN_POINT('Ctrl Pts',(-0.203156094896101,-1.,3.74449296983004));
#59817=CARTESIAN_POINT('Ctrl Pts',(-0.203156094896101,-0.666666666666667,
3.74449296983004));
#59818=CARTESIAN_POINT('Ctrl Pts',(-0.203156094896101,-0.333333333333333,
3.74449296983004));
#59819=CARTESIAN_POINT('Ctrl Pts',(-0.203156094896101,0.333333333333333,
3.74449296983004));
#59820=CARTESIAN_POINT('Ctrl Pts',(-0.203156094896101,0.666666666666667,
3.74449296983004));
#59821=CARTESIAN_POINT('Ctrl Pts',(-0.203156094896101,1.,3.74449296983004));
#59822=CARTESIAN_POINT('',(-0.0760622897878249,1.,4.19931119685982));
#59823=CARTESIAN_POINT('',(-0.0760622897878249,0.,4.19931119685982));
#59824=CARTESIAN_POINT('Ctrl Pts',(-0.203156094896101,1.,3.74449296983004));
#59825=CARTESIAN_POINT('Ctrl Pts',(-0.203188003946657,1.,3.74453008995092));
#59826=CARTESIAN_POINT('Ctrl Pts',(-0.203266610110531,1.,3.74471097893845));
#59827=CARTESIAN_POINT('Ctrl Pts',(-0.203375226874122,1.,3.74535749969115));
#59828=CARTESIAN_POINT('Ctrl Pts',(-0.203484186269415,1.,3.74703926501752));
#59829=CARTESIAN_POINT('Ctrl Pts',(-0.203550035479166,1.,3.75054693397875));
#59830=CARTESIAN_POINT('Ctrl Pts',(-0.203530796848322,1.,3.75585118707734));
#59831=CARTESIAN_POINT('Ctrl Pts',(-0.203414634707479,1.,3.76242717936885));
#59832=CARTESIAN_POINT('Ctrl Pts',(-0.203192390045165,1.,3.7699207159487));
#59833=CARTESIAN_POINT('Ctrl Pts',(-0.202854729699081,1.,3.77793553476614));
#59834=CARTESIAN_POINT('Ctrl Pts',(-0.20239426051216,1.,3.78609175019242));
#59835=CARTESIAN_POINT('Ctrl Pts',(-0.201807533800837,1.,3.7940835418736));
#59836=CARTESIAN_POINT('Ctrl Pts',(-0.201097756307326,1.,3.80175247447337));
#59837=CARTESIAN_POINT('Ctrl Pts',(-0.200274679433365,1.,3.80909529318669));
#59838=CARTESIAN_POINT('Ctrl Pts',(-0.199351525297447,1.,3.81620203429815));
#59839=CARTESIAN_POINT('Ctrl Pts',(-0.198342616900487,1.,3.82321127349016));
#59840=CARTESIAN_POINT('Ctrl Pts',(-0.197260935827362,1.,3.83026221776456));
#59841=CARTESIAN_POINT('Ctrl Pts',(-0.196115198971859,1.,3.83743910616195));
#59842=CARTESIAN_POINT('Ctrl Pts',(-0.194909009460221,1.,3.84475203346977));
#59843=CARTESIAN_POINT('Ctrl Pts',(-0.193642806777723,1.,3.85216762263966));
#59844=CARTESIAN_POINT('Ctrl Pts',(-0.192315153044971,1.,3.85962774407633));
#59845=CARTESIAN_POINT('Ctrl Pts',(-0.19092419041862,1.,3.86707158624783));
#59846=CARTESIAN_POINT('Ctrl Pts',(-0.189469253358273,1.,3.87445976418412));
#59847=CARTESIAN_POINT('Ctrl Pts',(-0.187951632512685,1.,3.88178563496228));
#59848=CARTESIAN_POINT('Ctrl Pts',(-0.186373724985281,1.,3.88906196725848));
#59849=CARTESIAN_POINT('Ctrl Pts',(-0.184738537728043,1.,3.89631300742646));
#59850=CARTESIAN_POINT('Ctrl Pts',(-0.183049081993191,1.,3.90356488555132));
#59851=CARTESIAN_POINT('Ctrl Pts',(-0.181307740731786,1.,3.91083557557175));
#59852=CARTESIAN_POINT('Ctrl Pts',(-0.179515885822882,1.,3.91812876180926));
#59853=CARTESIAN_POINT('Ctrl Pts',(-0.177674246152318,1.,3.92543942697655));
#59854=CARTESIAN_POINT('Ctrl Pts',(-0.175783136893868,1.,3.93275726771042));
#59855=CARTESIAN_POINT('Ctrl Pts',(-0.17384273497461,1.,3.94007083096217));
#59856=CARTESIAN_POINT('Ctrl Pts',(-0.17185335536924,1.,3.94737164900868));
#59857=CARTESIAN_POINT('Ctrl Pts',(-0.169815666374139,1.,3.95465744665268));
#59858=CARTESIAN_POINT('Ctrl Pts',(-0.16773054702332,1.,3.96192990160296));
#59859=CARTESIAN_POINT('Ctrl Pts',(-0.165598992851102,1.,3.96919313621407));
#59860=CARTESIAN_POINT('Ctrl Pts',(-0.163422004609999,1.,3.97645194630943));
#59861=CARTESIAN_POINT('Ctrl Pts',(-0.161200482186085,1.,3.98371010319872));
#59862=CARTESIAN_POINT('Ctrl Pts',(-0.158935123982793,1.,3.99096873945878));
#59863=CARTESIAN_POINT('Ctrl Pts',(-0.156626481393734,1.,3.99822717425893));
#59864=CARTESIAN_POINT('Ctrl Pts',(-0.154275004872311,1.,4.00548360245319));
#59865=CARTESIAN_POINT('Ctrl Pts',(-0.151881094022911,1.,4.01273584234689));
#59866=CARTESIAN_POINT('Ctrl Pts',(-0.149445144968707,1.,4.01998203715564));
#59867=CARTESIAN_POINT('Ctrl Pts',(-0.146967602878994,1.,4.02722143146994));
#59868=CARTESIAN_POINT('Ctrl Pts',(-0.144448947038345,1.,4.03445411510333));
#59869=CARTESIAN_POINT('Ctrl Pts',(-0.1418896714855,1.,4.04168069633781));
#59870=CARTESIAN_POINT('Ctrl Pts',(-0.139290267180057,1.,4.04890199238036));
#59871=CARTESIAN_POINT('Ctrl Pts',(-0.136651205046119,1.,4.05611873400172));
#59872=CARTESIAN_POINT('Ctrl Pts',(-0.133972916144245,1.,4.06333121018596));
#59873=CARTESIAN_POINT('Ctrl Pts',(-0.131255793548941,1.,4.0705393152874));
#59874=CARTESIAN_POINT('Ctrl Pts',(-0.128500200484838,1.,4.07774270738954));
#59875=CARTESIAN_POINT('Ctrl Pts',(-0.12570647682254,1.,4.08494093372377));
#59876=CARTESIAN_POINT('Ctrl Pts',(-0.122874946249107,1.,4.09213355850756));
#59877=CARTESIAN_POINT('Ctrl Pts',(-0.120005924388124,1.,4.09932031767002));
#59878=CARTESIAN_POINT('Ctrl Pts',(-0.117099722731648,1.,4.10650113381833));
#59879=CARTESIAN_POINT('Ctrl Pts',(-0.114156649609546,1.,4.11367603924961));
#59880=CARTESIAN_POINT('Ctrl Pts',(-0.111177012683347,1.,4.1208451250225));
#59881=CARTESIAN_POINT('Ctrl Pts',(-0.10816112052837,1.,4.12800848371504));
#59882=CARTESIAN_POINT('Ctrl Pts',(-0.105109286538945,1.,4.13516614458895));
#59883=CARTESIAN_POINT('Ctrl Pts',(-0.102021826577584,1.,4.14231804939538));
#59884=CARTESIAN_POINT('Ctrl Pts',(-0.0988990478901228,1.,4.14946408918485));
#59885=CARTESIAN_POINT('Ctrl Pts',(-0.0957412403298009,1.,4.15660412653577));
#59886=CARTESIAN_POINT('Ctrl Pts',(-0.0925486672167534,1.,4.16373802265839));
#59887=CARTESIAN_POINT('Ctrl Pts',(-0.0893215560848652,1.,4.17086566490794));
#59888=CARTESIAN_POINT('Ctrl Pts',(-0.0860600915549399,1.,4.17798698668094));
#59889=CARTESIAN_POINT('Ctrl Pts',(-0.0827644164385681,1.,4.18510195327123));
#59890=CARTESIAN_POINT('Ctrl Pts',(-0.0801005887114322,1.,4.19078883320504));
#59891=CARTESIAN_POINT('Ctrl Pts',(-0.07808739562424,1.,4.19505112859416));
#59892=CARTESIAN_POINT('Ctrl Pts',(-0.0767384596141467,1.,4.1978913862118));
#59893=CARTESIAN_POINT('Ctrl Pts',(-0.0760622897878249,1.,4.19931119685982));
#59894=CARTESIAN_POINT('Origin',(-0.0760622897878249,0.,4.19931119685982));
#59895=CARTESIAN_POINT('',(0.0760622897878233,1.,4.19931119685982));
#59896=CARTESIAN_POINT('Origin',(0.,0.,0.));
#59897=CARTESIAN_POINT('',(-0.385112848330762,1.,3.73017266276651));
#59898=CARTESIAN_POINT('Origin',(0.,1.,0.));
#59899=CARTESIAN_POINT('Ctrl Pts',(-0.385112848330762,1.,3.73017266276651));
#59900=CARTESIAN_POINT('Ctrl Pts',(-0.385112848330762,0.666666666666667,
3.73017266276651));
#59901=CARTESIAN_POINT('Ctrl Pts',(-0.385112848330762,0.333333333333333,
3.73017266276651));
#59902=CARTESIAN_POINT('Ctrl Pts',(-0.385112848330762,-0.333333333333333,
3.73017266276651));
#59903=CARTESIAN_POINT('Ctrl Pts',(-0.385112848330762,-0.666666666666667,
3.73017266276651));
#59904=CARTESIAN_POINT('Ctrl Pts',(-0.385112848330762,-1.,3.73017266276651));
#59905=CARTESIAN_POINT('Ctrl Pts',(-0.581791163835815,-1.,4.15950947128175));
#59906=CARTESIAN_POINT('Ctrl Pts',(-0.581791163835815,1.,4.15950947128175));
#59907=CARTESIAN_POINT('Ctrl Pts',(-0.580901211463535,-1.,4.1582129171283));
#59908=CARTESIAN_POINT('Ctrl Pts',(-0.580901211463535,1.,4.1582129171283));
#59909=CARTESIAN_POINT('Ctrl Pts',(-0.579124568914235,-1.,4.15561864788576));
#59910=CARTESIAN_POINT('Ctrl Pts',(-0.579124568914235,1.,4.15561864788576));
#59911=CARTESIAN_POINT('Ctrl Pts',(-0.576469391676688,-1.,4.151723761217));
#59912=CARTESIAN_POINT('Ctrl Pts',(-0.576469391676688,1.,4.151723761217));
#59913=CARTESIAN_POINT('Ctrl Pts',(-0.572948736069522,-1.,4.14652361068081));
#59914=CARTESIAN_POINT('Ctrl Pts',(-0.572948736069522,1.,4.14652361068081));
#59915=CARTESIAN_POINT('Ctrl Pts',(-0.568580610189775,-1.,4.14001179830547));
#59916=CARTESIAN_POINT('Ctrl Pts',(-0.568580610189775,1.,4.14001179830547));
#59917=CARTESIAN_POINT('Ctrl Pts',(-0.564245279537149,-1.,4.13348835727104));
#59918=CARTESIAN_POINT('Ctrl Pts',(-0.564245279537149,1.,4.13348835727104));
#59919=CARTESIAN_POINT('Ctrl Pts',(-0.559942890594774,-1.,4.12695329951961));
#59920=CARTESIAN_POINT('Ctrl Pts',(-0.559942890594774,1.,4.12695329951961));
#59921=CARTESIAN_POINT('Ctrl Pts',(-0.555673636129977,-1.,4.12040666195664));
#59922=CARTESIAN_POINT('Ctrl Pts',(-0.555673636129977,1.,4.12040666195664));
#59923=CARTESIAN_POINT('Ctrl Pts',(-0.551437758497033,-1.,4.11384852024721));
#59924=CARTESIAN_POINT('Ctrl Pts',(-0.551437758497033,1.,4.11384852024721));
#59925=CARTESIAN_POINT('Ctrl Pts',(-0.547235539485637,-1.,4.10727897027977));
#59926=CARTESIAN_POINT('Ctrl Pts',(-0.547235539485637,1.,4.10727897027977));
#59927=CARTESIAN_POINT('Ctrl Pts',(-0.543067286877757,-1.,4.10069810243979));
#59928=CARTESIAN_POINT('Ctrl Pts',(-0.543067286877757,1.,4.10069810243979));
#59929=CARTESIAN_POINT('Ctrl Pts',(-0.538933321179756,-1.,4.09410597627));
#59930=CARTESIAN_POINT('Ctrl Pts',(-0.538933321179756,1.,4.09410597627));
#59931=CARTESIAN_POINT('Ctrl Pts',(-0.534833963477273,-1.,4.08750259988885));
#59932=CARTESIAN_POINT('Ctrl Pts',(-0.534833963477273,1.,4.08750259988885));
#59933=CARTESIAN_POINT('Ctrl Pts',(-0.530769518728571,-1.,4.08088789536836));
#59934=CARTESIAN_POINT('Ctrl Pts',(-0.530769518728571,1.,4.08088789536836));
#59935=CARTESIAN_POINT('Ctrl Pts',(-0.526740277227498,-1.,4.07426172299847));
#59936=CARTESIAN_POINT('Ctrl Pts',(-0.526740277227498,1.,4.07426172299847));
#59937=CARTESIAN_POINT('Ctrl Pts',(-0.522746528603107,-1.,4.06762394471314));
#59938=CARTESIAN_POINT('Ctrl Pts',(-0.522746528603107,1.,4.06762394471314));
#59939=CARTESIAN_POINT('Ctrl Pts',(-0.518788572336924,-1.,4.06097448038013));
#59940=CARTESIAN_POINT('Ctrl Pts',(-0.518788572336924,1.,4.06097448038013));
#59941=CARTESIAN_POINT('Ctrl Pts',(-0.514866728193017,-1.,4.05431335771199));
#59942=CARTESIAN_POINT('Ctrl Pts',(-0.514866728193017,1.,4.05431335771199));
#59943=CARTESIAN_POINT('Ctrl Pts',(-0.51098134921897,-1.,4.04764078815447));
#59944=CARTESIAN_POINT('Ctrl Pts',(-0.51098134921897,1.,4.04764078815447));
#59945=CARTESIAN_POINT('Ctrl Pts',(-0.507132823288136,-1.,4.04095715148915));
#59946=CARTESIAN_POINT('Ctrl Pts',(-0.507132823288136,1.,4.04095715148915));
#59947=CARTESIAN_POINT('Ctrl Pts',(-0.503321556915346,-1.,4.03426284174272));
#59948=CARTESIAN_POINT('Ctrl Pts',(-0.503321556915346,1.,4.03426284174272));
#59949=CARTESIAN_POINT('Ctrl Pts',(-0.499547962340821,-1.,4.02755813980101));
#59950=CARTESIAN_POINT('Ctrl Pts',(-0.499547962340821,1.,4.02755813980101));
#59951=CARTESIAN_POINT('Ctrl Pts',(-0.495812444326251,-1.,4.02084308851832));
#59952=CARTESIAN_POINT('Ctrl Pts',(-0.495812444326251,1.,4.02084308851832));
#59953=CARTESIAN_POINT('Ctrl Pts',(-0.492115383418018,-1.,4.01411733503546));
#59954=CARTESIAN_POINT('Ctrl Pts',(-0.492115383418018,1.,4.01411733503546));
#59955=CARTESIAN_POINT('Ctrl Pts',(-0.488457130424633,-1.,4.0073800839099));
#59956=CARTESIAN_POINT('Ctrl Pts',(-0.488457130424633,1.,4.0073800839099));
#59957=CARTESIAN_POINT('Ctrl Pts',(-0.484838042421835,-1.,4.00063045119288));
#59958=CARTESIAN_POINT('Ctrl Pts',(-0.484838042421835,1.,4.00063045119288));
#59959=CARTESIAN_POINT('Ctrl Pts',(-0.481258512209675,-1.,3.99386775880679));
#59960=CARTESIAN_POINT('Ctrl Pts',(-0.481258512209675,1.,3.99386775880679));
#59961=CARTESIAN_POINT('Ctrl Pts',(-0.477718999122027,-1.,3.98709184306738));
#59962=CARTESIAN_POINT('Ctrl Pts',(-0.477718999122027,1.,3.98709184306738));
#59963=CARTESIAN_POINT('Ctrl Pts',(-0.47422006101951,-1.,3.98030338044409));
#59964=CARTESIAN_POINT('Ctrl Pts',(-0.47422006101951,1.,3.98030338044409));
#59965=CARTESIAN_POINT('Ctrl Pts',(-0.470762379613439,-1.,3.97350414289392));
#59966=CARTESIAN_POINT('Ctrl Pts',(-0.470762379613439,1.,3.97350414289392));
#59967=CARTESIAN_POINT('Ctrl Pts',(-0.467346690880643,-1.,3.9666962227393));
#59968=CARTESIAN_POINT('Ctrl Pts',(-0.467346690880643,1.,3.9666962227393));
#59969=CARTESIAN_POINT('Ctrl Pts',(-0.463973722115733,-1.,3.95988133243538));
#59970=CARTESIAN_POINT('Ctrl Pts',(-0.463973722115733,1.,3.95988133243538));
#59971=CARTESIAN_POINT('Ctrl Pts',(-0.460644124429121,-1.,3.95306005817364));
#59972=CARTESIAN_POINT('Ctrl Pts',(-0.460644124429121,1.,3.95306005817364));
#59973=CARTESIAN_POINT('Ctrl Pts',(-0.457358410451683,-1.,3.94623117206678));
#59974=CARTESIAN_POINT('Ctrl Pts',(-0.457358410451683,1.,3.94623117206678));
#59975=CARTESIAN_POINT('Ctrl Pts',(-0.454116879027584,-1.,3.93939080846298));
#59976=CARTESIAN_POINT('Ctrl Pts',(-0.454116879027584,1.,3.93939080846298));
#59977=CARTESIAN_POINT('Ctrl Pts',(-0.450919768356348,-1.,3.93253407403123));
#59978=CARTESIAN_POINT('Ctrl Pts',(-0.450919768356348,1.,3.93253407403123));
#59979=CARTESIAN_POINT('Ctrl Pts',(-0.447767416837293,-1.,3.92565674143416));
#59980=CARTESIAN_POINT('Ctrl Pts',(-0.447767416837293,1.,3.92565674143416));
#59981=CARTESIAN_POINT('Ctrl Pts',(-0.444660430230591,-1.,3.91875701610719));
#59982=CARTESIAN_POINT('Ctrl Pts',(-0.444660430230591,1.,3.91875701610719));
#59983=CARTESIAN_POINT('Ctrl Pts',(-0.441599824524054,-1.,3.91183704069153));
#59984=CARTESIAN_POINT('Ctrl Pts',(-0.441599824524054,1.,3.91183704069153));
#59985=CARTESIAN_POINT('Ctrl Pts',(-0.43858723545825,-1.,3.90490512938563));
#59986=CARTESIAN_POINT('Ctrl Pts',(-0.43858723545825,1.,3.90490512938563));
#59987=CARTESIAN_POINT('Ctrl Pts',(-0.435624629433528,-1.,3.89797256655462));
#59988=CARTESIAN_POINT('Ctrl Pts',(-0.435624629433528,1.,3.89797256655462));
#59989=CARTESIAN_POINT('Ctrl Pts',(-0.432713929544458,-1.,3.89104947940611));
#59990=CARTESIAN_POINT('Ctrl Pts',(-0.432713929544458,1.,3.89104947940611));
#59991=CARTESIAN_POINT('Ctrl Pts',(-0.429856640579741,-1.,3.88414070943341));
#59992=CARTESIAN_POINT('Ctrl Pts',(-0.429856640579741,1.,3.88414070943341));
#59993=CARTESIAN_POINT('Ctrl Pts',(-0.427053541173457,-1.,3.87724240306597));
#59994=CARTESIAN_POINT('Ctrl Pts',(-0.427053541173457,1.,3.87724240306597));
#59995=CARTESIAN_POINT('Ctrl Pts',(-0.424304173195111,-1.,3.87033643487851));
#59996=CARTESIAN_POINT('Ctrl Pts',(-0.424304173195111,1.,3.87033643487851));
#59997=CARTESIAN_POINT('Ctrl Pts',(-0.421607423177534,-1.,3.86339652542709));
#59998=CARTESIAN_POINT('Ctrl Pts',(-0.421607423177534,1.,3.86339652542709));
#59999=CARTESIAN_POINT('Ctrl Pts',(-0.418962468086773,-1.,3.85639825647996));
#60000=CARTESIAN_POINT('Ctrl Pts',(-0.418962468086773,1.,3.85639825647996));
#60001=CARTESIAN_POINT('Ctrl Pts',(-0.416369678052907,-1.,3.84932864157497));
#60002=CARTESIAN_POINT('Ctrl Pts',(-0.416369678052907,1.,3.84932864157497));
#60003=CARTESIAN_POINT('Ctrl Pts',(-0.413831367016748,-1.,3.84219403994762));
#60004=CARTESIAN_POINT('Ctrl Pts',(-0.413831367016748,1.,3.84219403994762));
#60005=CARTESIAN_POINT('Ctrl Pts',(-0.411353038798519,-1.,3.83503345578698));
#60006=CARTESIAN_POINT('Ctrl Pts',(-0.411353038798519,1.,3.83503345578698));
#60007=CARTESIAN_POINT('Ctrl Pts',(-0.40894237144746,-1.,3.82790724256471));
#60008=CARTESIAN_POINT('Ctrl Pts',(-0.40894237144746,1.,3.82790724256471));
#60009=CARTESIAN_POINT('Ctrl Pts',(-0.406607038258985,-1.,3.8208730391381));
#60010=CARTESIAN_POINT('Ctrl Pts',(-0.406607038258985,1.,3.8208730391381));
#60011=CARTESIAN_POINT('Ctrl Pts',(-0.404352694628273,-1.,3.81396374287793));
#60012=CARTESIAN_POINT('Ctrl Pts',(-0.404352694628273,1.,3.81396374287793));
#60013=CARTESIAN_POINT('Ctrl Pts',(-0.402181320148436,-1.,3.80716881962728));
#60014=CARTESIAN_POINT('Ctrl Pts',(-0.402181320148436,1.,3.80716881962728));
#60015=CARTESIAN_POINT('Ctrl Pts',(-0.4000883465046,-1.,3.80040370384546));
#60016=CARTESIAN_POINT('Ctrl Pts',(-0.4000883465046,1.,3.80040370384546));
#60017=CARTESIAN_POINT('Ctrl Pts',(-0.39806481868397,-1.,3.7935288716329));
#60018=CARTESIAN_POINT('Ctrl Pts',(-0.39806481868397,1.,3.7935288716329));
#60019=CARTESIAN_POINT('Ctrl Pts',(-0.396103205334841,-1.,3.78640521279313));
#60020=CARTESIAN_POINT('Ctrl Pts',(-0.396103205334841,1.,3.78640521279313));
#60021=CARTESIAN_POINT('Ctrl Pts',(-0.394202481011499,-1.,3.77894173114283));
#60022=CARTESIAN_POINT('Ctrl Pts',(-0.394202481011499,1.,3.77894173114283));
#60023=CARTESIAN_POINT('Ctrl Pts',(-0.392372786223433,-1.,3.77114011595967));
#60024=CARTESIAN_POINT('Ctrl Pts',(-0.392372786223433,1.,3.77114011595967));
#60025=CARTESIAN_POINT('Ctrl Pts',(-0.39064207297956,-1.,3.76315635033257));
#60026=CARTESIAN_POINT('Ctrl Pts',(-0.39064207297956,1.,3.76315635033257));
#60027=CARTESIAN_POINT('Ctrl Pts',(-0.389054775898702,-1.,3.75529302895152));
#60028=CARTESIAN_POINT('Ctrl Pts',(-0.389054775898702,1.,3.75529302895152));
#60029=CARTESIAN_POINT('Ctrl Pts',(-0.387663020050836,-1.,3.74792651696654));
#60030=CARTESIAN_POINT('Ctrl Pts',(-0.387663020050836,1.,3.74792651696654));
#60031=CARTESIAN_POINT('Ctrl Pts',(-0.386519576222251,-1.,3.74144965781276));
#60032=CARTESIAN_POINT('Ctrl Pts',(-0.386519576222251,1.,3.74144965781276));
#60033=CARTESIAN_POINT('Ctrl Pts',(-0.385670806454566,-1.,3.73621371845318));
#60034=CARTESIAN_POINT('Ctrl Pts',(-0.385670806454566,1.,3.73621371845318));
#60035=CARTESIAN_POINT('Ctrl Pts',(-0.385147887988951,-1.,3.73245705638843));
#60036=CARTESIAN_POINT('Ctrl Pts',(-0.385147887988951,1.,3.73245705638843));
#60037=CARTESIAN_POINT('Ctrl Pts',(-0.385001870183213,-1.,3.73072465900175));
#60038=CARTESIAN_POINT('Ctrl Pts',(-0.385001870183213,1.,3.73072465900175));
#60039=CARTESIAN_POINT('Ctrl Pts',(-0.385047711603462,-1.,3.73015851028356));
#60040=CARTESIAN_POINT('Ctrl Pts',(-0.385047711603462,1.,3.73015851028356));
#60041=CARTESIAN_POINT('Ctrl Pts',(-0.385147278814642,-1.,3.73010668803042));
#60042=CARTESIAN_POINT('Ctrl Pts',(-0.385147278814642,1.,3.73010668803042));
#60043=CARTESIAN_POINT('Ctrl Pts',(-0.38521431477633,-1.,3.73016218570874));
#60044=CARTESIAN_POINT('Ctrl Pts',(-0.38521431477633,1.,3.73016218570874));
#60045=CARTESIAN_POINT('',(-0.581791163835815,1.,4.15950947128175));
#60046=CARTESIAN_POINT('Ctrl Pts',(-0.581791163835815,1.,4.15950947128175));
#60047=CARTESIAN_POINT('Ctrl Pts',(-0.580901211463535,1.,4.1582129171283));
#60048=CARTESIAN_POINT('Ctrl Pts',(-0.579124568914235,1.,4.15561864788576));
#60049=CARTESIAN_POINT('Ctrl Pts',(-0.576469391676688,1.,4.151723761217));
#60050=CARTESIAN_POINT('Ctrl Pts',(-0.572948736069522,1.,4.14652361068081));
#60051=CARTESIAN_POINT('Ctrl Pts',(-0.568580610189775,1.,4.14001179830547));
#60052=CARTESIAN_POINT('Ctrl Pts',(-0.564245279537149,1.,4.13348835727104));
#60053=CARTESIAN_POINT('Ctrl Pts',(-0.559942890594774,1.,4.12695329951961));
#60054=CARTESIAN_POINT('Ctrl Pts',(-0.555673636129977,1.,4.12040666195664));
#60055=CARTESIAN_POINT('Ctrl Pts',(-0.551437758497033,1.,4.11384852024721));
#60056=CARTESIAN_POINT('Ctrl Pts',(-0.547235539485637,1.,4.10727897027977));
#60057=CARTESIAN_POINT('Ctrl Pts',(-0.543067286877757,1.,4.10069810243979));
#60058=CARTESIAN_POINT('Ctrl Pts',(-0.538933321179756,1.,4.09410597627));
#60059=CARTESIAN_POINT('Ctrl Pts',(-0.534833963477273,1.,4.08750259988885));
#60060=CARTESIAN_POINT('Ctrl Pts',(-0.530769518728571,1.,4.08088789536836));
#60061=CARTESIAN_POINT('Ctrl Pts',(-0.526740277227498,1.,4.07426172299847));
#60062=CARTESIAN_POINT('Ctrl Pts',(-0.522746528603107,1.,4.06762394471314));
#60063=CARTESIAN_POINT('Ctrl Pts',(-0.518788572336924,1.,4.06097448038013));
#60064=CARTESIAN_POINT('Ctrl Pts',(-0.514866728193017,1.,4.05431335771199));
#60065=CARTESIAN_POINT('Ctrl Pts',(-0.51098134921897,1.,4.04764078815447));
#60066=CARTESIAN_POINT('Ctrl Pts',(-0.507132823288136,1.,4.04095715148915));
#60067=CARTESIAN_POINT('Ctrl Pts',(-0.503321556915346,1.,4.03426284174272));
#60068=CARTESIAN_POINT('Ctrl Pts',(-0.499547962340821,1.,4.02755813980101));
#60069=CARTESIAN_POINT('Ctrl Pts',(-0.495812444326251,1.,4.02084308851832));
#60070=CARTESIAN_POINT('Ctrl Pts',(-0.492115383418018,1.,4.01411733503546));
#60071=CARTESIAN_POINT('Ctrl Pts',(-0.488457130424633,1.,4.0073800839099));
#60072=CARTESIAN_POINT('Ctrl Pts',(-0.484838042421835,1.,4.00063045119288));
#60073=CARTESIAN_POINT('Ctrl Pts',(-0.481258512209675,1.,3.99386775880679));
#60074=CARTESIAN_POINT('Ctrl Pts',(-0.477718999122027,1.,3.98709184306738));
#60075=CARTESIAN_POINT('Ctrl Pts',(-0.47422006101951,1.,3.98030338044409));
#60076=CARTESIAN_POINT('Ctrl Pts',(-0.470762379613439,1.,3.97350414289392));
#60077=CARTESIAN_POINT('Ctrl Pts',(-0.467346690880643,1.,3.9666962227393));
#60078=CARTESIAN_POINT('Ctrl Pts',(-0.463973722115733,1.,3.95988133243538));
#60079=CARTESIAN_POINT('Ctrl Pts',(-0.460644124429121,1.,3.95306005817364));
#60080=CARTESIAN_POINT('Ctrl Pts',(-0.457358410451683,1.,3.94623117206678));
#60081=CARTESIAN_POINT('Ctrl Pts',(-0.454116879027584,1.,3.93939080846298));
#60082=CARTESIAN_POINT('Ctrl Pts',(-0.450919768356348,1.,3.93253407403123));
#60083=CARTESIAN_POINT('Ctrl Pts',(-0.447767416837293,1.,3.92565674143416));
#60084=CARTESIAN_POINT('Ctrl Pts',(-0.444660430230591,1.,3.91875701610719));
#60085=CARTESIAN_POINT('Ctrl Pts',(-0.441599824524054,1.,3.91183704069153));
#60086=CARTESIAN_POINT('Ctrl Pts',(-0.43858723545825,1.,3.90490512938563));
#60087=CARTESIAN_POINT('Ctrl Pts',(-0.435624629433528,1.,3.89797256655462));
#60088=CARTESIAN_POINT('Ctrl Pts',(-0.432713929544458,1.,3.89104947940611));
#60089=CARTESIAN_POINT('Ctrl Pts',(-0.429856640579741,1.,3.88414070943341));
#60090=CARTESIAN_POINT('Ctrl Pts',(-0.427053541173457,1.,3.87724240306597));
#60091=CARTESIAN_POINT('Ctrl Pts',(-0.424304173195111,1.,3.87033643487851));
#60092=CARTESIAN_POINT('Ctrl Pts',(-0.421607423177534,1.,3.86339652542709));
#60093=CARTESIAN_POINT('Ctrl Pts',(-0.418962468086773,1.,3.85639825647996));
#60094=CARTESIAN_POINT('Ctrl Pts',(-0.416369678052907,1.,3.84932864157497));
#60095=CARTESIAN_POINT('Ctrl Pts',(-0.413831367016748,1.,3.84219403994762));
#60096=CARTESIAN_POINT('Ctrl Pts',(-0.411353038798519,1.,3.83503345578698));
#60097=CARTESIAN_POINT('Ctrl Pts',(-0.40894237144746,1.,3.82790724256471));
#60098=CARTESIAN_POINT('Ctrl Pts',(-0.406607038258985,1.,3.8208730391381));
#60099=CARTESIAN_POINT('Ctrl Pts',(-0.404352694628273,1.,3.81396374287793));
#60100=CARTESIAN_POINT('Ctrl Pts',(-0.402181320148436,1.,3.80716881962728));
#60101=CARTESIAN_POINT('Ctrl Pts',(-0.4000883465046,1.,3.80040370384546));
#60102=CARTESIAN_POINT('Ctrl Pts',(-0.39806481868397,1.,3.7935288716329));
#60103=CARTESIAN_POINT('Ctrl Pts',(-0.396103205334841,1.,3.78640521279313));
#60104=CARTESIAN_POINT('Ctrl Pts',(-0.394202481011499,1.,3.77894173114283));
#60105=CARTESIAN_POINT('Ctrl Pts',(-0.392372786223433,1.,3.77114011595967));
#60106=CARTESIAN_POINT('Ctrl Pts',(-0.39064207297956,1.,3.76315635033257));
#60107=CARTESIAN_POINT('Ctrl Pts',(-0.389054775898702,1.,3.75529302895152));
#60108=CARTESIAN_POINT('Ctrl Pts',(-0.387663020050836,1.,3.74792651696654));
#60109=CARTESIAN_POINT('Ctrl Pts',(-0.386519576222251,1.,3.74144965781276));
#60110=CARTESIAN_POINT('Ctrl Pts',(-0.385670806454566,1.,3.73621371845318));
#60111=CARTESIAN_POINT('Ctrl Pts',(-0.385187124634206,1.,3.73273893363406));
#60112=CARTESIAN_POINT('Ctrl Pts',(-0.385031656499164,1.,3.73106082862548));
#60113=CARTESIAN_POINT('Ctrl Pts',(-0.385037797881504,1.,3.73040527621055));
#60114=CARTESIAN_POINT('Ctrl Pts',(-0.385087139000375,1.,3.73021431755274));
#60115=CARTESIAN_POINT('Ctrl Pts',(-0.385112848330762,1.,3.73017266276651));
#60116=CARTESIAN_POINT('',(-0.581791163835815,0.,4.15950947128175));
#60117=CARTESIAN_POINT('Ctrl Pts',(-0.7863229229206,-1.,3.66663282329846));
#60118=CARTESIAN_POINT('Ctrl Pts',(-0.7863229229206,1.,3.66663282329846));
#60119=CARTESIAN_POINT('Ctrl Pts',(-0.786369528183326,-1.,3.66655932661986));
#60120=CARTESIAN_POINT('Ctrl Pts',(-0.786369528183326,1.,3.66655932661986));
#60121=CARTESIAN_POINT('Ctrl Pts',(-0.786480236185697,-1.,3.66657784455334));
#60122=CARTESIAN_POINT('Ctrl Pts',(-0.786480236185697,1.,3.66657784455334));
#60123=CARTESIAN_POINT('Ctrl Pts',(-0.786698783542764,-1.,3.66710211820482));
#60124=CARTESIAN_POINT('Ctrl Pts',(-0.786698783542764,1.,3.66710211820482));
#60125=CARTESIAN_POINT('Ctrl Pts',(-0.787095252590501,-1.,3.66879484801113));
#60126=CARTESIAN_POINT('Ctrl Pts',(-0.787095252590501,1.,3.66879484801113));
#60127=CARTESIAN_POINT('Ctrl Pts',(-0.787758799995743,-1.,3.67252923663655));
#60128=CARTESIAN_POINT('Ctrl Pts',(-0.787758799995743,1.,3.67252923663655));
#60129=CARTESIAN_POINT('Ctrl Pts',(-0.788569566220285,-1.,3.67777119516252));
#60130=CARTESIAN_POINT('Ctrl Pts',(-0.788569566220285,1.,3.67777119516252));
#60131=CARTESIAN_POINT('Ctrl Pts',(-0.789483546064387,-1.,3.68428439783905));
#60132=CARTESIAN_POINT('Ctrl Pts',(-0.789483546064387,1.,3.68428439783905));
#60133=CARTESIAN_POINT('Ctrl Pts',(-0.790436284988788,-1.,3.69172044327364));
#60134=CARTESIAN_POINT('Ctrl Pts',(-0.790436284988788,1.,3.69172044327364));
#60135=CARTESIAN_POINT('Ctrl Pts',(-0.79135657569598,-1.,3.69968940808721));
#60136=CARTESIAN_POINT('Ctrl Pts',(-0.79135657569598,1.,3.69968940808721));
#60137=CARTESIAN_POINT('Ctrl Pts',(-0.792177688845818,-1.,3.70781724021806));
#60138=CARTESIAN_POINT('Ctrl Pts',(-0.792177688845818,1.,3.70781724021806));
#60139=CARTESIAN_POINT('Ctrl Pts',(-0.792848377370287,-1.,3.71580242396124));
#60140=CARTESIAN_POINT('Ctrl Pts',(-0.792848377370287,1.,3.71580242396124));
#60141=CARTESIAN_POINT('Ctrl Pts',(-0.793347023784205,-1.,3.72348797293734));
#60142=CARTESIAN_POINT('Ctrl Pts',(-0.793347023784205,1.,3.72348797293734));
#60143=CARTESIAN_POINT('Ctrl Pts',(-0.793682750269684,-1.,3.73086914695805));
#60144=CARTESIAN_POINT('Ctrl Pts',(-0.793682750269684,1.,3.73086914695805));
#60145=CARTESIAN_POINT('Ctrl Pts',(-0.793882700937017,-1.,3.73803280541687));
#60146=CARTESIAN_POINT('Ctrl Pts',(-0.793882700937017,1.,3.73803280541687));
#60147=CARTESIAN_POINT('Ctrl Pts',(-0.793982700459952,-1.,3.74511357728861));
#60148=CARTESIAN_POINT('Ctrl Pts',(-0.793982700459952,1.,3.74511357728861));
#60149=CARTESIAN_POINT('Ctrl Pts',(-0.794017347371377,-1.,3.75224692493864));
#60150=CARTESIAN_POINT('Ctrl Pts',(-0.794017347371377,1.,3.75224692493864));
#60151=CARTESIAN_POINT('Ctrl Pts',(-0.794008429134907,-1.,3.75951468666257));
#60152=CARTESIAN_POINT('Ctrl Pts',(-0.794008429134907,1.,3.75951468666257));
#60153=CARTESIAN_POINT('Ctrl Pts',(-0.793961083688992,-1.,3.76692626931111));
#60154=CARTESIAN_POINT('Ctrl Pts',(-0.793961083688992,1.,3.76692626931111));
#60155=CARTESIAN_POINT('Ctrl Pts',(-0.793870523787408,-1.,3.77444863801212));
#60156=CARTESIAN_POINT('Ctrl Pts',(-0.793870523787408,1.,3.77444863801212));
#60157=CARTESIAN_POINT('Ctrl Pts',(-0.7937262357813,-1.,3.78202460377598));
#60158=CARTESIAN_POINT('Ctrl Pts',(-0.7937262357813,1.,3.78202460377598));
#60159=CARTESIAN_POINT('Ctrl Pts',(-0.793516871680993,-1.,3.78959439439235));
#60160=CARTESIAN_POINT('Ctrl Pts',(-0.793516871680993,1.,3.78959439439235));
#60161=CARTESIAN_POINT('Ctrl Pts',(-0.793235612973273,-1.,3.79711921389897));
#60162=CARTESIAN_POINT('Ctrl Pts',(-0.793235612973273,1.,3.79711921389897));
#60163=CARTESIAN_POINT('Ctrl Pts',(-0.792882695234778,-1.,3.80459229925637));
#60164=CARTESIAN_POINT('Ctrl Pts',(-0.792882695234778,1.,3.80459229925637));
#60165=CARTESIAN_POINT('Ctrl Pts',(-0.792462483517634,-1.,3.81202588694756));
#60166=CARTESIAN_POINT('Ctrl Pts',(-0.792462483517634,1.,3.81202588694756));
#60167=CARTESIAN_POINT('Ctrl Pts',(-0.791981740718635,-1.,3.81944345442249));
#60168=CARTESIAN_POINT('Ctrl Pts',(-0.791981740718635,1.,3.81944345442249));
#60169=CARTESIAN_POINT('Ctrl Pts',(-0.791447528662369,-1.,3.82687033899792));
#60170=CARTESIAN_POINT('Ctrl Pts',(-0.791447528662369,1.,3.82687033899792));
#60171=CARTESIAN_POINT('Ctrl Pts',(-0.790865012705301,-1.,3.83432392054786));
#60172=CARTESIAN_POINT('Ctrl Pts',(-0.790865012705301,1.,3.83432392054786));
#60173=CARTESIAN_POINT('Ctrl Pts',(-0.790236124191242,-1.,3.84180762342454));
#60174=CARTESIAN_POINT('Ctrl Pts',(-0.790236124191242,1.,3.84180762342454));
#60175=CARTESIAN_POINT('Ctrl Pts',(-0.789560798155582,-1.,3.84931637808894));
#60176=CARTESIAN_POINT('Ctrl Pts',(-0.789560798155582,1.,3.84931637808894));
#60177=CARTESIAN_POINT('Ctrl Pts',(-0.788837734090672,-1.,3.85683995872529));
#60178=CARTESIAN_POINT('Ctrl Pts',(-0.788837734090672,1.,3.85683995872529));
#60179=CARTESIAN_POINT('Ctrl Pts',(-0.788065315093778,-1.,3.86436702561345));
#60180=CARTESIAN_POINT('Ctrl Pts',(-0.788065315093778,1.,3.86436702561345));
#60181=CARTESIAN_POINT('Ctrl Pts',(-0.787242527617999,-1.,3.87188916600912));
#60182=CARTESIAN_POINT('Ctrl Pts',(-0.787242527617999,1.,3.87188916600912));
#60183=CARTESIAN_POINT('Ctrl Pts',(-0.786369675812609,-1.,3.8794040281819));
#60184=CARTESIAN_POINT('Ctrl Pts',(-0.786369675812609,1.,3.8794040281819));
#60185=CARTESIAN_POINT('Ctrl Pts',(-0.78544789034073,-1.,3.88691313167398));
#60186=CARTESIAN_POINT('Ctrl Pts',(-0.78544789034073,1.,3.88691313167398));
#60187=CARTESIAN_POINT('Ctrl Pts',(-0.784478799358336,-1.,3.89442039235103));
#60188=CARTESIAN_POINT('Ctrl Pts',(-0.784478799358336,1.,3.89442039235103));
#60189=CARTESIAN_POINT('Ctrl Pts',(-0.783464141529081,-1.,3.9019303904397));
#60190=CARTESIAN_POINT('Ctrl Pts',(-0.783464141529081,1.,3.9019303904397));
#60191=CARTESIAN_POINT('Ctrl Pts',(-0.782405395622764,-1.,3.90944671004542));
#60192=CARTESIAN_POINT('Ctrl Pts',(-0.782405395622764,1.,3.90944671004542));
#60193=CARTESIAN_POINT('Ctrl Pts',(-0.781303428618367,-1.,3.91697036054676));
#60194=CARTESIAN_POINT('Ctrl Pts',(-0.781303428618367,1.,3.91697036054676));
#60195=CARTESIAN_POINT('Ctrl Pts',(-0.780158678615543,-1.,3.92450058323823));
#60196=CARTESIAN_POINT('Ctrl Pts',(-0.780158678615543,1.,3.92450058323823));
#60197=CARTESIAN_POINT('Ctrl Pts',(-0.778971308134821,-1.,3.93203552473174));
#60198=CARTESIAN_POINT('Ctrl Pts',(-0.778971308134821,1.,3.93203552473174));
#60199=CARTESIAN_POINT('Ctrl Pts',(-0.777741370568559,-1.,3.93957296768103));
#60200=CARTESIAN_POINT('Ctrl Pts',(-0.777741370568559,1.,3.93957296768103));
#60201=CARTESIAN_POINT('Ctrl Pts',(-0.776468966697921,-1.,3.94711101619447));
#60202=CARTESIAN_POINT('Ctrl Pts',(-0.776468966697921,1.,3.94711101619447));
#60203=CARTESIAN_POINT('Ctrl Pts',(-0.775154418039352,-1.,3.9546488545231));
#60204=CARTESIAN_POINT('Ctrl Pts',(-0.775154418039352,1.,3.9546488545231));
#60205=CARTESIAN_POINT('Ctrl Pts',(-0.773798212026566,-1.,3.96218649639807));
#60206=CARTESIAN_POINT('Ctrl Pts',(-0.773798212026566,1.,3.96218649639807));
#60207=CARTESIAN_POINT('Ctrl Pts',(-0.772400931772136,-1.,3.96972446532772));
#60208=CARTESIAN_POINT('Ctrl Pts',(-0.772400931772136,1.,3.96972446532772));
#60209=CARTESIAN_POINT('Ctrl Pts',(-0.770963190030471,-1.,3.97726349165488));
#60210=CARTESIAN_POINT('Ctrl Pts',(-0.770963190030471,1.,3.97726349165488));
#60211=CARTESIAN_POINT('Ctrl Pts',(-0.769485566245544,-1.,3.98480422348451));
#60212=CARTESIAN_POINT('Ctrl Pts',(-0.769485566245544,1.,3.98480422348451));
#60213=CARTESIAN_POINT('Ctrl Pts',(-0.767968531377915,-1.,3.9923468788101));
#60214=CARTESIAN_POINT('Ctrl Pts',(-0.767968531377915,1.,3.9923468788101));
#60215=CARTESIAN_POINT('Ctrl Pts',(-0.766412457136064,-1.,3.99989129179622));
#60216=CARTESIAN_POINT('Ctrl Pts',(-0.766412457136064,1.,3.99989129179622));
#60217=CARTESIAN_POINT('Ctrl Pts',(-0.764817648785198,-1.,4.00743706791509));
#60218=CARTESIAN_POINT('Ctrl Pts',(-0.764817648785198,1.,4.00743706791509));
#60219=CARTESIAN_POINT('Ctrl Pts',(-0.763184371182935,-1.,4.01498370680496));
#60220=CARTESIAN_POINT('Ctrl Pts',(-0.763184371182935,1.,4.01498370680496));
#60221=CARTESIAN_POINT('Ctrl Pts',(-0.761512875859804,-1.,4.02253072741268));
#60222=CARTESIAN_POINT('Ctrl Pts',(-0.761512875859804,1.,4.02253072741268));
#60223=CARTESIAN_POINT('Ctrl Pts',(-0.759803433243752,-1.,4.03007781954412));
#60224=CARTESIAN_POINT('Ctrl Pts',(-0.759803433243752,1.,4.03007781954412));
#60225=CARTESIAN_POINT('Ctrl Pts',(-0.758056338884944,-1.,4.03762485803119));
#60226=CARTESIAN_POINT('Ctrl Pts',(-0.758056338884944,1.,4.03762485803119));
#60227=CARTESIAN_POINT('Ctrl Pts',(-0.756271902369581,-1.,4.04517182653997));
#60228=CARTESIAN_POINT('Ctrl Pts',(-0.756271902369581,1.,4.04517182653997));
#60229=CARTESIAN_POINT('Ctrl Pts',(-0.754450441816078,-1.,4.05271876687915));
#60230=CARTESIAN_POINT('Ctrl Pts',(-0.754450441816078,1.,4.05271876687915));
#60231=CARTESIAN_POINT('Ctrl Pts',(-0.752592276483072,-1.,4.06026572221515));
#60232=CARTESIAN_POINT('Ctrl Pts',(-0.752592276483072,1.,4.06026572221515));
#60233=CARTESIAN_POINT('Ctrl Pts',(-0.750697720484036,-1.,4.06781267242378));
#60234=CARTESIAN_POINT('Ctrl Pts',(-0.750697720484036,1.,4.06781267242378));
#60235=CARTESIAN_POINT('Ctrl Pts',(-0.748767076680557,-1.,4.07535951056152));
#60236=CARTESIAN_POINT('Ctrl Pts',(-0.748767076680557,1.,4.07535951056152));
#60237=CARTESIAN_POINT('Ctrl Pts',(-0.746800631492315,-1.,4.08290608095642));
#60238=CARTESIAN_POINT('Ctrl Pts',(-0.746800631492315,1.,4.08290608095642));
#60239=CARTESIAN_POINT('Ctrl Pts',(-0.7447986497065,-1.,4.09045220253573));
#60240=CARTESIAN_POINT('Ctrl Pts',(-0.7447986497065,1.,4.09045220253573));
#60241=CARTESIAN_POINT('Ctrl Pts',(-0.742761369689841,-1.,4.09799769702611));
#60242=CARTESIAN_POINT('Ctrl Pts',(-0.742761369689841,1.,4.09799769702611));
#60243=CARTESIAN_POINT('Ctrl Pts',(-0.740688998553377,-1.,4.10554241757547));
#60244=CARTESIAN_POINT('Ctrl Pts',(-0.740688998553377,1.,4.10554241757547));
#60245=CARTESIAN_POINT('Ctrl Pts',(-0.738581708225844,-1.,4.11308626951927));
#60246=CARTESIAN_POINT('Ctrl Pts',(-0.738581708225844,1.,4.11308626951927));
#60247=CARTESIAN_POINT('Ctrl Pts',(-0.736439634331345,-1.,4.120629196238));
#60248=CARTESIAN_POINT('Ctrl Pts',(-0.736439634331345,1.,4.120629196238));
#60249=CARTESIAN_POINT('Ctrl Pts',(-0.734698226764092,-1.,4.12666277570844));
#60250=CARTESIAN_POINT('Ctrl Pts',(-0.734698226764092,1.,4.12666277570844));
#60251=CARTESIAN_POINT('Ctrl Pts',(-0.733376589323546,-1.,4.13118752795207));
#60252=CARTESIAN_POINT('Ctrl Pts',(-0.733376589323546,1.,4.13118752795207));
#60253=CARTESIAN_POINT('Ctrl Pts',(-0.73248857513516,-1.,4.1342038373684));
#60254=CARTESIAN_POINT('Ctrl Pts',(-0.73248857513516,1.,4.1342038373684));
#60255=CARTESIAN_POINT('Ctrl Pts',(-0.73204283740062,-1.,4.13571194405636));
#60256=CARTESIAN_POINT('Ctrl Pts',(-0.73204283740062,1.,4.13571194405636));
#60257=CARTESIAN_POINT('',(-0.786422660831985,1.,3.66661143271685));
#60258=CARTESIAN_POINT('Ctrl Pts',(-0.786422660831985,-1.,3.66661143271685));
#60259=CARTESIAN_POINT('Ctrl Pts',(-0.786422660831985,-0.666666666666667,
3.66661143271685));
#60260=CARTESIAN_POINT('Ctrl Pts',(-0.786422660831985,-0.333333333333333,
3.66661143271685));
#60261=CARTESIAN_POINT('Ctrl Pts',(-0.786422660831985,0.333333333333333,
3.66661143271685));
#60262=CARTESIAN_POINT('Ctrl Pts',(-0.786422660831985,0.666666666666667,
3.66661143271685));
#60263=CARTESIAN_POINT('Ctrl Pts',(-0.786422660831985,1.,3.66661143271685));
#60264=CARTESIAN_POINT('',(-0.73204283740062,1.,4.13571194405636));
#60265=CARTESIAN_POINT('',(-0.73204283740062,0.,4.13571194405636));
#60266=CARTESIAN_POINT('Ctrl Pts',(-0.786422660831985,1.,3.66661143271685));
#60267=CARTESIAN_POINT('Ctrl Pts',(-0.786459983895432,1.,3.6666431041522));
#60268=CARTESIAN_POINT('Ctrl Pts',(-0.786565919558984,1.,3.66680946938292));
#60269=CARTESIAN_POINT('Ctrl Pts',(-0.786774337198062,1.,3.66743103898702));
#60270=CARTESIAN_POINT('Ctrl Pts',(-0.787145041181546,1.,3.66907505398677));
#60271=CARTESIAN_POINT('Ctrl Pts',(-0.787758799995743,1.,3.67252923663655));
#60272=CARTESIAN_POINT('Ctrl Pts',(-0.788569566220285,1.,3.67777119516252));
#60273=CARTESIAN_POINT('Ctrl Pts',(-0.789483546064387,1.,3.68428439783905));
#60274=CARTESIAN_POINT('Ctrl Pts',(-0.790436284988788,1.,3.69172044327364));
#60275=CARTESIAN_POINT('Ctrl Pts',(-0.79135657569598,1.,3.69968940808721));
#60276=CARTESIAN_POINT('Ctrl Pts',(-0.792177688845818,1.,3.70781724021806));
#60277=CARTESIAN_POINT('Ctrl Pts',(-0.792848377370287,1.,3.71580242396124));
#60278=CARTESIAN_POINT('Ctrl Pts',(-0.793347023784205,1.,3.72348797293734));
#60279=CARTESIAN_POINT('Ctrl Pts',(-0.793682750269684,1.,3.73086914695805));
#60280=CARTESIAN_POINT('Ctrl Pts',(-0.793882700937017,1.,3.73803280541687));
#60281=CARTESIAN_POINT('Ctrl Pts',(-0.793982700459952,1.,3.74511357728861));
#60282=CARTESIAN_POINT('Ctrl Pts',(-0.794017347371377,1.,3.75224692493864));
#60283=CARTESIAN_POINT('Ctrl Pts',(-0.794008429134907,1.,3.75951468666257));
#60284=CARTESIAN_POINT('Ctrl Pts',(-0.793961083688992,1.,3.76692626931111));
#60285=CARTESIAN_POINT('Ctrl Pts',(-0.793870523787408,1.,3.77444863801212));
#60286=CARTESIAN_POINT('Ctrl Pts',(-0.7937262357813,1.,3.78202460377598));
#60287=CARTESIAN_POINT('Ctrl Pts',(-0.793516871680993,1.,3.78959439439235));
#60288=CARTESIAN_POINT('Ctrl Pts',(-0.793235612973273,1.,3.79711921389897));
#60289=CARTESIAN_POINT('Ctrl Pts',(-0.792882695234778,1.,3.80459229925637));
#60290=CARTESIAN_POINT('Ctrl Pts',(-0.792462483517634,1.,3.81202588694756));
#60291=CARTESIAN_POINT('Ctrl Pts',(-0.791981740718635,1.,3.81944345442249));
#60292=CARTESIAN_POINT('Ctrl Pts',(-0.791447528662369,1.,3.82687033899792));
#60293=CARTESIAN_POINT('Ctrl Pts',(-0.790865012705301,1.,3.83432392054786));
#60294=CARTESIAN_POINT('Ctrl Pts',(-0.790236124191242,1.,3.84180762342454));
#60295=CARTESIAN_POINT('Ctrl Pts',(-0.789560798155582,1.,3.84931637808894));
#60296=CARTESIAN_POINT('Ctrl Pts',(-0.788837734090672,1.,3.85683995872529));
#60297=CARTESIAN_POINT('Ctrl Pts',(-0.788065315093778,1.,3.86436702561345));
#60298=CARTESIAN_POINT('Ctrl Pts',(-0.787242527617999,1.,3.87188916600912));
#60299=CARTESIAN_POINT('Ctrl Pts',(-0.786369675812609,1.,3.8794040281819));
#60300=CARTESIAN_POINT('Ctrl Pts',(-0.78544789034073,1.,3.88691313167398));
#60301=CARTESIAN_POINT('Ctrl Pts',(-0.784478799358336,1.,3.89442039235103));
#60302=CARTESIAN_POINT('Ctrl Pts',(-0.783464141529081,1.,3.9019303904397));
#60303=CARTESIAN_POINT('Ctrl Pts',(-0.782405395622764,1.,3.90944671004542));
#60304=CARTESIAN_POINT('Ctrl Pts',(-0.781303428618367,1.,3.91697036054676));
#60305=CARTESIAN_POINT('Ctrl Pts',(-0.780158678615543,1.,3.92450058323823));
#60306=CARTESIAN_POINT('Ctrl Pts',(-0.778971308134821,1.,3.93203552473174));
#60307=CARTESIAN_POINT('Ctrl Pts',(-0.777741370568559,1.,3.93957296768103));
#60308=CARTESIAN_POINT('Ctrl Pts',(-0.776468966697921,1.,3.94711101619447));
#60309=CARTESIAN_POINT('Ctrl Pts',(-0.775154418039352,1.,3.9546488545231));
#60310=CARTESIAN_POINT('Ctrl Pts',(-0.773798212026566,1.,3.96218649639807));
#60311=CARTESIAN_POINT('Ctrl Pts',(-0.772400931772136,1.,3.96972446532772));
#60312=CARTESIAN_POINT('Ctrl Pts',(-0.770963190030471,1.,3.97726349165488));
#60313=CARTESIAN_POINT('Ctrl Pts',(-0.769485566245544,1.,3.98480422348451));
#60314=CARTESIAN_POINT('Ctrl Pts',(-0.767968531377915,1.,3.9923468788101));
#60315=CARTESIAN_POINT('Ctrl Pts',(-0.766412457136064,1.,3.99989129179622));
#60316=CARTESIAN_POINT('Ctrl Pts',(-0.764817648785198,1.,4.00743706791509));
#60317=CARTESIAN_POINT('Ctrl Pts',(-0.763184371182935,1.,4.01498370680496));
#60318=CARTESIAN_POINT('Ctrl Pts',(-0.761512875859804,1.,4.02253072741268));
#60319=CARTESIAN_POINT('Ctrl Pts',(-0.759803433243752,1.,4.03007781954412));
#60320=CARTESIAN_POINT('Ctrl Pts',(-0.758056338884944,1.,4.03762485803119));
#60321=CARTESIAN_POINT('Ctrl Pts',(-0.756271902369581,1.,4.04517182653997));
#60322=CARTESIAN_POINT('Ctrl Pts',(-0.754450441816078,1.,4.05271876687915));
#60323=CARTESIAN_POINT('Ctrl Pts',(-0.752592276483072,1.,4.06026572221515));
#60324=CARTESIAN_POINT('Ctrl Pts',(-0.750697720484036,1.,4.06781267242378));
#60325=CARTESIAN_POINT('Ctrl Pts',(-0.748767076680557,1.,4.07535951056152));
#60326=CARTESIAN_POINT('Ctrl Pts',(-0.746800631492315,1.,4.08290608095642));
#60327=CARTESIAN_POINT('Ctrl Pts',(-0.7447986497065,1.,4.09045220253573));
#60328=CARTESIAN_POINT('Ctrl Pts',(-0.742761369689841,1.,4.09799769702611));
#60329=CARTESIAN_POINT('Ctrl Pts',(-0.740688998553377,1.,4.10554241757547));
#60330=CARTESIAN_POINT('Ctrl Pts',(-0.738581708225844,1.,4.11308626951927));
#60331=CARTESIAN_POINT('Ctrl Pts',(-0.736439634331345,1.,4.120629196238));
#60332=CARTESIAN_POINT('Ctrl Pts',(-0.734698226764092,1.,4.12666277570844));
#60333=CARTESIAN_POINT('Ctrl Pts',(-0.733376589323546,1.,4.13118752795207));
#60334=CARTESIAN_POINT('Ctrl Pts',(-0.73248857513516,1.,4.1342038373684));
#60335=CARTESIAN_POINT('Ctrl Pts',(-0.73204283740062,1.,4.13571194405636));
#60336=CARTESIAN_POINT('Origin',(-0.73204283740062,0.,4.13571194405636));
#60337=CARTESIAN_POINT('',(-0.581791163835815,1.,4.15950947128175));
#60338=CARTESIAN_POINT('Origin',(0.,0.,0.));
#60339=CARTESIAN_POINT('',(-0.963899035117249,1.,3.62400312501245));
#60340=CARTESIAN_POINT('Origin',(0.,1.,0.));
#60341=CARTESIAN_POINT('Ctrl Pts',(-0.963899035117249,1.,3.62400312501245));
#60342=CARTESIAN_POINT('Ctrl Pts',(-0.963899035117249,0.666666666666667,
3.62400312501245));
#60343=CARTESIAN_POINT('Ctrl Pts',(-0.963899035117249,0.333333333333333,
3.62400312501245));
#60344=CARTESIAN_POINT('Ctrl Pts',(-0.963899035117249,-0.333333333333333,
3.62400312501245));
#60345=CARTESIAN_POINT('Ctrl Pts',(-0.963899035117249,-0.666666666666667,
3.62400312501245));
#60346=CARTESIAN_POINT('Ctrl Pts',(-0.963899035117249,-1.,3.62400312501245));
#60347=CARTESIAN_POINT('Ctrl Pts',(-1.22531898815164,-1.,4.01728681790024));
#60348=CARTESIAN_POINT('Ctrl Pts',(-1.22531898815164,1.,4.01728681790024));
#60349=CARTESIAN_POINT('Ctrl Pts',(-1.22423716681447,-1.,4.0161454457032));
#60350=CARTESIAN_POINT('Ctrl Pts',(-1.22423716681447,1.,4.0161454457032));
#60351=CARTESIAN_POINT('Ctrl Pts',(-1.22207656456199,-1.,4.01386104434674));
#60352=CARTESIAN_POINT('Ctrl Pts',(-1.22207656456199,1.,4.01386104434674));
#60353=CARTESIAN_POINT('Ctrl Pts',(-1.21884478244983,-1.,4.01042947142681));
#60354=CARTESIAN_POINT('Ctrl Pts',(-1.21884478244983,1.,4.01042947142681));
#60355=CARTESIAN_POINT('Ctrl Pts',(-1.21455398918813,-1.,4.00584409524937));
#60356=CARTESIAN_POINT('Ctrl Pts',(-1.21455398918813,1.,4.00584409524937));
#60357=CARTESIAN_POINT('Ctrl Pts',(-1.20922097030107,-1.,4.00009577952534));
#60358=CARTESIAN_POINT('Ctrl Pts',(-1.20922097030107,1.,4.00009577952534));
#60359=CARTESIAN_POINT('Ctrl Pts',(-1.2039185237544,-1.,3.99433084800649));
#60360=CARTESIAN_POINT('Ctrl Pts',(-1.2039185237544,1.,3.99433084800649));
#60361=CARTESIAN_POINT('Ctrl Pts',(-1.19864679609596,-1.,3.98854928957287));
#60362=CARTESIAN_POINT('Ctrl Pts',(-1.19864679609596,1.,3.98854928957287));
#60363=CARTESIAN_POINT('Ctrl Pts',(-1.19340598349307,-1.,3.98275111052015));
#60364=CARTESIAN_POINT('Ctrl Pts',(-1.19340598349307,1.,3.98275111052015));
#60365=CARTESIAN_POINT('Ctrl Pts',(-1.18819633715285,-1.,3.97693634766926));
#60366=CARTESIAN_POINT('Ctrl Pts',(-1.18819633715285,1.,3.97693634766926));
#60367=CARTESIAN_POINT('Ctrl Pts',(-1.18301815039596,-1.,3.9711050516465));
#60368=CARTESIAN_POINT('Ctrl Pts',(-1.18301815039596,1.,3.9711050516465));
#60369=CARTESIAN_POINT('Ctrl Pts',(-1.17787174135445,-1.,3.96525726357682));
#60370=CARTESIAN_POINT('Ctrl Pts',(-1.17787174135445,1.,3.96525726357682));
#60371=CARTESIAN_POINT('Ctrl Pts',(-1.17275743590327,-1.,3.95939299213164));
#60372=CARTESIAN_POINT('Ctrl Pts',(-1.17275743590327,1.,3.95939299213164));
#60373=CARTESIAN_POINT('Ctrl Pts',(-1.16767555244495,-1.,3.95351219510062));
#60374=CARTESIAN_POINT('Ctrl Pts',(-1.16767555244495,1.,3.95351219510062));
#60375=CARTESIAN_POINT('Ctrl Pts',(-1.16262637999261,-1.,3.9476147478092));
#60376=CARTESIAN_POINT('Ctrl Pts',(-1.16262637999261,1.,3.9476147478092));
#60377=CARTESIAN_POINT('Ctrl Pts',(-1.1576101834106,-1.,3.94170046685542));
#60378=CARTESIAN_POINT('Ctrl Pts',(-1.1576101834106,1.,3.94170046685542));
#60379=CARTESIAN_POINT('Ctrl Pts',(-1.15262722716391,-1.,3.9357691705651));
#60380=CARTESIAN_POINT('Ctrl Pts',(-1.15262722716391,1.,3.9357691705651));
#60381=CARTESIAN_POINT('Ctrl Pts',(-1.14767779451147,-1.,3.92982073294334));
#60382=CARTESIAN_POINT('Ctrl Pts',(-1.14767779451147,1.,3.92982073294334));
#60383=CARTESIAN_POINT('Ctrl Pts',(-1.14276220561575,-1.,3.92385513133937));
#60384=CARTESIAN_POINT('Ctrl Pts',(-1.14276220561575,1.,3.92385513133937));
#60385=CARTESIAN_POINT('Ctrl Pts',(-1.13788084225511,-1.,3.91787251936688));
#60386=CARTESIAN_POINT('Ctrl Pts',(-1.13788084225511,1.,3.91787251936688));
#60387=CARTESIAN_POINT('Ctrl Pts',(-1.13303414693849,-1.,3.91187321145495));
#60388=CARTESIAN_POINT('Ctrl Pts',(-1.13303414693849,1.,3.91187321145495));
#60389=CARTESIAN_POINT('Ctrl Pts',(-1.12822258281518,-1.,3.90585753318622));
#60390=CARTESIAN_POINT('Ctrl Pts',(-1.12822258281518,1.,3.90585753318622));
#60391=CARTESIAN_POINT('Ctrl Pts',(-1.12344660099029,-1.,3.89982569749978));
#60392=CARTESIAN_POINT('Ctrl Pts',(-1.12344660099029,1.,3.89982569749978));
#60393=CARTESIAN_POINT('Ctrl Pts',(-1.11870660794609,-1.,3.89377768340362));
#60394=CARTESIAN_POINT('Ctrl Pts',(-1.11870660794609,1.,3.89377768340362));
#60395=CARTESIAN_POINT('Ctrl Pts',(-1.11400292434447,-1.,3.88771308285229));
#60396=CARTESIAN_POINT('Ctrl Pts',(-1.11400292434447,1.,3.88771308285229));
#60397=CARTESIAN_POINT('Ctrl Pts',(-1.10933577224029,-1.,3.88163105531791));
#60398=CARTESIAN_POINT('Ctrl Pts',(-1.10933577224029,1.,3.88163105531791));
#60399=CARTESIAN_POINT('Ctrl Pts',(-1.10470536603303,-1.,3.87553067187566));
#60400=CARTESIAN_POINT('Ctrl Pts',(-1.10470536603303,1.,3.87553067187566));
#60401=CARTESIAN_POINT('Ctrl Pts',(-1.10011198761202,-1.,3.86941120134872));
#60402=CARTESIAN_POINT('Ctrl Pts',(-1.10011198761202,1.,3.86941120134872));
#60403=CARTESIAN_POINT('Ctrl Pts',(-1.09555606505012,-1.,3.86327241021242));
#60404=CARTESIAN_POINT('Ctrl Pts',(-1.09555606505012,1.,3.86327241021242));
#60405=CARTESIAN_POINT('Ctrl Pts',(-1.09103825516288,-1.,3.85711487933911));
#60406=CARTESIAN_POINT('Ctrl Pts',(-1.09103825516288,1.,3.85711487933911));
#60407=CARTESIAN_POINT('Ctrl Pts',(-1.08655950846377,-1.,3.8509402522269));
#60408=CARTESIAN_POINT('Ctrl Pts',(-1.08655950846377,1.,3.8509402522269));
#60409=CARTESIAN_POINT('Ctrl Pts',(-1.08212087917986,-1.,3.84475048030615));
#60410=CARTESIAN_POINT('Ctrl Pts',(-1.08212087917986,1.,3.84475048030615));
#60411=CARTESIAN_POINT('Ctrl Pts',(-1.07772335353856,-1.,3.83854714117486));
#60412=CARTESIAN_POINT('Ctrl Pts',(-1.07772335353856,1.,3.83854714117486));
#60413=CARTESIAN_POINT('Ctrl Pts',(-1.0733676663346,-1.,3.83233071195145));
#60414=CARTESIAN_POINT('Ctrl Pts',(-1.0733676663346,1.,3.83233071195145));
#60415=CARTESIAN_POINT('Ctrl Pts',(-1.0690541318036,-1.,3.82609989967278));
#60416=CARTESIAN_POINT('Ctrl Pts',(-1.0690541318036,1.,3.82609989967278));
#60417=CARTESIAN_POINT('Ctrl Pts',(-1.06478244038931,-1.,3.81985083953012));
#60418=CARTESIAN_POINT('Ctrl Pts',(-1.06478244038931,1.,3.81985083953012));
#60419=CARTESIAN_POINT('Ctrl Pts',(-1.06055206187298,-1.,3.81357866117485));
#60420=CARTESIAN_POINT('Ctrl Pts',(-1.06055206187298,1.,3.81357866117485));
#60421=CARTESIAN_POINT('Ctrl Pts',(-1.05636266918643,-1.,3.80727913637784));
#60422=CARTESIAN_POINT('Ctrl Pts',(-1.05636266918643,1.,3.80727913637784));
#60423=CARTESIAN_POINT('Ctrl Pts',(-1.05221457990015,-1.,3.80095039790678));
#60424=CARTESIAN_POINT('Ctrl Pts',(-1.05221457990015,1.,3.80095039790678));
#60425=CARTESIAN_POINT('Ctrl Pts',(-1.04810913267641,-1.,3.79459440308793));
#60426=CARTESIAN_POINT('Ctrl Pts',(-1.04810913267641,1.,3.79459440308793));
#60427=CARTESIAN_POINT('Ctrl Pts',(-1.04404924374426,-1.,3.78821910787195));
#60428=CARTESIAN_POINT('Ctrl Pts',(-1.04404924374426,1.,3.78821910787195));
#60429=CARTESIAN_POINT('Ctrl Pts',(-1.04003862055804,-1.,3.78183535008192));
#60430=CARTESIAN_POINT('Ctrl Pts',(-1.04003862055804,1.,3.78183535008192));
#60431=CARTESIAN_POINT('Ctrl Pts',(-1.03608074678013,-1.,3.77545283140445));
#60432=CARTESIAN_POINT('Ctrl Pts',(-1.03608074678013,1.,3.77545283140445));
#60433=CARTESIAN_POINT('Ctrl Pts',(-1.0321778660492,-1.,3.76907609832522));
#60434=CARTESIAN_POINT('Ctrl Pts',(-1.0321778660492,1.,3.76907609832522));
#60435=CARTESIAN_POINT('Ctrl Pts',(-1.02833014458181,-1.,3.76270122291232));
#60436=CARTESIAN_POINT('Ctrl Pts',(-1.02833014458181,1.,3.76270122291232));
#60437=CARTESIAN_POINT('Ctrl Pts',(-1.0245342944466,-1.,3.75631037456194));
#60438=CARTESIAN_POINT('Ctrl Pts',(-1.0245342944466,1.,3.75631037456194));
#60439=CARTESIAN_POINT('Ctrl Pts',(-1.02078510487428,-1.,3.74987777155834));
#60440=CARTESIAN_POINT('Ctrl Pts',(-1.02078510487428,1.,3.74987777155834));
#60441=CARTESIAN_POINT('Ctrl Pts',(-1.01707794311079,-1.,3.74337942504959));
#60442=CARTESIAN_POINT('Ctrl Pts',(-1.01707794311079,1.,3.74337942504959));
#60443=CARTESIAN_POINT('Ctrl Pts',(-1.01341114319903,-1.,3.73680245055734));
#60444=CARTESIAN_POINT('Ctrl Pts',(-1.01341114319903,1.,3.73680245055734));
#60445=CARTESIAN_POINT('Ctrl Pts',(-1.00978798539496,-1.,3.73015276704426));
#60446=CARTESIAN_POINT('Ctrl Pts',(-1.00978798539496,1.,3.73015276704426));
#60447=CARTESIAN_POINT('Ctrl Pts',(-1.0062200073571,-1.,3.72346803750595));
#60448=CARTESIAN_POINT('Ctrl Pts',(-1.0062200073571,1.,3.72346803750595));
#60449=CARTESIAN_POINT('Ctrl Pts',(-1.00272423396822,-1.,3.71680667125118));
#60450=CARTESIAN_POINT('Ctrl Pts',(-1.00272423396822,1.,3.71680667125118));
#60451=CARTESIAN_POINT('Ctrl Pts',(-0.999317260756531,-1.,3.71022439713938));
#60452=CARTESIAN_POINT('Ctrl Pts',(-0.999317260756531,1.,3.71022439713938));
#60453=CARTESIAN_POINT('Ctrl Pts',(-0.996009819772518,-1.,3.70375282282138));
#60454=CARTESIAN_POINT('Ctrl Pts',(-0.996009819772518,1.,3.70375282282138));
#60455=CARTESIAN_POINT('Ctrl Pts',(-0.99280221833201,-1.,3.69738123415662));
#60456=CARTESIAN_POINT('Ctrl Pts',(-0.99280221833201,1.,3.69738123415662));
#60457=CARTESIAN_POINT('Ctrl Pts',(-0.989676715398558,-1.,3.69102682138846));
#60458=CARTESIAN_POINT('Ctrl Pts',(-0.989676715398558,1.,3.69102682138846));
#60459=CARTESIAN_POINT('Ctrl Pts',(-0.986602639863838,-1.,3.68455317926068));
#60460=CARTESIAN_POINT('Ctrl Pts',(-0.986602639863838,1.,3.68455317926068));
#60461=CARTESIAN_POINT('Ctrl Pts',(-0.983550791470419,-1.,3.67782408841715));
#60462=CARTESIAN_POINT('Ctrl Pts',(-0.983550791470419,1.,3.67782408841715));
#60463=CARTESIAN_POINT('Ctrl Pts',(-0.980505922458267,-1.,3.67074983340361));
#60464=CARTESIAN_POINT('Ctrl Pts',(-0.980505922458267,1.,3.67074983340361));
#60465=CARTESIAN_POINT('Ctrl Pts',(-0.977478312751618,-1.,3.66333049637475));
#60466=CARTESIAN_POINT('Ctrl Pts',(-0.977478312751618,1.,3.66333049637475));
#60467=CARTESIAN_POINT('Ctrl Pts',(-0.974519971354848,-1.,3.65571576735126));
#60468=CARTESIAN_POINT('Ctrl Pts',(-0.974519971354848,1.,3.65571576735126));
#60469=CARTESIAN_POINT('Ctrl Pts',(-0.971722122061341,-1.,3.64819756447455));
#60470=CARTESIAN_POINT('Ctrl Pts',(-0.971722122061341,1.,3.64819756447455));
#60471=CARTESIAN_POINT('Ctrl Pts',(-0.969195124675866,-1.,3.64113946505766));
#60472=CARTESIAN_POINT('Ctrl Pts',(-0.969195124675866,1.,3.64113946505766));
#60473=CARTESIAN_POINT('Ctrl Pts',(-0.967052554541386,-1.,3.63492122081143));
#60474=CARTESIAN_POINT('Ctrl Pts',(-0.967052554541386,1.,3.63492122081143));
#60475=CARTESIAN_POINT('Ctrl Pts',(-0.965395153165293,-1.,3.62988252139846));
#60476=CARTESIAN_POINT('Ctrl Pts',(-0.965395153165293,1.,3.62988252139846));
#60477=CARTESIAN_POINT('Ctrl Pts',(-0.964291001273288,-1.,3.62625391254797));
#60478=CARTESIAN_POINT('Ctrl Pts',(-0.964291001273288,1.,3.62625391254797));
#60479=CARTESIAN_POINT('Ctrl Pts',(-0.963875774530619,-1.,3.6245656860652));
#60480=CARTESIAN_POINT('Ctrl Pts',(-0.963875774530619,1.,3.6245656860652));
#60481=CARTESIAN_POINT('Ctrl Pts',(-0.963832486395051,-1.,3.62399933639914));
#60482=CARTESIAN_POINT('Ctrl Pts',(-0.963832486395051,1.,3.62399933639914));
#60483=CARTESIAN_POINT('Ctrl Pts',(-0.963922720982193,-1.,3.62393257642052));
#60484=CARTESIAN_POINT('Ctrl Pts',(-0.963922720982193,1.,3.62393257642052));
#60485=CARTESIAN_POINT('Ctrl Pts',(-0.963997613369571,-1.,3.62397690409552));
#60486=CARTESIAN_POINT('Ctrl Pts',(-0.963997613369571,1.,3.62397690409552));
#60487=CARTESIAN_POINT('',(-1.22531898815164,1.,4.01728681790024));
#60488=CARTESIAN_POINT('Ctrl Pts',(-1.22531898815164,1.,4.01728681790024));
#60489=CARTESIAN_POINT('Ctrl Pts',(-1.22423716681447,1.,4.0161454457032));
#60490=CARTESIAN_POINT('Ctrl Pts',(-1.22207656456199,1.,4.01386104434674));
#60491=CARTESIAN_POINT('Ctrl Pts',(-1.21884478244983,1.,4.01042947142681));
#60492=CARTESIAN_POINT('Ctrl Pts',(-1.21455398918813,1.,4.00584409524937));
#60493=CARTESIAN_POINT('Ctrl Pts',(-1.20922097030107,1.,4.00009577952534));
#60494=CARTESIAN_POINT('Ctrl Pts',(-1.2039185237544,1.,3.99433084800649));
#60495=CARTESIAN_POINT('Ctrl Pts',(-1.19864679609596,1.,3.98854928957287));
#60496=CARTESIAN_POINT('Ctrl Pts',(-1.19340598349307,1.,3.98275111052015));
#60497=CARTESIAN_POINT('Ctrl Pts',(-1.18819633715285,1.,3.97693634766926));
#60498=CARTESIAN_POINT('Ctrl Pts',(-1.18301815039596,1.,3.9711050516465));
#60499=CARTESIAN_POINT('Ctrl Pts',(-1.17787174135445,1.,3.96525726357682));
#60500=CARTESIAN_POINT('Ctrl Pts',(-1.17275743590327,1.,3.95939299213164));
#60501=CARTESIAN_POINT('Ctrl Pts',(-1.16767555244495,1.,3.95351219510062));
#60502=CARTESIAN_POINT('Ctrl Pts',(-1.16262637999261,1.,3.9476147478092));
#60503=CARTESIAN_POINT('Ctrl Pts',(-1.1576101834106,1.,3.94170046685542));
#60504=CARTESIAN_POINT('Ctrl Pts',(-1.15262722716391,1.,3.9357691705651));
#60505=CARTESIAN_POINT('Ctrl Pts',(-1.14767779451147,1.,3.92982073294334));
#60506=CARTESIAN_POINT('Ctrl Pts',(-1.14276220561575,1.,3.92385513133937));
#60507=CARTESIAN_POINT('Ctrl Pts',(-1.13788084225511,1.,3.91787251936688));
#60508=CARTESIAN_POINT('Ctrl Pts',(-1.13303414693849,1.,3.91187321145495));
#60509=CARTESIAN_POINT('Ctrl Pts',(-1.12822258281518,1.,3.90585753318622));
#60510=CARTESIAN_POINT('Ctrl Pts',(-1.12344660099029,1.,3.89982569749978));
#60511=CARTESIAN_POINT('Ctrl Pts',(-1.11870660794609,1.,3.89377768340362));
#60512=CARTESIAN_POINT('Ctrl Pts',(-1.11400292434447,1.,3.88771308285229));
#60513=CARTESIAN_POINT('Ctrl Pts',(-1.10933577224029,1.,3.88163105531791));
#60514=CARTESIAN_POINT('Ctrl Pts',(-1.10470536603303,1.,3.87553067187566));
#60515=CARTESIAN_POINT('Ctrl Pts',(-1.10011198761202,1.,3.86941120134872));
#60516=CARTESIAN_POINT('Ctrl Pts',(-1.09555606505012,1.,3.86327241021242));
#60517=CARTESIAN_POINT('Ctrl Pts',(-1.09103825516288,1.,3.85711487933911));
#60518=CARTESIAN_POINT('Ctrl Pts',(-1.08655950846377,1.,3.8509402522269));
#60519=CARTESIAN_POINT('Ctrl Pts',(-1.08212087917986,1.,3.84475048030615));
#60520=CARTESIAN_POINT('Ctrl Pts',(-1.07772335353856,1.,3.83854714117486));
#60521=CARTESIAN_POINT('Ctrl Pts',(-1.0733676663346,1.,3.83233071195145));
#60522=CARTESIAN_POINT('Ctrl Pts',(-1.0690541318036,1.,3.82609989967278));
#60523=CARTESIAN_POINT('Ctrl Pts',(-1.06478244038931,1.,3.81985083953012));
#60524=CARTESIAN_POINT('Ctrl Pts',(-1.06055206187298,1.,3.81357866117485));
#60525=CARTESIAN_POINT('Ctrl Pts',(-1.05636266918643,1.,3.80727913637784));
#60526=CARTESIAN_POINT('Ctrl Pts',(-1.05221457990015,1.,3.80095039790678));
#60527=CARTESIAN_POINT('Ctrl Pts',(-1.04810913267641,1.,3.79459440308793));
#60528=CARTESIAN_POINT('Ctrl Pts',(-1.04404924374426,1.,3.78821910787195));
#60529=CARTESIAN_POINT('Ctrl Pts',(-1.04003862055804,1.,3.78183535008192));
#60530=CARTESIAN_POINT('Ctrl Pts',(-1.03608074678013,1.,3.77545283140445));
#60531=CARTESIAN_POINT('Ctrl Pts',(-1.0321778660492,1.,3.76907609832522));
#60532=CARTESIAN_POINT('Ctrl Pts',(-1.02833014458181,1.,3.76270122291232));
#60533=CARTESIAN_POINT('Ctrl Pts',(-1.0245342944466,1.,3.75631037456194));
#60534=CARTESIAN_POINT('Ctrl Pts',(-1.02078510487428,1.,3.74987777155834));
#60535=CARTESIAN_POINT('Ctrl Pts',(-1.01707794311079,1.,3.74337942504959));
#60536=CARTESIAN_POINT('Ctrl Pts',(-1.01341114319903,1.,3.73680245055734));
#60537=CARTESIAN_POINT('Ctrl Pts',(-1.00978798539496,1.,3.73015276704426));
#60538=CARTESIAN_POINT('Ctrl Pts',(-1.0062200073571,1.,3.72346803750595));
#60539=CARTESIAN_POINT('Ctrl Pts',(-1.00272423396822,1.,3.71680667125118));
#60540=CARTESIAN_POINT('Ctrl Pts',(-0.999317260756531,1.,3.71022439713938));
#60541=CARTESIAN_POINT('Ctrl Pts',(-0.996009819772518,1.,3.70375282282138));
#60542=CARTESIAN_POINT('Ctrl Pts',(-0.99280221833201,1.,3.69738123415662));
#60543=CARTESIAN_POINT('Ctrl Pts',(-0.989676715398558,1.,3.69102682138846));
#60544=CARTESIAN_POINT('Ctrl Pts',(-0.986602639863838,1.,3.68455317926068));
#60545=CARTESIAN_POINT('Ctrl Pts',(-0.983550791470419,1.,3.67782408841715));
#60546=CARTESIAN_POINT('Ctrl Pts',(-0.980505922458267,1.,3.67074983340361));
#60547=CARTESIAN_POINT('Ctrl Pts',(-0.977478312751618,1.,3.66333049637475));
#60548=CARTESIAN_POINT('Ctrl Pts',(-0.974519971354848,1.,3.65571576735126));
#60549=CARTESIAN_POINT('Ctrl Pts',(-0.971722122061341,1.,3.64819756447455));
#60550=CARTESIAN_POINT('Ctrl Pts',(-0.969195124675866,1.,3.64113946505766));
#60551=CARTESIAN_POINT('Ctrl Pts',(-0.967052554541386,1.,3.63492122081143));
#60552=CARTESIAN_POINT('Ctrl Pts',(-0.965395153165293,1.,3.62988252139846));
#60553=CARTESIAN_POINT('Ctrl Pts',(-0.964373850166457,1.,3.62652618145335));
#60554=CARTESIAN_POINT('Ctrl Pts',(-0.963957782642843,1.,3.62489305727662));
#60555=CARTESIAN_POINT('Ctrl Pts',(-0.963861297423241,1.,3.62424461507588));
#60556=CARTESIAN_POINT('Ctrl Pts',(-0.963880158555582,1.,3.6240482887845));
#60557=CARTESIAN_POINT('Ctrl Pts',(-0.963899035117249,1.,3.62400312501245));
#60558=CARTESIAN_POINT('',(-1.22531898815164,0.,4.01728681790024));
#60559=CARTESIAN_POINT('Ctrl Pts',(-1.35022972712301,-1.,3.49848248301936));
#60560=CARTESIAN_POINT('Ctrl Pts',(-1.35022972712301,1.,3.49848248301936));
#60561=CARTESIAN_POINT('Ctrl Pts',(-1.35026426118402,-1.,3.4984026005375));
#60562=CARTESIAN_POINT('Ctrl Pts',(-1.35026426118402,1.,3.4984026005375));
#60563=CARTESIAN_POINT('Ctrl Pts',(-1.35037650303019,-1.,3.49840357193736));
#60564=CARTESIAN_POINT('Ctrl Pts',(-1.35037650303019,1.,3.49840357193736));
#60565=CARTESIAN_POINT('Ctrl Pts',(-1.35067437417483,-1.,3.49888720257132));
#60566=CARTESIAN_POINT('Ctrl Pts',(-1.35067437417483,1.,3.49888720257132));
#60567=CARTESIAN_POINT('Ctrl Pts',(-1.3513307633124,-1.,3.5004970706414));
#60568=CARTESIAN_POINT('Ctrl Pts',(-1.3513307633124,1.,3.5004970706414));
#60569=CARTESIAN_POINT('Ctrl Pts',(-1.35257032843486,-1.,3.50408168106261));
#60570=CARTESIAN_POINT('Ctrl Pts',(-1.35257032843486,1.,3.50408168106261));
#60571=CARTESIAN_POINT('Ctrl Pts',(-1.35419113575956,-1.,3.50913227059999));
#60572=CARTESIAN_POINT('Ctrl Pts',(-1.35419113575956,1.,3.50913227059999));
#60573=CARTESIAN_POINT('Ctrl Pts',(-1.35611275237152,-1.,3.51542230699556));
#60574=CARTESIAN_POINT('Ctrl Pts',(-1.35611275237152,1.,3.51542230699556));
#60575=CARTESIAN_POINT('Ctrl Pts',(-1.35821701528836,-1.,3.52261776116748));
#60576=CARTESIAN_POINT('Ctrl Pts',(-1.35821701528836,1.,3.52261776116748));
#60577=CARTESIAN_POINT('Ctrl Pts',(-1.36037259643734,-1.,3.530344649616));
#60578=CARTESIAN_POINT('Ctrl Pts',(-1.36037259643734,1.,3.530344649616));
#60579=CARTESIAN_POINT('Ctrl Pts',(-1.36245507339307,-1.,3.53824396424961));
#60580=CARTESIAN_POINT('Ctrl Pts',(-1.36245507339307,1.,3.53824396424961));
#60581=CARTESIAN_POINT('Ctrl Pts',(-1.36436666257598,-1.,3.54602591832973));
#60582=CARTESIAN_POINT('Ctrl Pts',(-1.36436666257598,1.,3.54602591832973));
#60583=CARTESIAN_POINT('Ctrl Pts',(-1.3660614545677,-1.,3.55353883995949));
#60584=CARTESIAN_POINT('Ctrl Pts',(-1.3660614545677,1.,3.55353883995949));
#60585=CARTESIAN_POINT('Ctrl Pts',(-1.36754771771233,-1.,3.56077662028649));
#60586=CARTESIAN_POINT('Ctrl Pts',(-1.36754771771233,1.,3.56077662028649));
#60587=CARTESIAN_POINT('Ctrl Pts',(-1.36886584973389,-1.,3.5678208030466));
#60588=CARTESIAN_POINT('Ctrl Pts',(-1.36886584973389,1.,3.5678208030466));
#60589=CARTESIAN_POINT('Ctrl Pts',(-1.37007229485659,-1.,3.57479875549486));
#60590=CARTESIAN_POINT('Ctrl Pts',(-1.37007229485659,1.,3.57479875549486));
#60591=CARTESIAN_POINT('Ctrl Pts',(-1.37122241663062,-1.,3.58183885982715));
#60592=CARTESIAN_POINT('Ctrl Pts',(-1.37122241663062,1.,3.58183885982715));
#60593=CARTESIAN_POINT('Ctrl Pts',(-1.37235053660976,-1.,3.58901853846365));
#60594=CARTESIAN_POINT('Ctrl Pts',(-1.37235053660976,1.,3.58901853846365));
#60595=CARTESIAN_POINT('Ctrl Pts',(-1.37346320103157,-1.,3.59634627869048));
#60596=CARTESIAN_POINT('Ctrl Pts',(-1.37346320103157,1.,3.59634627869048));
#60597=CARTESIAN_POINT('Ctrl Pts',(-1.37455051379623,-1.,3.60379020123988));
#60598=CARTESIAN_POINT('Ctrl Pts',(-1.37455051379623,1.,3.60379020123988));
#60599=CARTESIAN_POINT('Ctrl Pts',(-1.37559314436634,-1.,3.61129546591064));
#60600=CARTESIAN_POINT('Ctrl Pts',(-1.37559314436634,1.,3.61129546591064));
#60601=CARTESIAN_POINT('Ctrl Pts',(-1.37657053403107,-1.,3.6188048116042));
#60602=CARTESIAN_POINT('Ctrl Pts',(-1.37657053403107,1.,3.6188048116042));
#60603=CARTESIAN_POINT('Ctrl Pts',(-1.37746987919881,-1.,3.62628098665145));
#60604=CARTESIAN_POINT('Ctrl Pts',(-1.37746987919881,1.,3.62628098665145));
#60605=CARTESIAN_POINT('Ctrl Pts',(-1.37829035457339,-1.,3.63371727442486));
#60606=CARTESIAN_POINT('Ctrl Pts',(-1.37829035457339,1.,3.63371727442486));
#60607=CARTESIAN_POINT('Ctrl Pts',(-1.37903818567359,-1.,3.64112507791141));
#60608=CARTESIAN_POINT('Ctrl Pts',(-1.37903818567359,1.,3.64112507791141));
#60609=CARTESIAN_POINT('Ctrl Pts',(-1.37972372481603,-1.,3.64852652756456));
#60610=CARTESIAN_POINT('Ctrl Pts',(-1.37972372481603,1.,3.64852652756456));
#60611=CARTESIAN_POINT('Ctrl Pts',(-1.38035791051213,-1.,3.6559455440439));
#60612=CARTESIAN_POINT('Ctrl Pts',(-1.38035791051213,1.,3.6559455440439));
#60613=CARTESIAN_POINT('Ctrl Pts',(-1.38094856333552,-1.,3.66339848520857));
#60614=CARTESIAN_POINT('Ctrl Pts',(-1.38094856333552,1.,3.66339848520857));
#60615=CARTESIAN_POINT('Ctrl Pts',(-1.38149812653868,-1.,3.67088843112262));
#60616=CARTESIAN_POINT('Ctrl Pts',(-1.38149812653868,1.,3.67088843112262));
#60617=CARTESIAN_POINT('Ctrl Pts',(-1.3820057429062,-1.,3.67841038482414));
#60618=CARTESIAN_POINT('Ctrl Pts',(-1.3820057429062,1.,3.67841038482414));
#60619=CARTESIAN_POINT('Ctrl Pts',(-1.38246852827182,-1.,3.68595444983837));
#60620=CARTESIAN_POINT('Ctrl Pts',(-1.38246852827182,1.,3.68595444983837));
#60621=CARTESIAN_POINT('Ctrl Pts',(-1.38288311171651,-1.,3.69350967899526));
#60622=CARTESIAN_POINT('Ctrl Pts',(-1.38288311171651,1.,3.69350967899526));
#60623=CARTESIAN_POINT('Ctrl Pts',(-1.38324717612865,-1.,3.701067921679));
#60624=CARTESIAN_POINT('Ctrl Pts',(-1.38324717612865,1.,3.701067921679));
#60625=CARTESIAN_POINT('Ctrl Pts',(-1.38356065402124,-1.,3.70862680753347));
#60626=CARTESIAN_POINT('Ctrl Pts',(-1.38356065402124,1.,3.70862680753347));
#60627=CARTESIAN_POINT('Ctrl Pts',(-1.38382489984586,-1.,3.7161876605181));
#60628=CARTESIAN_POINT('Ctrl Pts',(-1.38382489984586,1.,3.7161876605181));
#60629=CARTESIAN_POINT('Ctrl Pts',(-1.3840421342895,-1.,3.72375409358803));
#60630=CARTESIAN_POINT('Ctrl Pts',(-1.3840421342895,1.,3.72375409358803));
#60631=CARTESIAN_POINT('Ctrl Pts',(-1.38421479111531,-1.,3.73133035859282));
#60632=CARTESIAN_POINT('Ctrl Pts',(-1.38421479111531,1.,3.73133035859282));
#60633=CARTESIAN_POINT('Ctrl Pts',(-1.38434489156458,-1.,3.73891976418104));
#60634=CARTESIAN_POINT('Ctrl Pts',(-1.38434489156458,1.,3.73891976418104));
#60635=CARTESIAN_POINT('Ctrl Pts',(-1.38443344984394,-1.,3.74652317167876));
#60636=CARTESIAN_POINT('Ctrl Pts',(-1.38443344984394,1.,3.74652317167876));
#60637=CARTESIAN_POINT('Ctrl Pts',(-1.38448077997163,-1.,3.7541397631875));
#60638=CARTESIAN_POINT('Ctrl Pts',(-1.38448077997163,1.,3.7541397631875));
#60639=CARTESIAN_POINT('Ctrl Pts',(-1.3844867525335,-1.,3.76176768271367));
#60640=CARTESIAN_POINT('Ctrl Pts',(-1.3844867525335,1.,3.76176768271367));
#60641=CARTESIAN_POINT('Ctrl Pts',(-1.38445107339518,-1.,3.76940473185779));
#60642=CARTESIAN_POINT('Ctrl Pts',(-1.38445107339518,1.,3.76940473185779));
#60643=CARTESIAN_POINT('Ctrl Pts',(-1.38437354551428,-1.,3.77704902230418));
#60644=CARTESIAN_POINT('Ctrl Pts',(-1.38437354551428,1.,3.77704902230418));
#60645=CARTESIAN_POINT('Ctrl Pts',(-1.38425435883756,-1.,3.78469969805082));
#60646=CARTESIAN_POINT('Ctrl Pts',(-1.38425435883756,1.,3.78469969805082));
#60647=CARTESIAN_POINT('Ctrl Pts',(-1.38409399694566,-1.,3.79235669640841));
#60648=CARTESIAN_POINT('Ctrl Pts',(-1.38409399694566,1.,3.79235669640841));
#60649=CARTESIAN_POINT('Ctrl Pts',(-1.38389311766682,-1.,3.80002044322111));
#60650=CARTESIAN_POINT('Ctrl Pts',(-1.38389311766682,1.,3.80002044322111));
#60651=CARTESIAN_POINT('Ctrl Pts',(-1.3836524404622,-1.,3.80769156398411));
#60652=CARTESIAN_POINT('Ctrl Pts',(-1.3836524404622,1.,3.80769156398411));
#60653=CARTESIAN_POINT('Ctrl Pts',(-1.38337263902782,-1.,3.81537060817811));
#60654=CARTESIAN_POINT('Ctrl Pts',(-1.38337263902782,1.,3.81537060817811));
#60655=CARTESIAN_POINT('Ctrl Pts',(-1.38305421262763,-1.,3.82305771743829));
#60656=CARTESIAN_POINT('Ctrl Pts',(-1.38305421262763,1.,3.82305771743829));
#60657=CARTESIAN_POINT('Ctrl Pts',(-1.38269750245138,-1.,3.8307526698229));
#60658=CARTESIAN_POINT('Ctrl Pts',(-1.38269750245138,1.,3.8307526698229));
#60659=CARTESIAN_POINT('Ctrl Pts',(-1.38230274828822,-1.,3.83845502790746));
#60660=CARTESIAN_POINT('Ctrl Pts',(-1.38230274828822,1.,3.83845502790746));
#60661=CARTESIAN_POINT('Ctrl Pts',(-1.38187013346109,-1.,3.84616425605764));
#60662=CARTESIAN_POINT('Ctrl Pts',(-1.38187013346109,1.,3.84616425605764));
#60663=CARTESIAN_POINT('Ctrl Pts',(-1.38139983115049,-1.,3.85387983979481));
#60664=CARTESIAN_POINT('Ctrl Pts',(-1.38139983115049,1.,3.85387983979481));
#60665=CARTESIAN_POINT('Ctrl Pts',(-1.38089205992989,-1.,3.86160143043959));
#60666=CARTESIAN_POINT('Ctrl Pts',(-1.38089205992989,1.,3.86160143043959));
#60667=CARTESIAN_POINT('Ctrl Pts',(-1.38034709213014,-1.,3.86932885813068));
#60668=CARTESIAN_POINT('Ctrl Pts',(-1.38034709213014,1.,3.86932885813068));
#60669=CARTESIAN_POINT('Ctrl Pts',(-1.37976523097073,-1.,3.87706205830532));
#60670=CARTESIAN_POINT('Ctrl Pts',(-1.37976523097073,1.,3.87706205830532));
#60671=CARTESIAN_POINT('Ctrl Pts',(-1.37914679719383,-1.,3.88480102249277));
#60672=CARTESIAN_POINT('Ctrl Pts',(-1.37914679719383,1.,3.88480102249277));
#60673=CARTESIAN_POINT('Ctrl Pts',(-1.3784921128802,-1.,3.89254574338496));
#60674=CARTESIAN_POINT('Ctrl Pts',(-1.3784921128802,1.,3.89254574338496));
#60675=CARTESIAN_POINT('Ctrl Pts',(-1.37780148512792,-1.,3.90029615196727));
#60676=CARTESIAN_POINT('Ctrl Pts',(-1.37780148512792,1.,3.90029615196727));
#60677=CARTESIAN_POINT('Ctrl Pts',(-1.3770751963402,-1.,3.90805209523486));
#60678=CARTESIAN_POINT('Ctrl Pts',(-1.3770751963402,1.,3.90805209523486));
#60679=CARTESIAN_POINT('Ctrl Pts',(-1.37631350505797,-1.,3.91581337462644));
#60680=CARTESIAN_POINT('Ctrl Pts',(-1.37631350505797,1.,3.91581337462644));
#60681=CARTESIAN_POINT('Ctrl Pts',(-1.37551664448242,-1.,3.92357976987672));
#60682=CARTESIAN_POINT('Ctrl Pts',(-1.37551664448242,1.,3.92357976987672));
#60683=CARTESIAN_POINT('Ctrl Pts',(-1.37468482215751,-1.,3.93135106761844));
#60684=CARTESIAN_POINT('Ctrl Pts',(-1.37468482215751,1.,3.93135106761844));
#60685=CARTESIAN_POINT('Ctrl Pts',(-1.37381821967165,-1.,3.93912709040818));
#60686=CARTESIAN_POINT('Ctrl Pts',(-1.37381821967165,1.,3.93912709040818));
#60687=CARTESIAN_POINT('Ctrl Pts',(-1.37291699202807,-1.,3.94690771785133));
#60688=CARTESIAN_POINT('Ctrl Pts',(-1.37291699202807,1.,3.94690771785133));
#60689=CARTESIAN_POINT('Ctrl Pts',(-1.37198126432386,-1.,3.95469287280914));
#60690=CARTESIAN_POINT('Ctrl Pts',(-1.37198126432386,1.,3.95469287280914));
#60691=CARTESIAN_POINT('Ctrl Pts',(-1.3712051561502,-1.,3.96092458506535));
#60692=CARTESIAN_POINT('Ctrl Pts',(-1.3712051561502,1.,3.96092458506535));
#60693=CARTESIAN_POINT('Ctrl Pts',(-1.37060761745635,-1.,3.96560037974645));
#60694=CARTESIAN_POINT('Ctrl Pts',(-1.37060761745635,1.,3.96560037974645));
#60695=CARTESIAN_POINT('Ctrl Pts',(-1.37020239094614,-1.,3.9687184694131));
#60696=CARTESIAN_POINT('Ctrl Pts',(-1.37020239094614,1.,3.9687184694131));
#60697=CARTESIAN_POINT('Ctrl Pts',(-1.36999806084572,-1.,3.97027773754922));
#60698=CARTESIAN_POINT('Ctrl Pts',(-1.36999806084572,1.,3.97027773754922));
#60699=CARTESIAN_POINT('',(-1.35032489087101,1.,3.4984457533445));
#60700=CARTESIAN_POINT('Ctrl Pts',(-1.35032489087101,-1.,3.4984457533445));
#60701=CARTESIAN_POINT('Ctrl Pts',(-1.35032489087101,-0.666666666666667,
3.4984457533445));
#60702=CARTESIAN_POINT('Ctrl Pts',(-1.35032489087101,-0.333333333333333,
3.4984457533445));
#60703=CARTESIAN_POINT('Ctrl Pts',(-1.35032489087101,0.333333333333333,
3.4984457533445));
#60704=CARTESIAN_POINT('Ctrl Pts',(-1.35032489087101,0.666666666666667,
3.4984457533445));
#60705=CARTESIAN_POINT('Ctrl Pts',(-1.35032489087101,1.,3.4984457533445));
#60706=CARTESIAN_POINT('',(-1.36999806084572,1.,3.97027773754922));
#60707=CARTESIAN_POINT('',(-1.36999806084572,0.,3.97027773754922));
#60708=CARTESIAN_POINT('Ctrl Pts',(-1.35032489087101,1.,3.4984457533445));
#60709=CARTESIAN_POINT('Ctrl Pts',(-1.35036670892966,1.,3.49847119623846));
#60710=CARTESIAN_POINT('Ctrl Pts',(-1.35049736560527,1.,3.49861894124827));
#60711=CARTESIAN_POINT('Ctrl Pts',(-1.35080045218587,1.,3.49920025459723));
#60712=CARTESIAN_POINT('Ctrl Pts',(-1.35142377279517,1.,3.5007660381649));
#60713=CARTESIAN_POINT('Ctrl Pts',(-1.35257032843486,1.,3.50408168106261));
#60714=CARTESIAN_POINT('Ctrl Pts',(-1.35419113575956,1.,3.50913227059999));
#60715=CARTESIAN_POINT('Ctrl Pts',(-1.35611275237152,1.,3.51542230699556));
#60716=CARTESIAN_POINT('Ctrl Pts',(-1.35821701528836,1.,3.52261776116748));
#60717=CARTESIAN_POINT('Ctrl Pts',(-1.36037259643734,1.,3.530344649616));
#60718=CARTESIAN_POINT('Ctrl Pts',(-1.36245507339307,1.,3.53824396424961));
#60719=CARTESIAN_POINT('Ctrl Pts',(-1.36436666257598,1.,3.54602591832973));
#60720=CARTESIAN_POINT('Ctrl Pts',(-1.3660614545677,1.,3.55353883995949));
#60721=CARTESIAN_POINT('Ctrl Pts',(-1.36754771771233,1.,3.56077662028649));
#60722=CARTESIAN_POINT('Ctrl Pts',(-1.36886584973389,1.,3.5678208030466));
#60723=CARTESIAN_POINT('Ctrl Pts',(-1.37007229485659,1.,3.57479875549486));
#60724=CARTESIAN_POINT('Ctrl Pts',(-1.37122241663062,1.,3.58183885982715));
#60725=CARTESIAN_POINT('Ctrl Pts',(-1.37235053660976,1.,3.58901853846365));
#60726=CARTESIAN_POINT('Ctrl Pts',(-1.37346320103157,1.,3.59634627869048));
#60727=CARTESIAN_POINT('Ctrl Pts',(-1.37455051379623,1.,3.60379020123988));
#60728=CARTESIAN_POINT('Ctrl Pts',(-1.37559314436634,1.,3.61129546591064));
#60729=CARTESIAN_POINT('Ctrl Pts',(-1.37657053403107,1.,3.6188048116042));
#60730=CARTESIAN_POINT('Ctrl Pts',(-1.37746987919881,1.,3.62628098665145));
#60731=CARTESIAN_POINT('Ctrl Pts',(-1.37829035457339,1.,3.63371727442486));
#60732=CARTESIAN_POINT('Ctrl Pts',(-1.37903818567359,1.,3.64112507791141));
#60733=CARTESIAN_POINT('Ctrl Pts',(-1.37972372481603,1.,3.64852652756456));
#60734=CARTESIAN_POINT('Ctrl Pts',(-1.38035791051213,1.,3.6559455440439));
#60735=CARTESIAN_POINT('Ctrl Pts',(-1.38094856333552,1.,3.66339848520857));
#60736=CARTESIAN_POINT('Ctrl Pts',(-1.38149812653868,1.,3.67088843112262));
#60737=CARTESIAN_POINT('Ctrl Pts',(-1.3820057429062,1.,3.67841038482414));
#60738=CARTESIAN_POINT('Ctrl Pts',(-1.38246852827182,1.,3.68595444983837));
#60739=CARTESIAN_POINT('Ctrl Pts',(-1.38288311171651,1.,3.69350967899526));
#60740=CARTESIAN_POINT('Ctrl Pts',(-1.38324717612865,1.,3.701067921679));
#60741=CARTESIAN_POINT('Ctrl Pts',(-1.38356065402124,1.,3.70862680753347));
#60742=CARTESIAN_POINT('Ctrl Pts',(-1.38382489984586,1.,3.7161876605181));
#60743=CARTESIAN_POINT('Ctrl Pts',(-1.3840421342895,1.,3.72375409358803));
#60744=CARTESIAN_POINT('Ctrl Pts',(-1.38421479111531,1.,3.73133035859282));
#60745=CARTESIAN_POINT('Ctrl Pts',(-1.38434489156458,1.,3.73891976418104));
#60746=CARTESIAN_POINT('Ctrl Pts',(-1.38443344984394,1.,3.74652317167876));
#60747=CARTESIAN_POINT('Ctrl Pts',(-1.38448077997163,1.,3.7541397631875));
#60748=CARTESIAN_POINT('Ctrl Pts',(-1.3844867525335,1.,3.76176768271367));
#60749=CARTESIAN_POINT('Ctrl Pts',(-1.38445107339518,1.,3.76940473185779));
#60750=CARTESIAN_POINT('Ctrl Pts',(-1.38437354551428,1.,3.77704902230418));
#60751=CARTESIAN_POINT('Ctrl Pts',(-1.38425435883756,1.,3.78469969805082));
#60752=CARTESIAN_POINT('Ctrl Pts',(-1.38409399694566,1.,3.79235669640841));
#60753=CARTESIAN_POINT('Ctrl Pts',(-1.38389311766682,1.,3.80002044322111));
#60754=CARTESIAN_POINT('Ctrl Pts',(-1.3836524404622,1.,3.80769156398411));
#60755=CARTESIAN_POINT('Ctrl Pts',(-1.38337263902782,1.,3.81537060817811));
#60756=CARTESIAN_POINT('Ctrl Pts',(-1.38305421262763,1.,3.82305771743829));
#60757=CARTESIAN_POINT('Ctrl Pts',(-1.38269750245138,1.,3.8307526698229));
#60758=CARTESIAN_POINT('Ctrl Pts',(-1.38230274828822,1.,3.83845502790746));
#60759=CARTESIAN_POINT('Ctrl Pts',(-1.38187013346109,1.,3.84616425605764));
#60760=CARTESIAN_POINT('Ctrl Pts',(-1.38139983115049,1.,3.85387983979481));
#60761=CARTESIAN_POINT('Ctrl Pts',(-1.38089205992989,1.,3.86160143043959));
#60762=CARTESIAN_POINT('Ctrl Pts',(-1.38034709213014,1.,3.86932885813068));
#60763=CARTESIAN_POINT('Ctrl Pts',(-1.37976523097073,1.,3.87706205830532));
#60764=CARTESIAN_POINT('Ctrl Pts',(-1.37914679719383,1.,3.88480102249277));
#60765=CARTESIAN_POINT('Ctrl Pts',(-1.3784921128802,1.,3.89254574338496));
#60766=CARTESIAN_POINT('Ctrl Pts',(-1.37780148512792,1.,3.90029615196727));
#60767=CARTESIAN_POINT('Ctrl Pts',(-1.3770751963402,1.,3.90805209523486));
#60768=CARTESIAN_POINT('Ctrl Pts',(-1.37631350505797,1.,3.91581337462644));
#60769=CARTESIAN_POINT('Ctrl Pts',(-1.37551664448242,1.,3.92357976987672));
#60770=CARTESIAN_POINT('Ctrl Pts',(-1.37468482215751,1.,3.93135106761844));
#60771=CARTESIAN_POINT('Ctrl Pts',(-1.37381821967165,1.,3.93912709040818));
#60772=CARTESIAN_POINT('Ctrl Pts',(-1.37291699202807,1.,3.94690771785133));
#60773=CARTESIAN_POINT('Ctrl Pts',(-1.37198126432386,1.,3.95469287280914));
#60774=CARTESIAN_POINT('Ctrl Pts',(-1.3712051561502,1.,3.96092458506535));
#60775=CARTESIAN_POINT('Ctrl Pts',(-1.37060761745635,1.,3.96560037974645));
#60776=CARTESIAN_POINT('Ctrl Pts',(-1.37020239094614,1.,3.9687184694131));
#60777=CARTESIAN_POINT('Ctrl Pts',(-1.36999806084572,1.,3.97027773754922));
#60778=CARTESIAN_POINT('Origin',(-1.36999806084572,0.,3.97027773754922));
#60779=CARTESIAN_POINT('',(-1.22531898815164,1.,4.01728681790024));
#60780=CARTESIAN_POINT('Origin',(0.,0.,0.));
#60781=CARTESIAN_POINT('',(-1.51895082866166,1.,3.42859860294378));
#60782=CARTESIAN_POINT('Origin',(0.,1.,0.));
#60783=CARTESIAN_POINT('Ctrl Pts',(-1.51895082866166,1.,3.42859860294378));
#60784=CARTESIAN_POINT('Ctrl Pts',(-1.51895082866166,0.666666666666667,
3.42859860294378));
#60785=CARTESIAN_POINT('Ctrl Pts',(-1.51895082866166,0.333333333333333,
3.42859860294378));
#60786=CARTESIAN_POINT('Ctrl Pts',(-1.51895082866166,-0.333333333333333,
3.42859860294378));
#60787=CARTESIAN_POINT('Ctrl Pts',(-1.51895082866166,-0.666666666666667,
3.42859860294378));
#60788=CARTESIAN_POINT('Ctrl Pts',(-1.51895082866166,-1.,3.42859860294378));
#60789=CARTESIAN_POINT('Ctrl Pts',(-1.83867539237861,-1.,3.77614523045147));
#60790=CARTESIAN_POINT('Ctrl Pts',(-1.83867539237861,1.,3.77614523045147));
#60791=CARTESIAN_POINT('Ctrl Pts',(-1.83742834010821,-1.,3.77518714458232));
#60792=CARTESIAN_POINT('Ctrl Pts',(-1.83742834010821,1.,3.77518714458232));
#60793=CARTESIAN_POINT('Ctrl Pts',(-1.83493697935064,-1.,3.77326886065484));
#60794=CARTESIAN_POINT('Ctrl Pts',(-1.83493697935064,1.,3.77326886065484));
#60795=CARTESIAN_POINT('Ctrl Pts',(-1.83120816956515,-1.,3.77038509819777));
#60796=CARTESIAN_POINT('Ctrl Pts',(-1.83120816956515,1.,3.77038509819777));
#60797=CARTESIAN_POINT('Ctrl Pts',(-1.82625289221933,-1.,3.76652740355856));
#60798=CARTESIAN_POINT('Ctrl Pts',(-1.82625289221933,1.,3.76652740355856));
#60799=CARTESIAN_POINT('Ctrl Pts',(-1.82008629694924,-1.,3.76168412709652));
#60800=CARTESIAN_POINT('Ctrl Pts',(-1.82008629694924,1.,3.76168412709652));
#60801=CARTESIAN_POINT('Ctrl Pts',(-1.81394729834032,-1.,3.75681965683995));
#60802=CARTESIAN_POINT('Ctrl Pts',(-1.81394729834032,1.,3.75681965683995));
#60803=CARTESIAN_POINT('Ctrl Pts',(-1.80783603939662,-1.,3.75193395888069));
#60804=CARTESIAN_POINT('Ctrl Pts',(-1.80783603939662,1.,3.75193395888069));
#60805=CARTESIAN_POINT('Ctrl Pts',(-1.80175271485519,-1.,3.74702700874954));
#60806=CARTESIAN_POINT('Ctrl Pts',(-1.80175271485519,1.,3.74702700874954));
#60807=CARTESIAN_POINT('Ctrl Pts',(-1.79569757859041,-1.,3.74209880351667));
#60808=CARTESIAN_POINT('Ctrl Pts',(-1.79569757859041,1.,3.74209880351667));
#60809=CARTESIAN_POINT('Ctrl Pts',(-1.78967092823139,-1.,3.73714934729962));
#60810=CARTESIAN_POINT('Ctrl Pts',(-1.78967092823139,1.,3.73714934729962));
#60811=CARTESIAN_POINT('Ctrl Pts',(-1.78367308442682,-1.,3.73217863095022));
#60812=CARTESIAN_POINT('Ctrl Pts',(-1.78367308442682,1.,3.73217863095022));
#60813=CARTESIAN_POINT('Ctrl Pts',(-1.77770437039606,-1.,3.72718661205504));
#60814=CARTESIAN_POINT('Ctrl Pts',(-1.77770437039606,1.,3.72718661205504));
#60815=CARTESIAN_POINT('Ctrl Pts',(-1.77176509401846,-1.,3.72217319911429));
#60816=CARTESIAN_POINT('Ctrl Pts',(-1.77176509401846,1.,3.72217319911429));
#60817=CARTESIAN_POINT('Ctrl Pts',(-1.76585552124549,-1.,3.71713822377675));
#60818=CARTESIAN_POINT('Ctrl Pts',(-1.76585552124549,1.,3.71713822377675));
#60819=CARTESIAN_POINT('Ctrl Pts',(-1.75997588499021,-1.,3.71208146346454));
#60820=CARTESIAN_POINT('Ctrl Pts',(-1.75997588499021,1.,3.71208146346454));
#60821=CARTESIAN_POINT('Ctrl Pts',(-1.75412641804148,-1.,3.70700269736876));
#60822=CARTESIAN_POINT('Ctrl Pts',(-1.75412641804148,1.,3.70700269736876));
#60823=CARTESIAN_POINT('Ctrl Pts',(-1.74830738046092,-1.,3.70190175673422));
#60824=CARTESIAN_POINT('Ctrl Pts',(-1.74830738046092,1.,3.70190175673422));
#60825=CARTESIAN_POINT('Ctrl Pts',(-1.74251908492589,-1.,3.6967785691046));
#60826=CARTESIAN_POINT('Ctrl Pts',(-1.74251908492589,1.,3.6967785691046));
#60827=CARTESIAN_POINT('Ctrl Pts',(-1.73676193254493,-1.,3.69163322647906));
#60828=CARTESIAN_POINT('Ctrl Pts',(-1.73676193254493,1.,3.69163322647906));
#60829=CARTESIAN_POINT('Ctrl Pts',(-1.73103640956647,-1.,3.68646597019188));
#60830=CARTESIAN_POINT('Ctrl Pts',(-1.73103640956647,1.,3.68646597019188));
#60831=CARTESIAN_POINT('Ctrl Pts',(-1.72534302437003,-1.,3.68127704936472));
#60832=CARTESIAN_POINT('Ctrl Pts',(-1.72534302437003,1.,3.68127704936472));
#60833=CARTESIAN_POINT('Ctrl Pts',(-1.71968225581787,-1.,3.67606660374665));
#60834=CARTESIAN_POINT('Ctrl Pts',(-1.71968225581787,1.,3.67606660374665));
#60835=CARTESIAN_POINT('Ctrl Pts',(-1.71405450210392,-1.,3.67083454901629));
#60836=CARTESIAN_POINT('Ctrl Pts',(-1.71405450210392,1.,3.67083454901629));
#60837=CARTESIAN_POINT('Ctrl Pts',(-1.70846001610983,-1.,3.6655804319893));
#60838=CARTESIAN_POINT('Ctrl Pts',(-1.70846001610983,1.,3.6655804319893));
#60839=CARTESIAN_POINT('Ctrl Pts',(-1.70289888566904,-1.,3.6603033877491));
#60840=CARTESIAN_POINT('Ctrl Pts',(-1.70289888566904,1.,3.6603033877491));
#60841=CARTESIAN_POINT('Ctrl Pts',(-1.69737117722559,-1.,3.65500246526798));
#60842=CARTESIAN_POINT('Ctrl Pts',(-1.69737117722559,1.,3.65500246526798));
#60843=CARTESIAN_POINT('Ctrl Pts',(-1.691877054817,-1.,3.64967689827393));
#60844=CARTESIAN_POINT('Ctrl Pts',(-1.691877054817,1.,3.64967689827393));
#60845=CARTESIAN_POINT('Ctrl Pts',(-1.68641690471455,-1.,3.64432638915199));
#60846=CARTESIAN_POINT('Ctrl Pts',(-1.68641690471455,1.,3.64432638915199));
#60847=CARTESIAN_POINT('Ctrl Pts',(-1.68099146651577,-1.,3.63895140887443));
#60848=CARTESIAN_POINT('Ctrl Pts',(-1.68099146651577,1.,3.63895140887443));
#60849=CARTESIAN_POINT('Ctrl Pts',(-1.67560193613145,-1.,3.63355343201211));
#60850=CARTESIAN_POINT('Ctrl Pts',(-1.67560193613145,1.,3.63355343201211));
#60851=CARTESIAN_POINT('Ctrl Pts',(-1.67024966008037,-1.,3.62813422105257));
#60852=CARTESIAN_POINT('Ctrl Pts',(-1.67024966008037,1.,3.62813422105257));
#60853=CARTESIAN_POINT('Ctrl Pts',(-1.66493585923853,-1.,3.62269517989104));
#60854=CARTESIAN_POINT('Ctrl Pts',(-1.66493585923853,1.,3.62269517989104));
#60855=CARTESIAN_POINT('Ctrl Pts',(-1.65966133399186,-1.,3.61723666482457));
#60856=CARTESIAN_POINT('Ctrl Pts',(-1.65966133399186,1.,3.61723666482457));
#60857=CARTESIAN_POINT('Ctrl Pts',(-1.65442619244327,-1.,3.61175734965129));
#60858=CARTESIAN_POINT('Ctrl Pts',(-1.65442619244327,1.,3.61175734965129));
#60859=CARTESIAN_POINT('Ctrl Pts',(-1.64922952425833,-1.,3.60625346556992));
#60860=CARTESIAN_POINT('Ctrl Pts',(-1.64922952425833,1.,3.60625346556992));
#60861=CARTESIAN_POINT('Ctrl Pts',(-1.6440700438558,-1.,3.6007202851384));
#60862=CARTESIAN_POINT('Ctrl Pts',(-1.6440700438558,1.,3.6007202851384));
#60863=CARTESIAN_POINT('Ctrl Pts',(-1.63894676675349,-1.,3.59515368334887));
#60864=CARTESIAN_POINT('Ctrl Pts',(-1.63894676675349,1.,3.59515368334887));
#60865=CARTESIAN_POINT('Ctrl Pts',(-1.63385971451259,-1.,3.58955176627876));
#60866=CARTESIAN_POINT('Ctrl Pts',(-1.63385971451259,1.,3.58955176627876));
#60867=CARTESIAN_POINT('Ctrl Pts',(-1.62881051550748,-1.,3.5839162577435));
#60868=CARTESIAN_POINT('Ctrl Pts',(-1.62881051550748,1.,3.5839162577435));
#60869=CARTESIAN_POINT('Ctrl Pts',(-1.62380329464851,-1.,3.57825455954405));
#60870=CARTESIAN_POINT('Ctrl Pts',(-1.62380329464851,1.,3.57825455954405));
#60871=CARTESIAN_POINT('Ctrl Pts',(-1.61884340915412,-1.,3.57257679609826));
#60872=CARTESIAN_POINT('Ctrl Pts',(-1.61884340915412,1.,3.57257679609826));
#60873=CARTESIAN_POINT('Ctrl Pts',(-1.61393581747522,-1.,3.56689200468404));
#60874=CARTESIAN_POINT('Ctrl Pts',(-1.61393581747522,1.,3.56689200468404));
#60875=CARTESIAN_POINT('Ctrl Pts',(-1.60908344685459,-1.,3.56120432482986));
#60876=CARTESIAN_POINT('Ctrl Pts',(-1.60908344685459,1.,3.56120432482986));
#60877=CARTESIAN_POINT('Ctrl Pts',(-1.60428584699848,-1.,3.55550985096117));
#60878=CARTESIAN_POINT('Ctrl Pts',(-1.60428584699848,1.,3.55550985096117));
#60879=CARTESIAN_POINT('Ctrl Pts',(-1.59953698113444,-1.,3.54979148634426));
#60880=CARTESIAN_POINT('Ctrl Pts',(-1.59953698113444,1.,3.54979148634426));
#60881=CARTESIAN_POINT('Ctrl Pts',(-1.5948276694975,-1.,3.544024581823));
#60882=CARTESIAN_POINT('Ctrl Pts',(-1.5948276694975,1.,3.544024581823));
#60883=CARTESIAN_POINT('Ctrl Pts',(-1.59014958368725,-1.,3.53818616861045));
#60884=CARTESIAN_POINT('Ctrl Pts',(-1.59014958368725,1.,3.53818616861045));
#60885=CARTESIAN_POINT('Ctrl Pts',(-1.58549906268083,-1.,3.53226378147068));
#60886=CARTESIAN_POINT('Ctrl Pts',(-1.58549906268083,1.,3.53226378147068));
#60887=CARTESIAN_POINT('Ctrl Pts',(-1.58088027227856,-1.,3.52626275334899));
#60888=CARTESIAN_POINT('Ctrl Pts',(-1.58088027227856,1.,3.52626275334899));
#60889=CARTESIAN_POINT('Ctrl Pts',(-1.5763104998818,-1.,3.52021847865961));
#60890=CARTESIAN_POINT('Ctrl Pts',(-1.5763104998818,1.,3.52021847865961));
#60891=CARTESIAN_POINT('Ctrl Pts',(-1.57181569799774,-1.,3.51418598431733));
#60892=CARTESIAN_POINT('Ctrl Pts',(-1.57181569799774,1.,3.51418598431733));
#60893=CARTESIAN_POINT('Ctrl Pts',(-1.56742097575041,-1.,3.50821771695427));
#60894=CARTESIAN_POINT('Ctrl Pts',(-1.56742097575041,1.,3.50821771695427));
#60895=CARTESIAN_POINT('Ctrl Pts',(-1.56314187758689,-1.,3.50234321621607));
#60896=CARTESIAN_POINT('Ctrl Pts',(-1.56314187758689,1.,3.50234321621607));
#60897=CARTESIAN_POINT('Ctrl Pts',(-1.55897703097859,-1.,3.49655185179623));
#60898=CARTESIAN_POINT('Ctrl Pts',(-1.55897703097859,1.,3.49655185179623));
#60899=CARTESIAN_POINT('Ctrl Pts',(-1.5548959590107,-1.,3.49076460877317));
#60900=CARTESIAN_POINT('Ctrl Pts',(-1.5548959590107,1.,3.49076460877317));
#60901=CARTESIAN_POINT('Ctrl Pts',(-1.55084702970382,-1.,3.48485155928414));
#60902=CARTESIAN_POINT('Ctrl Pts',(-1.55084702970382,1.,3.48485155928414));
#60903=CARTESIAN_POINT('Ctrl Pts',(-1.54678009290207,-1.,3.47868272898599));
#60904=CARTESIAN_POINT('Ctrl Pts',(-1.54678009290207,1.,3.47868272898599));
#60905=CARTESIAN_POINT('Ctrl Pts',(-1.54266605398152,-1.,3.47217189224576));
#60906=CARTESIAN_POINT('Ctrl Pts',(-1.54266605398152,1.,3.47217189224576));
#60907=CARTESIAN_POINT('Ctrl Pts',(-1.53851507915533,-1.,3.46531752207222));
#60908=CARTESIAN_POINT('Ctrl Pts',(-1.53851507915533,1.,3.46531752207222));
#60909=CARTESIAN_POINT('Ctrl Pts',(-1.53440195378902,-1.,3.45825932955273));
#60910=CARTESIAN_POINT('Ctrl Pts',(-1.53440195378902,1.,3.45825932955273));
#60911=CARTESIAN_POINT('Ctrl Pts',(-1.530462444618,-1.,3.45127136828667));
#60912=CARTESIAN_POINT('Ctrl Pts',(-1.530462444618,1.,3.45127136828667));
#60913=CARTESIAN_POINT('Ctrl Pts',(-1.52686242875717,-1.,3.44469547527));
#60914=CARTESIAN_POINT('Ctrl Pts',(-1.52686242875717,1.,3.44469547527));
#60915=CARTESIAN_POINT('Ctrl Pts',(-1.52377348950429,-1.,3.43888895974182));
#60916=CARTESIAN_POINT('Ctrl Pts',(-1.52377348950429,1.,3.43888895974182));
#60917=CARTESIAN_POINT('Ctrl Pts',(-1.52134826724227,-1.,3.43417156977749));
#60918=CARTESIAN_POINT('Ctrl Pts',(-1.52134826724227,1.,3.43417156977749));
#60919=CARTESIAN_POINT('Ctrl Pts',(-1.51969006980792,-1.,3.43076036253384));
#60920=CARTESIAN_POINT('Ctrl Pts',(-1.51969006980792,1.,3.43076036253384));
#60921=CARTESIAN_POINT('Ctrl Pts',(-1.51901585838879,-1.,3.42915787669388));
#60922=CARTESIAN_POINT('Ctrl Pts',(-1.51901585838879,1.,3.42915787669388));
#60923=CARTESIAN_POINT('Ctrl Pts',(-1.51888450659497,-1.,3.42860527148835));
#60924=CARTESIAN_POINT('Ctrl Pts',(-1.51888450659497,1.,3.42860527148835));
#60925=CARTESIAN_POINT('Ctrl Pts',(-1.51896318668306,-1.,3.42852521763648));
#60926=CARTESIAN_POINT('Ctrl Pts',(-1.51896318668306,1.,3.42852521763648));
#60927=CARTESIAN_POINT('Ctrl Pts',(-1.519044091397,-1.,3.42855728381368));
#60928=CARTESIAN_POINT('Ctrl Pts',(-1.519044091397,1.,3.42855728381368));
#60929=CARTESIAN_POINT('',(-1.83867539237861,1.,3.77614523045147));
#60930=CARTESIAN_POINT('Ctrl Pts',(-1.83867539237861,1.,3.77614523045147));
#60931=CARTESIAN_POINT('Ctrl Pts',(-1.83742834010821,1.,3.77518714458232));
#60932=CARTESIAN_POINT('Ctrl Pts',(-1.83493697935064,1.,3.77326886065484));
#60933=CARTESIAN_POINT('Ctrl Pts',(-1.83120816956515,1.,3.77038509819777));
#60934=CARTESIAN_POINT('Ctrl Pts',(-1.82625289221933,1.,3.76652740355856));
#60935=CARTESIAN_POINT('Ctrl Pts',(-1.82008629694924,1.,3.76168412709652));
#60936=CARTESIAN_POINT('Ctrl Pts',(-1.81394729834032,1.,3.75681965683995));
#60937=CARTESIAN_POINT('Ctrl Pts',(-1.80783603939662,1.,3.75193395888069));
#60938=CARTESIAN_POINT('Ctrl Pts',(-1.80175271485519,1.,3.74702700874954));
#60939=CARTESIAN_POINT('Ctrl Pts',(-1.79569757859041,1.,3.74209880351667));
#60940=CARTESIAN_POINT('Ctrl Pts',(-1.78967092823139,1.,3.73714934729962));
#60941=CARTESIAN_POINT('Ctrl Pts',(-1.78367308442682,1.,3.73217863095022));
#60942=CARTESIAN_POINT('Ctrl Pts',(-1.77770437039606,1.,3.72718661205504));
#60943=CARTESIAN_POINT('Ctrl Pts',(-1.77176509401846,1.,3.72217319911429));
#60944=CARTESIAN_POINT('Ctrl Pts',(-1.76585552124549,1.,3.71713822377675));
#60945=CARTESIAN_POINT('Ctrl Pts',(-1.75997588499021,1.,3.71208146346454));
#60946=CARTESIAN_POINT('Ctrl Pts',(-1.75412641804148,1.,3.70700269736876));
#60947=CARTESIAN_POINT('Ctrl Pts',(-1.74830738046092,1.,3.70190175673422));
#60948=CARTESIAN_POINT('Ctrl Pts',(-1.74251908492589,1.,3.6967785691046));
#60949=CARTESIAN_POINT('Ctrl Pts',(-1.73676193254493,1.,3.69163322647906));
#60950=CARTESIAN_POINT('Ctrl Pts',(-1.73103640956647,1.,3.68646597019188));
#60951=CARTESIAN_POINT('Ctrl Pts',(-1.72534302437003,1.,3.68127704936472));
#60952=CARTESIAN_POINT('Ctrl Pts',(-1.71968225581787,1.,3.67606660374665));
#60953=CARTESIAN_POINT('Ctrl Pts',(-1.71405450210392,1.,3.67083454901629));
#60954=CARTESIAN_POINT('Ctrl Pts',(-1.70846001610983,1.,3.6655804319893));
#60955=CARTESIAN_POINT('Ctrl Pts',(-1.70289888566904,1.,3.6603033877491));
#60956=CARTESIAN_POINT('Ctrl Pts',(-1.69737117722559,1.,3.65500246526798));
#60957=CARTESIAN_POINT('Ctrl Pts',(-1.691877054817,1.,3.64967689827393));
#60958=CARTESIAN_POINT('Ctrl Pts',(-1.68641690471455,1.,3.64432638915199));
#60959=CARTESIAN_POINT('Ctrl Pts',(-1.68099146651577,1.,3.63895140887443));
#60960=CARTESIAN_POINT('Ctrl Pts',(-1.67560193613145,1.,3.63355343201211));
#60961=CARTESIAN_POINT('Ctrl Pts',(-1.67024966008037,1.,3.62813422105257));
#60962=CARTESIAN_POINT('Ctrl Pts',(-1.66493585923853,1.,3.62269517989104));
#60963=CARTESIAN_POINT('Ctrl Pts',(-1.65966133399186,1.,3.61723666482457));
#60964=CARTESIAN_POINT('Ctrl Pts',(-1.65442619244327,1.,3.61175734965129));
#60965=CARTESIAN_POINT('Ctrl Pts',(-1.64922952425833,1.,3.60625346556992));
#60966=CARTESIAN_POINT('Ctrl Pts',(-1.6440700438558,1.,3.6007202851384));
#60967=CARTESIAN_POINT('Ctrl Pts',(-1.63894676675349,1.,3.59515368334887));
#60968=CARTESIAN_POINT('Ctrl Pts',(-1.63385971451259,1.,3.58955176627876));
#60969=CARTESIAN_POINT('Ctrl Pts',(-1.62881051550748,1.,3.5839162577435));
#60970=CARTESIAN_POINT('Ctrl Pts',(-1.62380329464851,1.,3.57825455954405));
#60971=CARTESIAN_POINT('Ctrl Pts',(-1.61884340915412,1.,3.57257679609826));
#60972=CARTESIAN_POINT('Ctrl Pts',(-1.61393581747522,1.,3.56689200468404));
#60973=CARTESIAN_POINT('Ctrl Pts',(-1.60908344685459,1.,3.56120432482986));
#60974=CARTESIAN_POINT('Ctrl Pts',(-1.60428584699848,1.,3.55550985096117));
#60975=CARTESIAN_POINT('Ctrl Pts',(-1.59953698113444,1.,3.54979148634426));
#60976=CARTESIAN_POINT('Ctrl Pts',(-1.5948276694975,1.,3.544024581823));
#60977=CARTESIAN_POINT('Ctrl Pts',(-1.59014958368725,1.,3.53818616861045));
#60978=CARTESIAN_POINT('Ctrl Pts',(-1.58549906268083,1.,3.53226378147068));
#60979=CARTESIAN_POINT('Ctrl Pts',(-1.58088027227856,1.,3.52626275334899));
#60980=CARTESIAN_POINT('Ctrl Pts',(-1.5763104998818,1.,3.52021847865961));
#60981=CARTESIAN_POINT('Ctrl Pts',(-1.57181569799774,1.,3.51418598431733));
#60982=CARTESIAN_POINT('Ctrl Pts',(-1.56742097575041,1.,3.50821771695427));
#60983=CARTESIAN_POINT('Ctrl Pts',(-1.56314187758689,1.,3.50234321621607));
#60984=CARTESIAN_POINT('Ctrl Pts',(-1.55897703097859,1.,3.49655185179623));
#60985=CARTESIAN_POINT('Ctrl Pts',(-1.5548959590107,1.,3.49076460877317));
#60986=CARTESIAN_POINT('Ctrl Pts',(-1.55084702970382,1.,3.48485155928414));
#60987=CARTESIAN_POINT('Ctrl Pts',(-1.54678009290207,1.,3.47868272898599));
#60988=CARTESIAN_POINT('Ctrl Pts',(-1.54266605398152,1.,3.47217189224576));
#60989=CARTESIAN_POINT('Ctrl Pts',(-1.53851507915533,1.,3.46531752207222));
#60990=CARTESIAN_POINT('Ctrl Pts',(-1.53440195378902,1.,3.45825932955273));
#60991=CARTESIAN_POINT('Ctrl Pts',(-1.530462444618,1.,3.45127136828667));
#60992=CARTESIAN_POINT('Ctrl Pts',(-1.52686242875717,1.,3.44469547527));
#60993=CARTESIAN_POINT('Ctrl Pts',(-1.52377348950429,1.,3.43888895974182));
#60994=CARTESIAN_POINT('Ctrl Pts',(-1.52134826724227,1.,3.43417156977749));
#60995=CARTESIAN_POINT('Ctrl Pts',(-1.5198144909343,1.,3.4310163189349));
#60996=CARTESIAN_POINT('Ctrl Pts',(-1.51914806898539,1.,3.42946838852728));
#60997=CARTESIAN_POINT('Ctrl Pts',(-1.51895133295017,1.,3.42884302333978));
#60998=CARTESIAN_POINT('Ctrl Pts',(-1.51893924967231,1.,3.42864616361967));
#60999=CARTESIAN_POINT('Ctrl Pts',(-1.51895082866166,1.,3.42859860294378));
#61000=CARTESIAN_POINT('',(-1.83867539237861,0.,3.77614523045147));
#61001=CARTESIAN_POINT('Ctrl Pts',(-1.88088939428811,-1.,3.24418789321065));
#61002=CARTESIAN_POINT('Ctrl Pts',(-1.88088939428811,1.,3.24418789321065));
#61003=CARTESIAN_POINT('Ctrl Pts',(-1.8809110068042,-1.,3.24410359189733));
#61004=CARTESIAN_POINT('Ctrl Pts',(-1.8809110068042,1.,3.24410359189733));
#61005=CARTESIAN_POINT('Ctrl Pts',(-1.8810220187274,-1.,3.24408699284449));
#61006=CARTESIAN_POINT('Ctrl Pts',(-1.8810220187274,1.,3.24408699284449));
#61007=CARTESIAN_POINT('Ctrl Pts',(-1.88139187908347,-1.,3.24451807186964));
#61008=CARTESIAN_POINT('Ctrl Pts',(-1.88139187908347,1.,3.24451807186964));
#61009=CARTESIAN_POINT('Ctrl Pts',(-1.88229202583187,-1.,3.24600543790876));
#61010=CARTESIAN_POINT('Ctrl Pts',(-1.88229202583187,1.,3.24600543790876));
#61011=CARTESIAN_POINT('Ctrl Pts',(-1.88407708646435,-1.,3.24935200512055));
#61012=CARTESIAN_POINT('Ctrl Pts',(-1.88407708646435,1.,3.24935200512055));
#61013=CARTESIAN_POINT('Ctrl Pts',(-1.88646802523372,-1.,3.25408686339298));
#61014=CARTESIAN_POINT('Ctrl Pts',(-1.88646802523372,1.,3.25408686339298));
#61015=CARTESIAN_POINT('Ctrl Pts',(-1.88934996203508,-1.,3.2599988519361));
#61016=CARTESIAN_POINT('Ctrl Pts',(-1.88934996203508,1.,3.2599988519361));
#61017=CARTESIAN_POINT('Ctrl Pts',(-1.89255393500769,-1.,3.2667765388833));
#61018=CARTESIAN_POINT('Ctrl Pts',(-1.89255393500769,1.,3.2667765388833));
#61019=CARTESIAN_POINT('Ctrl Pts',(-1.89589172903662,-1.,3.27407108932908));
#61020=CARTESIAN_POINT('Ctrl Pts',(-1.89589172903662,1.,3.27407108932908));
#61021=CARTESIAN_POINT('Ctrl Pts',(-1.89918429230425,-1.,3.28154737912287));
#61022=CARTESIAN_POINT('Ctrl Pts',(-1.89918429230425,1.,3.28154737912287));
#61023=CARTESIAN_POINT('Ctrl Pts',(-1.9022897124757,-1.,3.28893448600364));
#61024=CARTESIAN_POINT('Ctrl Pts',(-1.9022897124757,1.,3.28893448600364));
#61025=CARTESIAN_POINT('Ctrl Pts',(-1.9051389186417,-1.,3.29608978722258));
#61026=CARTESIAN_POINT('Ctrl Pts',(-1.9051389186417,1.,3.29608978722258));
#61027=CARTESIAN_POINT('Ctrl Pts',(-1.90773912171424,-1.,3.30300595568341));
#61028=CARTESIAN_POINT('Ctrl Pts',(-1.90773912171424,1.,3.30300595568341));
#61029=CARTESIAN_POINT('Ctrl Pts',(-1.91014297830502,-1.,3.30975721158694));
#61030=CARTESIAN_POINT('Ctrl Pts',(-1.91014297830502,1.,3.30975721158694));
#61031=CARTESIAN_POINT('Ctrl Pts',(-1.91242616234459,-1.,3.31646052426395));
#61032=CARTESIAN_POINT('Ctrl Pts',(-1.91242616234459,1.,3.31646052426395));
#61033=CARTESIAN_POINT('Ctrl Pts',(-1.91466343916612,-1.,3.32323403454507));
#61034=CARTESIAN_POINT('Ctrl Pts',(-1.91466343916612,1.,3.32323403454507));
#61035=CARTESIAN_POINT('Ctrl Pts',(-1.91690081930297,-1.,3.33014884257812));
#61036=CARTESIAN_POINT('Ctrl Pts',(-1.91690081930297,1.,3.33014884257812));
#61037=CARTESIAN_POINT('Ctrl Pts',(-1.91914609610173,-1.,3.33721230709948));
#61038=CARTESIAN_POINT('Ctrl Pts',(-1.91914609610173,1.,3.33721230709948));
#61039=CARTESIAN_POINT('Ctrl Pts',(-1.92138450828378,-1.,3.34439448941915));
#61040=CARTESIAN_POINT('Ctrl Pts',(-1.92138450828378,1.,3.34439448941915));
#61041=CARTESIAN_POINT('Ctrl Pts',(-1.92358838440518,-1.,3.35164424847206));
#61042=CARTESIAN_POINT('Ctrl Pts',(-1.92358838440518,1.,3.35164424847206));
#61043=CARTESIAN_POINT('Ctrl Pts',(-1.92572846125763,-1.,3.35890824422976));
#61044=CARTESIAN_POINT('Ctrl Pts',(-1.92572846125763,1.,3.35890824422976));
#61045=CARTESIAN_POINT('Ctrl Pts',(-1.92778626543803,-1.,3.36615168657597));
#61046=CARTESIAN_POINT('Ctrl Pts',(-1.92778626543803,1.,3.36615168657597));
#61047=CARTESIAN_POINT('Ctrl Pts',(-1.92975993109897,-1.,3.37336807068078));
#61048=CARTESIAN_POINT('Ctrl Pts',(-1.92975993109897,1.,3.37336807068078));
#61049=CARTESIAN_POINT('Ctrl Pts',(-1.93165739093292,-1.,3.38056768525577));
#61050=CARTESIAN_POINT('Ctrl Pts',(-1.93165739093292,1.,3.38056768525577));
#61051=CARTESIAN_POINT('Ctrl Pts',(-1.93349233176794,-1.,3.38777076883267));
#61052=CARTESIAN_POINT('Ctrl Pts',(-1.93349233176794,1.,3.38777076883267));
#61053=CARTESIAN_POINT('Ctrl Pts',(-1.93527929945982,-1.,3.39499923640789));
#61054=CARTESIAN_POINT('Ctrl Pts',(-1.93527929945982,1.,3.39499923640789));
#61055=CARTESIAN_POINT('Ctrl Pts',(-1.93702857723089,-1.,3.40226802104093));
#61056=CARTESIAN_POINT('Ctrl Pts',(-1.93702857723089,1.,3.40226802104093));
#61057=CARTESIAN_POINT('Ctrl Pts',(-1.93874306008132,-1.,3.40957978266622));
#61058=CARTESIAN_POINT('Ctrl Pts',(-1.93874306008132,1.,3.40957978266622));
#61059=CARTESIAN_POINT('Ctrl Pts',(-1.94042111965237,-1.,3.41692971994082));
#61060=CARTESIAN_POINT('Ctrl Pts',(-1.94042111965237,1.,3.41692971994082));
#61061=CARTESIAN_POINT('Ctrl Pts',(-1.94205835913692,-1.,3.42430850941497));
#61062=CARTESIAN_POINT('Ctrl Pts',(-1.94205835913692,1.,3.42430850941497));
#61063=CARTESIAN_POINT('Ctrl Pts',(-1.94364973660285,-1.,3.43170586602436));
#61064=CARTESIAN_POINT('Ctrl Pts',(-1.94364973660285,1.,3.43170586602436));
#61065=CARTESIAN_POINT('Ctrl Pts',(-1.94519168842883,-1.,3.43911410197693));
#61066=CARTESIAN_POINT('Ctrl Pts',(-1.94519168842883,1.,3.43911410197693));
#61067=CARTESIAN_POINT('Ctrl Pts',(-1.94668377715332,-1.,3.44653088665685));
#61068=CARTESIAN_POINT('Ctrl Pts',(-1.94668377715332,1.,3.44653088665685));
#61069=CARTESIAN_POINT('Ctrl Pts',(-1.94812754766524,-1.,3.45395731584051));
#61070=CARTESIAN_POINT('Ctrl Pts',(-1.94812754766524,1.,3.45395731584051));
#61071=CARTESIAN_POINT('Ctrl Pts',(-1.94952575850196,-1.,3.46139661060959));
#61072=CARTESIAN_POINT('Ctrl Pts',(-1.94952575850196,1.,3.46139661060959));
#61073=CARTESIAN_POINT('Ctrl Pts',(-1.95088147859876,-1.,3.4688525897419));
#61074=CARTESIAN_POINT('Ctrl Pts',(-1.95088147859876,1.,3.4688525897419));
#61075=CARTESIAN_POINT('Ctrl Pts',(-1.95219722189878,-1.,3.47632820495926));
#61076=CARTESIAN_POINT('Ctrl Pts',(-1.95219722189878,1.,3.47632820495926));
#61077=CARTESIAN_POINT('Ctrl Pts',(-1.95347412486316,-1.,3.48382414832648));
#61078=CARTESIAN_POINT('Ctrl Pts',(-1.95347412486316,1.,3.48382414832648));
#61079=CARTESIAN_POINT('Ctrl Pts',(-1.95471236969653,-1.,3.49133956289154));
#61080=CARTESIAN_POINT('Ctrl Pts',(-1.95471236969653,1.,3.49133956289154));
#61081=CARTESIAN_POINT('Ctrl Pts',(-1.9559115382367,-1.,3.49887263575602));
#61082=CARTESIAN_POINT('Ctrl Pts',(-1.9559115382367,1.,3.49887263575602));
#61083=CARTESIAN_POINT('Ctrl Pts',(-1.95707099606514,-1.,3.50642124159913));
#61084=CARTESIAN_POINT('Ctrl Pts',(-1.95707099606514,1.,3.50642124159913));
#61085=CARTESIAN_POINT('Ctrl Pts',(-1.95819025316768,-1.,3.51398354617772));
#61086=CARTESIAN_POINT('Ctrl Pts',(-1.95819025316768,1.,3.51398354617772));
#61087=CARTESIAN_POINT('Ctrl Pts',(-1.95926936324436,-1.,3.52155867431438));
#61088=CARTESIAN_POINT('Ctrl Pts',(-1.95926936324436,1.,3.52155867431438));
#61089=CARTESIAN_POINT('Ctrl Pts',(-1.96030879411534,-1.,3.52914648844289));
#61090=CARTESIAN_POINT('Ctrl Pts',(-1.96030879411534,1.,3.52914648844289));
#61091=CARTESIAN_POINT('Ctrl Pts',(-1.96130926212661,-1.,3.53674730625759));
#61092=CARTESIAN_POINT('Ctrl Pts',(-1.96130926212661,1.,3.53674730625759));
#61093=CARTESIAN_POINT('Ctrl Pts',(-1.96227157573058,-1.,3.54436163300425));
#61094=CARTESIAN_POINT('Ctrl Pts',(-1.96227157573058,1.,3.54436163300425));
#61095=CARTESIAN_POINT('Ctrl Pts',(-1.96319648628667,-1.,3.55198990600929));
#61096=CARTESIAN_POINT('Ctrl Pts',(-1.96319648628667,1.,3.55198990600929));
#61097=CARTESIAN_POINT('Ctrl Pts',(-1.96408450906868,-1.,3.55963218706201));
#61098=CARTESIAN_POINT('Ctrl Pts',(-1.96408450906868,1.,3.55963218706201));
#61099=CARTESIAN_POINT('Ctrl Pts',(-1.96493594634643,-1.,3.56728820357933));
#61100=CARTESIAN_POINT('Ctrl Pts',(-1.96493594634643,1.,3.56728820357933));
#61101=CARTESIAN_POINT('Ctrl Pts',(-1.96575096652857,-1.,3.57495748601088));
#61102=CARTESIAN_POINT('Ctrl Pts',(-1.96575096652857,1.,3.57495748601088));
#61103=CARTESIAN_POINT('Ctrl Pts',(-1.9665296668894,-1.,3.58263947663884));
#61104=CARTESIAN_POINT('Ctrl Pts',(-1.9665296668894,1.,3.58263947663884));
#61105=CARTESIAN_POINT('Ctrl Pts',(-1.96727213799507,-1.,3.5903336402273));
#61106=CARTESIAN_POINT('Ctrl Pts',(-1.96727213799507,1.,3.5903336402273));
#61107=CARTESIAN_POINT('Ctrl Pts',(-1.96797854118257,-1.,3.59803959819725));
#61108=CARTESIAN_POINT('Ctrl Pts',(-1.96797854118257,1.,3.59803959819725));
#61109=CARTESIAN_POINT('Ctrl Pts',(-1.96864911885775,-1.,3.60575714017676));
#61110=CARTESIAN_POINT('Ctrl Pts',(-1.96864911885775,1.,3.60575714017676));
#61111=CARTESIAN_POINT('Ctrl Pts',(-1.96928416040712,-1.,3.61348615496393));
#61112=CARTESIAN_POINT('Ctrl Pts',(-1.96928416040712,1.,3.61348615496393));
#61113=CARTESIAN_POINT('Ctrl Pts',(-1.96988398129888,-1.,3.62122658401722));
#61114=CARTESIAN_POINT('Ctrl Pts',(-1.96988398129888,1.,3.62122658401722));
#61115=CARTESIAN_POINT('Ctrl Pts',(-1.97044889850518,-1.,3.62897836973397));
#61116=CARTESIAN_POINT('Ctrl Pts',(-1.97044889850518,1.,3.62897836973397));
#61117=CARTESIAN_POINT('Ctrl Pts',(-1.97097920454698,-1.,3.63674139590853));
#61118=CARTESIAN_POINT('Ctrl Pts',(-1.97097920454698,1.,3.63674139590853));
#61119=CARTESIAN_POINT('Ctrl Pts',(-1.97147515441539,-1.,3.64451546724221));
#61120=CARTESIAN_POINT('Ctrl Pts',(-1.97147515441539,1.,3.64451546724221));
#61121=CARTESIAN_POINT('Ctrl Pts',(-1.97193697240645,-1.,3.65230034717364));
#61122=CARTESIAN_POINT('Ctrl Pts',(-1.97193697240645,1.,3.65230034717364));
#61123=CARTESIAN_POINT('Ctrl Pts',(-1.97236485439317,-1.,3.66009578166865));
#61124=CARTESIAN_POINT('Ctrl Pts',(-1.97236485439317,1.,3.66009578166865));
#61125=CARTESIAN_POINT('Ctrl Pts',(-1.9727589719863,-1.,3.66790152751984));
#61126=CARTESIAN_POINT('Ctrl Pts',(-1.9727589719863,1.,3.66790152751984));
#61127=CARTESIAN_POINT('Ctrl Pts',(-1.97311947678035,-1.,3.67571738106175));
#61128=CARTESIAN_POINT('Ctrl Pts',(-1.97311947678035,1.,3.67571738106175));
#61129=CARTESIAN_POINT('Ctrl Pts',(-1.97344650303631,-1.,3.68354319913416));
#61130=CARTESIAN_POINT('Ctrl Pts',(-1.97344650303631,1.,3.68354319913416));
#61131=CARTESIAN_POINT('Ctrl Pts',(-1.97374016224397,-1.,3.69137888597855));
#61132=CARTESIAN_POINT('Ctrl Pts',(-1.97374016224397,1.,3.69137888597855));
#61133=CARTESIAN_POINT('Ctrl Pts',(-1.97394846382289,-1.,3.69765528558292));
#61134=CARTESIAN_POINT('Ctrl Pts',(-1.97394846382289,1.,3.69765528558292));
#61135=CARTESIAN_POINT('Ctrl Pts',(-1.97408973726149,-1.,3.70236698911837));
#61136=CARTESIAN_POINT('Ctrl Pts',(-1.97408973726149,1.,3.70236698911837));
#61137=CARTESIAN_POINT('Ctrl Pts',(-1.974177276451,-1.,3.7055100813194));
#61138=CARTESIAN_POINT('Ctrl Pts',(-1.974177276451,1.,3.7055100813194));
#61139=CARTESIAN_POINT('Ctrl Pts',(-1.97421938526992,-1.,3.70708211654725));
#61140=CARTESIAN_POINT('Ctrl Pts',(-1.97421938526992,1.,3.70708211654725));
#61141=CARTESIAN_POINT('',(-1.88097764062542,1.,3.24413672884902));
#61142=CARTESIAN_POINT('Ctrl Pts',(-1.88097764062542,-1.,3.24413672884902));
#61143=CARTESIAN_POINT('Ctrl Pts',(-1.88097764062542,-0.666666666666667,
3.24413672884902));
#61144=CARTESIAN_POINT('Ctrl Pts',(-1.88097764062542,-0.333333333333333,
3.24413672884902));
#61145=CARTESIAN_POINT('Ctrl Pts',(-1.88097764062542,0.333333333333333,
3.24413672884902));
#61146=CARTESIAN_POINT('Ctrl Pts',(-1.88097764062542,0.666666666666667,
3.24413672884902));
#61147=CARTESIAN_POINT('Ctrl Pts',(-1.88097764062542,1.,3.24413672884902));
#61148=CARTESIAN_POINT('',(-1.97421938526992,1.,3.70708211654725));
#61149=CARTESIAN_POINT('',(-1.97421938526992,0.,3.70708211654725));
#61150=CARTESIAN_POINT('Ctrl Pts',(-1.88097764062542,1.,3.24413672884902));
#61151=CARTESIAN_POINT('Ctrl Pts',(-1.88102292397987,1.,3.24415531671311));
#61152=CARTESIAN_POINT('Ctrl Pts',(-1.88117508446657,1.,3.24428080352952));
#61153=CARTESIAN_POINT('Ctrl Pts',(-1.88156537699118,1.,3.24480754675942));
#61154=CARTESIAN_POINT('Ctrl Pts',(-1.88242596600422,1.,3.24625654410705));
#61155=CARTESIAN_POINT('Ctrl Pts',(-1.88407708646435,1.,3.24935200512055));
#61156=CARTESIAN_POINT('Ctrl Pts',(-1.88646802523372,1.,3.25408686339298));
#61157=CARTESIAN_POINT('Ctrl Pts',(-1.88934996203508,1.,3.2599988519361));
#61158=CARTESIAN_POINT('Ctrl Pts',(-1.89255393500769,1.,3.2667765388833));
#61159=CARTESIAN_POINT('Ctrl Pts',(-1.89589172903662,1.,3.27407108932908));
#61160=CARTESIAN_POINT('Ctrl Pts',(-1.89918429230425,1.,3.28154737912287));
#61161=CARTESIAN_POINT('Ctrl Pts',(-1.9022897124757,1.,3.28893448600364));
#61162=CARTESIAN_POINT('Ctrl Pts',(-1.9051389186417,1.,3.29608978722258));
#61163=CARTESIAN_POINT('Ctrl Pts',(-1.90773912171424,1.,3.30300595568341));
#61164=CARTESIAN_POINT('Ctrl Pts',(-1.91014297830502,1.,3.30975721158694));
#61165=CARTESIAN_POINT('Ctrl Pts',(-1.91242616234459,1.,3.31646052426395));
#61166=CARTESIAN_POINT('Ctrl Pts',(-1.91466343916612,1.,3.32323403454507));
#61167=CARTESIAN_POINT('Ctrl Pts',(-1.91690081930297,1.,3.33014884257812));
#61168=CARTESIAN_POINT('Ctrl Pts',(-1.91914609610173,1.,3.33721230709948));
#61169=CARTESIAN_POINT('Ctrl Pts',(-1.92138450828378,1.,3.34439448941915));
#61170=CARTESIAN_POINT('Ctrl Pts',(-1.92358838440518,1.,3.35164424847206));
#61171=CARTESIAN_POINT('Ctrl Pts',(-1.92572846125763,1.,3.35890824422976));
#61172=CARTESIAN_POINT('Ctrl Pts',(-1.92778626543803,1.,3.36615168657597));
#61173=CARTESIAN_POINT('Ctrl Pts',(-1.92975993109897,1.,3.37336807068078));
#61174=CARTESIAN_POINT('Ctrl Pts',(-1.93165739093292,1.,3.38056768525577));
#61175=CARTESIAN_POINT('Ctrl Pts',(-1.93349233176794,1.,3.38777076883267));
#61176=CARTESIAN_POINT('Ctrl Pts',(-1.93527929945982,1.,3.39499923640789));
#61177=CARTESIAN_POINT('Ctrl Pts',(-1.93702857723089,1.,3.40226802104093));
#61178=CARTESIAN_POINT('Ctrl Pts',(-1.93874306008132,1.,3.40957978266622));
#61179=CARTESIAN_POINT('Ctrl Pts',(-1.94042111965237,1.,3.41692971994082));
#61180=CARTESIAN_POINT('Ctrl Pts',(-1.94205835913692,1.,3.42430850941497));
#61181=CARTESIAN_POINT('Ctrl Pts',(-1.94364973660285,1.,3.43170586602436));
#61182=CARTESIAN_POINT('Ctrl Pts',(-1.94519168842883,1.,3.43911410197693));
#61183=CARTESIAN_POINT('Ctrl Pts',(-1.94668377715332,1.,3.44653088665685));
#61184=CARTESIAN_POINT('Ctrl Pts',(-1.94812754766524,1.,3.45395731584051));
#61185=CARTESIAN_POINT('Ctrl Pts',(-1.94952575850196,1.,3.46139661060959));
#61186=CARTESIAN_POINT('Ctrl Pts',(-1.95088147859876,1.,3.4688525897419));
#61187=CARTESIAN_POINT('Ctrl Pts',(-1.95219722189878,1.,3.47632820495926));
#61188=CARTESIAN_POINT('Ctrl Pts',(-1.95347412486316,1.,3.48382414832648));
#61189=CARTESIAN_POINT('Ctrl Pts',(-1.95471236969653,1.,3.49133956289154));
#61190=CARTESIAN_POINT('Ctrl Pts',(-1.9559115382367,1.,3.49887263575602));
#61191=CARTESIAN_POINT('Ctrl Pts',(-1.95707099606514,1.,3.50642124159913));
#61192=CARTESIAN_POINT('Ctrl Pts',(-1.95819025316768,1.,3.51398354617772));
#61193=CARTESIAN_POINT('Ctrl Pts',(-1.95926936324436,1.,3.52155867431438));
#61194=CARTESIAN_POINT('Ctrl Pts',(-1.96030879411534,1.,3.52914648844289));
#61195=CARTESIAN_POINT('Ctrl Pts',(-1.96130926212661,1.,3.53674730625759));
#61196=CARTESIAN_POINT('Ctrl Pts',(-1.96227157573058,1.,3.54436163300425));
#61197=CARTESIAN_POINT('Ctrl Pts',(-1.96319648628667,1.,3.55198990600929));
#61198=CARTESIAN_POINT('Ctrl Pts',(-1.96408450906868,1.,3.55963218706201));
#61199=CARTESIAN_POINT('Ctrl Pts',(-1.96493594634643,1.,3.56728820357933));
#61200=CARTESIAN_POINT('Ctrl Pts',(-1.96575096652857,1.,3.57495748601088));
#61201=CARTESIAN_POINT('Ctrl Pts',(-1.9665296668894,1.,3.58263947663884));
#61202=CARTESIAN_POINT('Ctrl Pts',(-1.96727213799507,1.,3.5903336402273));
#61203=CARTESIAN_POINT('Ctrl Pts',(-1.96797854118257,1.,3.59803959819725));
#61204=CARTESIAN_POINT('Ctrl Pts',(-1.96864911885775,1.,3.60575714017676));
#61205=CARTESIAN_POINT('Ctrl Pts',(-1.96928416040712,1.,3.61348615496393));
#61206=CARTESIAN_POINT('Ctrl Pts',(-1.96988398129888,1.,3.62122658401722));
#61207=CARTESIAN_POINT('Ctrl Pts',(-1.97044889850518,1.,3.62897836973397));
#61208=CARTESIAN_POINT('Ctrl Pts',(-1.97097920454698,1.,3.63674139590853));
#61209=CARTESIAN_POINT('Ctrl Pts',(-1.97147515441539,1.,3.64451546724221));
#61210=CARTESIAN_POINT('Ctrl Pts',(-1.97193697240645,1.,3.65230034717364));
#61211=CARTESIAN_POINT('Ctrl Pts',(-1.97236485439317,1.,3.66009578166865));
#61212=CARTESIAN_POINT('Ctrl Pts',(-1.9727589719863,1.,3.66790152751984));
#61213=CARTESIAN_POINT('Ctrl Pts',(-1.97311947678035,1.,3.67571738106175));
#61214=CARTESIAN_POINT('Ctrl Pts',(-1.97344650303631,1.,3.68354319913416));
#61215=CARTESIAN_POINT('Ctrl Pts',(-1.97374016224397,1.,3.69137888597855));
#61216=CARTESIAN_POINT('Ctrl Pts',(-1.97394846382289,1.,3.69765528558292));
#61217=CARTESIAN_POINT('Ctrl Pts',(-1.97408973726149,1.,3.70236698911837));
#61218=CARTESIAN_POINT('Ctrl Pts',(-1.974177276451,1.,3.7055100813194));
#61219=CARTESIAN_POINT('Ctrl Pts',(-1.97421938526992,1.,3.70708211654725));
#61220=CARTESIAN_POINT('Origin',(-1.97421938526992,0.,3.70708211654725));
#61221=CARTESIAN_POINT('',(-1.83867539237861,1.,3.77614523045147));
#61222=CARTESIAN_POINT('Origin',(0.,0.,0.));
#61223=CARTESIAN_POINT('',(-2.03660101169564,1.,3.14877060440425));
#61224=CARTESIAN_POINT('Origin',(0.,1.,0.));
#61225=CARTESIAN_POINT('Ctrl Pts',(-2.03660101169564,1.,3.14877060440425));
#61226=CARTESIAN_POINT('Ctrl Pts',(-2.03660101169564,0.666666666666667,
3.14877060440425));
#61227=CARTESIAN_POINT('Ctrl Pts',(-2.03660101169564,0.333333333333333,
3.14877060440425));
#61228=CARTESIAN_POINT('Ctrl Pts',(-2.03660101169564,-0.333333333333333,
3.14877060440425));
#61229=CARTESIAN_POINT('Ctrl Pts',(-2.03660101169564,-0.666666666666667,
3.14877060440425));
#61230=CARTESIAN_POINT('Ctrl Pts',(-2.03660101169564,-1.,3.14877060440425));
#61231=CARTESIAN_POINT('Ctrl Pts',(-2.40675750623143,-1.,3.44202241512147));
#61232=CARTESIAN_POINT('Ctrl Pts',(-2.40675750623143,1.,3.44202241512147));
#61233=CARTESIAN_POINT('Ctrl Pts',(-2.40537592959345,-1.,3.44127120683402));
#61234=CARTESIAN_POINT('Ctrl Pts',(-2.40537592959345,1.,3.44127120683402));
#61235=CARTESIAN_POINT('Ctrl Pts',(-2.40261515590099,-1.,3.43976627485223));
#61236=CARTESIAN_POINT('Ctrl Pts',(-2.40261515590099,1.,3.43976627485223));
#61237=CARTESIAN_POINT('Ctrl Pts',(-2.39848113411429,-1.,3.43750133066036));
#61238=CARTESIAN_POINT('Ctrl Pts',(-2.39848113411429,1.,3.43750133066036));
#61239=CARTESIAN_POINT('Ctrl Pts',(-2.39298338805823,-1.,3.43446630680436));
#61240=CARTESIAN_POINT('Ctrl Pts',(-2.39298338805823,1.,3.43446630680436));
#61241=CARTESIAN_POINT('Ctrl Pts',(-2.38613505844641,-1.,3.43064732714472));
#61242=CARTESIAN_POINT('Ctrl Pts',(-2.38613505844641,1.,3.43064732714472));
#61243=CARTESIAN_POINT('Ctrl Pts',(-2.37931067029517,-1.,3.42680309755241));
#61244=CARTESIAN_POINT('Ctrl Pts',(-2.37931067029517,1.,3.42680309755241));
#61245=CARTESIAN_POINT('Ctrl Pts',(-2.37251035954351,-1.,3.42293356216595));
#61246=CARTESIAN_POINT('Ctrl Pts',(-2.37251035954351,1.,3.42293356216595));
#61247=CARTESIAN_POINT('Ctrl Pts',(-2.36573431470314,-1.,3.41903866635384));
#61248=CARTESIAN_POINT('Ctrl Pts',(-2.36573431470314,1.,3.41903866635384));
#61249=CARTESIAN_POINT('Ctrl Pts',(-2.35898278606449,-1.,3.4151183675076));
#61250=CARTESIAN_POINT('Ctrl Pts',(-2.35898278606449,1.,3.4151183675076));
#61251=CARTESIAN_POINT('Ctrl Pts',(-2.35225606823649,-1.,3.41117262313464));
#61252=CARTESIAN_POINT('Ctrl Pts',(-2.35225606823649,1.,3.41117262313464));
#61253=CARTESIAN_POINT('Ctrl Pts',(-2.34555447648901,-1.,3.40720137403888));
#61254=CARTESIAN_POINT('Ctrl Pts',(-2.34555447648901,1.,3.40720137403888));
#61255=CARTESIAN_POINT('Ctrl Pts',(-2.33887832342715,-1.,3.40320452776646));
#61256=CARTESIAN_POINT('Ctrl Pts',(-2.33887832342715,1.,3.40320452776646));
#61257=CARTESIAN_POINT('Ctrl Pts',(-2.33222789882601,-1.,3.39918194578115));
#61258=CARTESIAN_POINT('Ctrl Pts',(-2.33222789882601,1.,3.39918194578115));
#61259=CARTESIAN_POINT('Ctrl Pts',(-2.32560343902683,-1.,3.39513342020045));
#61260=CARTESIAN_POINT('Ctrl Pts',(-2.32560343902683,1.,3.39513342020045));
#61261=CARTESIAN_POINT('Ctrl Pts',(-2.31900513925627,-1.,3.39105869475112));
#61262=CARTESIAN_POINT('Ctrl Pts',(-2.31900513925627,1.,3.39105869475112));
#61263=CARTESIAN_POINT('Ctrl Pts',(-2.31243319489505,-1.,3.38695751492659));
#61264=CARTESIAN_POINT('Ctrl Pts',(-2.31243319489505,1.,3.38695751492659));
#61265=CARTESIAN_POINT('Ctrl Pts',(-2.30588783640389,-1.,3.38282967336676));
#61266=CARTESIAN_POINT('Ctrl Pts',(-2.30588783640389,1.,3.38282967336676));
#61267=CARTESIAN_POINT('Ctrl Pts',(-2.29936936127588,-1.,3.37867504959382));
#61268=CARTESIAN_POINT('Ctrl Pts',(-2.29936936127588,1.,3.37867504959382));
#61269=CARTESIAN_POINT('Ctrl Pts',(-2.2928781800731,-1.,3.37449367172707));
#61270=CARTESIAN_POINT('Ctrl Pts',(-2.2928781800731,1.,3.37449367172707));
#61271=CARTESIAN_POINT('Ctrl Pts',(-2.28641481081045,-1.,3.37028570206357));
#61272=CARTESIAN_POINT('Ctrl Pts',(-2.28641481081045,1.,3.37028570206357));
#61273=CARTESIAN_POINT('Ctrl Pts',(-2.27997979457968,-1.,3.36605130712978));
#61274=CARTESIAN_POINT('Ctrl Pts',(-2.27997979457968,1.,3.36605130712978));
#61275=CARTESIAN_POINT('Ctrl Pts',(-2.27357362620902,-1.,3.36179055004369));
#61276=CARTESIAN_POINT('Ctrl Pts',(-2.27357362620902,1.,3.36179055004369));
#61277=CARTESIAN_POINT('Ctrl Pts',(-2.26719668579921,-1.,3.35750328523077));
#61278=CARTESIAN_POINT('Ctrl Pts',(-2.26719668579921,1.,3.35750328523077));
#61279=CARTESIAN_POINT('Ctrl Pts',(-2.26084915222484,-1.,3.35318902552676));
#61280=CARTESIAN_POINT('Ctrl Pts',(-2.26084915222484,1.,3.35318902552676));
#61281=CARTESIAN_POINT('Ctrl Pts',(-2.25453097693524,-1.,3.34884690292342));
#61282=CARTESIAN_POINT('Ctrl Pts',(-2.25453097693524,1.,3.34884690292342));
#61283=CARTESIAN_POINT('Ctrl Pts',(-2.24824207678288,-1.,3.34447596770768));
#61284=CARTESIAN_POINT('Ctrl Pts',(-2.24824207678288,1.,3.34447596770768));
#61285=CARTESIAN_POINT('Ctrl Pts',(-2.24198249391437,-1.,3.34007543738044));
#61286=CARTESIAN_POINT('Ctrl Pts',(-2.24198249391437,1.,3.34007543738044));
#61287=CARTESIAN_POINT('Ctrl Pts',(-2.2357525632881,-1.,3.33564495756478));
#61288=CARTESIAN_POINT('Ctrl Pts',(-2.2357525632881,1.,3.33564495756478));
#61289=CARTESIAN_POINT('Ctrl Pts',(-2.22955308907221,-1.,3.33118487773593));
#61290=CARTESIAN_POINT('Ctrl Pts',(-2.22955308907221,1.,3.33118487773593));
#61291=CARTESIAN_POINT('Ctrl Pts',(-2.22338548312758,-1.,3.32669646722871));
#61292=CARTESIAN_POINT('Ctrl Pts',(-2.22338548312758,1.,3.32669646722871));
#61293=CARTESIAN_POINT('Ctrl Pts',(-2.21725135110889,-1.,3.32218125618955));
#61294=CARTESIAN_POINT('Ctrl Pts',(-2.21725135110889,1.,3.32218125618955));
#61295=CARTESIAN_POINT('Ctrl Pts',(-2.21115211847872,-1.,3.31764044024231));
#61296=CARTESIAN_POINT('Ctrl Pts',(-2.21115211847872,1.,3.31764044024231));
#61297=CARTESIAN_POINT('Ctrl Pts',(-2.20508863150608,-1.,3.3130742460895));
#61298=CARTESIAN_POINT('Ctrl Pts',(-2.20508863150608,1.,3.3130742460895));
#61299=CARTESIAN_POINT('Ctrl Pts',(-2.19906078949924,-1.,3.30848134694596));
#61300=CARTESIAN_POINT('Ctrl Pts',(-2.19906078949924,1.,3.30848134694596));
#61301=CARTESIAN_POINT('Ctrl Pts',(-2.19306710376112,-1.,3.30385816281831));
#61302=CARTESIAN_POINT('Ctrl Pts',(-2.19306710376112,1.,3.30385816281831));
#61303=CARTESIAN_POINT('Ctrl Pts',(-2.18710556500325,-1.,3.29920022557635));
#61304=CARTESIAN_POINT('Ctrl Pts',(-2.18710556500325,1.,3.29920022557635));
#61305=CARTESIAN_POINT('Ctrl Pts',(-2.18117455557062,-1.,3.29450361500484));
#61306=CARTESIAN_POINT('Ctrl Pts',(-2.18117455557062,1.,3.29450361500484));
#61307=CARTESIAN_POINT('Ctrl Pts',(-2.17527380048422,-1.,3.28976645712566));
#61308=CARTESIAN_POINT('Ctrl Pts',(-2.17527380048422,1.,3.28976645712566));
#61309=CARTESIAN_POINT('Ctrl Pts',(-2.16940517773459,-1.,3.2849901997973));
#61310=CARTESIAN_POINT('Ctrl Pts',(-2.16940517773459,1.,3.2849901997973));
#61311=CARTESIAN_POINT('Ctrl Pts',(-2.16357391934434,-1.,3.28018150841414));
#61312=CARTESIAN_POINT('Ctrl Pts',(-2.16357391934434,1.,3.28018150841414));
#61313=CARTESIAN_POINT('Ctrl Pts',(-2.15778690038359,-1.,3.27534954469206));
#61314=CARTESIAN_POINT('Ctrl Pts',(-2.15778690038359,1.,3.27534954469206));
#61315=CARTESIAN_POINT('Ctrl Pts',(-2.15205043199818,-1.,3.27050245897244));
#61316=CARTESIAN_POINT('Ctrl Pts',(-2.15205043199818,1.,3.27050245897244));
#61317=CARTESIAN_POINT('Ctrl Pts',(-2.14636805295663,-1.,3.26564388189764));
#61318=CARTESIAN_POINT('Ctrl Pts',(-2.14636805295663,1.,3.26564388189764));
#61319=CARTESIAN_POINT('Ctrl Pts',(-2.14073870754257,-1.,3.26077002641868));
#61320=CARTESIAN_POINT('Ctrl Pts',(-2.14073870754257,1.,3.26077002641868));
#61321=CARTESIAN_POINT('Ctrl Pts',(-2.13515375878786,-1.,3.25586495065027));
#61322=CARTESIAN_POINT('Ctrl Pts',(-2.13515375878786,1.,3.25586495065027));
#61323=CARTESIAN_POINT('Ctrl Pts',(-2.1296002839681,-1.,3.25090574493994));
#61324=CARTESIAN_POINT('Ctrl Pts',(-2.1296002839681,1.,3.25090574493994));
#61325=CARTESIAN_POINT('Ctrl Pts',(-2.12406646410943,-1.,3.24587102613347));
#61326=CARTESIAN_POINT('Ctrl Pts',(-2.12406646410943,1.,3.24587102613347));
#61327=CARTESIAN_POINT('Ctrl Pts',(-2.11854673326972,-1.,3.24074905517282));
#61328=CARTESIAN_POINT('Ctrl Pts',(-2.11854673326972,1.,3.24074905517282));
#61329=CARTESIAN_POINT('Ctrl Pts',(-2.11304604021784,-1.,3.23554444767115));
#61330=CARTESIAN_POINT('Ctrl Pts',(-2.11304604021784,1.,3.23554444767115));
#61331=CARTESIAN_POINT('Ctrl Pts',(-2.1075869964248,-1.,3.23028945793334));
#61332=CARTESIAN_POINT('Ctrl Pts',(-2.1075869964248,1.,3.23028945793334));
#61333=CARTESIAN_POINT('Ctrl Pts',(-2.10220384298533,-1.,3.22503437553496));
#61334=CARTESIAN_POINT('Ctrl Pts',(-2.10220384298533,1.,3.22503437553496));
#61335=CARTESIAN_POINT('Ctrl Pts',(-2.09692958434933,-1.,3.21982707347067));
#61336=CARTESIAN_POINT('Ctrl Pts',(-2.09692958434933,1.,3.21982707347067));
#61337=CARTESIAN_POINT('Ctrl Pts',(-2.0917841946046,-1.,3.2146942960168));
#61338=CARTESIAN_POINT('Ctrl Pts',(-2.0917841946046,1.,3.2146942960168));
#61339=CARTESIAN_POINT('Ctrl Pts',(-2.08676465517435,-1.,3.20962575845433));
#61340=CARTESIAN_POINT('Ctrl Pts',(-2.08676465517435,1.,3.20962575845433));
#61341=CARTESIAN_POINT('Ctrl Pts',(-2.08182850370816,-1.,3.20454818630635));
#61342=CARTESIAN_POINT('Ctrl Pts',(-2.08182850370816,1.,3.20454818630635));
#61343=CARTESIAN_POINT('Ctrl Pts',(-2.0769044187063,-1.,3.19934132835879));
#61344=CARTESIAN_POINT('Ctrl Pts',(-2.0769044187063,1.,3.19934132835879));
#61345=CARTESIAN_POINT('Ctrl Pts',(-2.07192253497765,-1.,3.19388465568113));
#61346=CARTESIAN_POINT('Ctrl Pts',(-2.07192253497765,1.,3.19388465568113));
#61347=CARTESIAN_POINT('Ctrl Pts',(-2.06684062744065,-1.,3.18809755562297));
#61348=CARTESIAN_POINT('Ctrl Pts',(-2.06684062744065,1.,3.18809755562297));
#61349=CARTESIAN_POINT('Ctrl Pts',(-2.06166849827143,-1.,3.18197692964677));
#61350=CARTESIAN_POINT('Ctrl Pts',(-2.06166849827143,1.,3.18197692964677));
#61351=CARTESIAN_POINT('Ctrl Pts',(-2.05650186773279,-1.,3.17564906975592));
#61352=CARTESIAN_POINT('Ctrl Pts',(-2.05650186773279,1.,3.17564906975592));
#61353=CARTESIAN_POINT('Ctrl Pts',(-2.05151770247452,-1.,3.16936341689859));
#61354=CARTESIAN_POINT('Ctrl Pts',(-2.05151770247452,1.,3.16936341689859));
#61355=CARTESIAN_POINT('Ctrl Pts',(-2.0469333124766,-1.,3.16343165059235));
#61356=CARTESIAN_POINT('Ctrl Pts',(-2.0469333124766,1.,3.16343165059235));
#61357=CARTESIAN_POINT('Ctrl Pts',(-2.04297406404132,-1.,3.15817983946525));
#61358=CARTESIAN_POINT('Ctrl Pts',(-2.04297406404132,1.,3.15817983946525));
#61359=CARTESIAN_POINT('Ctrl Pts',(-2.03984073791432,-1.,3.1538999167466));
#61360=CARTESIAN_POINT('Ctrl Pts',(-2.03984073791432,1.,3.1538999167466));
#61361=CARTESIAN_POINT('Ctrl Pts',(-2.03766932526171,-1.,3.15079010635326));
#61362=CARTESIAN_POINT('Ctrl Pts',(-2.03766932526171,1.,3.15079010635326));
#61363=CARTESIAN_POINT('Ctrl Pts',(-2.03675273048882,-1.,3.14931281967585));
#61364=CARTESIAN_POINT('Ctrl Pts',(-2.03675273048882,1.,3.14931281967585));
#61365=CARTESIAN_POINT('Ctrl Pts',(-2.03653654935384,-1.,3.14878756590499));
#61366=CARTESIAN_POINT('Ctrl Pts',(-2.03653654935384,1.,3.14878756590499));
#61367=CARTESIAN_POINT('Ctrl Pts',(-2.036601737578,-1.,3.14869618937138));
#61368=CARTESIAN_POINT('Ctrl Pts',(-2.036601737578,1.,3.14869618937138));
#61369=CARTESIAN_POINT('Ctrl Pts',(-2.03668666247593,-1.,3.1487152044751));
#61370=CARTESIAN_POINT('Ctrl Pts',(-2.03668666247593,1.,3.1487152044751));
#61371=CARTESIAN_POINT('',(-2.40675750623143,1.,3.44202241512147));
#61372=CARTESIAN_POINT('Ctrl Pts',(-2.40675750623143,1.,3.44202241512147));
#61373=CARTESIAN_POINT('Ctrl Pts',(-2.40537592959345,1.,3.44127120683402));
#61374=CARTESIAN_POINT('Ctrl Pts',(-2.40261515590099,1.,3.43976627485223));
#61375=CARTESIAN_POINT('Ctrl Pts',(-2.39848113411429,1.,3.43750133066036));
#61376=CARTESIAN_POINT('Ctrl Pts',(-2.39298338805823,1.,3.43446630680436));
#61377=CARTESIAN_POINT('Ctrl Pts',(-2.38613505844641,1.,3.43064732714472));
#61378=CARTESIAN_POINT('Ctrl Pts',(-2.37931067029517,1.,3.42680309755241));
#61379=CARTESIAN_POINT('Ctrl Pts',(-2.37251035954351,1.,3.42293356216595));
#61380=CARTESIAN_POINT('Ctrl Pts',(-2.36573431470314,1.,3.41903866635384));
#61381=CARTESIAN_POINT('Ctrl Pts',(-2.35898278606449,1.,3.4151183675076));
#61382=CARTESIAN_POINT('Ctrl Pts',(-2.35225606823649,1.,3.41117262313464));
#61383=CARTESIAN_POINT('Ctrl Pts',(-2.34555447648901,1.,3.40720137403888));
#61384=CARTESIAN_POINT('Ctrl Pts',(-2.33887832342715,1.,3.40320452776646));
#61385=CARTESIAN_POINT('Ctrl Pts',(-2.33222789882601,1.,3.39918194578115));
#61386=CARTESIAN_POINT('Ctrl Pts',(-2.32560343902683,1.,3.39513342020045));
#61387=CARTESIAN_POINT('Ctrl Pts',(-2.31900513925627,1.,3.39105869475112));
#61388=CARTESIAN_POINT('Ctrl Pts',(-2.31243319489505,1.,3.38695751492659));
#61389=CARTESIAN_POINT('Ctrl Pts',(-2.30588783640389,1.,3.38282967336676));
#61390=CARTESIAN_POINT('Ctrl Pts',(-2.29936936127588,1.,3.37867504959382));
#61391=CARTESIAN_POINT('Ctrl Pts',(-2.2928781800731,1.,3.37449367172707));
#61392=CARTESIAN_POINT('Ctrl Pts',(-2.28641481081045,1.,3.37028570206357));
#61393=CARTESIAN_POINT('Ctrl Pts',(-2.27997979457968,1.,3.36605130712978));
#61394=CARTESIAN_POINT('Ctrl Pts',(-2.27357362620902,1.,3.36179055004369));
#61395=CARTESIAN_POINT('Ctrl Pts',(-2.26719668579921,1.,3.35750328523077));
#61396=CARTESIAN_POINT('Ctrl Pts',(-2.26084915222484,1.,3.35318902552676));
#61397=CARTESIAN_POINT('Ctrl Pts',(-2.25453097693524,1.,3.34884690292342));
#61398=CARTESIAN_POINT('Ctrl Pts',(-2.24824207678288,1.,3.34447596770768));
#61399=CARTESIAN_POINT('Ctrl Pts',(-2.24198249391437,1.,3.34007543738044));
#61400=CARTESIAN_POINT('Ctrl Pts',(-2.2357525632881,1.,3.33564495756478));
#61401=CARTESIAN_POINT('Ctrl Pts',(-2.22955308907221,1.,3.33118487773593));
#61402=CARTESIAN_POINT('Ctrl Pts',(-2.22338548312758,1.,3.32669646722871));
#61403=CARTESIAN_POINT('Ctrl Pts',(-2.21725135110889,1.,3.32218125618955));
#61404=CARTESIAN_POINT('Ctrl Pts',(-2.21115211847872,1.,3.31764044024231));
#61405=CARTESIAN_POINT('Ctrl Pts',(-2.20508863150608,1.,3.3130742460895));
#61406=CARTESIAN_POINT('Ctrl Pts',(-2.19906078949924,1.,3.30848134694596));
#61407=CARTESIAN_POINT('Ctrl Pts',(-2.19306710376112,1.,3.30385816281831));
#61408=CARTESIAN_POINT('Ctrl Pts',(-2.18710556500325,1.,3.29920022557635));
#61409=CARTESIAN_POINT('Ctrl Pts',(-2.18117455557062,1.,3.29450361500484));
#61410=CARTESIAN_POINT('Ctrl Pts',(-2.17527380048422,1.,3.28976645712566));
#61411=CARTESIAN_POINT('Ctrl Pts',(-2.16940517773459,1.,3.2849901997973));
#61412=CARTESIAN_POINT('Ctrl Pts',(-2.16357391934434,1.,3.28018150841414));
#61413=CARTESIAN_POINT('Ctrl Pts',(-2.15778690038359,1.,3.27534954469206));
#61414=CARTESIAN_POINT('Ctrl Pts',(-2.15205043199818,1.,3.27050245897244));
#61415=CARTESIAN_POINT('Ctrl Pts',(-2.14636805295663,1.,3.26564388189764));
#61416=CARTESIAN_POINT('Ctrl Pts',(-2.14073870754257,1.,3.26077002641868));
#61417=CARTESIAN_POINT('Ctrl Pts',(-2.13515375878786,1.,3.25586495065027));
#61418=CARTESIAN_POINT('Ctrl Pts',(-2.1296002839681,1.,3.25090574493994));
#61419=CARTESIAN_POINT('Ctrl Pts',(-2.12406646410943,1.,3.24587102613347));
#61420=CARTESIAN_POINT('Ctrl Pts',(-2.11854673326972,1.,3.24074905517282));
#61421=CARTESIAN_POINT('Ctrl Pts',(-2.11304604021784,1.,3.23554444767115));
#61422=CARTESIAN_POINT('Ctrl Pts',(-2.1075869964248,1.,3.23028945793334));
#61423=CARTESIAN_POINT('Ctrl Pts',(-2.10220384298533,1.,3.22503437553496));
#61424=CARTESIAN_POINT('Ctrl Pts',(-2.09692958434933,1.,3.21982707347067));
#61425=CARTESIAN_POINT('Ctrl Pts',(-2.0917841946046,1.,3.2146942960168));
#61426=CARTESIAN_POINT('Ctrl Pts',(-2.08676465517435,1.,3.20962575845433));
#61427=CARTESIAN_POINT('Ctrl Pts',(-2.08182850370816,1.,3.20454818630635));
#61428=CARTESIAN_POINT('Ctrl Pts',(-2.0769044187063,1.,3.19934132835879));
#61429=CARTESIAN_POINT('Ctrl Pts',(-2.07192253497765,1.,3.19388465568113));
#61430=CARTESIAN_POINT('Ctrl Pts',(-2.06684062744065,1.,3.18809755562297));
#61431=CARTESIAN_POINT('Ctrl Pts',(-2.06166849827143,1.,3.18197692964677));
#61432=CARTESIAN_POINT('Ctrl Pts',(-2.05650186773279,1.,3.17564906975592));
#61433=CARTESIAN_POINT('Ctrl Pts',(-2.05151770247452,1.,3.16936341689859));
#61434=CARTESIAN_POINT('Ctrl Pts',(-2.0469333124766,1.,3.16343165059235));
#61435=CARTESIAN_POINT('Ctrl Pts',(-2.04297406404132,1.,3.15817983946525));
#61436=CARTESIAN_POINT('Ctrl Pts',(-2.03984073791432,1.,3.1538999167466));
#61437=CARTESIAN_POINT('Ctrl Pts',(-2.03783225496023,1.,3.15102344775396));
#61438=CARTESIAN_POINT('Ctrl Pts',(-2.03693188810614,1.,3.14959882629936));
#61439=CARTESIAN_POINT('Ctrl Pts',(-2.03663974554941,1.,3.14901193669147));
#61440=CARTESIAN_POINT('Ctrl Pts',(-2.03659701539175,1.,3.1488193908823));
#61441=CARTESIAN_POINT('Ctrl Pts',(-2.03660101169564,1.,3.14877060440425));
#61442=CARTESIAN_POINT('',(-2.40675750623143,0.,3.44202241512147));
#61443=CARTESIAN_POINT('Ctrl Pts',(-2.36523532225181,-1.,2.91001063062876));
#61444=CARTESIAN_POINT('Ctrl Pts',(-2.36523532225181,1.,2.91001063062876));
#61445=CARTESIAN_POINT('Ctrl Pts',(-2.36524348105112,-1.,2.90992398626211));
#61446=CARTESIAN_POINT('Ctrl Pts',(-2.36524348105112,1.,2.90992398626211));
#61447=CARTESIAN_POINT('Ctrl Pts',(-2.36535052956938,-1.,2.90989022548032));
#61448=CARTESIAN_POINT('Ctrl Pts',(-2.36535052956938,1.,2.90989022548032));
#61449=CARTESIAN_POINT('Ctrl Pts',(-2.36578327194741,-1.,2.91025813830041));
#61450=CARTESIAN_POINT('Ctrl Pts',(-2.36578327194741,1.,2.91025813830041));
#61451=CARTESIAN_POINT('Ctrl Pts',(-2.36690501170627,-1.,2.9115863784204));
#61452=CARTESIAN_POINT('Ctrl Pts',(-2.36690501170627,1.,2.9115863784204));
#61453=CARTESIAN_POINT('Ctrl Pts',(-2.36919161373173,-1.,2.9146124988314));
#61454=CARTESIAN_POINT('Ctrl Pts',(-2.36919161373173,1.,2.9146124988314));
#61455=CARTESIAN_POINT('Ctrl Pts',(-2.37229381109821,-1.,2.91891503791411));
#61456=CARTESIAN_POINT('Ctrl Pts',(-2.37229381109821,1.,2.91891503791411));
#61457=CARTESIAN_POINT('Ctrl Pts',(-2.3760651052403,-1.,2.92430340582608));
#61458=CARTESIAN_POINT('Ctrl Pts',(-2.3760651052403,1.,2.92430340582608));
#61459=CARTESIAN_POINT('Ctrl Pts',(-2.38028989582073,-1.,2.93049643640206));
#61460=CARTESIAN_POINT('Ctrl Pts',(-2.38028989582073,1.,2.93049643640206));
#61461=CARTESIAN_POINT('Ctrl Pts',(-2.38472771516311,-1.,2.93717903280391));
#61462=CARTESIAN_POINT('Ctrl Pts',(-2.38472771516311,1.,2.93717903280391));
#61463=CARTESIAN_POINT('Ctrl Pts',(-2.38914929090759,-1.,2.94404820669076));
#61464=CARTESIAN_POINT('Ctrl Pts',(-2.38914929090759,1.,2.94404820669076));
#61465=CARTESIAN_POINT('Ctrl Pts',(-2.39337207631667,-1.,2.95085857128439));
#61466=CARTESIAN_POINT('Ctrl Pts',(-2.39337207631667,1.,2.95085857128439));
#61467=CARTESIAN_POINT('Ctrl Pts',(-2.39730553974517,-1.,2.95748006482942));
#61468=CARTESIAN_POINT('Ctrl Pts',(-2.39730553974517,1.,2.95748006482942));
#61469=CARTESIAN_POINT('Ctrl Pts',(-2.4009556571164,-1.,2.96390432240312));
#61470=CARTESIAN_POINT('Ctrl Pts',(-2.4009556571164,1.,2.96390432240312));
#61471=CARTESIAN_POINT('Ctrl Pts',(-2.40438604734919,-1.,2.9701964131236));
#61472=CARTESIAN_POINT('Ctrl Pts',(-2.40438604734919,1.,2.9701964131236));
#61473=CARTESIAN_POINT('Ctrl Pts',(-2.40768975073713,-1.,2.97646002822422));
#61474=CARTESIAN_POINT('Ctrl Pts',(-2.40768975073713,1.,2.97646002822422));
#61475=CARTESIAN_POINT('Ctrl Pts',(-2.41095909342571,-1.,2.98280015815107));
#61476=CARTESIAN_POINT('Ctrl Pts',(-2.41095909342571,1.,2.98280015815107));
#61477=CARTESIAN_POINT('Ctrl Pts',(-2.41425064199586,-1.,2.98927983005796));
#61478=CARTESIAN_POINT('Ctrl Pts',(-2.41425064199586,1.,2.98927983005796));
#61479=CARTESIAN_POINT('Ctrl Pts',(-2.41757324500514,-1.,2.99590509293503));
#61480=CARTESIAN_POINT('Ctrl Pts',(-2.41757324500514,1.,2.99590509293503));
#61481=CARTESIAN_POINT('Ctrl Pts',(-2.42090763946779,-1.,3.00264868585996));
#61482=CARTESIAN_POINT('Ctrl Pts',(-2.42090763946779,1.,3.00264868585996));
#61483=CARTESIAN_POINT('Ctrl Pts',(-2.42421849439613,-1.,3.00946442616658));
#61484=CARTESIAN_POINT('Ctrl Pts',(-2.42421849439613,1.,3.00946442616658));
#61485=CARTESIAN_POINT('Ctrl Pts',(-2.42746856264168,-1.,3.01630420830504));
#61486=CARTESIAN_POINT('Ctrl Pts',(-2.42746856264168,1.,3.01630420830504));
#61487=CARTESIAN_POINT('Ctrl Pts',(-2.43063415586637,-1.,3.02313656036004));
#61488=CARTESIAN_POINT('Ctrl Pts',(-2.43063415586637,1.,3.02313656036004));
#61489=CARTESIAN_POINT('Ctrl Pts',(-2.43371241361488,-1.,3.02995534946978));
#61490=CARTESIAN_POINT('Ctrl Pts',(-2.43371241361488,1.,3.02995534946978));
#61491=CARTESIAN_POINT('Ctrl Pts',(-2.43671278042414,-1.,3.03676949672821));
#61492=CARTESIAN_POINT('Ctrl Pts',(-2.43671278042414,1.,3.03676949672821));
#61493=CARTESIAN_POINT('Ctrl Pts',(-2.43965194061857,-1.,3.04359685040555));
#61494=CARTESIAN_POINT('Ctrl Pts',(-2.43965194061857,1.,3.04359685040555));
#61495=CARTESIAN_POINT('Ctrl Pts',(-2.44254768923105,-1.,3.05045678021504));
#61496=CARTESIAN_POINT('Ctrl Pts',(-2.44254768923105,1.,3.05045678021504));
#61497=CARTESIAN_POINT('Ctrl Pts',(-2.44541251892556,-1.,3.05736242671506));
#61498=CARTESIAN_POINT('Ctrl Pts',(-2.44541251892556,1.,3.05736242671506));
#61499=CARTESIAN_POINT('Ctrl Pts',(-2.44824970516544,-1.,3.06431596421405));
#61500=CARTESIAN_POINT('Ctrl Pts',(-2.44824970516544,1.,3.06431596421405));
#61501=CARTESIAN_POINT('Ctrl Pts',(-2.45105688854422,-1.,3.07131290521297));
#61502=CARTESIAN_POINT('Ctrl Pts',(-2.45105688854422,1.,3.07131290521297));
#61503=CARTESIAN_POINT('Ctrl Pts',(-2.4538282678779,-1.,3.07834472886139));
#61504=CARTESIAN_POINT('Ctrl Pts',(-2.4538282678779,1.,3.07834472886139));
#61505=CARTESIAN_POINT('Ctrl Pts',(-2.45655725437039,-1.,3.08540206545315));
#61506=CARTESIAN_POINT('Ctrl Pts',(-2.45655725437039,1.,3.08540206545315));
#61507=CARTESIAN_POINT('Ctrl Pts',(-2.4592391256388,-1.,3.09247787931887));
#61508=CARTESIAN_POINT('Ctrl Pts',(-2.4592391256388,1.,3.09247787931887));
#61509=CARTESIAN_POINT('Ctrl Pts',(-2.46187308501884,-1.,3.09956993697052));
#61510=CARTESIAN_POINT('Ctrl Pts',(-2.46187308501884,1.,3.09956993697052));
#61511=CARTESIAN_POINT('Ctrl Pts',(-2.46446082979646,-1.,3.1066790790198));
#61512=CARTESIAN_POINT('Ctrl Pts',(-2.46446082979646,1.,3.1066790790198));
#61513=CARTESIAN_POINT('Ctrl Pts',(-2.46700558843506,-1.,3.11380805536122));
#61514=CARTESIAN_POINT('Ctrl Pts',(-2.46700558843506,1.,3.11380805536122));
#61515=CARTESIAN_POINT('Ctrl Pts',(-2.46951098947469,-1.,3.12096015766983));
#61516=CARTESIAN_POINT('Ctrl Pts',(-2.46951098947469,1.,3.12096015766983));
#61517=CARTESIAN_POINT('Ctrl Pts',(-2.47197997765871,-1.,3.12813790805952));
#61518=CARTESIAN_POINT('Ctrl Pts',(-2.47197997765871,1.,3.12813790805952));
#61519=CARTESIAN_POINT('Ctrl Pts',(-2.47441378371932,-1.,3.13534181229295));
#61520=CARTESIAN_POINT('Ctrl Pts',(-2.47441378371932,1.,3.13534181229295));
#61521=CARTESIAN_POINT('Ctrl Pts',(-2.47681245356109,-1.,3.1425709954655));
#61522=CARTESIAN_POINT('Ctrl Pts',(-2.47681245356109,1.,3.1425709954655));
#61523=CARTESIAN_POINT('Ctrl Pts',(-2.47917529057029,-1.,3.14982373241352));
#61524=CARTESIAN_POINT('Ctrl Pts',(-2.47917529057029,1.,3.14982373241352));
#61525=CARTESIAN_POINT('Ctrl Pts',(-2.48150133566571,-1.,3.15709802322739));
#61526=CARTESIAN_POINT('Ctrl Pts',(-2.48150133566571,1.,3.15709802322739));
#61527=CARTESIAN_POINT('Ctrl Pts',(-2.48378981792725,-1.,3.16439213290161));
#61528=CARTESIAN_POINT('Ctrl Pts',(-2.48378981792725,1.,3.16439213290161));
#61529=CARTESIAN_POINT('Ctrl Pts',(-2.48604065348587,-1.,3.17170518863313));
#61530=CARTESIAN_POINT('Ctrl Pts',(-2.48604065348587,1.,3.17170518863313));
#61531=CARTESIAN_POINT('Ctrl Pts',(-2.48825428288201,-1.,3.17903698136622));
#61532=CARTESIAN_POINT('Ctrl Pts',(-2.48825428288201,1.,3.17903698136622));
#61533=CARTESIAN_POINT('Ctrl Pts',(-2.49043146334059,-1.,3.18638771282266));
#61534=CARTESIAN_POINT('Ctrl Pts',(-2.49043146334059,1.,3.18638771282266));
#61535=CARTESIAN_POINT('Ctrl Pts',(-2.49257307239848,-1.,3.19375775555798));
#61536=CARTESIAN_POINT('Ctrl Pts',(-2.49257307239848,1.,3.19375775555798));
#61537=CARTESIAN_POINT('Ctrl Pts',(-2.49467992057755,-1.,3.20114742397588));
#61538=CARTESIAN_POINT('Ctrl Pts',(-2.49467992057755,1.,3.20114742397588));
#61539=CARTESIAN_POINT('Ctrl Pts',(-2.4967525264737,-1.,3.20855669849836));
#61540=CARTESIAN_POINT('Ctrl Pts',(-2.4967525264737,1.,3.20855669849836));
#61541=CARTESIAN_POINT('Ctrl Pts',(-2.4987911459939,-1.,3.21598526261286));
#61542=CARTESIAN_POINT('Ctrl Pts',(-2.4987911459939,1.,3.21598526261286));
#61543=CARTESIAN_POINT('Ctrl Pts',(-2.50079587201957,-1.,3.22343262620503));
#61544=CARTESIAN_POINT('Ctrl Pts',(-2.50079587201957,1.,3.22343262620503));
#61545=CARTESIAN_POINT('Ctrl Pts',(-2.50276671338111,-1.,3.23089822320646));
#61546=CARTESIAN_POINT('Ctrl Pts',(-2.50276671338111,1.,3.23089822320646));
#61547=CARTESIAN_POINT('Ctrl Pts',(-2.5047036758003,-1.,3.23838151080319));
#61548=CARTESIAN_POINT('Ctrl Pts',(-2.5047036758003,1.,3.23838151080319));
#61549=CARTESIAN_POINT('Ctrl Pts',(-2.506606859405,-1.,3.24588208983849));
#61550=CARTESIAN_POINT('Ctrl Pts',(-2.506606859405,1.,3.24588208983849));
#61551=CARTESIAN_POINT('Ctrl Pts',(-2.50847647070723,-1.,3.25339971460982));
#61552=CARTESIAN_POINT('Ctrl Pts',(-2.50847647070723,1.,3.25339971460982));
#61553=CARTESIAN_POINT('Ctrl Pts',(-2.51031277813486,-1.,3.26093423001434));
#61554=CARTESIAN_POINT('Ctrl Pts',(-2.51031277813486,1.,3.26093423001434));
#61555=CARTESIAN_POINT('Ctrl Pts',(-2.51211608411423,-1.,3.26848552888115));
#61556=CARTESIAN_POINT('Ctrl Pts',(-2.51211608411423,1.,3.26848552888115));
#61557=CARTESIAN_POINT('Ctrl Pts',(-2.513886692704,-1.,3.27605350473142));
#61558=CARTESIAN_POINT('Ctrl Pts',(-2.513886692704,1.,3.27605350473142));
#61559=CARTESIAN_POINT('Ctrl Pts',(-2.51562487464514,-1.,3.28363799702982));
#61560=CARTESIAN_POINT('Ctrl Pts',(-2.51562487464514,1.,3.28363799702982));
#61561=CARTESIAN_POINT('Ctrl Pts',(-2.51733085123797,-1.,3.2912387729927));
#61562=CARTESIAN_POINT('Ctrl Pts',(-2.51733085123797,1.,3.2912387729927));
#61563=CARTESIAN_POINT('Ctrl Pts',(-2.51900480701069,-1.,3.29885556388352));
#61564=CARTESIAN_POINT('Ctrl Pts',(-2.51900480701069,1.,3.29885556388352));
#61565=CARTESIAN_POINT('Ctrl Pts',(-2.52064689568511,-1.,3.30648808815442));
#61566=CARTESIAN_POINT('Ctrl Pts',(-2.52064689568511,1.,3.30648808815442));
#61567=CARTESIAN_POINT('Ctrl Pts',(-2.52225724871313,-1.,3.31413607874645));
#61568=CARTESIAN_POINT('Ctrl Pts',(-2.52225724871313,1.,3.31413607874645));
#61569=CARTESIAN_POINT('Ctrl Pts',(-2.5238359839626,-1.,3.32179931078699));
#61570=CARTESIAN_POINT('Ctrl Pts',(-2.5238359839626,1.,3.32179931078699));
#61571=CARTESIAN_POINT('Ctrl Pts',(-2.52538321164634,-1.,3.32947762187533));
#61572=CARTESIAN_POINT('Ctrl Pts',(-2.52538321164634,1.,3.32947762187533));
#61573=CARTESIAN_POINT('Ctrl Pts',(-2.52689902690158,-1.,3.33717089999103));
#61574=CARTESIAN_POINT('Ctrl Pts',(-2.52689902690158,1.,3.33717089999103));
#61575=CARTESIAN_POINT('Ctrl Pts',(-2.52808660915689,-1.,3.34333744115511));
#61576=CARTESIAN_POINT('Ctrl Pts',(-2.52808660915689,1.,3.34333744115511));
#61577=CARTESIAN_POINT('Ctrl Pts',(-2.52896321610703,-1.,3.34796903576663));
#61578=CARTESIAN_POINT('Ctrl Pts',(-2.52896321610703,1.,3.34796903576663));
#61579=CARTESIAN_POINT('Ctrl Pts',(-2.5295413654909,-1.,3.35105973714071));
#61580=CARTESIAN_POINT('Ctrl Pts',(-2.5295413654909,1.,3.35105973714071));
#61581=CARTESIAN_POINT('Ctrl Pts',(-2.52982887637028,-1.,3.35260583073571));
#61582=CARTESIAN_POINT('Ctrl Pts',(-2.52982887637028,1.,3.35260583073571));
#61583=CARTESIAN_POINT('',(-2.36531447826073,1.,2.90994629141676));
#61584=CARTESIAN_POINT('Ctrl Pts',(-2.36531447826073,-1.,2.90994629141676));
#61585=CARTESIAN_POINT('Ctrl Pts',(-2.36531447826073,-0.666666666666667,
2.90994629141676));
#61586=CARTESIAN_POINT('Ctrl Pts',(-2.36531447826073,-0.333333333333333,
2.90994629141676));
#61587=CARTESIAN_POINT('Ctrl Pts',(-2.36531447826073,0.333333333333333,
2.90994629141676));
#61588=CARTESIAN_POINT('Ctrl Pts',(-2.36531447826073,0.666666666666667,
2.90994629141676));
#61589=CARTESIAN_POINT('Ctrl Pts',(-2.36531447826073,1.,2.90994629141676));
#61590=CARTESIAN_POINT('',(-2.52982887637028,1.,3.35260583073571));
#61591=CARTESIAN_POINT('',(-2.52982887637028,0.,3.35260583073571));
#61592=CARTESIAN_POINT('Ctrl Pts',(-2.36531447826073,1.,2.90994629141676));
#61593=CARTESIAN_POINT('Ctrl Pts',(-2.36536211188453,1.,2.90995756655606));
#61594=CARTESIAN_POINT('Ctrl Pts',(-2.36553202948613,1.,2.91005770527719));
#61595=CARTESIAN_POINT('Ctrl Pts',(-2.36599991765749,1.,2.91051690822156));
#61596=CARTESIAN_POINT('Ctrl Pts',(-2.36707658451664,1.,2.91181344022549));
#61597=CARTESIAN_POINT('Ctrl Pts',(-2.36919161373173,1.,2.9146124988314));
#61598=CARTESIAN_POINT('Ctrl Pts',(-2.37229381109821,1.,2.91891503791411));
#61599=CARTESIAN_POINT('Ctrl Pts',(-2.3760651052403,1.,2.92430340582608));
#61600=CARTESIAN_POINT('Ctrl Pts',(-2.38028989582073,1.,2.93049643640206));
#61601=CARTESIAN_POINT('Ctrl Pts',(-2.38472771516311,1.,2.93717903280391));
#61602=CARTESIAN_POINT('Ctrl Pts',(-2.38914929090759,1.,2.94404820669076));
#61603=CARTESIAN_POINT('Ctrl Pts',(-2.39337207631667,1.,2.95085857128439));
#61604=CARTESIAN_POINT('Ctrl Pts',(-2.39730553974517,1.,2.95748006482942));
#61605=CARTESIAN_POINT('Ctrl Pts',(-2.4009556571164,1.,2.96390432240312));
#61606=CARTESIAN_POINT('Ctrl Pts',(-2.40438604734919,1.,2.9701964131236));
#61607=CARTESIAN_POINT('Ctrl Pts',(-2.40768975073713,1.,2.97646002822422));
#61608=CARTESIAN_POINT('Ctrl Pts',(-2.41095909342571,1.,2.98280015815107));
#61609=CARTESIAN_POINT('Ctrl Pts',(-2.41425064199586,1.,2.98927983005796));
#61610=CARTESIAN_POINT('Ctrl Pts',(-2.41757324500514,1.,2.99590509293503));
#61611=CARTESIAN_POINT('Ctrl Pts',(-2.42090763946779,1.,3.00264868585996));
#61612=CARTESIAN_POINT('Ctrl Pts',(-2.42421849439613,1.,3.00946442616658));
#61613=CARTESIAN_POINT('Ctrl Pts',(-2.42746856264168,1.,3.01630420830504));
#61614=CARTESIAN_POINT('Ctrl Pts',(-2.43063415586637,1.,3.02313656036004));
#61615=CARTESIAN_POINT('Ctrl Pts',(-2.43371241361488,1.,3.02995534946978));
#61616=CARTESIAN_POINT('Ctrl Pts',(-2.43671278042414,1.,3.03676949672821));
#61617=CARTESIAN_POINT('Ctrl Pts',(-2.43965194061857,1.,3.04359685040555));
#61618=CARTESIAN_POINT('Ctrl Pts',(-2.44254768923105,1.,3.05045678021504));
#61619=CARTESIAN_POINT('Ctrl Pts',(-2.44541251892556,1.,3.05736242671506));
#61620=CARTESIAN_POINT('Ctrl Pts',(-2.44824970516544,1.,3.06431596421405));
#61621=CARTESIAN_POINT('Ctrl Pts',(-2.45105688854422,1.,3.07131290521297));
#61622=CARTESIAN_POINT('Ctrl Pts',(-2.4538282678779,1.,3.07834472886139));
#61623=CARTESIAN_POINT('Ctrl Pts',(-2.45655725437039,1.,3.08540206545315));
#61624=CARTESIAN_POINT('Ctrl Pts',(-2.4592391256388,1.,3.09247787931887));
#61625=CARTESIAN_POINT('Ctrl Pts',(-2.46187308501884,1.,3.09956993697052));
#61626=CARTESIAN_POINT('Ctrl Pts',(-2.46446082979646,1.,3.1066790790198));
#61627=CARTESIAN_POINT('Ctrl Pts',(-2.46700558843506,1.,3.11380805536122));
#61628=CARTESIAN_POINT('Ctrl Pts',(-2.46951098947469,1.,3.12096015766983));
#61629=CARTESIAN_POINT('Ctrl Pts',(-2.47197997765871,1.,3.12813790805952));
#61630=CARTESIAN_POINT('Ctrl Pts',(-2.47441378371932,1.,3.13534181229295));
#61631=CARTESIAN_POINT('Ctrl Pts',(-2.47681245356109,1.,3.1425709954655));
#61632=CARTESIAN_POINT('Ctrl Pts',(-2.47917529057029,1.,3.14982373241352));
#61633=CARTESIAN_POINT('Ctrl Pts',(-2.48150133566571,1.,3.15709802322739));
#61634=CARTESIAN_POINT('Ctrl Pts',(-2.48378981792725,1.,3.16439213290161));
#61635=CARTESIAN_POINT('Ctrl Pts',(-2.48604065348587,1.,3.17170518863313));
#61636=CARTESIAN_POINT('Ctrl Pts',(-2.48825428288201,1.,3.17903698136622));
#61637=CARTESIAN_POINT('Ctrl Pts',(-2.49043146334059,1.,3.18638771282266));
#61638=CARTESIAN_POINT('Ctrl Pts',(-2.49257307239848,1.,3.19375775555798));
#61639=CARTESIAN_POINT('Ctrl Pts',(-2.49467992057755,1.,3.20114742397588));
#61640=CARTESIAN_POINT('Ctrl Pts',(-2.4967525264737,1.,3.20855669849836));
#61641=CARTESIAN_POINT('Ctrl Pts',(-2.4987911459939,1.,3.21598526261286));
#61642=CARTESIAN_POINT('Ctrl Pts',(-2.50079587201957,1.,3.22343262620503));
#61643=CARTESIAN_POINT('Ctrl Pts',(-2.50276671338111,1.,3.23089822320646));
#61644=CARTESIAN_POINT('Ctrl Pts',(-2.5047036758003,1.,3.23838151080319));
#61645=CARTESIAN_POINT('Ctrl Pts',(-2.506606859405,1.,3.24588208983849));
#61646=CARTESIAN_POINT('Ctrl Pts',(-2.50847647070723,1.,3.25339971460982));
#61647=CARTESIAN_POINT('Ctrl Pts',(-2.51031277813486,1.,3.26093423001434));
#61648=CARTESIAN_POINT('Ctrl Pts',(-2.51211608411423,1.,3.26848552888115));
#61649=CARTESIAN_POINT('Ctrl Pts',(-2.513886692704,1.,3.27605350473142));
#61650=CARTESIAN_POINT('Ctrl Pts',(-2.51562487464514,1.,3.28363799702982));
#61651=CARTESIAN_POINT('Ctrl Pts',(-2.51733085123797,1.,3.2912387729927));
#61652=CARTESIAN_POINT('Ctrl Pts',(-2.51900480701069,1.,3.29885556388352));
#61653=CARTESIAN_POINT('Ctrl Pts',(-2.52064689568511,1.,3.30648808815442));
#61654=CARTESIAN_POINT('Ctrl Pts',(-2.52225724871313,1.,3.31413607874645));
#61655=CARTESIAN_POINT('Ctrl Pts',(-2.5238359839626,1.,3.32179931078699));
#61656=CARTESIAN_POINT('Ctrl Pts',(-2.52538321164634,1.,3.32947762187533));
#61657=CARTESIAN_POINT('Ctrl Pts',(-2.52689902690158,1.,3.33717089999103));
#61658=CARTESIAN_POINT('Ctrl Pts',(-2.52808660915689,1.,3.34333744115511));
#61659=CARTESIAN_POINT('Ctrl Pts',(-2.52896321610703,1.,3.34796903576663));
#61660=CARTESIAN_POINT('Ctrl Pts',(-2.5295413654909,1.,3.35105973714071));
#61661=CARTESIAN_POINT('Ctrl Pts',(-2.52982887637028,1.,3.35260583073571));
#61662=CARTESIAN_POINT('Origin',(-2.52982887637028,0.,3.35260583073571));
#61663=CARTESIAN_POINT('',(-2.40675750623143,1.,3.44202241512147));
#61664=CARTESIAN_POINT('Origin',(0.,0.,0.));
#61665=CARTESIAN_POINT('',(-2.50410331873042,1.,2.79140942341378));
#61666=CARTESIAN_POINT('Origin',(0.,1.,0.));
#61667=CARTESIAN_POINT('Ctrl Pts',(-2.50410331873042,1.,2.79140942341378));
#61668=CARTESIAN_POINT('Ctrl Pts',(-2.50410331873042,0.666666666666667,
2.79140942341378));
#61669=CARTESIAN_POINT('Ctrl Pts',(-2.50410331873043,0.333333333333333,
2.79140942341378));
#61670=CARTESIAN_POINT('Ctrl Pts',(-2.50410331873043,-0.333333333333333,
2.79140942341378));
#61671=CARTESIAN_POINT('Ctrl Pts',(-2.50410331873043,-0.666666666666667,
2.79140942341378));
#61672=CARTESIAN_POINT('Ctrl Pts',(-2.50410331873043,-1.,2.79140942341378));
#61673=CARTESIAN_POINT('Ctrl Pts',(-2.91557726271063,-1.,3.02314558451372));
#61674=CARTESIAN_POINT('Ctrl Pts',(-2.91557726271063,1.,3.02314558451372));
#61675=CARTESIAN_POINT('Ctrl Pts',(-2.91409518070707,-1.,3.02261975104912));
#61676=CARTESIAN_POINT('Ctrl Pts',(-2.91409518070707,1.,3.02261975104912));
#61677=CARTESIAN_POINT('Ctrl Pts',(-2.91113297349052,-1.,3.02156522743299));
#61678=CARTESIAN_POINT('Ctrl Pts',(-2.91113297349052,1.,3.02156522743299));
#61679=CARTESIAN_POINT('Ctrl Pts',(-2.90669553303902,-1.,3.01997487194926));
#61680=CARTESIAN_POINT('Ctrl Pts',(-2.90669553303902,1.,3.01997487194926));
#61681=CARTESIAN_POINT('Ctrl Pts',(-2.90079069102661,-1.,3.01783725123646));
#61682=CARTESIAN_POINT('Ctrl Pts',(-2.90079069102661,1.,3.01783725123646));
#61683=CARTESIAN_POINT('Ctrl Pts',(-2.8934292556764,-1.,3.01513660433291));
#61684=CARTESIAN_POINT('Ctrl Pts',(-2.8934292556764,1.,3.01513660433291));
#61685=CARTESIAN_POINT('Ctrl Pts',(-2.88608751706796,-1.,3.01240727309568));
#61686=CARTESIAN_POINT('Ctrl Pts',(-2.88608751706796,1.,3.01240727309568));
#61687=CARTESIAN_POINT('Ctrl Pts',(-2.87876560072799,-1.,3.0096491810855));
#61688=CARTESIAN_POINT('Ctrl Pts',(-2.87876560072799,1.,3.0096491810855));
#61689=CARTESIAN_POINT('Ctrl Pts',(-2.87146368430104,-1.,3.00686224485374));
#61690=CARTESIAN_POINT('Ctrl Pts',(-2.87146368430104,1.,3.00686224485374));
#61691=CARTESIAN_POINT('Ctrl Pts',(-2.86418200833065,-1.,3.00404638316245));
#61692=CARTESIAN_POINT('Ctrl Pts',(-2.86418200833065,1.,3.00404638316245));
#61693=CARTESIAN_POINT('Ctrl Pts',(-2.85692085715129,-1.,3.0012015079552));
#61694=CARTESIAN_POINT('Ctrl Pts',(-2.85692085715129,1.,3.0012015079552));
#61695=CARTESIAN_POINT('Ctrl Pts',(-2.84968053289104,-1.,2.99832751144566));
#61696=CARTESIAN_POINT('Ctrl Pts',(-2.84968053289104,1.,2.99832751144566));
#61697=CARTESIAN_POINT('Ctrl Pts',(-2.84246132984334,-1.,2.995424253416));
#61698=CARTESIAN_POINT('Ctrl Pts',(-2.84246132984334,1.,2.995424253416));
#61699=CARTESIAN_POINT('Ctrl Pts',(-2.83526351254383,-1.,2.99249155170479));
#61700=CARTESIAN_POINT('Ctrl Pts',(-2.83526351254383,1.,2.99249155170479));
#61701=CARTESIAN_POINT('Ctrl Pts',(-2.82808728190402,-1.,2.98952916401699));
#61702=CARTESIAN_POINT('Ctrl Pts',(-2.82808728190402,1.,2.98952916401699));
#61703=CARTESIAN_POINT('Ctrl Pts',(-2.82093279065704,-1.,2.98653680669434));
#61704=CARTESIAN_POINT('Ctrl Pts',(-2.82093279065704,1.,2.98653680669434));
#61705=CARTESIAN_POINT('Ctrl Pts',(-2.81380019196454,-1.,2.9835141977994));
#61706=CARTESIAN_POINT('Ctrl Pts',(-2.81380019196454,1.,2.9835141977994));
#61707=CARTESIAN_POINT('Ctrl Pts',(-2.80668968101162,-1.,2.98046109647299));
#61708=CARTESIAN_POINT('Ctrl Pts',(-2.80668968101162,1.,2.98046109647299));
#61709=CARTESIAN_POINT('Ctrl Pts',(-2.79960153278186,-1.,2.97737733718242));
#61710=CARTESIAN_POINT('Ctrl Pts',(-2.79960153278186,1.,2.97737733718242));
#61711=CARTESIAN_POINT('Ctrl Pts',(-2.79253615718147,-1.,2.97426288347475));
#61712=CARTESIAN_POINT('Ctrl Pts',(-2.79253615718147,1.,2.97426288347475));
#61713=CARTESIAN_POINT('Ctrl Pts',(-2.78549409123657,-1.,2.97111781461349));
#61714=CARTESIAN_POINT('Ctrl Pts',(-2.78549409123657,1.,2.97111781461349));
#61715=CARTESIAN_POINT('Ctrl Pts',(-2.77847589542767,-1.,2.9679422104295));
#61716=CARTESIAN_POINT('Ctrl Pts',(-2.77847589542767,1.,2.9679422104295));
#61717=CARTESIAN_POINT('Ctrl Pts',(-2.77148206836464,-1.,2.96473605585548));
#61718=CARTESIAN_POINT('Ctrl Pts',(-2.77148206836464,1.,2.96473605585548));
#61719=CARTESIAN_POINT('Ctrl Pts',(-2.76451296269571,-1.,2.96149914764832));
#61720=CARTESIAN_POINT('Ctrl Pts',(-2.76451296269571,1.,2.96149914764832));
#61721=CARTESIAN_POINT('Ctrl Pts',(-2.75756867888393,-1.,2.9582309766594));
#61722=CARTESIAN_POINT('Ctrl Pts',(-2.75756867888393,1.,2.9582309766594));
#61723=CARTESIAN_POINT('Ctrl Pts',(-2.75064903318996,-1.,2.95493069316211));
#61724=CARTESIAN_POINT('Ctrl Pts',(-2.75064903318996,1.,2.95493069316211));
#61725=CARTESIAN_POINT('Ctrl Pts',(-2.7437537949221,-1.,2.95159737214305));
#61726=CARTESIAN_POINT('Ctrl Pts',(-2.7437537949221,1.,2.95159737214305));
#61727=CARTESIAN_POINT('Ctrl Pts',(-2.73688288329825,-1.,2.94823023414381));
#61728=CARTESIAN_POINT('Ctrl Pts',(-2.73688288329825,1.,2.94823023414381));
#61729=CARTESIAN_POINT('Ctrl Pts',(-2.73003657371613,-1.,2.94482887675139));
#61730=CARTESIAN_POINT('Ctrl Pts',(-2.73003657371613,1.,2.94482887675139));
#61731=CARTESIAN_POINT('Ctrl Pts',(-2.72321571511322,-1.,2.94139351933882));
#61732=CARTESIAN_POINT('Ctrl Pts',(-2.72321571511322,1.,2.94139351933882));
#61733=CARTESIAN_POINT('Ctrl Pts',(-2.71642190053575,-1.,2.93792519474955));
#61734=CARTESIAN_POINT('Ctrl Pts',(-2.71642190053575,1.,2.93792519474955));
#61735=CARTESIAN_POINT('Ctrl Pts',(-2.70965695523776,-1.,2.93442516311168));
#61736=CARTESIAN_POINT('Ctrl Pts',(-2.70965695523776,1.,2.93442516311168));
#61737=CARTESIAN_POINT('Ctrl Pts',(-2.70292247416881,-1.,2.93089438233746));
#61738=CARTESIAN_POINT('Ctrl Pts',(-2.70292247416881,1.,2.93089438233746));
#61739=CARTESIAN_POINT('Ctrl Pts',(-2.69621932864302,-1.,2.92733294395268));
#61740=CARTESIAN_POINT('Ctrl Pts',(-2.69621932864302,1.,2.92733294395268));
#61741=CARTESIAN_POINT('Ctrl Pts',(-2.68954721165342,-1.,2.92373955325876));
#61742=CARTESIAN_POINT('Ctrl Pts',(-2.68954721165342,1.,2.92373955325876));
#61743=CARTESIAN_POINT('Ctrl Pts',(-2.68290409279689,-1.,2.92011090722152));
#61744=CARTESIAN_POINT('Ctrl Pts',(-2.68290409279689,1.,2.92011090722152));
#61745=CARTESIAN_POINT('Ctrl Pts',(-2.67628728855309,-1.,2.91644290704281));
#61746=CARTESIAN_POINT('Ctrl Pts',(-2.67628728855309,1.,2.91644290704281));
#61747=CARTESIAN_POINT('Ctrl Pts',(-2.66969458792627,-1.,2.91273193382876));
#61748=CARTESIAN_POINT('Ctrl Pts',(-2.66969458792627,1.,2.91273193382876));
#61749=CARTESIAN_POINT('Ctrl Pts',(-2.66312542616809,-1.,2.90897617968921));
#61750=CARTESIAN_POINT('Ctrl Pts',(-2.66312542616809,1.,2.90897617968921));
#61751=CARTESIAN_POINT('Ctrl Pts',(-2.65658188464287,-1.,2.90517678087467));
#61752=CARTESIAN_POINT('Ctrl Pts',(-2.65658188464287,1.,2.90517678087467));
#61753=CARTESIAN_POINT('Ctrl Pts',(-2.65007017365576,-1.,2.90133950224879));
#61754=CARTESIAN_POINT('Ctrl Pts',(-2.65007017365576,1.,2.90133950224879));
#61755=CARTESIAN_POINT('Ctrl Pts',(-2.64359851684146,-1.,2.89747231723361));
#61756=CARTESIAN_POINT('Ctrl Pts',(-2.64359851684146,1.,2.89747231723361));
#61757=CARTESIAN_POINT('Ctrl Pts',(-2.63717442263944,-1.,2.89358228854557));
#61758=CARTESIAN_POINT('Ctrl Pts',(-2.63717442263944,1.,2.89358228854557));
#61759=CARTESIAN_POINT('Ctrl Pts',(-2.63080195420771,-1.,2.88967244854243));
#61760=CARTESIAN_POINT('Ctrl Pts',(-2.63080195420771,1.,2.88967244854243));
#61761=CARTESIAN_POINT('Ctrl Pts',(-2.62447947640253,-1.,2.88573922195049));
#61762=CARTESIAN_POINT('Ctrl Pts',(-2.62447947640253,1.,2.88573922195049));
#61763=CARTESIAN_POINT('Ctrl Pts',(-2.61819596473087,-1.,2.88176821427502));
#61764=CARTESIAN_POINT('Ctrl Pts',(-2.61819596473087,1.,2.88176821427502));
#61765=CARTESIAN_POINT('Ctrl Pts',(-2.61193507170928,-1.,2.87773881947885));
#61766=CARTESIAN_POINT('Ctrl Pts',(-2.61193507170928,1.,2.87773881947885));
#61767=CARTESIAN_POINT('Ctrl Pts',(-2.6056817788128,-1.,2.87363176656475));
#61768=CARTESIAN_POINT('Ctrl Pts',(-2.6056817788128,1.,2.87363176656475));
#61769=CARTESIAN_POINT('Ctrl Pts',(-2.59942875223202,-1.,2.86943633170712));
#61770=CARTESIAN_POINT('Ctrl Pts',(-2.59942875223202,1.,2.86943633170712));
#61771=CARTESIAN_POINT('Ctrl Pts',(-2.59318160184921,-1.,2.86515629953528));
#61772=CARTESIAN_POINT('Ctrl Pts',(-2.59318160184921,1.,2.86515629953528));
#61773=CARTESIAN_POINT('Ctrl Pts',(-2.5869677064356,-1.,2.86081999003668));
#61774=CARTESIAN_POINT('Ctrl Pts',(-2.5869677064356,1.,2.86081999003668));
#61775=CARTESIAN_POINT('Ctrl Pts',(-2.58082875254407,-1.,2.85647171715147));
#61776=CARTESIAN_POINT('Ctrl Pts',(-2.58082875254407,1.,2.85647171715147));
#61777=CARTESIAN_POINT('Ctrl Pts',(-2.57480482727128,-1.,2.85215360144483));
#61778=CARTESIAN_POINT('Ctrl Pts',(-2.57480482727128,1.,2.85215360144483));
#61779=CARTESIAN_POINT('Ctrl Pts',(-2.56891984251743,-1.,2.84788893329091));
#61780=CARTESIAN_POINT('Ctrl Pts',(-2.56891984251743,1.,2.84788893329091));
#61781=CARTESIAN_POINT('Ctrl Pts',(-2.56316920798489,-1.,2.84366802680211));
#61782=CARTESIAN_POINT('Ctrl Pts',(-2.56316920798489,1.,2.84366802680211));
#61783=CARTESIAN_POINT('Ctrl Pts',(-2.55749952145165,-1.,2.83942515220699));
#61784=CARTESIAN_POINT('Ctrl Pts',(-2.55749952145165,1.,2.83942515220699));
#61785=CARTESIAN_POINT('Ctrl Pts',(-2.55182152806964,-1.,2.83505269592412));
#61786=CARTESIAN_POINT('Ctrl Pts',(-2.55182152806964,1.,2.83505269592412));
#61787=CARTESIAN_POINT('Ctrl Pts',(-2.54604736792542,-1.,2.83044254225794));
#61788=CARTESIAN_POINT('Ctrl Pts',(-2.54604736792542,1.,2.83044254225794));
#61789=CARTESIAN_POINT('Ctrl Pts',(-2.54012272520141,-1.,2.82552167649157));
#61790=CARTESIAN_POINT('Ctrl Pts',(-2.54012272520141,1.,2.82552167649157));
#61791=CARTESIAN_POINT('Ctrl Pts',(-2.53405679667463,-1.,2.82028550483744));
#61792=CARTESIAN_POINT('Ctrl Pts',(-2.53405679667463,1.,2.82028550483744));
#61793=CARTESIAN_POINT('Ctrl Pts',(-2.52796388055457,-1.,2.8148437904867));
#61794=CARTESIAN_POINT('Ctrl Pts',(-2.52796388055457,1.,2.8148437904867));
#61795=CARTESIAN_POINT('Ctrl Pts',(-2.52205778589922,-1.,2.80941521967234));
#61796=CARTESIAN_POINT('Ctrl Pts',(-2.52205778589922,1.,2.80941521967234));
#61797=CARTESIAN_POINT('Ctrl Pts',(-2.51660190466067,-1.,2.80427363984939));
#61798=CARTESIAN_POINT('Ctrl Pts',(-2.51660190466067,1.,2.80427363984939));
#61799=CARTESIAN_POINT('Ctrl Pts',(-2.51186983687947,-1.,2.79970585014308));
#61800=CARTESIAN_POINT('Ctrl Pts',(-2.51186983687947,1.,2.79970585014308));
#61801=CARTESIAN_POINT('Ctrl Pts',(-2.50810555977564,-1.,2.7959687805717));
#61802=CARTESIAN_POINT('Ctrl Pts',(-2.50810555977564,1.,2.7959687805717));
#61803=CARTESIAN_POINT('Ctrl Pts',(-2.50547439929077,-1.,2.79323694088143));
#61804=CARTESIAN_POINT('Ctrl Pts',(-2.50547439929077,1.,2.79323694088143));
#61805=CARTESIAN_POINT('Ctrl Pts',(-2.50433799076945,-1.,2.79192122906739));
#61806=CARTESIAN_POINT('Ctrl Pts',(-2.50433799076945,1.,2.79192122906739));
#61807=CARTESIAN_POINT('Ctrl Pts',(-2.50404230339032,-1.,2.79143626022225));
#61808=CARTESIAN_POINT('Ctrl Pts',(-2.50404230339032,1.,2.79143626022225));
#61809=CARTESIAN_POINT('Ctrl Pts',(-2.50409239460011,-1.,2.79133581100044));
#61810=CARTESIAN_POINT('Ctrl Pts',(-2.50409239460011,1.,2.79133581100044));
#61811=CARTESIAN_POINT('Ctrl Pts',(-2.50417924854921,-1.,2.79134130681569));
#61812=CARTESIAN_POINT('Ctrl Pts',(-2.50417924854921,1.,2.79134130681569));
#61813=CARTESIAN_POINT('',(-2.91557726271063,1.,3.02314558451372));
#61814=CARTESIAN_POINT('Ctrl Pts',(-2.91557726271063,1.,3.02314558451372));
#61815=CARTESIAN_POINT('Ctrl Pts',(-2.91409518070707,1.,3.02261975104912));
#61816=CARTESIAN_POINT('Ctrl Pts',(-2.91113297349052,1.,3.02156522743299));
#61817=CARTESIAN_POINT('Ctrl Pts',(-2.90669553303902,1.,3.01997487194926));
#61818=CARTESIAN_POINT('Ctrl Pts',(-2.90079069102661,1.,3.01783725123646));
#61819=CARTESIAN_POINT('Ctrl Pts',(-2.8934292556764,1.,3.01513660433291));
#61820=CARTESIAN_POINT('Ctrl Pts',(-2.88608751706796,1.,3.01240727309568));
#61821=CARTESIAN_POINT('Ctrl Pts',(-2.87876560072799,1.,3.0096491810855));
#61822=CARTESIAN_POINT('Ctrl Pts',(-2.87146368430104,1.,3.00686224485374));
#61823=CARTESIAN_POINT('Ctrl Pts',(-2.86418200833065,1.,3.00404638316245));
#61824=CARTESIAN_POINT('Ctrl Pts',(-2.85692085715129,1.,3.0012015079552));
#61825=CARTESIAN_POINT('Ctrl Pts',(-2.84968053289104,1.,2.99832751144566));
#61826=CARTESIAN_POINT('Ctrl Pts',(-2.84246132984334,1.,2.995424253416));
#61827=CARTESIAN_POINT('Ctrl Pts',(-2.83526351254383,1.,2.99249155170479));
#61828=CARTESIAN_POINT('Ctrl Pts',(-2.82808728190402,1.,2.98952916401699));
#61829=CARTESIAN_POINT('Ctrl Pts',(-2.82093279065704,1.,2.98653680669434));
#61830=CARTESIAN_POINT('Ctrl Pts',(-2.81380019196454,1.,2.9835141977994));
#61831=CARTESIAN_POINT('Ctrl Pts',(-2.80668968101162,1.,2.98046109647299));
#61832=CARTESIAN_POINT('Ctrl Pts',(-2.79960153278186,1.,2.97737733718242));
#61833=CARTESIAN_POINT('Ctrl Pts',(-2.79253615718147,1.,2.97426288347475));
#61834=CARTESIAN_POINT('Ctrl Pts',(-2.78549409123657,1.,2.97111781461349));
#61835=CARTESIAN_POINT('Ctrl Pts',(-2.77847589542767,1.,2.9679422104295));
#61836=CARTESIAN_POINT('Ctrl Pts',(-2.77148206836464,1.,2.96473605585548));
#61837=CARTESIAN_POINT('Ctrl Pts',(-2.76451296269571,1.,2.96149914764832));
#61838=CARTESIAN_POINT('Ctrl Pts',(-2.75756867888393,1.,2.9582309766594));
#61839=CARTESIAN_POINT('Ctrl Pts',(-2.75064903318996,1.,2.95493069316211));
#61840=CARTESIAN_POINT('Ctrl Pts',(-2.7437537949221,1.,2.95159737214305));
#61841=CARTESIAN_POINT('Ctrl Pts',(-2.73688288329825,1.,2.94823023414381));
#61842=CARTESIAN_POINT('Ctrl Pts',(-2.73003657371613,1.,2.94482887675139));
#61843=CARTESIAN_POINT('Ctrl Pts',(-2.72321571511322,1.,2.94139351933882));
#61844=CARTESIAN_POINT('Ctrl Pts',(-2.71642190053575,1.,2.93792519474955));
#61845=CARTESIAN_POINT('Ctrl Pts',(-2.70965695523776,1.,2.93442516311168));
#61846=CARTESIAN_POINT('Ctrl Pts',(-2.70292247416881,1.,2.93089438233746));
#61847=CARTESIAN_POINT('Ctrl Pts',(-2.69621932864302,1.,2.92733294395268));
#61848=CARTESIAN_POINT('Ctrl Pts',(-2.68954721165342,1.,2.92373955325876));
#61849=CARTESIAN_POINT('Ctrl Pts',(-2.68290409279689,1.,2.92011090722152));
#61850=CARTESIAN_POINT('Ctrl Pts',(-2.67628728855309,1.,2.91644290704281));
#61851=CARTESIAN_POINT('Ctrl Pts',(-2.66969458792627,1.,2.91273193382876));
#61852=CARTESIAN_POINT('Ctrl Pts',(-2.66312542616809,1.,2.90897617968921));
#61853=CARTESIAN_POINT('Ctrl Pts',(-2.65658188464287,1.,2.90517678087467));
#61854=CARTESIAN_POINT('Ctrl Pts',(-2.65007017365576,1.,2.90133950224879));
#61855=CARTESIAN_POINT('Ctrl Pts',(-2.64359851684146,1.,2.89747231723361));
#61856=CARTESIAN_POINT('Ctrl Pts',(-2.63717442263944,1.,2.89358228854557));
#61857=CARTESIAN_POINT('Ctrl Pts',(-2.63080195420771,1.,2.88967244854243));
#61858=CARTESIAN_POINT('Ctrl Pts',(-2.62447947640253,1.,2.88573922195049));
#61859=CARTESIAN_POINT('Ctrl Pts',(-2.61819596473087,1.,2.88176821427502));
#61860=CARTESIAN_POINT('Ctrl Pts',(-2.61193507170928,1.,2.87773881947885));
#61861=CARTESIAN_POINT('Ctrl Pts',(-2.6056817788128,1.,2.87363176656475));
#61862=CARTESIAN_POINT('Ctrl Pts',(-2.59942875223202,1.,2.86943633170712));
#61863=CARTESIAN_POINT('Ctrl Pts',(-2.59318160184921,1.,2.86515629953528));
#61864=CARTESIAN_POINT('Ctrl Pts',(-2.5869677064356,1.,2.86081999003668));
#61865=CARTESIAN_POINT('Ctrl Pts',(-2.58082875254407,1.,2.85647171715147));
#61866=CARTESIAN_POINT('Ctrl Pts',(-2.57480482727128,1.,2.85215360144483));
#61867=CARTESIAN_POINT('Ctrl Pts',(-2.56891984251743,1.,2.84788893329091));
#61868=CARTESIAN_POINT('Ctrl Pts',(-2.56316920798489,1.,2.84366802680211));
#61869=CARTESIAN_POINT('Ctrl Pts',(-2.55749952145165,1.,2.83942515220699));
#61870=CARTESIAN_POINT('Ctrl Pts',(-2.55182152806964,1.,2.83505269592412));
#61871=CARTESIAN_POINT('Ctrl Pts',(-2.54604736792542,1.,2.83044254225794));
#61872=CARTESIAN_POINT('Ctrl Pts',(-2.54012272520141,1.,2.82552167649157));
#61873=CARTESIAN_POINT('Ctrl Pts',(-2.53405679667463,1.,2.82028550483744));
#61874=CARTESIAN_POINT('Ctrl Pts',(-2.52796388055457,1.,2.8148437904867));
#61875=CARTESIAN_POINT('Ctrl Pts',(-2.52205778589922,1.,2.80941521967234));
#61876=CARTESIAN_POINT('Ctrl Pts',(-2.51660190466067,1.,2.80427363984939));
#61877=CARTESIAN_POINT('Ctrl Pts',(-2.51186983687947,1.,2.79970585014308));
#61878=CARTESIAN_POINT('Ctrl Pts',(-2.50810555977564,1.,2.7959687805717));
#61879=CARTESIAN_POINT('Ctrl Pts',(-2.50567182569153,1.,2.79344192164204));
#61880=CARTESIAN_POINT('Ctrl Pts',(-2.50455968395235,1.,2.79217568804874));
#61881=CARTESIAN_POINT('Ctrl Pts',(-2.50417932839343,1.,2.79164172519039));
#61882=CARTESIAN_POINT('Ctrl Pts',(-2.50410700351427,1.,2.79145823440899));
#61883=CARTESIAN_POINT('Ctrl Pts',(-2.50410331873043,1.,2.79140942341378));
#61884=CARTESIAN_POINT('',(-2.91557726271063,0.,3.02314558451372));
#61885=CARTESIAN_POINT('Ctrl Pts',(-2.79134130681569,-1.,2.50417924854921));
#61886=CARTESIAN_POINT('Ctrl Pts',(-2.79134130681569,1.,2.50417924854921));
#61887=CARTESIAN_POINT('Ctrl Pts',(-2.7913358110015,-1.,2.50409239460108));
#61888=CARTESIAN_POINT('Ctrl Pts',(-2.7913358110015,1.,2.50409239460108));
#61889=CARTESIAN_POINT('Ctrl Pts',(-2.79143626022503,-1.,2.50404230339286));
#61890=CARTESIAN_POINT('Ctrl Pts',(-2.79143626022503,1.,2.50404230339286));
#61891=CARTESIAN_POINT('Ctrl Pts',(-2.79192122907148,-1.,2.5043379907732));
#61892=CARTESIAN_POINT('Ctrl Pts',(-2.79192122907148,1.,2.5043379907732));
#61893=CARTESIAN_POINT('Ctrl Pts',(-2.7932369408851,-1.,2.50547439929414));
#61894=CARTESIAN_POINT('Ctrl Pts',(-2.7932369408851,1.,2.50547439929414));
#61895=CARTESIAN_POINT('Ctrl Pts',(-2.79596878057287,-1.,2.50810555977671));
#61896=CARTESIAN_POINT('Ctrl Pts',(-2.79596878057287,1.,2.50810555977671));
#61897=CARTESIAN_POINT('Ctrl Pts',(-2.79970585014168,-1.,2.51186983687818));
#61898=CARTESIAN_POINT('Ctrl Pts',(-2.79970585014168,1.,2.51186983687818));
#61899=CARTESIAN_POINT('Ctrl Pts',(-2.80427363984653,-1.,2.51660190465805));
#61900=CARTESIAN_POINT('Ctrl Pts',(-2.80427363984653,1.,2.51660190465805));
#61901=CARTESIAN_POINT('Ctrl Pts',(-2.80941521966941,-1.,2.52205778589653));
#61902=CARTESIAN_POINT('Ctrl Pts',(-2.80941521966941,1.,2.52205778589653));
#61903=CARTESIAN_POINT('Ctrl Pts',(-2.81484379048475,-1.,2.52796388055278));
#61904=CARTESIAN_POINT('Ctrl Pts',(-2.81484379048475,1.,2.52796388055278));
#61905=CARTESIAN_POINT('Ctrl Pts',(-2.82028550483689,-1.,2.53405679667412));
#61906=CARTESIAN_POINT('Ctrl Pts',(-2.82028550483689,1.,2.53405679667412));
#61907=CARTESIAN_POINT('Ctrl Pts',(-2.8255216764922,-1.,2.54012272520199));
#61908=CARTESIAN_POINT('Ctrl Pts',(-2.8255216764922,1.,2.54012272520199));
#61909=CARTESIAN_POINT('Ctrl Pts',(-2.83044254225917,-1.,2.54604736792655));
#61910=CARTESIAN_POINT('Ctrl Pts',(-2.83044254225917,1.,2.54604736792655));
#61911=CARTESIAN_POINT('Ctrl Pts',(-2.83505269592536,-1.,2.55182152807077));
#61912=CARTESIAN_POINT('Ctrl Pts',(-2.83505269592536,1.,2.55182152807077));
#61913=CARTESIAN_POINT('Ctrl Pts',(-2.83942515220782,-1.,2.55749952145241));
#61914=CARTESIAN_POINT('Ctrl Pts',(-2.83942515220782,1.,2.55749952145241));
#61915=CARTESIAN_POINT('Ctrl Pts',(-2.84366802680237,-1.,2.56316920798513));
#61916=CARTESIAN_POINT('Ctrl Pts',(-2.84366802680237,1.,2.56316920798513));
#61917=CARTESIAN_POINT('Ctrl Pts',(-2.84788893329067,-1.,2.56891984251721));
#61918=CARTESIAN_POINT('Ctrl Pts',(-2.84788893329067,1.,2.56891984251721));
#61919=CARTESIAN_POINT('Ctrl Pts',(-2.85215360144431,-1.,2.57480482727081));
#61920=CARTESIAN_POINT('Ctrl Pts',(-2.85215360144431,1.,2.57480482727081));
#61921=CARTESIAN_POINT('Ctrl Pts',(-2.85647171715092,-1.,2.58082875254357));
#61922=CARTESIAN_POINT('Ctrl Pts',(-2.85647171715092,1.,2.58082875254357));
#61923=CARTESIAN_POINT('Ctrl Pts',(-2.86081999003629,-1.,2.58696770643524));
#61924=CARTESIAN_POINT('Ctrl Pts',(-2.86081999003629,1.,2.58696770643524));
#61925=CARTESIAN_POINT('Ctrl Pts',(-2.86515629953513,-1.,2.59318160184908));
#61926=CARTESIAN_POINT('Ctrl Pts',(-2.86515629953513,1.,2.59318160184908));
#61927=CARTESIAN_POINT('Ctrl Pts',(-2.86943633170722,-1.,2.5994287522321));
#61928=CARTESIAN_POINT('Ctrl Pts',(-2.86943633170722,1.,2.5994287522321));
#61929=CARTESIAN_POINT('Ctrl Pts',(-2.87363176656501,-1.,2.60568177881303));
#61930=CARTESIAN_POINT('Ctrl Pts',(-2.87363176656501,1.,2.60568177881303));
#61931=CARTESIAN_POINT('Ctrl Pts',(-2.87773881947916,-1.,2.61193507170955));
#61932=CARTESIAN_POINT('Ctrl Pts',(-2.87773881947916,1.,2.61193507170955));
#61933=CARTESIAN_POINT('Ctrl Pts',(-2.88176821427525,-1.,2.61819596473108));
#61934=CARTESIAN_POINT('Ctrl Pts',(-2.88176821427525,1.,2.61819596473108));
#61935=CARTESIAN_POINT('Ctrl Pts',(-2.88573922195059,-1.,2.62447947640262));
#61936=CARTESIAN_POINT('Ctrl Pts',(-2.88573922195059,1.,2.62447947640262));
#61937=CARTESIAN_POINT('Ctrl Pts',(-2.88967244854239,-1.,2.63080195420767));
#61938=CARTESIAN_POINT('Ctrl Pts',(-2.88967244854239,1.,2.63080195420767));
#61939=CARTESIAN_POINT('Ctrl Pts',(-2.89358228854544,-1.,2.63717442263932));
#61940=CARTESIAN_POINT('Ctrl Pts',(-2.89358228854544,1.,2.63717442263932));
#61941=CARTESIAN_POINT('Ctrl Pts',(-2.89747231723345,-1.,2.64359851684131));
#61942=CARTESIAN_POINT('Ctrl Pts',(-2.89747231723345,1.,2.64359851684131));
#61943=CARTESIAN_POINT('Ctrl Pts',(-2.90133950224867,-1.,2.65007017365564));
#61944=CARTESIAN_POINT('Ctrl Pts',(-2.90133950224867,1.,2.65007017365564));
#61945=CARTESIAN_POINT('Ctrl Pts',(-2.90517678087461,-1.,2.65658188464282));
#61946=CARTESIAN_POINT('Ctrl Pts',(-2.90517678087461,1.,2.65658188464282));
#61947=CARTESIAN_POINT('Ctrl Pts',(-2.90897617968923,-1.,2.6631254261681));
#61948=CARTESIAN_POINT('Ctrl Pts',(-2.90897617968923,1.,2.6631254261681));
#61949=CARTESIAN_POINT('Ctrl Pts',(-2.91273193382882,-1.,2.66969458792631));
#61950=CARTESIAN_POINT('Ctrl Pts',(-2.91273193382882,1.,2.66969458792631));
#61951=CARTESIAN_POINT('Ctrl Pts',(-2.91644290704285,-1.,2.67628728855312));
#61952=CARTESIAN_POINT('Ctrl Pts',(-2.91644290704285,1.,2.67628728855312));
#61953=CARTESIAN_POINT('Ctrl Pts',(-2.92011090722152,-1.,2.68290409279688));
#61954=CARTESIAN_POINT('Ctrl Pts',(-2.92011090722152,1.,2.68290409279688));
#61955=CARTESIAN_POINT('Ctrl Pts',(-2.92373955325875,-1.,2.68954721165339));
#61956=CARTESIAN_POINT('Ctrl Pts',(-2.92373955325875,1.,2.68954721165339));
#61957=CARTESIAN_POINT('Ctrl Pts',(-2.92733294395267,-1.,2.69621932864301));
#61958=CARTESIAN_POINT('Ctrl Pts',(-2.92733294395267,1.,2.69621932864301));
#61959=CARTESIAN_POINT('Ctrl Pts',(-2.9308943823375,-1.,2.70292247416885));
#61960=CARTESIAN_POINT('Ctrl Pts',(-2.9308943823375,1.,2.70292247416885));
#61961=CARTESIAN_POINT('Ctrl Pts',(-2.93442516311179,-1.,2.70965695523787));
#61962=CARTESIAN_POINT('Ctrl Pts',(-2.93442516311179,1.,2.70965695523787));
#61963=CARTESIAN_POINT('Ctrl Pts',(-2.93792519474972,-1.,2.71642190053592));
#61964=CARTESIAN_POINT('Ctrl Pts',(-2.93792519474972,1.,2.71642190053592));
#61965=CARTESIAN_POINT('Ctrl Pts',(-2.94139351933897,-1.,2.72321571511337));
#61966=CARTESIAN_POINT('Ctrl Pts',(-2.94139351933897,1.,2.72321571511337));
#61967=CARTESIAN_POINT('Ctrl Pts',(-2.94482887675143,-1.,2.73003657371617));
#61968=CARTESIAN_POINT('Ctrl Pts',(-2.94482887675143,1.,2.73003657371617));
#61969=CARTESIAN_POINT('Ctrl Pts',(-2.94823023414364,-1.,2.73688288329808));
#61970=CARTESIAN_POINT('Ctrl Pts',(-2.94823023414364,1.,2.73688288329808));
#61971=CARTESIAN_POINT('Ctrl Pts',(-2.95159737214266,-1.,2.74375379492172));
#61972=CARTESIAN_POINT('Ctrl Pts',(-2.95159737214266,1.,2.74375379492172));
#61973=CARTESIAN_POINT('Ctrl Pts',(-2.95493069316161,-1.,2.75064903318947));
#61974=CARTESIAN_POINT('Ctrl Pts',(-2.95493069316161,1.,2.75064903318947));
#61975=CARTESIAN_POINT('Ctrl Pts',(-2.95823097665896,-1.,2.7575686788835));
#61976=CARTESIAN_POINT('Ctrl Pts',(-2.95823097665896,1.,2.7575686788835));
#61977=CARTESIAN_POINT('Ctrl Pts',(-2.96149914764818,-1.,2.76451296269557));
#61978=CARTESIAN_POINT('Ctrl Pts',(-2.96149914764818,1.,2.76451296269557));
#61979=CARTESIAN_POINT('Ctrl Pts',(-2.96473605585583,-1.,2.77148206836498));
#61980=CARTESIAN_POINT('Ctrl Pts',(-2.96473605585583,1.,2.77148206836498));
#61981=CARTESIAN_POINT('Ctrl Pts',(-2.96794221043036,-1.,2.7784758954285));
#61982=CARTESIAN_POINT('Ctrl Pts',(-2.96794221043036,1.,2.7784758954285));
#61983=CARTESIAN_POINT('Ctrl Pts',(-2.97111781461465,-1.,2.78549409123769));
#61984=CARTESIAN_POINT('Ctrl Pts',(-2.97111781461465,1.,2.78549409123769));
#61985=CARTESIAN_POINT('Ctrl Pts',(-2.9742628834758,-1.,2.79253615718248));
#61986=CARTESIAN_POINT('Ctrl Pts',(-2.9742628834758,1.,2.79253615718248));
#61987=CARTESIAN_POINT('Ctrl Pts',(-2.97737733718287,-1.,2.7996015327823));
#61988=CARTESIAN_POINT('Ctrl Pts',(-2.97737733718287,1.,2.7996015327823));
#61989=CARTESIAN_POINT('Ctrl Pts',(-2.98046109647241,-1.,2.80668968101106));
#61990=CARTESIAN_POINT('Ctrl Pts',(-2.98046109647241,1.,2.80668968101106));
#61991=CARTESIAN_POINT('Ctrl Pts',(-2.98351419779767,-1.,2.81380019196286));
#61992=CARTESIAN_POINT('Ctrl Pts',(-2.98351419779767,1.,2.81380019196286));
#61993=CARTESIAN_POINT('Ctrl Pts',(-2.9865368066918,-1.,2.82093279065457));
#61994=CARTESIAN_POINT('Ctrl Pts',(-2.9865368066918,1.,2.82093279065457));
#61995=CARTESIAN_POINT('Ctrl Pts',(-2.98952916401446,-1.,2.82808728190157));
#61996=CARTESIAN_POINT('Ctrl Pts',(-2.98952916401446,1.,2.82808728190157));
#61997=CARTESIAN_POINT('Ctrl Pts',(-2.9924915517034,-1.,2.83526351254248));
#61998=CARTESIAN_POINT('Ctrl Pts',(-2.9924915517034,1.,2.83526351254248));
#61999=CARTESIAN_POINT('Ctrl Pts',(-2.99542425341685,-1.,2.84246132984415));
#62000=CARTESIAN_POINT('Ctrl Pts',(-2.99542425341685,1.,2.84246132984415));
#62001=CARTESIAN_POINT('Ctrl Pts',(-2.99832751144925,-1.,2.84968053289451));
#62002=CARTESIAN_POINT('Ctrl Pts',(-2.99832751144925,1.,2.84968053289451));
#62003=CARTESIAN_POINT('Ctrl Pts',(-3.00120150796095,-1.,2.85692085715686));
#62004=CARTESIAN_POINT('Ctrl Pts',(-3.00120150796095,1.,2.85692085715686));
#62005=CARTESIAN_POINT('Ctrl Pts',(-3.00404638316867,-1.,2.86418200833667));
#62006=CARTESIAN_POINT('Ctrl Pts',(-3.00404638316867,1.,2.86418200833667));
#62007=CARTESIAN_POINT('Ctrl Pts',(-3.00686224485784,-1.,2.87146368430502));
#62008=CARTESIAN_POINT('Ctrl Pts',(-3.00686224485784,1.,2.87146368430502));
#62009=CARTESIAN_POINT('Ctrl Pts',(-3.00964918108476,-1.,2.87876560072727));
#62010=CARTESIAN_POINT('Ctrl Pts',(-3.00964918108476,1.,2.87876560072727));
#62011=CARTESIAN_POINT('Ctrl Pts',(-3.01240727308829,-1.,2.8860875170608));
#62012=CARTESIAN_POINT('Ctrl Pts',(-3.01240727308829,1.,2.8860875170608));
#62013=CARTESIAN_POINT('Ctrl Pts',(-3.01513660431928,-1.,2.89342925566321));
#62014=CARTESIAN_POINT('Ctrl Pts',(-3.01513660431928,1.,2.89342925566321));
#62015=CARTESIAN_POINT('Ctrl Pts',(-3.01783725121981,-1.,2.9007906910105));
#62016=CARTESIAN_POINT('Ctrl Pts',(-3.01783725121981,1.,2.9007906910105));
#62017=CARTESIAN_POINT('Ctrl Pts',(-3.01997487193503,-1.,2.90669553302526));
#62018=CARTESIAN_POINT('Ctrl Pts',(-3.01997487193503,1.,2.90669553302526));
#62019=CARTESIAN_POINT('Ctrl Pts',(-3.02156522742431,-1.,2.91113297348212));
#62020=CARTESIAN_POINT('Ctrl Pts',(-3.02156522742431,1.,2.91113297348212));
#62021=CARTESIAN_POINT('Ctrl Pts',(-3.02261975104593,-1.,2.91409518070399));
#62022=CARTESIAN_POINT('Ctrl Pts',(-3.02261975104593,1.,2.91409518070399));
#62023=CARTESIAN_POINT('Ctrl Pts',(-3.02314558451372,-1.,2.91557726271063));
#62024=CARTESIAN_POINT('Ctrl Pts',(-3.02314558451372,1.,2.91557726271063));
#62025=CARTESIAN_POINT('',(-2.79140942341258,1.,2.50410331873176));
#62026=CARTESIAN_POINT('Ctrl Pts',(-2.79140942341258,-1.,2.50410331873176));
#62027=CARTESIAN_POINT('Ctrl Pts',(-2.79140942341258,-0.666666666666667,
2.50410331873176));
#62028=CARTESIAN_POINT('Ctrl Pts',(-2.79140942341258,-0.333333333333333,
2.50410331873176));
#62029=CARTESIAN_POINT('Ctrl Pts',(-2.79140942341258,0.333333333333333,
2.50410331873176));
#62030=CARTESIAN_POINT('Ctrl Pts',(-2.79140942341258,0.666666666666667,
2.50410331873176));
#62031=CARTESIAN_POINT('Ctrl Pts',(-2.79140942341258,1.,2.50410331873176));
#62032=CARTESIAN_POINT('',(-3.02314558451372,1.,2.91557726271063));
#62033=CARTESIAN_POINT('',(-3.02314558451372,0.,2.91557726271063));
#62034=CARTESIAN_POINT('Ctrl Pts',(-2.79140942341258,1.,2.50410331873176));
#62035=CARTESIAN_POINT('Ctrl Pts',(-2.79145823440781,1.,2.50410700351493));
#62036=CARTESIAN_POINT('Ctrl Pts',(-2.79164172518905,1.,2.50417932839313));
#62037=CARTESIAN_POINT('Ctrl Pts',(-2.79217568804755,1.,2.50455968395146));
#62038=CARTESIAN_POINT('Ctrl Pts',(-2.79344192164147,1.,2.50567182569081));
#62039=CARTESIAN_POINT('Ctrl Pts',(-2.79596878057287,1.,2.50810555977671));
#62040=CARTESIAN_POINT('Ctrl Pts',(-2.79970585014168,1.,2.51186983687818));
#62041=CARTESIAN_POINT('Ctrl Pts',(-2.80427363984653,1.,2.51660190465805));
#62042=CARTESIAN_POINT('Ctrl Pts',(-2.80941521966941,1.,2.52205778589653));
#62043=CARTESIAN_POINT('Ctrl Pts',(-2.81484379048475,1.,2.52796388055278));
#62044=CARTESIAN_POINT('Ctrl Pts',(-2.82028550483689,1.,2.53405679667412));
#62045=CARTESIAN_POINT('Ctrl Pts',(-2.8255216764922,1.,2.54012272520199));
#62046=CARTESIAN_POINT('Ctrl Pts',(-2.83044254225917,1.,2.54604736792655));
#62047=CARTESIAN_POINT('Ctrl Pts',(-2.83505269592536,1.,2.55182152807077));
#62048=CARTESIAN_POINT('Ctrl Pts',(-2.83942515220782,1.,2.55749952145241));
#62049=CARTESIAN_POINT('Ctrl Pts',(-2.84366802680237,1.,2.56316920798513));
#62050=CARTESIAN_POINT('Ctrl Pts',(-2.84788893329067,1.,2.56891984251721));
#62051=CARTESIAN_POINT('Ctrl Pts',(-2.85215360144431,1.,2.57480482727081));
#62052=CARTESIAN_POINT('Ctrl Pts',(-2.85647171715092,1.,2.58082875254357));
#62053=CARTESIAN_POINT('Ctrl Pts',(-2.86081999003629,1.,2.58696770643524));
#62054=CARTESIAN_POINT('Ctrl Pts',(-2.86515629953513,1.,2.59318160184908));
#62055=CARTESIAN_POINT('Ctrl Pts',(-2.86943633170722,1.,2.5994287522321));
#62056=CARTESIAN_POINT('Ctrl Pts',(-2.87363176656501,1.,2.60568177881303));
#62057=CARTESIAN_POINT('Ctrl Pts',(-2.87773881947916,1.,2.61193507170955));
#62058=CARTESIAN_POINT('Ctrl Pts',(-2.88176821427525,1.,2.61819596473108));
#62059=CARTESIAN_POINT('Ctrl Pts',(-2.88573922195059,1.,2.62447947640262));
#62060=CARTESIAN_POINT('Ctrl Pts',(-2.88967244854239,1.,2.63080195420767));
#62061=CARTESIAN_POINT('Ctrl Pts',(-2.89358228854544,1.,2.63717442263932));
#62062=CARTESIAN_POINT('Ctrl Pts',(-2.89747231723345,1.,2.64359851684131));
#62063=CARTESIAN_POINT('Ctrl Pts',(-2.90133950224867,1.,2.65007017365564));
#62064=CARTESIAN_POINT('Ctrl Pts',(-2.90517678087461,1.,2.65658188464282));
#62065=CARTESIAN_POINT('Ctrl Pts',(-2.90897617968923,1.,2.6631254261681));
#62066=CARTESIAN_POINT('Ctrl Pts',(-2.91273193382882,1.,2.66969458792631));
#62067=CARTESIAN_POINT('Ctrl Pts',(-2.91644290704285,1.,2.67628728855312));
#62068=CARTESIAN_POINT('Ctrl Pts',(-2.92011090722152,1.,2.68290409279688));
#62069=CARTESIAN_POINT('Ctrl Pts',(-2.92373955325875,1.,2.68954721165339));
#62070=CARTESIAN_POINT('Ctrl Pts',(-2.92733294395267,1.,2.69621932864301));
#62071=CARTESIAN_POINT('Ctrl Pts',(-2.9308943823375,1.,2.70292247416885));
#62072=CARTESIAN_POINT('Ctrl Pts',(-2.93442516311179,1.,2.70965695523787));
#62073=CARTESIAN_POINT('Ctrl Pts',(-2.93792519474972,1.,2.71642190053592));
#62074=CARTESIAN_POINT('Ctrl Pts',(-2.94139351933897,1.,2.72321571511337));
#62075=CARTESIAN_POINT('Ctrl Pts',(-2.94482887675143,1.,2.73003657371617));
#62076=CARTESIAN_POINT('Ctrl Pts',(-2.94823023414364,1.,2.73688288329808));
#62077=CARTESIAN_POINT('Ctrl Pts',(-2.95159737214266,1.,2.74375379492172));
#62078=CARTESIAN_POINT('Ctrl Pts',(-2.95493069316161,1.,2.75064903318947));
#62079=CARTESIAN_POINT('Ctrl Pts',(-2.95823097665896,1.,2.7575686788835));
#62080=CARTESIAN_POINT('Ctrl Pts',(-2.96149914764818,1.,2.76451296269557));
#62081=CARTESIAN_POINT('Ctrl Pts',(-2.96473605585583,1.,2.77148206836498));
#62082=CARTESIAN_POINT('Ctrl Pts',(-2.96794221043036,1.,2.7784758954285));
#62083=CARTESIAN_POINT('Ctrl Pts',(-2.97111781461465,1.,2.78549409123769));
#62084=CARTESIAN_POINT('Ctrl Pts',(-2.9742628834758,1.,2.79253615718248));
#62085=CARTESIAN_POINT('Ctrl Pts',(-2.97737733718287,1.,2.7996015327823));
#62086=CARTESIAN_POINT('Ctrl Pts',(-2.98046109647241,1.,2.80668968101106));
#62087=CARTESIAN_POINT('Ctrl Pts',(-2.98351419779767,1.,2.81380019196286));
#62088=CARTESIAN_POINT('Ctrl Pts',(-2.9865368066918,1.,2.82093279065457));
#62089=CARTESIAN_POINT('Ctrl Pts',(-2.98952916401446,1.,2.82808728190157));
#62090=CARTESIAN_POINT('Ctrl Pts',(-2.9924915517034,1.,2.83526351254248));
#62091=CARTESIAN_POINT('Ctrl Pts',(-2.99542425341685,1.,2.84246132984415));
#62092=CARTESIAN_POINT('Ctrl Pts',(-2.99832751144925,1.,2.84968053289451));
#62093=CARTESIAN_POINT('Ctrl Pts',(-3.00120150796095,1.,2.85692085715686));
#62094=CARTESIAN_POINT('Ctrl Pts',(-3.00404638316867,1.,2.86418200833667));
#62095=CARTESIAN_POINT('Ctrl Pts',(-3.00686224485784,1.,2.87146368430502));
#62096=CARTESIAN_POINT('Ctrl Pts',(-3.00964918108476,1.,2.87876560072727));
#62097=CARTESIAN_POINT('Ctrl Pts',(-3.01240727308829,1.,2.8860875170608));
#62098=CARTESIAN_POINT('Ctrl Pts',(-3.01513660431928,1.,2.89342925566321));
#62099=CARTESIAN_POINT('Ctrl Pts',(-3.01783725121981,1.,2.9007906910105));
#62100=CARTESIAN_POINT('Ctrl Pts',(-3.01997487193503,1.,2.90669553302526));
#62101=CARTESIAN_POINT('Ctrl Pts',(-3.02156522742431,1.,2.91113297348212));
#62102=CARTESIAN_POINT('Ctrl Pts',(-3.02261975104593,1.,2.91409518070399));
#62103=CARTESIAN_POINT('Ctrl Pts',(-3.02314558451372,1.,2.91557726271063));
#62104=CARTESIAN_POINT('Origin',(-3.02314558451372,0.,2.91557726271063));
#62105=CARTESIAN_POINT('',(-2.91557726271063,1.,3.02314558451372));
#62106=CARTESIAN_POINT('Origin',(0.,0.,0.));
#62107=CARTESIAN_POINT('',(-2.90994629141562,1.,2.36531447826213));
#62108=CARTESIAN_POINT('Origin',(0.,1.,0.));
#62109=CARTESIAN_POINT('Ctrl Pts',(-2.90994629141562,1.,2.36531447826213));
#62110=CARTESIAN_POINT('Ctrl Pts',(-2.90994629141562,0.666666666666667,
2.36531447826213));
#62111=CARTESIAN_POINT('Ctrl Pts',(-2.90994629141562,0.333333333333333,
2.36531447826213));
#62112=CARTESIAN_POINT('Ctrl Pts',(-2.90994629141562,-0.333333333333333,
2.36531447826213));
#62113=CARTESIAN_POINT('Ctrl Pts',(-2.90994629141562,-0.666666666666667,
2.36531447826213));
#62114=CARTESIAN_POINT('Ctrl Pts',(-2.90994629141562,-1.,2.36531447826213));
#62115=CARTESIAN_POINT('Ctrl Pts',(-3.35260583073571,-1.,2.52982887637028));
#62116=CARTESIAN_POINT('Ctrl Pts',(-3.35260583073571,1.,2.52982887637028));
#62117=CARTESIAN_POINT('Ctrl Pts',(-3.35105973714426,-1.,2.52954136549357));
#62118=CARTESIAN_POINT('Ctrl Pts',(-3.35105973714426,1.,2.52954136549357));
#62119=CARTESIAN_POINT('Ctrl Pts',(-3.34796903577628,-1.,2.5289632161143));
#62120=CARTESIAN_POINT('Ctrl Pts',(-3.34796903577628,1.,2.5289632161143));
#62121=CARTESIAN_POINT('Ctrl Pts',(-3.34333744117093,-1.,2.52808660916879));
#62122=CARTESIAN_POINT('Ctrl Pts',(-3.34333744117093,1.,2.52808660916879));
#62123=CARTESIAN_POINT('Ctrl Pts',(-3.33717090000955,-1.,2.52689902691551));
#62124=CARTESIAN_POINT('Ctrl Pts',(-3.33717090000955,1.,2.52689902691551));
#62125=CARTESIAN_POINT('Ctrl Pts',(-3.32947762189049,-1.,2.52538321165774));
#62126=CARTESIAN_POINT('Ctrl Pts',(-3.32947762189049,1.,2.52538321165774));
#62127=CARTESIAN_POINT('Ctrl Pts',(-3.32179931079521,-1.,2.52383598396878));
#62128=CARTESIAN_POINT('Ctrl Pts',(-3.32179931079521,1.,2.52383598396878));
#62129=CARTESIAN_POINT('Ctrl Pts',(-3.31413607874727,-1.,2.52225724871375));
#62130=CARTESIAN_POINT('Ctrl Pts',(-3.31413607874727,1.,2.52225724871375));
#62131=CARTESIAN_POINT('Ctrl Pts',(-3.30648808814986,-1.,2.52064689568167));
#62132=CARTESIAN_POINT('Ctrl Pts',(-3.30648808814986,1.,2.52064689568167));
#62133=CARTESIAN_POINT('Ctrl Pts',(-3.29885556387661,-1.,2.51900480700548));
#62134=CARTESIAN_POINT('Ctrl Pts',(-3.29885556387661,1.,2.51900480700548));
#62135=CARTESIAN_POINT('Ctrl Pts',(-3.2912387729863,-1.,2.51733085123316));
#62136=CARTESIAN_POINT('Ctrl Pts',(-3.2912387729863,1.,2.51733085123316));
#62137=CARTESIAN_POINT('Ctrl Pts',(-3.28363799702583,-1.,2.51562487464215));
#62138=CARTESIAN_POINT('Ctrl Pts',(-3.28363799702583,1.,2.51562487464215));
#62139=CARTESIAN_POINT('Ctrl Pts',(-3.27605350473048,-1.,2.51388669270329));
#62140=CARTESIAN_POINT('Ctrl Pts',(-3.27605350473048,1.,2.51388669270329));
#62141=CARTESIAN_POINT('Ctrl Pts',(-3.26848552888271,-1.,2.51211608411539));
#62142=CARTESIAN_POINT('Ctrl Pts',(-3.26848552888271,1.,2.51211608411539));
#62143=CARTESIAN_POINT('Ctrl Pts',(-3.26093423001716,-1.,2.51031277813697));
#62144=CARTESIAN_POINT('Ctrl Pts',(-3.26093423001716,1.,2.51031277813697));
#62145=CARTESIAN_POINT('Ctrl Pts',(-3.25339971461265,-1.,2.50847647070936));
#62146=CARTESIAN_POINT('Ctrl Pts',(-3.25339971461265,1.,2.50847647070936));
#62147=CARTESIAN_POINT('Ctrl Pts',(-3.24588208984042,-1.,2.50660685940645));
#62148=CARTESIAN_POINT('Ctrl Pts',(-3.24588208984042,1.,2.50660685940645));
#62149=CARTESIAN_POINT('Ctrl Pts',(-3.23838151080383,-1.,2.50470367580078));
#62150=CARTESIAN_POINT('Ctrl Pts',(-3.23838151080383,1.,2.50470367580078));
#62151=CARTESIAN_POINT('Ctrl Pts',(-3.23089822320596,-1.,2.50276671338074));
#62152=CARTESIAN_POINT('Ctrl Pts',(-3.23089822320596,1.,2.50276671338074));
#62153=CARTESIAN_POINT('Ctrl Pts',(-3.22343262620387,-1.,2.5007958720187));
#62154=CARTESIAN_POINT('Ctrl Pts',(-3.22343262620387,1.,2.5007958720187));
#62155=CARTESIAN_POINT('Ctrl Pts',(-3.21598526261157,-1.,2.49879114599293));
#62156=CARTESIAN_POINT('Ctrl Pts',(-3.21598526261157,1.,2.49879114599293));
#62157=CARTESIAN_POINT('Ctrl Pts',(-3.2085566984974,-1.,2.49675252647298));
#62158=CARTESIAN_POINT('Ctrl Pts',(-3.2085566984974,1.,2.49675252647298));
#62159=CARTESIAN_POINT('Ctrl Pts',(-3.20114742397549,-1.,2.49467992057726));
#62160=CARTESIAN_POINT('Ctrl Pts',(-3.20114742397549,1.,2.49467992057726));
#62161=CARTESIAN_POINT('Ctrl Pts',(-3.19375775555814,-1.,2.4925730723986));
#62162=CARTESIAN_POINT('Ctrl Pts',(-3.19375775555814,1.,2.4925730723986));
#62163=CARTESIAN_POINT('Ctrl Pts',(-3.18638771282315,-1.,2.49043146334095));
#62164=CARTESIAN_POINT('Ctrl Pts',(-3.18638771282315,1.,2.49043146334095));
#62165=CARTESIAN_POINT('Ctrl Pts',(-3.17903698136679,-1.,2.48825428288243));
#62166=CARTESIAN_POINT('Ctrl Pts',(-3.17903698136679,1.,2.48825428288243));
#62167=CARTESIAN_POINT('Ctrl Pts',(-3.17170518863357,-1.,2.48604065348619));
#62168=CARTESIAN_POINT('Ctrl Pts',(-3.17170518863357,1.,2.48604065348619));
#62169=CARTESIAN_POINT('Ctrl Pts',(-3.16439213290181,-1.,2.48378981792739));
#62170=CARTESIAN_POINT('Ctrl Pts',(-3.16439213290181,1.,2.48378981792739));
#62171=CARTESIAN_POINT('Ctrl Pts',(-3.15709802322735,-1.,2.48150133566568));
#62172=CARTESIAN_POINT('Ctrl Pts',(-3.15709802322735,1.,2.48150133566568));
#62173=CARTESIAN_POINT('Ctrl Pts',(-3.14982373241335,-1.,2.47917529057016));
#62174=CARTESIAN_POINT('Ctrl Pts',(-3.14982373241335,1.,2.47917529057016));
#62175=CARTESIAN_POINT('Ctrl Pts',(-3.14257099546531,-1.,2.47681245356095));
#62176=CARTESIAN_POINT('Ctrl Pts',(-3.14257099546531,1.,2.47681245356095));
#62177=CARTESIAN_POINT('Ctrl Pts',(-3.13534181229282,-1.,2.47441378371923));
#62178=CARTESIAN_POINT('Ctrl Pts',(-3.13534181229282,1.,2.47441378371923));
#62179=CARTESIAN_POINT('Ctrl Pts',(-3.12813790805948,-1.,2.47197997765868));
#62180=CARTESIAN_POINT('Ctrl Pts',(-3.12813790805948,1.,2.47197997765868));
#62181=CARTESIAN_POINT('Ctrl Pts',(-3.12096015766984,-1.,2.4695109894747));
#62182=CARTESIAN_POINT('Ctrl Pts',(-3.12096015766984,1.,2.4695109894747));
#62183=CARTESIAN_POINT('Ctrl Pts',(-3.11380805536124,-1.,2.46700558843507));
#62184=CARTESIAN_POINT('Ctrl Pts',(-3.11380805536124,1.,2.46700558843507));
#62185=CARTESIAN_POINT('Ctrl Pts',(-3.10667907901981,-1.,2.46446082979645));
#62186=CARTESIAN_POINT('Ctrl Pts',(-3.10667907901981,1.,2.46446082979645));
#62187=CARTESIAN_POINT('Ctrl Pts',(-3.09956993697048,-1.,2.4618730850188));
#62188=CARTESIAN_POINT('Ctrl Pts',(-3.09956993697048,1.,2.4618730850188));
#62189=CARTESIAN_POINT('Ctrl Pts',(-3.09247787931881,-1.,2.45923912563875));
#62190=CARTESIAN_POINT('Ctrl Pts',(-3.09247787931881,1.,2.45923912563875));
#62191=CARTESIAN_POINT('Ctrl Pts',(-3.08540206545313,-1.,2.45655725437037));
#62192=CARTESIAN_POINT('Ctrl Pts',(-3.08540206545313,1.,2.45655725437037));
#62193=CARTESIAN_POINT('Ctrl Pts',(-3.07834472886145,-1.,2.45382826787795));
#62194=CARTESIAN_POINT('Ctrl Pts',(-3.07834472886145,1.,2.45382826787795));
#62195=CARTESIAN_POINT('Ctrl Pts',(-3.0713129052131,-1.,2.45105688854432));
#62196=CARTESIAN_POINT('Ctrl Pts',(-3.0713129052131,1.,2.45105688854432));
#62197=CARTESIAN_POINT('Ctrl Pts',(-3.06431596421422,-1.,2.44824970516558));
#62198=CARTESIAN_POINT('Ctrl Pts',(-3.06431596421422,1.,2.44824970516558));
#62199=CARTESIAN_POINT('Ctrl Pts',(-3.05736242671521,-1.,2.44541251892568));
#62200=CARTESIAN_POINT('Ctrl Pts',(-3.05736242671521,1.,2.44541251892568));
#62201=CARTESIAN_POINT('Ctrl Pts',(-3.05045678021509,-1.,2.44254768923109));
#62202=CARTESIAN_POINT('Ctrl Pts',(-3.05045678021509,1.,2.44254768923109));
#62203=CARTESIAN_POINT('Ctrl Pts',(-3.04359685040545,-1.,2.43965194061849));
#62204=CARTESIAN_POINT('Ctrl Pts',(-3.04359685040545,1.,2.43965194061849));
#62205=CARTESIAN_POINT('Ctrl Pts',(-3.03676949672797,-1.,2.43671278042394));
#62206=CARTESIAN_POINT('Ctrl Pts',(-3.03676949672797,1.,2.43671278042394));
#62207=CARTESIAN_POINT('Ctrl Pts',(-3.02995534946946,-1.,2.43371241361462));
#62208=CARTESIAN_POINT('Ctrl Pts',(-3.02995534946946,1.,2.43371241361462));
#62209=CARTESIAN_POINT('Ctrl Pts',(-3.02313656035977,-1.,2.43063415586615));
#62210=CARTESIAN_POINT('Ctrl Pts',(-3.02313656035977,1.,2.43063415586615));
#62211=CARTESIAN_POINT('Ctrl Pts',(-3.01630420830494,-1.,2.4274685626416));
#62212=CARTESIAN_POINT('Ctrl Pts',(-3.01630420830494,1.,2.4274685626416));
#62213=CARTESIAN_POINT('Ctrl Pts',(-3.00946442616674,-1.,2.42421849439625));
#62214=CARTESIAN_POINT('Ctrl Pts',(-3.00946442616674,1.,2.42421849439625));
#62215=CARTESIAN_POINT('Ctrl Pts',(-3.00264868586038,-1.,2.42090763946812));
#62216=CARTESIAN_POINT('Ctrl Pts',(-3.00264868586038,1.,2.42090763946812));
#62217=CARTESIAN_POINT('Ctrl Pts',(-2.99590509293561,-1.,2.4175732450056));
#62218=CARTESIAN_POINT('Ctrl Pts',(-2.99590509293561,1.,2.4175732450056));
#62219=CARTESIAN_POINT('Ctrl Pts',(-2.98927983005851,-1.,2.4142506419963));
#62220=CARTESIAN_POINT('Ctrl Pts',(-2.98927983005851,1.,2.4142506419963));
#62221=CARTESIAN_POINT('Ctrl Pts',(-2.98280015815132,-1.,2.41095909342591));
#62222=CARTESIAN_POINT('Ctrl Pts',(-2.98280015815132,1.,2.41095909342591));
#62223=CARTESIAN_POINT('Ctrl Pts',(-2.97646002822395,-1.,2.40768975073691));
#62224=CARTESIAN_POINT('Ctrl Pts',(-2.97646002822395,1.,2.40768975073691));
#62225=CARTESIAN_POINT('Ctrl Pts',(-2.97019641312272,-1.,2.40438604734848));
#62226=CARTESIAN_POINT('Ctrl Pts',(-2.97019641312272,1.,2.40438604734848));
#62227=CARTESIAN_POINT('Ctrl Pts',(-2.96390432240181,-1.,2.40095565711535));
#62228=CARTESIAN_POINT('Ctrl Pts',(-2.96390432240181,1.,2.40095565711535));
#62229=CARTESIAN_POINT('Ctrl Pts',(-2.95748006482811,-1.,2.39730553974412));
#62230=CARTESIAN_POINT('Ctrl Pts',(-2.95748006482811,1.,2.39730553974412));
#62231=CARTESIAN_POINT('Ctrl Pts',(-2.95085857128372,-1.,2.39337207631613));
#62232=CARTESIAN_POINT('Ctrl Pts',(-2.95085857128372,1.,2.39337207631613));
#62233=CARTESIAN_POINT('Ctrl Pts',(-2.94404820669135,-1.,2.38914929090806));
#62234=CARTESIAN_POINT('Ctrl Pts',(-2.94404820669135,1.,2.38914929090806));
#62235=CARTESIAN_POINT('Ctrl Pts',(-2.93717903280599,-1.,2.38472771516476));
#62236=CARTESIAN_POINT('Ctrl Pts',(-2.93717903280599,1.,2.38472771516476));
#62237=CARTESIAN_POINT('Ctrl Pts',(-2.93049643640517,-1.,2.3802898958232));
#62238=CARTESIAN_POINT('Ctrl Pts',(-2.93049643640517,1.,2.3802898958232));
#62239=CARTESIAN_POINT('Ctrl Pts',(-2.92430340582912,-1.,2.37606510524271));
#62240=CARTESIAN_POINT('Ctrl Pts',(-2.92430340582912,1.,2.37606510524271));
#62241=CARTESIAN_POINT('Ctrl Pts',(-2.9189150379156,-1.,2.37229381109939));
#62242=CARTESIAN_POINT('Ctrl Pts',(-2.9189150379156,1.,2.37229381109939));
#62243=CARTESIAN_POINT('Ctrl Pts',(-2.91461249883016,-1.,2.36919161373074));
#62244=CARTESIAN_POINT('Ctrl Pts',(-2.91461249883016,1.,2.36919161373074));
#62245=CARTESIAN_POINT('Ctrl Pts',(-2.9115863784165,-1.,2.36690501170317));
#62246=CARTESIAN_POINT('Ctrl Pts',(-2.9115863784165,1.,2.36690501170317));
#62247=CARTESIAN_POINT('Ctrl Pts',(-2.91025813829606,-1.,2.36578327194396));
#62248=CARTESIAN_POINT('Ctrl Pts',(-2.91025813829606,1.,2.36578327194396));
#62249=CARTESIAN_POINT('Ctrl Pts',(-2.90989022547738,-1.,2.36535052956704));
#62250=CARTESIAN_POINT('Ctrl Pts',(-2.90989022547738,1.,2.36535052956704));
#62251=CARTESIAN_POINT('Ctrl Pts',(-2.90992398626098,-1.,2.36524348105023));
#62252=CARTESIAN_POINT('Ctrl Pts',(-2.90992398626098,1.,2.36524348105023));
#62253=CARTESIAN_POINT('Ctrl Pts',(-2.91001063062876,-1.,2.36523532225181));
#62254=CARTESIAN_POINT('Ctrl Pts',(-2.91001063062876,1.,2.36523532225181));
#62255=CARTESIAN_POINT('',(-3.35260583073571,1.,2.52982887637028));
#62256=CARTESIAN_POINT('Ctrl Pts',(-3.35260583073571,1.,2.52982887637028));
#62257=CARTESIAN_POINT('Ctrl Pts',(-3.35105973714426,1.,2.52954136549357));
#62258=CARTESIAN_POINT('Ctrl Pts',(-3.34796903577628,1.,2.5289632161143));
#62259=CARTESIAN_POINT('Ctrl Pts',(-3.34333744117093,1.,2.52808660916879));
#62260=CARTESIAN_POINT('Ctrl Pts',(-3.33717090000955,1.,2.52689902691551));
#62261=CARTESIAN_POINT('Ctrl Pts',(-3.32947762189049,1.,2.52538321165774));
#62262=CARTESIAN_POINT('Ctrl Pts',(-3.32179931079521,1.,2.52383598396878));
#62263=CARTESIAN_POINT('Ctrl Pts',(-3.31413607874727,1.,2.52225724871375));
#62264=CARTESIAN_POINT('Ctrl Pts',(-3.30648808814986,1.,2.52064689568167));
#62265=CARTESIAN_POINT('Ctrl Pts',(-3.29885556387661,1.,2.51900480700548));
#62266=CARTESIAN_POINT('Ctrl Pts',(-3.2912387729863,1.,2.51733085123316));
#62267=CARTESIAN_POINT('Ctrl Pts',(-3.28363799702583,1.,2.51562487464215));
#62268=CARTESIAN_POINT('Ctrl Pts',(-3.27605350473048,1.,2.51388669270329));
#62269=CARTESIAN_POINT('Ctrl Pts',(-3.26848552888271,1.,2.51211608411539));
#62270=CARTESIAN_POINT('Ctrl Pts',(-3.26093423001716,1.,2.51031277813697));
#62271=CARTESIAN_POINT('Ctrl Pts',(-3.25339971461265,1.,2.50847647070936));
#62272=CARTESIAN_POINT('Ctrl Pts',(-3.24588208984042,1.,2.50660685940645));
#62273=CARTESIAN_POINT('Ctrl Pts',(-3.23838151080383,1.,2.50470367580078));
#62274=CARTESIAN_POINT('Ctrl Pts',(-3.23089822320596,1.,2.50276671338074));
#62275=CARTESIAN_POINT('Ctrl Pts',(-3.22343262620387,1.,2.5007958720187));
#62276=CARTESIAN_POINT('Ctrl Pts',(-3.21598526261157,1.,2.49879114599293));
#62277=CARTESIAN_POINT('Ctrl Pts',(-3.2085566984974,1.,2.49675252647298));
#62278=CARTESIAN_POINT('Ctrl Pts',(-3.20114742397549,1.,2.49467992057726));
#62279=CARTESIAN_POINT('Ctrl Pts',(-3.19375775555814,1.,2.4925730723986));
#62280=CARTESIAN_POINT('Ctrl Pts',(-3.18638771282315,1.,2.49043146334095));
#62281=CARTESIAN_POINT('Ctrl Pts',(-3.17903698136679,1.,2.48825428288243));
#62282=CARTESIAN_POINT('Ctrl Pts',(-3.17170518863357,1.,2.48604065348619));
#62283=CARTESIAN_POINT('Ctrl Pts',(-3.16439213290181,1.,2.48378981792739));
#62284=CARTESIAN_POINT('Ctrl Pts',(-3.15709802322735,1.,2.48150133566568));
#62285=CARTESIAN_POINT('Ctrl Pts',(-3.14982373241335,1.,2.47917529057016));
#62286=CARTESIAN_POINT('Ctrl Pts',(-3.14257099546531,1.,2.47681245356095));
#62287=CARTESIAN_POINT('Ctrl Pts',(-3.13534181229282,1.,2.47441378371923));
#62288=CARTESIAN_POINT('Ctrl Pts',(-3.12813790805948,1.,2.47197997765868));
#62289=CARTESIAN_POINT('Ctrl Pts',(-3.12096015766984,1.,2.4695109894747));
#62290=CARTESIAN_POINT('Ctrl Pts',(-3.11380805536124,1.,2.46700558843507));
#62291=CARTESIAN_POINT('Ctrl Pts',(-3.10667907901981,1.,2.46446082979645));
#62292=CARTESIAN_POINT('Ctrl Pts',(-3.09956993697048,1.,2.4618730850188));
#62293=CARTESIAN_POINT('Ctrl Pts',(-3.09247787931881,1.,2.45923912563875));
#62294=CARTESIAN_POINT('Ctrl Pts',(-3.08540206545313,1.,2.45655725437037));
#62295=CARTESIAN_POINT('Ctrl Pts',(-3.07834472886145,1.,2.45382826787795));
#62296=CARTESIAN_POINT('Ctrl Pts',(-3.0713129052131,1.,2.45105688854432));
#62297=CARTESIAN_POINT('Ctrl Pts',(-3.06431596421422,1.,2.44824970516558));
#62298=CARTESIAN_POINT('Ctrl Pts',(-3.05736242671521,1.,2.44541251892568));
#62299=CARTESIAN_POINT('Ctrl Pts',(-3.05045678021509,1.,2.44254768923109));
#62300=CARTESIAN_POINT('Ctrl Pts',(-3.04359685040545,1.,2.43965194061849));
#62301=CARTESIAN_POINT('Ctrl Pts',(-3.03676949672797,1.,2.43671278042394));
#62302=CARTESIAN_POINT('Ctrl Pts',(-3.02995534946946,1.,2.43371241361462));
#62303=CARTESIAN_POINT('Ctrl Pts',(-3.02313656035977,1.,2.43063415586615));
#62304=CARTESIAN_POINT('Ctrl Pts',(-3.01630420830494,1.,2.4274685626416));
#62305=CARTESIAN_POINT('Ctrl Pts',(-3.00946442616674,1.,2.42421849439625));
#62306=CARTESIAN_POINT('Ctrl Pts',(-3.00264868586038,1.,2.42090763946812));
#62307=CARTESIAN_POINT('Ctrl Pts',(-2.99590509293561,1.,2.4175732450056));
#62308=CARTESIAN_POINT('Ctrl Pts',(-2.98927983005851,1.,2.4142506419963));
#62309=CARTESIAN_POINT('Ctrl Pts',(-2.98280015815132,1.,2.41095909342591));
#62310=CARTESIAN_POINT('Ctrl Pts',(-2.97646002822395,1.,2.40768975073691));
#62311=CARTESIAN_POINT('Ctrl Pts',(-2.97019641312272,1.,2.40438604734848));
#62312=CARTESIAN_POINT('Ctrl Pts',(-2.96390432240181,1.,2.40095565711535));
#62313=CARTESIAN_POINT('Ctrl Pts',(-2.95748006482811,1.,2.39730553974412));
#62314=CARTESIAN_POINT('Ctrl Pts',(-2.95085857128372,1.,2.39337207631613));
#62315=CARTESIAN_POINT('Ctrl Pts',(-2.94404820669135,1.,2.38914929090806));
#62316=CARTESIAN_POINT('Ctrl Pts',(-2.93717903280599,1.,2.38472771516476));
#62317=CARTESIAN_POINT('Ctrl Pts',(-2.93049643640517,1.,2.3802898958232));
#62318=CARTESIAN_POINT('Ctrl Pts',(-2.92430340582912,1.,2.37606510524271));
#62319=CARTESIAN_POINT('Ctrl Pts',(-2.9189150379156,1.,2.37229381109939));
#62320=CARTESIAN_POINT('Ctrl Pts',(-2.91461249883016,1.,2.36919161373074));
#62321=CARTESIAN_POINT('Ctrl Pts',(-2.91181344022628,1.,2.36707658451709));
#62322=CARTESIAN_POINT('Ctrl Pts',(-2.91051690822262,1.,2.36599991765853));
#62323=CARTESIAN_POINT('Ctrl Pts',(-2.9100577052777,1.,2.36553202948741));
#62324=CARTESIAN_POINT('Ctrl Pts',(-2.90995756655559,1.,2.3653621118858));
#62325=CARTESIAN_POINT('Ctrl Pts',(-2.90994629141563,1.,2.36531447826213));
#62326=CARTESIAN_POINT('',(-3.35260583073571,0.,2.52982887637028));
#62327=CARTESIAN_POINT('Ctrl Pts',(-3.1487152044751,-1.,2.03668666247593));
#62328=CARTESIAN_POINT('Ctrl Pts',(-3.1487152044751,1.,2.03668666247593));
#62329=CARTESIAN_POINT('Ctrl Pts',(-3.14869618937258,-1.,2.03660173757879));
#62330=CARTESIAN_POINT('Ctrl Pts',(-3.14869618937258,1.,2.03660173757879));
#62331=CARTESIAN_POINT('Ctrl Pts',(-3.14878756590812,-1.,2.03653654935592));
#62332=CARTESIAN_POINT('Ctrl Pts',(-3.14878756590812,1.,2.03653654935592));
#62333=CARTESIAN_POINT('Ctrl Pts',(-3.14931281968048,-1.,2.03675273049189));
#62334=CARTESIAN_POINT('Ctrl Pts',(-3.14931281968048,1.,2.03675273049189));
#62335=CARTESIAN_POINT('Ctrl Pts',(-3.15079010635742,-1.,2.03766932526445));
#62336=CARTESIAN_POINT('Ctrl Pts',(-3.15079010635742,1.,2.03766932526445));
#62337=CARTESIAN_POINT('Ctrl Pts',(-3.15389991674792,-1.,2.03984073791519));
#62338=CARTESIAN_POINT('Ctrl Pts',(-3.15389991674792,1.,2.03984073791519));
#62339=CARTESIAN_POINT('Ctrl Pts',(-3.15817983946367,-1.,2.04297406404027));
#62340=CARTESIAN_POINT('Ctrl Pts',(-3.15817983946367,1.,2.04297406404027));
#62341=CARTESIAN_POINT('Ctrl Pts',(-3.16343165058912,-1.,2.04693331247446));
#62342=CARTESIAN_POINT('Ctrl Pts',(-3.16343165058912,1.,2.04693331247446));
#62343=CARTESIAN_POINT('Ctrl Pts',(-3.16936341689527,-1.,2.05151770247233));
#62344=CARTESIAN_POINT('Ctrl Pts',(-3.16936341689527,1.,2.05151770247233));
#62345=CARTESIAN_POINT('Ctrl Pts',(-3.17564906975371,-1.,2.05650186773132));
#62346=CARTESIAN_POINT('Ctrl Pts',(-3.17564906975371,1.,2.05650186773132));
#62347=CARTESIAN_POINT('Ctrl Pts',(-3.18197692964614,-1.,2.06166849827101));
#62348=CARTESIAN_POINT('Ctrl Pts',(-3.18197692964614,1.,2.06166849827101));
#62349=CARTESIAN_POINT('Ctrl Pts',(-3.18809755562368,-1.,2.06684062744112));
#62350=CARTESIAN_POINT('Ctrl Pts',(-3.18809755562368,1.,2.06684062744112));
#62351=CARTESIAN_POINT('Ctrl Pts',(-3.19388465568252,-1.,2.07192253497857));
#62352=CARTESIAN_POINT('Ctrl Pts',(-3.19388465568252,1.,2.07192253497857));
#62353=CARTESIAN_POINT('Ctrl Pts',(-3.19934132836019,-1.,2.07690441870722));
#62354=CARTESIAN_POINT('Ctrl Pts',(-3.19934132836019,1.,2.07690441870722));
#62355=CARTESIAN_POINT('Ctrl Pts',(-3.2045481863073,-1.,2.08182850370878));
#62356=CARTESIAN_POINT('Ctrl Pts',(-3.2045481863073,1.,2.08182850370878));
#62357=CARTESIAN_POINT('Ctrl Pts',(-3.20962575845463,-1.,2.08676465517455));
#62358=CARTESIAN_POINT('Ctrl Pts',(-3.20962575845463,1.,2.08676465517455));
#62359=CARTESIAN_POINT('Ctrl Pts',(-3.21469429601654,-1.,2.09178419460443));
#62360=CARTESIAN_POINT('Ctrl Pts',(-3.21469429601654,1.,2.09178419460443));
#62361=CARTESIAN_POINT('Ctrl Pts',(-3.21982707347009,-1.,2.09692958434895));
#62362=CARTESIAN_POINT('Ctrl Pts',(-3.21982707347009,1.,2.09692958434895));
#62363=CARTESIAN_POINT('Ctrl Pts',(-3.22503437553434,-1.,2.10220384298492));
#62364=CARTESIAN_POINT('Ctrl Pts',(-3.22503437553434,1.,2.10220384298492));
#62365=CARTESIAN_POINT('Ctrl Pts',(-3.23028945793289,-1.,2.10758699642451));
#62366=CARTESIAN_POINT('Ctrl Pts',(-3.23028945793289,1.,2.10758699642451));
#62367=CARTESIAN_POINT('Ctrl Pts',(-3.23554444767099,-1.,2.11304604021773));
#62368=CARTESIAN_POINT('Ctrl Pts',(-3.23554444767099,1.,2.11304604021773));
#62369=CARTESIAN_POINT('Ctrl Pts',(-3.24074905517293,-1.,2.11854673326979));
#62370=CARTESIAN_POINT('Ctrl Pts',(-3.24074905517293,1.,2.11854673326979));
#62371=CARTESIAN_POINT('Ctrl Pts',(-3.24587102613376,-1.,2.12406646410962));
#62372=CARTESIAN_POINT('Ctrl Pts',(-3.24587102613376,1.,2.12406646410962));
#62373=CARTESIAN_POINT('Ctrl Pts',(-3.25090574494028,-1.,2.12960028396832));
#62374=CARTESIAN_POINT('Ctrl Pts',(-3.25090574494028,1.,2.12960028396832));
#62375=CARTESIAN_POINT('Ctrl Pts',(-3.25586495065054,-1.,2.13515375878803));
#62376=CARTESIAN_POINT('Ctrl Pts',(-3.25586495065054,1.,2.13515375878803));
#62377=CARTESIAN_POINT('Ctrl Pts',(-3.26077002641879,-1.,2.14073870754264));
#62378=CARTESIAN_POINT('Ctrl Pts',(-3.26077002641879,1.,2.14073870754264));
#62379=CARTESIAN_POINT('Ctrl Pts',(-3.26564388189759,-1.,2.1463680529566));
#62380=CARTESIAN_POINT('Ctrl Pts',(-3.26564388189759,1.,2.1463680529566));
#62381=CARTESIAN_POINT('Ctrl Pts',(-3.27050245897228,-1.,2.15205043199808));
#62382=CARTESIAN_POINT('Ctrl Pts',(-3.27050245897228,1.,2.15205043199808));
#62383=CARTESIAN_POINT('Ctrl Pts',(-3.27534954469187,-1.,2.15778690038347));
#62384=CARTESIAN_POINT('Ctrl Pts',(-3.27534954469187,1.,2.15778690038347));
#62385=CARTESIAN_POINT('Ctrl Pts',(-3.280181508414,-1.,2.16357391934425));
#62386=CARTESIAN_POINT('Ctrl Pts',(-3.280181508414,1.,2.16357391934425));
#62387=CARTESIAN_POINT('Ctrl Pts',(-3.28499019979724,-1.,2.16940517773455));
#62388=CARTESIAN_POINT('Ctrl Pts',(-3.28499019979724,1.,2.16940517773455));
#62389=CARTESIAN_POINT('Ctrl Pts',(-3.28976645712568,-1.,2.17527380048423));
#62390=CARTESIAN_POINT('Ctrl Pts',(-3.28976645712568,1.,2.17527380048423));
#62391=CARTESIAN_POINT('Ctrl Pts',(-3.2945036150049,-1.,2.18117455557065));
#62392=CARTESIAN_POINT('Ctrl Pts',(-3.2945036150049,1.,2.18117455557065));
#62393=CARTESIAN_POINT('Ctrl Pts',(-3.29920022557639,-1.,2.18710556500327));
#62394=CARTESIAN_POINT('Ctrl Pts',(-3.29920022557639,1.,2.18710556500327));
#62395=CARTESIAN_POINT('Ctrl Pts',(-3.30385816281831,-1.,2.19306710376111));
#62396=CARTESIAN_POINT('Ctrl Pts',(-3.30385816281831,1.,2.19306710376111));
#62397=CARTESIAN_POINT('Ctrl Pts',(-3.30848134694595,-1.,2.19906078949923));
#62398=CARTESIAN_POINT('Ctrl Pts',(-3.30848134694595,1.,2.19906078949923));
#62399=CARTESIAN_POINT('Ctrl Pts',(-3.31307424608949,-1.,2.20508863150607));
#62400=CARTESIAN_POINT('Ctrl Pts',(-3.31307424608949,1.,2.20508863150607));
#62401=CARTESIAN_POINT('Ctrl Pts',(-3.31764044024235,-1.,2.21115211847875));
#62402=CARTESIAN_POINT('Ctrl Pts',(-3.31764044024235,1.,2.21115211847875));
#62403=CARTESIAN_POINT('Ctrl Pts',(-3.32218125618968,-1.,2.21725135110898));
#62404=CARTESIAN_POINT('Ctrl Pts',(-3.32218125618968,1.,2.21725135110898));
#62405=CARTESIAN_POINT('Ctrl Pts',(-3.3266964672289,-1.,2.22338548312772));
#62406=CARTESIAN_POINT('Ctrl Pts',(-3.3266964672289,1.,2.22338548312772));
#62407=CARTESIAN_POINT('Ctrl Pts',(-3.33118487773611,-1.,2.22955308907233));
#62408=CARTESIAN_POINT('Ctrl Pts',(-3.33118487773611,1.,2.22955308907233));
#62409=CARTESIAN_POINT('Ctrl Pts',(-3.33564495756482,-1.,2.23575256328812));
#62410=CARTESIAN_POINT('Ctrl Pts',(-3.33564495756482,1.,2.23575256328812));
#62411=CARTESIAN_POINT('Ctrl Pts',(-3.34007543738025,-1.,2.24198249391422));
#62412=CARTESIAN_POINT('Ctrl Pts',(-3.34007543738025,1.,2.24198249391422));
#62413=CARTESIAN_POINT('Ctrl Pts',(-3.34447596770723,-1.,2.24824207678256));
#62414=CARTESIAN_POINT('Ctrl Pts',(-3.34447596770723,1.,2.24824207678256));
#62415=CARTESIAN_POINT('Ctrl Pts',(-3.34884690292285,-1.,2.25453097693483));
#62416=CARTESIAN_POINT('Ctrl Pts',(-3.34884690292285,1.,2.25453097693483));
#62417=CARTESIAN_POINT('Ctrl Pts',(-3.35318902552626,-1.,2.26084915222449));
#62418=CARTESIAN_POINT('Ctrl Pts',(-3.35318902552626,1.,2.26084915222449));
#62419=CARTESIAN_POINT('Ctrl Pts',(-3.35750328523061,-1.,2.2671966857991));
#62420=CARTESIAN_POINT('Ctrl Pts',(-3.35750328523061,1.,2.2671966857991));
#62421=CARTESIAN_POINT('Ctrl Pts',(-3.36179055004409,-1.,2.2735736262093));
#62422=CARTESIAN_POINT('Ctrl Pts',(-3.36179055004409,1.,2.2735736262093));
#62423=CARTESIAN_POINT('Ctrl Pts',(-3.36605130713076,-1.,2.27997979458037));
#62424=CARTESIAN_POINT('Ctrl Pts',(-3.36605130713076,1.,2.27997979458037));
#62425=CARTESIAN_POINT('Ctrl Pts',(-3.37028570206488,-1.,2.28641481081137));
#62426=CARTESIAN_POINT('Ctrl Pts',(-3.37028570206488,1.,2.28641481081137));
#62427=CARTESIAN_POINT('Ctrl Pts',(-3.37449367172826,-1.,2.29287818007393));
#62428=CARTESIAN_POINT('Ctrl Pts',(-3.37449367172826,1.,2.29287818007393));
#62429=CARTESIAN_POINT('Ctrl Pts',(-3.37867504959433,-1.,2.29936936127624));
#62430=CARTESIAN_POINT('Ctrl Pts',(-3.37867504959433,1.,2.29936936127624));
#62431=CARTESIAN_POINT('Ctrl Pts',(-3.3828296733661,-1.,2.30588783640343));
#62432=CARTESIAN_POINT('Ctrl Pts',(-3.3828296733661,1.,2.30588783640343));
#62433=CARTESIAN_POINT('Ctrl Pts',(-3.38695751492462,-1.,2.31243319489367));
#62434=CARTESIAN_POINT('Ctrl Pts',(-3.38695751492462,1.,2.31243319489367));
#62435=CARTESIAN_POINT('Ctrl Pts',(-3.39105869474822,-1.,2.31900513925424));
#62436=CARTESIAN_POINT('Ctrl Pts',(-3.39105869474822,1.,2.31900513925424));
#62437=CARTESIAN_POINT('Ctrl Pts',(-3.39513342019756,-1.,2.3256034390248));
#62438=CARTESIAN_POINT('Ctrl Pts',(-3.39513342019756,1.,2.3256034390248));
#62439=CARTESIAN_POINT('Ctrl Pts',(-3.39918194577956,-1.,2.33222789882489));
#62440=CARTESIAN_POINT('Ctrl Pts',(-3.39918194577956,1.,2.33222789882489));
#62441=CARTESIAN_POINT('Ctrl Pts',(-3.40320452776743,-1.,2.33887832342782));
#62442=CARTESIAN_POINT('Ctrl Pts',(-3.40320452776743,1.,2.33887832342782));
#62443=CARTESIAN_POINT('Ctrl Pts',(-3.40720137404297,-1.,2.34555447649188));
#62444=CARTESIAN_POINT('Ctrl Pts',(-3.40720137404297,1.,2.34555447649188));
#62445=CARTESIAN_POINT('Ctrl Pts',(-3.41117262314119,-1.,2.35225606824109));
#62446=CARTESIAN_POINT('Ctrl Pts',(-3.41117262314119,1.,2.35225606824109));
#62447=CARTESIAN_POINT('Ctrl Pts',(-3.41511836751469,-1.,2.35898278606946));
#62448=CARTESIAN_POINT('Ctrl Pts',(-3.41511836751469,1.,2.35898278606946));
#62449=CARTESIAN_POINT('Ctrl Pts',(-3.41903866635852,-1.,2.36573431470642));
#62450=CARTESIAN_POINT('Ctrl Pts',(-3.41903866635852,1.,2.36573431470642));
#62451=CARTESIAN_POINT('Ctrl Pts',(-3.42293356216511,-1.,2.37251035954292));
#62452=CARTESIAN_POINT('Ctrl Pts',(-3.42293356216511,1.,2.37251035954292));
#62453=CARTESIAN_POINT('Ctrl Pts',(-3.42680309754399,-1.,2.37931067028926));
#62454=CARTESIAN_POINT('Ctrl Pts',(-3.42680309754399,1.,2.37931067028926));
#62455=CARTESIAN_POINT('Ctrl Pts',(-3.4306473271292,-1.,2.38613505843552));
#62456=CARTESIAN_POINT('Ctrl Pts',(-3.4306473271292,1.,2.38613505843552));
#62457=CARTESIAN_POINT('Ctrl Pts',(-3.4344663067854,-1.,2.39298338804493));
#62458=CARTESIAN_POINT('Ctrl Pts',(-3.4344663067854,1.,2.39298338804493));
#62459=CARTESIAN_POINT('Ctrl Pts',(-3.43750133064416,-1.,2.39848113410292));
#62460=CARTESIAN_POINT('Ctrl Pts',(-3.43750133064416,1.,2.39848113410292));
#62461=CARTESIAN_POINT('Ctrl Pts',(-3.43976627484234,-1.,2.40261515589405));
#62462=CARTESIAN_POINT('Ctrl Pts',(-3.43976627484234,1.,2.40261515589405));
#62463=CARTESIAN_POINT('Ctrl Pts',(-3.44127120683039,-1.,2.4053759295909));
#62464=CARTESIAN_POINT('Ctrl Pts',(-3.44127120683039,1.,2.4053759295909));
#62465=CARTESIAN_POINT('Ctrl Pts',(-3.44202241512147,-1.,2.40675750623143));
#62466=CARTESIAN_POINT('Ctrl Pts',(-3.44202241512147,1.,2.40675750623143));
#62467=CARTESIAN_POINT('',(-3.14877060440327,1.,2.03660101169715));
#62468=CARTESIAN_POINT('Ctrl Pts',(-3.14877060440327,-1.,2.03660101169715));
#62469=CARTESIAN_POINT('Ctrl Pts',(-3.14877060440327,-0.666666666666667,
2.03660101169715));
#62470=CARTESIAN_POINT('Ctrl Pts',(-3.14877060440327,-0.333333333333333,
2.03660101169715));
#62471=CARTESIAN_POINT('Ctrl Pts',(-3.14877060440327,0.333333333333333,
2.03660101169715));
#62472=CARTESIAN_POINT('Ctrl Pts',(-3.14877060440327,0.666666666666667,
2.03660101169715));
#62473=CARTESIAN_POINT('Ctrl Pts',(-3.14877060440327,1.,2.03660101169715));
#62474=CARTESIAN_POINT('',(-3.44202241512147,1.,2.40675750623143));
#62475=CARTESIAN_POINT('',(-3.44202241512147,0.,2.40675750623143));
#62476=CARTESIAN_POINT('Ctrl Pts',(-3.14877060440327,1.,2.03660101169715));
#62477=CARTESIAN_POINT('Ctrl Pts',(-3.14881939088124,1.,2.03659701539259));
#62478=CARTESIAN_POINT('Ctrl Pts',(-3.1490119366901,1.,2.03663974554932));
#62479=CARTESIAN_POINT('Ctrl Pts',(-3.14959882629805,1.,2.03693188810544));
#62480=CARTESIAN_POINT('Ctrl Pts',(-3.15102344775328,1.,2.03783225495961));
#62481=CARTESIAN_POINT('Ctrl Pts',(-3.15389991674792,1.,2.03984073791519));
#62482=CARTESIAN_POINT('Ctrl Pts',(-3.15817983946367,1.,2.04297406404027));
#62483=CARTESIAN_POINT('Ctrl Pts',(-3.16343165058912,1.,2.04693331247446));
#62484=CARTESIAN_POINT('Ctrl Pts',(-3.16936341689527,1.,2.05151770247233));
#62485=CARTESIAN_POINT('Ctrl Pts',(-3.17564906975371,1.,2.05650186773132));
#62486=CARTESIAN_POINT('Ctrl Pts',(-3.18197692964614,1.,2.06166849827101));
#62487=CARTESIAN_POINT('Ctrl Pts',(-3.18809755562368,1.,2.06684062744112));
#62488=CARTESIAN_POINT('Ctrl Pts',(-3.19388465568252,1.,2.07192253497857));
#62489=CARTESIAN_POINT('Ctrl Pts',(-3.19934132836019,1.,2.07690441870722));
#62490=CARTESIAN_POINT('Ctrl Pts',(-3.2045481863073,1.,2.08182850370878));
#62491=CARTESIAN_POINT('Ctrl Pts',(-3.20962575845463,1.,2.08676465517455));
#62492=CARTESIAN_POINT('Ctrl Pts',(-3.21469429601654,1.,2.09178419460443));
#62493=CARTESIAN_POINT('Ctrl Pts',(-3.21982707347009,1.,2.09692958434895));
#62494=CARTESIAN_POINT('Ctrl Pts',(-3.22503437553434,1.,2.10220384298492));
#62495=CARTESIAN_POINT('Ctrl Pts',(-3.23028945793289,1.,2.10758699642451));
#62496=CARTESIAN_POINT('Ctrl Pts',(-3.23554444767099,1.,2.11304604021773));
#62497=CARTESIAN_POINT('Ctrl Pts',(-3.24074905517293,1.,2.11854673326979));
#62498=CARTESIAN_POINT('Ctrl Pts',(-3.24587102613376,1.,2.12406646410962));
#62499=CARTESIAN_POINT('Ctrl Pts',(-3.25090574494028,1.,2.12960028396832));
#62500=CARTESIAN_POINT('Ctrl Pts',(-3.25586495065054,1.,2.13515375878803));
#62501=CARTESIAN_POINT('Ctrl Pts',(-3.26077002641879,1.,2.14073870754264));
#62502=CARTESIAN_POINT('Ctrl Pts',(-3.26564388189759,1.,2.1463680529566));
#62503=CARTESIAN_POINT('Ctrl Pts',(-3.27050245897228,1.,2.15205043199808));
#62504=CARTESIAN_POINT('Ctrl Pts',(-3.27534954469187,1.,2.15778690038347));
#62505=CARTESIAN_POINT('Ctrl Pts',(-3.280181508414,1.,2.16357391934425));
#62506=CARTESIAN_POINT('Ctrl Pts',(-3.28499019979724,1.,2.16940517773455));
#62507=CARTESIAN_POINT('Ctrl Pts',(-3.28976645712568,1.,2.17527380048423));
#62508=CARTESIAN_POINT('Ctrl Pts',(-3.2945036150049,1.,2.18117455557065));
#62509=CARTESIAN_POINT('Ctrl Pts',(-3.29920022557639,1.,2.18710556500327));
#62510=CARTESIAN_POINT('Ctrl Pts',(-3.30385816281831,1.,2.19306710376111));
#62511=CARTESIAN_POINT('Ctrl Pts',(-3.30848134694595,1.,2.19906078949923));
#62512=CARTESIAN_POINT('Ctrl Pts',(-3.31307424608949,1.,2.20508863150607));
#62513=CARTESIAN_POINT('Ctrl Pts',(-3.31764044024235,1.,2.21115211847875));
#62514=CARTESIAN_POINT('Ctrl Pts',(-3.32218125618968,1.,2.21725135110898));
#62515=CARTESIAN_POINT('Ctrl Pts',(-3.3266964672289,1.,2.22338548312772));
#62516=CARTESIAN_POINT('Ctrl Pts',(-3.33118487773611,1.,2.22955308907233));
#62517=CARTESIAN_POINT('Ctrl Pts',(-3.33564495756482,1.,2.23575256328812));
#62518=CARTESIAN_POINT('Ctrl Pts',(-3.34007543738025,1.,2.24198249391422));
#62519=CARTESIAN_POINT('Ctrl Pts',(-3.34447596770723,1.,2.24824207678256));
#62520=CARTESIAN_POINT('Ctrl Pts',(-3.34884690292285,1.,2.25453097693483));
#62521=CARTESIAN_POINT('Ctrl Pts',(-3.35318902552626,1.,2.26084915222449));
#62522=CARTESIAN_POINT('Ctrl Pts',(-3.35750328523061,1.,2.2671966857991));
#62523=CARTESIAN_POINT('Ctrl Pts',(-3.36179055004409,1.,2.2735736262093));
#62524=CARTESIAN_POINT('Ctrl Pts',(-3.36605130713076,1.,2.27997979458037));
#62525=CARTESIAN_POINT('Ctrl Pts',(-3.37028570206488,1.,2.28641481081137));
#62526=CARTESIAN_POINT('Ctrl Pts',(-3.37449367172826,1.,2.29287818007393));
#62527=CARTESIAN_POINT('Ctrl Pts',(-3.37867504959433,1.,2.29936936127624));
#62528=CARTESIAN_POINT('Ctrl Pts',(-3.3828296733661,1.,2.30588783640343));
#62529=CARTESIAN_POINT('Ctrl Pts',(-3.38695751492462,1.,2.31243319489367));
#62530=CARTESIAN_POINT('Ctrl Pts',(-3.39105869474822,1.,2.31900513925424));
#62531=CARTESIAN_POINT('Ctrl Pts',(-3.39513342019756,1.,2.3256034390248));
#62532=CARTESIAN_POINT('Ctrl Pts',(-3.39918194577956,1.,2.33222789882489));
#62533=CARTESIAN_POINT('Ctrl Pts',(-3.40320452776743,1.,2.33887832342782));
#62534=CARTESIAN_POINT('Ctrl Pts',(-3.40720137404297,1.,2.34555447649188));
#62535=CARTESIAN_POINT('Ctrl Pts',(-3.41117262314119,1.,2.35225606824109));
#62536=CARTESIAN_POINT('Ctrl Pts',(-3.41511836751469,1.,2.35898278606946));
#62537=CARTESIAN_POINT('Ctrl Pts',(-3.41903866635852,1.,2.36573431470642));
#62538=CARTESIAN_POINT('Ctrl Pts',(-3.42293356216511,1.,2.37251035954292));
#62539=CARTESIAN_POINT('Ctrl Pts',(-3.42680309754399,1.,2.37931067028926));
#62540=CARTESIAN_POINT('Ctrl Pts',(-3.4306473271292,1.,2.38613505843552));
#62541=CARTESIAN_POINT('Ctrl Pts',(-3.4344663067854,1.,2.39298338804493));
#62542=CARTESIAN_POINT('Ctrl Pts',(-3.43750133064416,1.,2.39848113410292));
#62543=CARTESIAN_POINT('Ctrl Pts',(-3.43976627484234,1.,2.40261515589405));
#62544=CARTESIAN_POINT('Ctrl Pts',(-3.44127120683039,1.,2.4053759295909));
#62545=CARTESIAN_POINT('Ctrl Pts',(-3.44202241512147,1.,2.40675750623143));
#62546=CARTESIAN_POINT('Origin',(-3.44202241512147,0.,2.40675750623143));
#62547=CARTESIAN_POINT('',(-3.35260583073571,1.,2.52982887637028));
#62548=CARTESIAN_POINT('Origin',(0.,0.,0.));
#62549=CARTESIAN_POINT('',(-3.24413672884812,1.,1.88097764062697));
#62550=CARTESIAN_POINT('Origin',(0.,1.,0.));
#62551=CARTESIAN_POINT('Ctrl Pts',(-3.24413672884812,1.,1.88097764062697));
#62552=CARTESIAN_POINT('Ctrl Pts',(-3.24413672884812,0.666666666666667,
1.88097764062697));
#62553=CARTESIAN_POINT('Ctrl Pts',(-3.24413672884812,0.333333333333333,
1.88097764062697));
#62554=CARTESIAN_POINT('Ctrl Pts',(-3.24413672884812,-0.333333333333333,
1.88097764062697));
#62555=CARTESIAN_POINT('Ctrl Pts',(-3.24413672884812,-0.666666666666667,
1.88097764062697));
#62556=CARTESIAN_POINT('Ctrl Pts',(-3.24413672884812,-1.,1.88097764062697));
#62557=CARTESIAN_POINT('Ctrl Pts',(-3.70708211654725,-1.,1.97421938526992));
#62558=CARTESIAN_POINT('Ctrl Pts',(-3.70708211654725,1.,1.97421938526992));
#62559=CARTESIAN_POINT('Ctrl Pts',(-3.70551008132332,-1.,1.97417727645308));
#62560=CARTESIAN_POINT('Ctrl Pts',(-3.70551008132332,1.,1.97417727645308));
#62561=CARTESIAN_POINT('Ctrl Pts',(-3.70236698912904,-1.,1.97408973726715));
#62562=CARTESIAN_POINT('Ctrl Pts',(-3.70236698912904,1.,1.97408973726715));
#62563=CARTESIAN_POINT('Ctrl Pts',(-3.6976552856004,-1.,1.97394846383216));
#62564=CARTESIAN_POINT('Ctrl Pts',(-3.6976552856004,1.,1.97394846383216));
#62565=CARTESIAN_POINT('Ctrl Pts',(-3.69137888599902,-1.,1.97374016225483));
#62566=CARTESIAN_POINT('Ctrl Pts',(-3.69137888599902,1.,1.97374016225483));
#62567=CARTESIAN_POINT('Ctrl Pts',(-3.68354319915092,-1.,1.97344650304519));
#62568=CARTESIAN_POINT('Ctrl Pts',(-3.68354319915092,1.,1.97344650304519));
#62569=CARTESIAN_POINT('Ctrl Pts',(-3.67571738107084,-1.,1.97311947678516));
#62570=CARTESIAN_POINT('Ctrl Pts',(-3.67571738107084,1.,1.97311947678516));
#62571=CARTESIAN_POINT('Ctrl Pts',(-3.66790152752075,-1.,1.97275897198678));
#62572=CARTESIAN_POINT('Ctrl Pts',(-3.66790152752075,1.,1.97275897198678));
#62573=CARTESIAN_POINT('Ctrl Pts',(-3.6600957816636,-1.,1.9723648543905));
#62574=CARTESIAN_POINT('Ctrl Pts',(-3.6600957816636,1.,1.9723648543905));
#62575=CARTESIAN_POINT('Ctrl Pts',(-3.652300347166,-1.,1.9719369724024));
#62576=CARTESIAN_POINT('Ctrl Pts',(-3.652300347166,1.,1.9719369724024));
#62577=CARTESIAN_POINT('Ctrl Pts',(-3.64451546723514,-1.,1.97147515441164));
#62578=CARTESIAN_POINT('Ctrl Pts',(-3.64451546723514,1.,1.97147515441164));
#62579=CARTESIAN_POINT('Ctrl Pts',(-3.63674139590412,-1.,1.97097920454464));
#62580=CARTESIAN_POINT('Ctrl Pts',(-3.63674139590412,1.,1.97097920454464));
#62581=CARTESIAN_POINT('Ctrl Pts',(-3.62897836973293,-1.,1.97044889850463));
#62582=CARTESIAN_POINT('Ctrl Pts',(-3.62897836973293,1.,1.97044889850463));
#62583=CARTESIAN_POINT('Ctrl Pts',(-3.62122658401893,-1.,1.96988398129978));
#62584=CARTESIAN_POINT('Ctrl Pts',(-3.62122658401893,1.,1.96988398129978));
#62585=CARTESIAN_POINT('Ctrl Pts',(-3.61348615496704,-1.,1.96928416040877));
#62586=CARTESIAN_POINT('Ctrl Pts',(-3.61348615496704,1.,1.96928416040877));
#62587=CARTESIAN_POINT('Ctrl Pts',(-3.60575714017989,-1.,1.9686491188594));
#62588=CARTESIAN_POINT('Ctrl Pts',(-3.60575714017989,1.,1.9686491188594));
#62589=CARTESIAN_POINT('Ctrl Pts',(-3.59803959819938,-1.,1.96797854118369));
#62590=CARTESIAN_POINT('Ctrl Pts',(-3.59803959819938,1.,1.96797854118369));
#62591=CARTESIAN_POINT('Ctrl Pts',(-3.59033364022801,-1.,1.96727213799544));
#62592=CARTESIAN_POINT('Ctrl Pts',(-3.59033364022801,1.,1.96727213799544));
#62593=CARTESIAN_POINT('Ctrl Pts',(-3.58263947663829,-1.,1.96652966688911));
#62594=CARTESIAN_POINT('Ctrl Pts',(-3.58263947663829,1.,1.96652966688911));
#62595=CARTESIAN_POINT('Ctrl Pts',(-3.57495748600959,-1.,1.96575096652789));
#62596=CARTESIAN_POINT('Ctrl Pts',(-3.57495748600959,1.,1.96575096652789));
#62597=CARTESIAN_POINT('Ctrl Pts',(-3.56728820357791,-1.,1.96493594634567));
#62598=CARTESIAN_POINT('Ctrl Pts',(-3.56728820357791,1.,1.96493594634567));
#62599=CARTESIAN_POINT('Ctrl Pts',(-3.55963218706096,-1.,1.96408450906812));
#62600=CARTESIAN_POINT('Ctrl Pts',(-3.55963218706096,1.,1.96408450906812));
#62601=CARTESIAN_POINT('Ctrl Pts',(-3.55198990600886,-1.,1.96319648628644));
#62602=CARTESIAN_POINT('Ctrl Pts',(-3.55198990600886,1.,1.96319648628644));
#62603=CARTESIAN_POINT('Ctrl Pts',(-3.54436163300443,-1.,1.96227157573067));
#62604=CARTESIAN_POINT('Ctrl Pts',(-3.54436163300443,1.,1.96227157573067));
#62605=CARTESIAN_POINT('Ctrl Pts',(-3.53674730625813,-1.,1.96130926212689));
#62606=CARTESIAN_POINT('Ctrl Pts',(-3.53674730625813,1.,1.96130926212689));
#62607=CARTESIAN_POINT('Ctrl Pts',(-3.52914648844351,-1.,1.96030879411566));
#62608=CARTESIAN_POINT('Ctrl Pts',(-3.52914648844351,1.,1.96030879411566));
#62609=CARTESIAN_POINT('Ctrl Pts',(-3.52155867431486,-1.,1.95926936324461));
#62610=CARTESIAN_POINT('Ctrl Pts',(-3.52155867431486,1.,1.95926936324461));
#62611=CARTESIAN_POINT('Ctrl Pts',(-3.51398354617794,-1.,1.95819025316779));
#62612=CARTESIAN_POINT('Ctrl Pts',(-3.51398354617794,1.,1.95819025316779));
#62613=CARTESIAN_POINT('Ctrl Pts',(-3.50642124159909,-1.,1.95707099606511));
#62614=CARTESIAN_POINT('Ctrl Pts',(-3.50642124159909,1.,1.95707099606511));
#62615=CARTESIAN_POINT('Ctrl Pts',(-3.49887263575583,-1.,1.95591153823661));
#62616=CARTESIAN_POINT('Ctrl Pts',(-3.49887263575583,1.,1.95591153823661));
#62617=CARTESIAN_POINT('Ctrl Pts',(-3.49133956289133,-1.,1.95471236969643));
#62618=CARTESIAN_POINT('Ctrl Pts',(-3.49133956289133,1.,1.95471236969643));
#62619=CARTESIAN_POINT('Ctrl Pts',(-3.48382414832634,-1.,1.95347412486308));
#62620=CARTESIAN_POINT('Ctrl Pts',(-3.48382414832634,1.,1.95347412486308));
#62621=CARTESIAN_POINT('Ctrl Pts',(-3.47632820495921,-1.,1.95219722189876));
#62622=CARTESIAN_POINT('Ctrl Pts',(-3.47632820495921,1.,1.95219722189876));
#62623=CARTESIAN_POINT('Ctrl Pts',(-3.46885258974191,-1.,1.95088147859876));
#62624=CARTESIAN_POINT('Ctrl Pts',(-3.46885258974191,1.,1.95088147859876));
#62625=CARTESIAN_POINT('Ctrl Pts',(-3.46139661060962,-1.,1.94952575850197));
#62626=CARTESIAN_POINT('Ctrl Pts',(-3.46139661060962,1.,1.94952575850197));
#62627=CARTESIAN_POINT('Ctrl Pts',(-3.45395731584051,-1.,1.94812754766524));
#62628=CARTESIAN_POINT('Ctrl Pts',(-3.45395731584051,1.,1.94812754766524));
#62629=CARTESIAN_POINT('Ctrl Pts',(-3.44653088665681,-1.,1.94668377715329));
#62630=CARTESIAN_POINT('Ctrl Pts',(-3.44653088665681,1.,1.94668377715329));
#62631=CARTESIAN_POINT('Ctrl Pts',(-3.43911410197687,-1.,1.94519168842879));
#62632=CARTESIAN_POINT('Ctrl Pts',(-3.43911410197687,1.,1.94519168842879));
#62633=CARTESIAN_POINT('Ctrl Pts',(-3.43170586602434,-1.,1.94364973660284));
#62634=CARTESIAN_POINT('Ctrl Pts',(-3.43170586602434,1.,1.94364973660284));
#62635=CARTESIAN_POINT('Ctrl Pts',(-3.42430850941503,-1.,1.94205835913696));
#62636=CARTESIAN_POINT('Ctrl Pts',(-3.42430850941503,1.,1.94205835913696));
#62637=CARTESIAN_POINT('Ctrl Pts',(-3.41692971994096,-1.,1.94042111965246));
#62638=CARTESIAN_POINT('Ctrl Pts',(-3.41692971994096,1.,1.94042111965246));
#62639=CARTESIAN_POINT('Ctrl Pts',(-3.40957978266642,-1.,1.93874306008143));
#62640=CARTESIAN_POINT('Ctrl Pts',(-3.40957978266642,1.,1.93874306008143));
#62641=CARTESIAN_POINT('Ctrl Pts',(-3.40226802104109,-1.,1.93702857723098));
#62642=CARTESIAN_POINT('Ctrl Pts',(-3.40226802104109,1.,1.93702857723098));
#62643=CARTESIAN_POINT('Ctrl Pts',(-3.39499923640795,-1.,1.93527929945985));
#62644=CARTESIAN_POINT('Ctrl Pts',(-3.39499923640795,1.,1.93527929945985));
#62645=CARTESIAN_POINT('Ctrl Pts',(-3.38777076883256,-1.,1.93349233176788));
#62646=CARTESIAN_POINT('Ctrl Pts',(-3.38777076883256,1.,1.93349233176788));
#62647=CARTESIAN_POINT('Ctrl Pts',(-3.3805676852555,-1.,1.93165739093276));
#62648=CARTESIAN_POINT('Ctrl Pts',(-3.3805676852555,1.,1.93165739093276));
#62649=CARTESIAN_POINT('Ctrl Pts',(-3.37336807068043,-1.,1.92975993109877));
#62650=CARTESIAN_POINT('Ctrl Pts',(-3.37336807068043,1.,1.92975993109877));
#62651=CARTESIAN_POINT('Ctrl Pts',(-3.36615168657567,-1.,1.92778626543786));
#62652=CARTESIAN_POINT('Ctrl Pts',(-3.36615168657567,1.,1.92778626543786));
#62653=CARTESIAN_POINT('Ctrl Pts',(-3.35890824422965,-1.,1.92572846125756));
#62654=CARTESIAN_POINT('Ctrl Pts',(-3.35890824422965,1.,1.92572846125756));
#62655=CARTESIAN_POINT('Ctrl Pts',(-3.35164424847223,-1.,1.92358838440528));
#62656=CARTESIAN_POINT('Ctrl Pts',(-3.35164424847223,1.,1.92358838440528));
#62657=CARTESIAN_POINT('Ctrl Pts',(-3.34439448941961,-1.,1.92138450828404));
#62658=CARTESIAN_POINT('Ctrl Pts',(-3.34439448941961,1.,1.92138450828404));
#62659=CARTESIAN_POINT('Ctrl Pts',(-3.33721230710012,-1.,1.9191460961021));
#62660=CARTESIAN_POINT('Ctrl Pts',(-3.33721230710012,1.,1.9191460961021));
#62661=CARTESIAN_POINT('Ctrl Pts',(-3.33014884257873,-1.,1.91690081930331));
#62662=CARTESIAN_POINT('Ctrl Pts',(-3.33014884257873,1.,1.91690081930331));
#62663=CARTESIAN_POINT('Ctrl Pts',(-3.32323403454535,-1.,1.91466343916628));
#62664=CARTESIAN_POINT('Ctrl Pts',(-3.32323403454535,1.,1.91466343916628));
#62665=CARTESIAN_POINT('Ctrl Pts',(-3.31646052426364,-1.,1.91242616234442));
#62666=CARTESIAN_POINT('Ctrl Pts',(-3.31646052426364,1.,1.91242616234442));
#62667=CARTESIAN_POINT('Ctrl Pts',(-3.30975721158596,-1.,1.91014297830446));
#62668=CARTESIAN_POINT('Ctrl Pts',(-3.30975721158596,1.,1.91014297830446));
#62669=CARTESIAN_POINT('Ctrl Pts',(-3.30300595568195,-1.,1.90773912171341));
#62670=CARTESIAN_POINT('Ctrl Pts',(-3.30300595568195,1.,1.90773912171341));
#62671=CARTESIAN_POINT('Ctrl Pts',(-3.29608978722113,-1.,1.90513891864087));
#62672=CARTESIAN_POINT('Ctrl Pts',(-3.29608978722113,1.,1.90513891864087));
#62673=CARTESIAN_POINT('Ctrl Pts',(-3.2889344860029,-1.,1.90228971247527));
#62674=CARTESIAN_POINT('Ctrl Pts',(-3.2889344860029,1.,1.90228971247527));
#62675=CARTESIAN_POINT('Ctrl Pts',(-3.28154737912352,-1.,1.89918429230462));
#62676=CARTESIAN_POINT('Ctrl Pts',(-3.28154737912352,1.,1.89918429230462));
#62677=CARTESIAN_POINT('Ctrl Pts',(-3.27407108933139,-1.,1.89589172903793));
#62678=CARTESIAN_POINT('Ctrl Pts',(-3.27407108933139,1.,1.89589172903793));
#62679=CARTESIAN_POINT('Ctrl Pts',(-3.26677653888676,-1.,1.89255393500965));
#62680=CARTESIAN_POINT('Ctrl Pts',(-3.26677653888676,1.,1.89255393500965));
#62681=CARTESIAN_POINT('Ctrl Pts',(-3.25999885193947,-1.,1.88934996203698));
#62682=CARTESIAN_POINT('Ctrl Pts',(-3.25999885193947,1.,1.88934996203698));
#62683=CARTESIAN_POINT('Ctrl Pts',(-3.25408686339463,-1.,1.88646802523466));
#62684=CARTESIAN_POINT('Ctrl Pts',(-3.25408686339463,1.,1.88646802523466));
#62685=CARTESIAN_POINT('Ctrl Pts',(-3.24935200511918,-1.,1.88407708646357));
#62686=CARTESIAN_POINT('Ctrl Pts',(-3.24935200511918,1.,1.88407708646357));
#62687=CARTESIAN_POINT('Ctrl Pts',(-3.24600543790443,-1.,1.88229202582941));
#62688=CARTESIAN_POINT('Ctrl Pts',(-3.24600543790443,1.,1.88229202582941));
#62689=CARTESIAN_POINT('Ctrl Pts',(-3.24451807186481,-1.,1.88139187908074));
#62690=CARTESIAN_POINT('Ctrl Pts',(-3.24451807186481,1.,1.88139187908074));
#62691=CARTESIAN_POINT('Ctrl Pts',(-3.24408699284121,-1.,1.88102201872555));
#62692=CARTESIAN_POINT('Ctrl Pts',(-3.24408699284121,1.,1.88102201872555));
#62693=CARTESIAN_POINT('Ctrl Pts',(-3.24410359189609,-1.,1.88091100680349));
#62694=CARTESIAN_POINT('Ctrl Pts',(-3.24410359189609,1.,1.88091100680349));
#62695=CARTESIAN_POINT('Ctrl Pts',(-3.24418789321065,-1.,1.8808893942881));
#62696=CARTESIAN_POINT('Ctrl Pts',(-3.24418789321065,1.,1.8808893942881));
#62697=CARTESIAN_POINT('',(-3.70708211654725,1.,1.97421938526992));
#62698=CARTESIAN_POINT('Ctrl Pts',(-3.70708211654725,1.,1.97421938526992));
#62699=CARTESIAN_POINT('Ctrl Pts',(-3.70551008132332,1.,1.97417727645308));
#62700=CARTESIAN_POINT('Ctrl Pts',(-3.70236698912904,1.,1.97408973726715));
#62701=CARTESIAN_POINT('Ctrl Pts',(-3.6976552856004,1.,1.97394846383216));
#62702=CARTESIAN_POINT('Ctrl Pts',(-3.69137888599902,1.,1.97374016225483));
#62703=CARTESIAN_POINT('Ctrl Pts',(-3.68354319915092,1.,1.97344650304519));
#62704=CARTESIAN_POINT('Ctrl Pts',(-3.67571738107084,1.,1.97311947678516));
#62705=CARTESIAN_POINT('Ctrl Pts',(-3.66790152752075,1.,1.97275897198678));
#62706=CARTESIAN_POINT('Ctrl Pts',(-3.6600957816636,1.,1.9723648543905));
#62707=CARTESIAN_POINT('Ctrl Pts',(-3.652300347166,1.,1.9719369724024));
#62708=CARTESIAN_POINT('Ctrl Pts',(-3.64451546723514,1.,1.97147515441164));
#62709=CARTESIAN_POINT('Ctrl Pts',(-3.63674139590412,1.,1.97097920454464));
#62710=CARTESIAN_POINT('Ctrl Pts',(-3.62897836973293,1.,1.97044889850463));
#62711=CARTESIAN_POINT('Ctrl Pts',(-3.62122658401893,1.,1.96988398129978));
#62712=CARTESIAN_POINT('Ctrl Pts',(-3.61348615496704,1.,1.96928416040877));
#62713=CARTESIAN_POINT('Ctrl Pts',(-3.60575714017989,1.,1.9686491188594));
#62714=CARTESIAN_POINT('Ctrl Pts',(-3.59803959819938,1.,1.96797854118369));
#62715=CARTESIAN_POINT('Ctrl Pts',(-3.59033364022801,1.,1.96727213799544));
#62716=CARTESIAN_POINT('Ctrl Pts',(-3.58263947663829,1.,1.96652966688911));
#62717=CARTESIAN_POINT('Ctrl Pts',(-3.57495748600959,1.,1.96575096652789));
#62718=CARTESIAN_POINT('Ctrl Pts',(-3.56728820357791,1.,1.96493594634567));
#62719=CARTESIAN_POINT('Ctrl Pts',(-3.55963218706096,1.,1.96408450906812));
#62720=CARTESIAN_POINT('Ctrl Pts',(-3.55198990600886,1.,1.96319648628644));
#62721=CARTESIAN_POINT('Ctrl Pts',(-3.54436163300443,1.,1.96227157573067));
#62722=CARTESIAN_POINT('Ctrl Pts',(-3.53674730625813,1.,1.96130926212689));
#62723=CARTESIAN_POINT('Ctrl Pts',(-3.52914648844351,1.,1.96030879411566));
#62724=CARTESIAN_POINT('Ctrl Pts',(-3.52155867431486,1.,1.95926936324461));
#62725=CARTESIAN_POINT('Ctrl Pts',(-3.51398354617794,1.,1.95819025316779));
#62726=CARTESIAN_POINT('Ctrl Pts',(-3.50642124159909,1.,1.95707099606511));
#62727=CARTESIAN_POINT('Ctrl Pts',(-3.49887263575583,1.,1.95591153823661));
#62728=CARTESIAN_POINT('Ctrl Pts',(-3.49133956289133,1.,1.95471236969643));
#62729=CARTESIAN_POINT('Ctrl Pts',(-3.48382414832634,1.,1.95347412486308));
#62730=CARTESIAN_POINT('Ctrl Pts',(-3.47632820495921,1.,1.95219722189876));
#62731=CARTESIAN_POINT('Ctrl Pts',(-3.46885258974191,1.,1.95088147859876));
#62732=CARTESIAN_POINT('Ctrl Pts',(-3.46139661060962,1.,1.94952575850197));
#62733=CARTESIAN_POINT('Ctrl Pts',(-3.45395731584051,1.,1.94812754766524));
#62734=CARTESIAN_POINT('Ctrl Pts',(-3.44653088665681,1.,1.94668377715329));
#62735=CARTESIAN_POINT('Ctrl Pts',(-3.43911410197687,1.,1.94519168842879));
#62736=CARTESIAN_POINT('Ctrl Pts',(-3.43170586602434,1.,1.94364973660284));
#62737=CARTESIAN_POINT('Ctrl Pts',(-3.42430850941503,1.,1.94205835913696));
#62738=CARTESIAN_POINT('Ctrl Pts',(-3.41692971994096,1.,1.94042111965246));
#62739=CARTESIAN_POINT('Ctrl Pts',(-3.40957978266642,1.,1.93874306008143));
#62740=CARTESIAN_POINT('Ctrl Pts',(-3.40226802104109,1.,1.93702857723098));
#62741=CARTESIAN_POINT('Ctrl Pts',(-3.39499923640795,1.,1.93527929945985));
#62742=CARTESIAN_POINT('Ctrl Pts',(-3.38777076883256,1.,1.93349233176788));
#62743=CARTESIAN_POINT('Ctrl Pts',(-3.3805676852555,1.,1.93165739093276));
#62744=CARTESIAN_POINT('Ctrl Pts',(-3.37336807068043,1.,1.92975993109877));
#62745=CARTESIAN_POINT('Ctrl Pts',(-3.36615168657567,1.,1.92778626543786));
#62746=CARTESIAN_POINT('Ctrl Pts',(-3.35890824422965,1.,1.92572846125756));
#62747=CARTESIAN_POINT('Ctrl Pts',(-3.35164424847223,1.,1.92358838440528));
#62748=CARTESIAN_POINT('Ctrl Pts',(-3.34439448941961,1.,1.92138450828404));
#62749=CARTESIAN_POINT('Ctrl Pts',(-3.33721230710012,1.,1.9191460961021));
#62750=CARTESIAN_POINT('Ctrl Pts',(-3.33014884257873,1.,1.91690081930331));
#62751=CARTESIAN_POINT('Ctrl Pts',(-3.32323403454535,1.,1.91466343916628));
#62752=CARTESIAN_POINT('Ctrl Pts',(-3.31646052426364,1.,1.91242616234442));
#62753=CARTESIAN_POINT('Ctrl Pts',(-3.30975721158596,1.,1.91014297830446));
#62754=CARTESIAN_POINT('Ctrl Pts',(-3.30300595568195,1.,1.90773912171341));
#62755=CARTESIAN_POINT('Ctrl Pts',(-3.29608978722113,1.,1.90513891864087));
#62756=CARTESIAN_POINT('Ctrl Pts',(-3.2889344860029,1.,1.90228971247527));
#62757=CARTESIAN_POINT('Ctrl Pts',(-3.28154737912352,1.,1.89918429230462));
#62758=CARTESIAN_POINT('Ctrl Pts',(-3.27407108933139,1.,1.89589172903793));
#62759=CARTESIAN_POINT('Ctrl Pts',(-3.26677653888676,1.,1.89255393500965));
#62760=CARTESIAN_POINT('Ctrl Pts',(-3.25999885193947,1.,1.88934996203698));
#62761=CARTESIAN_POINT('Ctrl Pts',(-3.25408686339463,1.,1.88646802523466));
#62762=CARTESIAN_POINT('Ctrl Pts',(-3.24935200511918,1.,1.88407708646357));
#62763=CARTESIAN_POINT('Ctrl Pts',(-3.2462565441079,1.,1.88242596600454));
#62764=CARTESIAN_POINT('Ctrl Pts',(-3.24480754676064,1.,1.88156537699203));
#62765=CARTESIAN_POINT('Ctrl Pts',(-3.24428080353022,1.,1.88117508446775));
#62766=CARTESIAN_POINT('Ctrl Pts',(-3.24415531671284,1.,1.8810229239812));
#62767=CARTESIAN_POINT('Ctrl Pts',(-3.24413672884812,1.,1.88097764062697));
#62768=CARTESIAN_POINT('',(-3.70708211654725,0.,1.97421938526992));
#62769=CARTESIAN_POINT('Ctrl Pts',(-3.42855728381368,-1.,1.519044091397));
#62770=CARTESIAN_POINT('Ctrl Pts',(-3.42855728381368,1.,1.519044091397));
#62771=CARTESIAN_POINT('Ctrl Pts',(-3.42852521763778,-1.,1.51896318668366));
#62772=CARTESIAN_POINT('Ctrl Pts',(-3.42852521763778,1.,1.51896318668366));
#62773=CARTESIAN_POINT('Ctrl Pts',(-3.42860527149177,-1.,1.51888450659652));
#62774=CARTESIAN_POINT('Ctrl Pts',(-3.42860527149177,1.,1.51888450659652));
#62775=CARTESIAN_POINT('Ctrl Pts',(-3.42915787669893,-1.,1.51901585839109));
#62776=CARTESIAN_POINT('Ctrl Pts',(-3.42915787669893,1.,1.51901585839109));
#62777=CARTESIAN_POINT('Ctrl Pts',(-3.43076036253837,-1.,1.51969006980999));
#62778=CARTESIAN_POINT('Ctrl Pts',(-3.43076036253837,1.,1.51969006980999));
#62779=CARTESIAN_POINT('Ctrl Pts',(-3.43417156977893,-1.,1.52134826724292));
#62780=CARTESIAN_POINT('Ctrl Pts',(-3.43417156977893,1.,1.52134826724292));
#62781=CARTESIAN_POINT('Ctrl Pts',(-3.4388889597401,-1.,1.5237734895035));
#62782=CARTESIAN_POINT('Ctrl Pts',(-3.4388889597401,1.,1.5237734895035));
#62783=CARTESIAN_POINT('Ctrl Pts',(-3.44469547526647,-1.,1.52686242875556));
#62784=CARTESIAN_POINT('Ctrl Pts',(-3.44469547526647,1.,1.52686242875556));
#62785=CARTESIAN_POINT('Ctrl Pts',(-3.45127136828305,-1.,1.53046244461635));
#62786=CARTESIAN_POINT('Ctrl Pts',(-3.45127136828305,1.,1.53046244461635));
#62787=CARTESIAN_POINT('Ctrl Pts',(-3.45825932955032,-1.,1.53440195378792));
#62788=CARTESIAN_POINT('Ctrl Pts',(-3.45825932955032,1.,1.53440195378792));
#62789=CARTESIAN_POINT('Ctrl Pts',(-3.46531752207153,-1.,1.53851507915502));
#62790=CARTESIAN_POINT('Ctrl Pts',(-3.46531752207153,1.,1.53851507915502));
#62791=CARTESIAN_POINT('Ctrl Pts',(-3.47217189224653,-1.,1.54266605398187));
#62792=CARTESIAN_POINT('Ctrl Pts',(-3.47217189224653,1.,1.54266605398187));
#62793=CARTESIAN_POINT('Ctrl Pts',(-3.47868272898751,-1.,1.54678009290276));
#62794=CARTESIAN_POINT('Ctrl Pts',(-3.47868272898751,1.,1.54678009290276));
#62795=CARTESIAN_POINT('Ctrl Pts',(-3.48485155928567,-1.,1.55084702970452));
#62796=CARTESIAN_POINT('Ctrl Pts',(-3.48485155928567,1.,1.55084702970452));
#62797=CARTESIAN_POINT('Ctrl Pts',(-3.4907646087742,-1.,1.55489595901116));
#62798=CARTESIAN_POINT('Ctrl Pts',(-3.4907646087742,1.,1.55489595901116));
#62799=CARTESIAN_POINT('Ctrl Pts',(-3.49655185179655,-1.,1.55897703097874));
#62800=CARTESIAN_POINT('Ctrl Pts',(-3.49655185179655,1.,1.55897703097874));
#62801=CARTESIAN_POINT('Ctrl Pts',(-3.50234321621578,-1.,1.56314187758675));
#62802=CARTESIAN_POINT('Ctrl Pts',(-3.50234321621578,1.,1.56314187758675));
#62803=CARTESIAN_POINT('Ctrl Pts',(-3.50821771695363,-1.,1.56742097575012));
#62804=CARTESIAN_POINT('Ctrl Pts',(-3.50821771695363,1.,1.56742097575012));
#62805=CARTESIAN_POINT('Ctrl Pts',(-3.51418598431665,-1.,1.57181569799743));
#62806=CARTESIAN_POINT('Ctrl Pts',(-3.51418598431665,1.,1.57181569799743));
#62807=CARTESIAN_POINT('Ctrl Pts',(-3.52021847865912,-1.,1.57631049988158));
#62808=CARTESIAN_POINT('Ctrl Pts',(-3.52021847865912,1.,1.57631049988158));
#62809=CARTESIAN_POINT('Ctrl Pts',(-3.52626275334881,-1.,1.58088027227848));
#62810=CARTESIAN_POINT('Ctrl Pts',(-3.52626275334881,1.,1.58088027227848));
#62811=CARTESIAN_POINT('Ctrl Pts',(-3.5322637814708,-1.,1.58549906268088));
#62812=CARTESIAN_POINT('Ctrl Pts',(-3.5322637814708,1.,1.58549906268088));
#62813=CARTESIAN_POINT('Ctrl Pts',(-3.53818616861077,-1.,1.59014958368739));
#62814=CARTESIAN_POINT('Ctrl Pts',(-3.53818616861077,1.,1.59014958368739));
#62815=CARTESIAN_POINT('Ctrl Pts',(-3.54402458182337,-1.,1.59482766949766));
#62816=CARTESIAN_POINT('Ctrl Pts',(-3.54402458182337,1.,1.59482766949766));
#62817=CARTESIAN_POINT('Ctrl Pts',(-3.54979148634454,-1.,1.59953698113457));
#62818=CARTESIAN_POINT('Ctrl Pts',(-3.54979148634454,1.,1.59953698113457));
#62819=CARTESIAN_POINT('Ctrl Pts',(-3.55550985096129,-1.,1.60428584699853));
#62820=CARTESIAN_POINT('Ctrl Pts',(-3.55550985096129,1.,1.60428584699853));
#62821=CARTESIAN_POINT('Ctrl Pts',(-3.5612043248298,-1.,1.60908344685457));
#62822=CARTESIAN_POINT('Ctrl Pts',(-3.5612043248298,1.,1.60908344685457));
#62823=CARTESIAN_POINT('Ctrl Pts',(-3.56689200468387,-1.,1.61393581747514));
#62824=CARTESIAN_POINT('Ctrl Pts',(-3.56689200468387,1.,1.61393581747514));
#62825=CARTESIAN_POINT('Ctrl Pts',(-3.57257679609806,-1.,1.61884340915404));
#62826=CARTESIAN_POINT('Ctrl Pts',(-3.57257679609806,1.,1.61884340915404));
#62827=CARTESIAN_POINT('Ctrl Pts',(-3.5782545595439,-1.,1.62380329464844));
#62828=CARTESIAN_POINT('Ctrl Pts',(-3.5782545595439,1.,1.62380329464844));
#62829=CARTESIAN_POINT('Ctrl Pts',(-3.58391625774343,-1.,1.62881051550745));
#62830=CARTESIAN_POINT('Ctrl Pts',(-3.58391625774343,1.,1.62881051550745));
#62831=CARTESIAN_POINT('Ctrl Pts',(-3.58955176627879,-1.,1.6338597145126));
#62832=CARTESIAN_POINT('Ctrl Pts',(-3.58955176627879,1.,1.6338597145126));
#62833=CARTESIAN_POINT('Ctrl Pts',(-3.59515368334893,-1.,1.63894676675352));
#62834=CARTESIAN_POINT('Ctrl Pts',(-3.59515368334893,1.,1.63894676675352));
#62835=CARTESIAN_POINT('Ctrl Pts',(-3.60072028513845,-1.,1.64407004385582));
#62836=CARTESIAN_POINT('Ctrl Pts',(-3.60072028513845,1.,1.64407004385582));
#62837=CARTESIAN_POINT('Ctrl Pts',(-3.60625346556992,-1.,1.64922952425832));
#62838=CARTESIAN_POINT('Ctrl Pts',(-3.60625346556992,1.,1.64922952425832));
#62839=CARTESIAN_POINT('Ctrl Pts',(-3.61175734965127,-1.,1.65442619244325));
#62840=CARTESIAN_POINT('Ctrl Pts',(-3.61175734965127,1.,1.65442619244325));
#62841=CARTESIAN_POINT('Ctrl Pts',(-3.61723666482456,-1.,1.65966133399186));
#62842=CARTESIAN_POINT('Ctrl Pts',(-3.61723666482456,1.,1.65966133399186));
#62843=CARTESIAN_POINT('Ctrl Pts',(-3.62269517989109,-1.,1.66493585923855));
#62844=CARTESIAN_POINT('Ctrl Pts',(-3.62269517989109,1.,1.66493585923855));
#62845=CARTESIAN_POINT('Ctrl Pts',(-3.62813422105271,-1.,1.67024966008045));
#62846=CARTESIAN_POINT('Ctrl Pts',(-3.62813422105271,1.,1.67024966008045));
#62847=CARTESIAN_POINT('Ctrl Pts',(-3.63355343201232,-1.,1.67560193613156));
#62848=CARTESIAN_POINT('Ctrl Pts',(-3.63355343201232,1.,1.67560193613156));
#62849=CARTESIAN_POINT('Ctrl Pts',(-3.63895140887462,-1.,1.68099146651586));
#62850=CARTESIAN_POINT('Ctrl Pts',(-3.63895140887462,1.,1.68099146651586));
#62851=CARTESIAN_POINT('Ctrl Pts',(-3.64432638915203,-1.,1.68641690471457));
#62852=CARTESIAN_POINT('Ctrl Pts',(-3.64432638915203,1.,1.68641690471457));
#62853=CARTESIAN_POINT('Ctrl Pts',(-3.64967689827371,-1.,1.69187705481689));
#62854=CARTESIAN_POINT('Ctrl Pts',(-3.64967689827371,1.,1.69187705481689));
#62855=CARTESIAN_POINT('Ctrl Pts',(-3.65500246526749,-1.,1.69737117722534));
#62856=CARTESIAN_POINT('Ctrl Pts',(-3.65500246526749,1.,1.69737117722534));
#62857=CARTESIAN_POINT('Ctrl Pts',(-3.66030338774847,-1.,1.70289888566873));
#62858=CARTESIAN_POINT('Ctrl Pts',(-3.66030338774847,1.,1.70289888566873));
#62859=CARTESIAN_POINT('Ctrl Pts',(-3.66558043198876,-1.,1.70846001610956));
#62860=CARTESIAN_POINT('Ctrl Pts',(-3.66558043198876,1.,1.70846001610956));
#62861=CARTESIAN_POINT('Ctrl Pts',(-3.67083454901611,-1.,1.71405450210383));
#62862=CARTESIAN_POINT('Ctrl Pts',(-3.67083454901611,1.,1.71405450210383));
#62863=CARTESIAN_POINT('Ctrl Pts',(-3.67606660374709,-1.,1.71968225581808));
#62864=CARTESIAN_POINT('Ctrl Pts',(-3.67606660374709,1.,1.71968225581808));
#62865=CARTESIAN_POINT('Ctrl Pts',(-3.68127704936579,-1.,1.72534302437056));
#62866=CARTESIAN_POINT('Ctrl Pts',(-3.68127704936579,1.,1.72534302437056));
#62867=CARTESIAN_POINT('Ctrl Pts',(-3.68646597019332,-1.,1.73103640956717));
#62868=CARTESIAN_POINT('Ctrl Pts',(-3.68646597019332,1.,1.73103640956717));
#62869=CARTESIAN_POINT('Ctrl Pts',(-3.69163322648036,-1.,1.73676193254557));
#62870=CARTESIAN_POINT('Ctrl Pts',(-3.69163322648036,1.,1.73676193254557));
#62871=CARTESIAN_POINT('Ctrl Pts',(-3.69677856910517,-1.,1.74251908492617));
#62872=CARTESIAN_POINT('Ctrl Pts',(-3.69677856910517,1.,1.74251908492617));
#62873=CARTESIAN_POINT('Ctrl Pts',(-3.7019017567335,-1.,1.74830738046057));
#62874=CARTESIAN_POINT('Ctrl Pts',(-3.7019017567335,1.,1.74830738046057));
#62875=CARTESIAN_POINT('Ctrl Pts',(-3.70700269736659,-1.,1.75412641804042));
#62876=CARTESIAN_POINT('Ctrl Pts',(-3.70700269736659,1.,1.75412641804042));
#62877=CARTESIAN_POINT('Ctrl Pts',(-3.71208146346136,-1.,1.75997588498865));
#62878=CARTESIAN_POINT('Ctrl Pts',(-3.71208146346136,1.,1.75997588498865));
#62879=CARTESIAN_POINT('Ctrl Pts',(-3.71713822377359,-1.,1.76585552124394));
#62880=CARTESIAN_POINT('Ctrl Pts',(-3.71713822377359,1.,1.76585552124394));
#62881=CARTESIAN_POINT('Ctrl Pts',(-3.72217319911254,-1.,1.77176509401761));
#62882=CARTESIAN_POINT('Ctrl Pts',(-3.72217319911254,1.,1.77176509401761));
#62883=CARTESIAN_POINT('Ctrl Pts',(-3.72718661205609,-1.,1.77770437039658));
#62884=CARTESIAN_POINT('Ctrl Pts',(-3.72718661205609,1.,1.77770437039658));
#62885=CARTESIAN_POINT('Ctrl Pts',(-3.7321786309547,-1.,1.78367308442901));
#62886=CARTESIAN_POINT('Ctrl Pts',(-3.7321786309547,1.,1.78367308442901));
#62887=CARTESIAN_POINT('Ctrl Pts',(-3.73714934730681,-1.,1.78967092823491));
#62888=CARTESIAN_POINT('Ctrl Pts',(-3.73714934730681,1.,1.78967092823491));
#62889=CARTESIAN_POINT('Ctrl Pts',(-3.74209880352445,-1.,1.79569757859422));
#62890=CARTESIAN_POINT('Ctrl Pts',(-3.74209880352445,1.,1.79569757859422));
#62891=CARTESIAN_POINT('Ctrl Pts',(-3.74702700875467,-1.,1.8017527148577));
#62892=CARTESIAN_POINT('Ctrl Pts',(-3.74702700875467,1.,1.8017527148577));
#62893=CARTESIAN_POINT('Ctrl Pts',(-3.75193395887977,-1.,1.80783603939617));
#62894=CARTESIAN_POINT('Ctrl Pts',(-3.75193395887977,1.,1.80783603939617));
#62895=CARTESIAN_POINT('Ctrl Pts',(-3.75681965683071,-1.,1.8139472983358));
#62896=CARTESIAN_POINT('Ctrl Pts',(-3.75681965683071,1.,1.8139472983358));
#62897=CARTESIAN_POINT('Ctrl Pts',(-3.76168412707948,-1.,1.82008629694091));
#62898=CARTESIAN_POINT('Ctrl Pts',(-3.76168412707948,1.,1.82008629694091));
#62899=CARTESIAN_POINT('Ctrl Pts',(-3.76652740353775,-1.,1.82625289220915));
#62900=CARTESIAN_POINT('Ctrl Pts',(-3.76652740353775,1.,1.82625289220915));
#62901=CARTESIAN_POINT('Ctrl Pts',(-3.77038509817999,-1.,1.83120816955645));
#62902=CARTESIAN_POINT('Ctrl Pts',(-3.77038509817999,1.,1.83120816955645));
#62903=CARTESIAN_POINT('Ctrl Pts',(-3.77326886064398,-1.,1.83493697934534));
#62904=CARTESIAN_POINT('Ctrl Pts',(-3.77326886064398,1.,1.83493697934534));
#62905=CARTESIAN_POINT('Ctrl Pts',(-3.77518714457833,-1.,1.83742834010626));
#62906=CARTESIAN_POINT('Ctrl Pts',(-3.77518714457833,1.,1.83742834010626));
#62907=CARTESIAN_POINT('Ctrl Pts',(-3.77614523045147,-1.,1.8386753923786));
#62908=CARTESIAN_POINT('Ctrl Pts',(-3.77614523045147,1.,1.8386753923786));
#62909=CARTESIAN_POINT('',(-3.42859860294306,1.,1.5189508286633));
#62910=CARTESIAN_POINT('Ctrl Pts',(-3.42859860294306,-1.,1.5189508286633));
#62911=CARTESIAN_POINT('Ctrl Pts',(-3.42859860294306,-0.666666666666667,
1.5189508286633));
#62912=CARTESIAN_POINT('Ctrl Pts',(-3.42859860294306,-0.333333333333333,
1.5189508286633));
#62913=CARTESIAN_POINT('Ctrl Pts',(-3.42859860294306,0.333333333333333,
1.5189508286633));
#62914=CARTESIAN_POINT('Ctrl Pts',(-3.42859860294306,0.666666666666667,
1.5189508286633));
#62915=CARTESIAN_POINT('Ctrl Pts',(-3.42859860294306,1.,1.5189508286633));
#62916=CARTESIAN_POINT('',(-3.77614523045147,1.,1.8386753923786));
#62917=CARTESIAN_POINT('',(-3.77614523045147,0.,1.8386753923786));
#62918=CARTESIAN_POINT('Ctrl Pts',(-3.42859860294306,1.,1.5189508286633));
#62919=CARTESIAN_POINT('Ctrl Pts',(-3.42864616361875,1.,1.51893924967331));
#62920=CARTESIAN_POINT('Ctrl Pts',(-3.42884302333841,1.,1.5189513329503));
#62921=CARTESIAN_POINT('Ctrl Pts',(-3.42946838852587,1.,1.51914806898491));
#62922=CARTESIAN_POINT('Ctrl Pts',(-3.43101631893414,1.,1.5198144909338));
#62923=CARTESIAN_POINT('Ctrl Pts',(-3.43417156977893,1.,1.52134826724292));
#62924=CARTESIAN_POINT('Ctrl Pts',(-3.4388889597401,1.,1.5237734895035));
#62925=CARTESIAN_POINT('Ctrl Pts',(-3.44469547526647,1.,1.52686242875556));
#62926=CARTESIAN_POINT('Ctrl Pts',(-3.45127136828305,1.,1.53046244461635));
#62927=CARTESIAN_POINT('Ctrl Pts',(-3.45825932955032,1.,1.53440195378792));
#62928=CARTESIAN_POINT('Ctrl Pts',(-3.46531752207153,1.,1.53851507915502));
#62929=CARTESIAN_POINT('Ctrl Pts',(-3.47217189224653,1.,1.54266605398187));
#62930=CARTESIAN_POINT('Ctrl Pts',(-3.47868272898751,1.,1.54678009290276));
#62931=CARTESIAN_POINT('Ctrl Pts',(-3.48485155928567,1.,1.55084702970452));
#62932=CARTESIAN_POINT('Ctrl Pts',(-3.4907646087742,1.,1.55489595901116));
#62933=CARTESIAN_POINT('Ctrl Pts',(-3.49655185179655,1.,1.55897703097874));
#62934=CARTESIAN_POINT('Ctrl Pts',(-3.50234321621578,1.,1.56314187758675));
#62935=CARTESIAN_POINT('Ctrl Pts',(-3.50821771695363,1.,1.56742097575012));
#62936=CARTESIAN_POINT('Ctrl Pts',(-3.51418598431665,1.,1.57181569799743));
#62937=CARTESIAN_POINT('Ctrl Pts',(-3.52021847865912,1.,1.57631049988158));
#62938=CARTESIAN_POINT('Ctrl Pts',(-3.52626275334881,1.,1.58088027227848));
#62939=CARTESIAN_POINT('Ctrl Pts',(-3.5322637814708,1.,1.58549906268088));
#62940=CARTESIAN_POINT('Ctrl Pts',(-3.53818616861077,1.,1.59014958368739));
#62941=CARTESIAN_POINT('Ctrl Pts',(-3.54402458182337,1.,1.59482766949766));
#62942=CARTESIAN_POINT('Ctrl Pts',(-3.54979148634454,1.,1.59953698113457));
#62943=CARTESIAN_POINT('Ctrl Pts',(-3.55550985096129,1.,1.60428584699853));
#62944=CARTESIAN_POINT('Ctrl Pts',(-3.5612043248298,1.,1.60908344685457));
#62945=CARTESIAN_POINT('Ctrl Pts',(-3.56689200468387,1.,1.61393581747514));
#62946=CARTESIAN_POINT('Ctrl Pts',(-3.57257679609806,1.,1.61884340915404));
#62947=CARTESIAN_POINT('Ctrl Pts',(-3.5782545595439,1.,1.62380329464844));
#62948=CARTESIAN_POINT('Ctrl Pts',(-3.58391625774343,1.,1.62881051550745));
#62949=CARTESIAN_POINT('Ctrl Pts',(-3.58955176627879,1.,1.6338597145126));
#62950=CARTESIAN_POINT('Ctrl Pts',(-3.59515368334893,1.,1.63894676675352));
#62951=CARTESIAN_POINT('Ctrl Pts',(-3.60072028513845,1.,1.64407004385582));
#62952=CARTESIAN_POINT('Ctrl Pts',(-3.60625346556992,1.,1.64922952425832));
#62953=CARTESIAN_POINT('Ctrl Pts',(-3.61175734965127,1.,1.65442619244325));
#62954=CARTESIAN_POINT('Ctrl Pts',(-3.61723666482456,1.,1.65966133399186));
#62955=CARTESIAN_POINT('Ctrl Pts',(-3.62269517989109,1.,1.66493585923855));
#62956=CARTESIAN_POINT('Ctrl Pts',(-3.62813422105271,1.,1.67024966008045));
#62957=CARTESIAN_POINT('Ctrl Pts',(-3.63355343201232,1.,1.67560193613156));
#62958=CARTESIAN_POINT('Ctrl Pts',(-3.63895140887462,1.,1.68099146651586));
#62959=CARTESIAN_POINT('Ctrl Pts',(-3.64432638915203,1.,1.68641690471457));
#62960=CARTESIAN_POINT('Ctrl Pts',(-3.64967689827371,1.,1.69187705481689));
#62961=CARTESIAN_POINT('Ctrl Pts',(-3.65500246526749,1.,1.69737117722534));
#62962=CARTESIAN_POINT('Ctrl Pts',(-3.66030338774847,1.,1.70289888566873));
#62963=CARTESIAN_POINT('Ctrl Pts',(-3.66558043198876,1.,1.70846001610956));
#62964=CARTESIAN_POINT('Ctrl Pts',(-3.67083454901611,1.,1.71405450210383));
#62965=CARTESIAN_POINT('Ctrl Pts',(-3.67606660374709,1.,1.71968225581808));
#62966=CARTESIAN_POINT('Ctrl Pts',(-3.68127704936579,1.,1.72534302437056));
#62967=CARTESIAN_POINT('Ctrl Pts',(-3.68646597019332,1.,1.73103640956717));
#62968=CARTESIAN_POINT('Ctrl Pts',(-3.69163322648036,1.,1.73676193254557));
#62969=CARTESIAN_POINT('Ctrl Pts',(-3.69677856910517,1.,1.74251908492617));
#62970=CARTESIAN_POINT('Ctrl Pts',(-3.7019017567335,1.,1.74830738046057));
#62971=CARTESIAN_POINT('Ctrl Pts',(-3.70700269736659,1.,1.75412641804042));
#62972=CARTESIAN_POINT('Ctrl Pts',(-3.71208146346136,1.,1.75997588498865));
#62973=CARTESIAN_POINT('Ctrl Pts',(-3.71713822377359,1.,1.76585552124394));
#62974=CARTESIAN_POINT('Ctrl Pts',(-3.72217319911254,1.,1.77176509401761));
#62975=CARTESIAN_POINT('Ctrl Pts',(-3.72718661205609,1.,1.77770437039658));
#62976=CARTESIAN_POINT('Ctrl Pts',(-3.7321786309547,1.,1.78367308442901));
#62977=CARTESIAN_POINT('Ctrl Pts',(-3.73714934730681,1.,1.78967092823491));
#62978=CARTESIAN_POINT('Ctrl Pts',(-3.74209880352445,1.,1.79569757859422));
#62979=CARTESIAN_POINT('Ctrl Pts',(-3.74702700875467,1.,1.8017527148577));
#62980=CARTESIAN_POINT('Ctrl Pts',(-3.75193395887977,1.,1.80783603939617));
#62981=CARTESIAN_POINT('Ctrl Pts',(-3.75681965683071,1.,1.8139472983358));
#62982=CARTESIAN_POINT('Ctrl Pts',(-3.76168412707948,1.,1.82008629694091));
#62983=CARTESIAN_POINT('Ctrl Pts',(-3.76652740353775,1.,1.82625289220915));
#62984=CARTESIAN_POINT('Ctrl Pts',(-3.77038509817999,1.,1.83120816955645));
#62985=CARTESIAN_POINT('Ctrl Pts',(-3.77326886064398,1.,1.83493697934534));
#62986=CARTESIAN_POINT('Ctrl Pts',(-3.77518714457833,1.,1.83742834010626));
#62987=CARTESIAN_POINT('Ctrl Pts',(-3.77614523045147,1.,1.8386753923786));
#62988=CARTESIAN_POINT('Origin',(-3.77614523045147,0.,1.8386753923786));
#62989=CARTESIAN_POINT('',(-3.70708211654725,1.,1.97421938526992));
#62990=CARTESIAN_POINT('Origin',(0.,0.,0.));
#62991=CARTESIAN_POINT('',(-3.49844575334386,1.,1.35032489087269));
#62992=CARTESIAN_POINT('Origin',(0.,1.,0.));
#62993=CARTESIAN_POINT('Ctrl Pts',(-3.49844575334386,1.,1.35032489087269));
#62994=CARTESIAN_POINT('Ctrl Pts',(-3.49844575334386,0.666666666666667,
1.35032489087269));
#62995=CARTESIAN_POINT('Ctrl Pts',(-3.49844575334386,0.333333333333333,
1.35032489087269));
#62996=CARTESIAN_POINT('Ctrl Pts',(-3.49844575334386,-0.333333333333333,
1.35032489087269));
#62997=CARTESIAN_POINT('Ctrl Pts',(-3.49844575334386,-0.666666666666667,
1.35032489087269));
#62998=CARTESIAN_POINT('Ctrl Pts',(-3.49844575334386,-1.,1.35032489087269));
#62999=CARTESIAN_POINT('Ctrl Pts',(-3.97027773754922,-1.,1.36999806084572));
#63000=CARTESIAN_POINT('Ctrl Pts',(-3.97027773754922,1.,1.36999806084572));
#63001=CARTESIAN_POINT('Ctrl Pts',(-3.9687184694173,-1.,1.37020239094758));
#63002=CARTESIAN_POINT('Ctrl Pts',(-3.9687184694173,1.,1.37020239094758));
#63003=CARTESIAN_POINT('Ctrl Pts',(-3.96560037975788,-1.,1.37060761746027));
#63004=CARTESIAN_POINT('Ctrl Pts',(-3.96560037975788,1.,1.37060761746027));
#63005=CARTESIAN_POINT('Ctrl Pts',(-3.96092458508407,-1.,1.37120515615663));
#63006=CARTESIAN_POINT('Ctrl Pts',(-3.96092458508407,1.,1.37120515615663));
#63007=CARTESIAN_POINT('Ctrl Pts',(-3.95469287283105,-1.,1.37198126433139));
#63008=CARTESIAN_POINT('Ctrl Pts',(-3.95469287283105,1.,1.37198126433139));
#63009=CARTESIAN_POINT('Ctrl Pts',(-3.94690771786926,-1.,1.37291699203423));
#63010=CARTESIAN_POINT('Ctrl Pts',(-3.94690771786926,1.,1.37291699203423));
#63011=CARTESIAN_POINT('Ctrl Pts',(-3.93912709041791,-1.,1.37381821967499));
#63012=CARTESIAN_POINT('Ctrl Pts',(-3.93912709041791,1.,1.37381821967499));
#63013=CARTESIAN_POINT('Ctrl Pts',(-3.93135106761941,-1.,1.37468482215784));
#63014=CARTESIAN_POINT('Ctrl Pts',(-3.93135106761941,1.,1.37468482215784));
#63015=CARTESIAN_POINT('Ctrl Pts',(-3.92357976987132,-1.,1.37551664448057));
#63016=CARTESIAN_POINT('Ctrl Pts',(-3.92357976987132,1.,1.37551664448057));
#63017=CARTESIAN_POINT('Ctrl Pts',(-3.91581337461825,-1.,1.37631350505516));
#63018=CARTESIAN_POINT('Ctrl Pts',(-3.91581337461825,1.,1.37631350505516));
#63019=CARTESIAN_POINT('Ctrl Pts',(-3.90805209522729,-1.,1.3770751963376));
#63020=CARTESIAN_POINT('Ctrl Pts',(-3.90805209522729,1.,1.3770751963376));
#63021=CARTESIAN_POINT('Ctrl Pts',(-3.90029615196255,-1.,1.3778014851263));
#63022=CARTESIAN_POINT('Ctrl Pts',(-3.90029615196255,1.,1.3778014851263));
#63023=CARTESIAN_POINT('Ctrl Pts',(-3.89254574338385,-1.,1.37849211287981));
#63024=CARTESIAN_POINT('Ctrl Pts',(-3.89254574338385,1.,1.37849211287981));
#63025=CARTESIAN_POINT('Ctrl Pts',(-3.88480102249461,-1.,1.37914679719446));
#63026=CARTESIAN_POINT('Ctrl Pts',(-3.88480102249461,1.,1.37914679719446));
#63027=CARTESIAN_POINT('Ctrl Pts',(-3.87706205830865,-1.,1.37976523097187));
#63028=CARTESIAN_POINT('Ctrl Pts',(-3.87706205830865,1.,1.37976523097187));
#63029=CARTESIAN_POINT('Ctrl Pts',(-3.86932885813403,-1.,1.38034709213129));
#63030=CARTESIAN_POINT('Ctrl Pts',(-3.86932885813403,1.,1.38034709213129));
#63031=CARTESIAN_POINT('Ctrl Pts',(-3.86160143044187,-1.,1.38089205993067));
#63032=CARTESIAN_POINT('Ctrl Pts',(-3.86160143044187,1.,1.38089205993067));
#63033=CARTESIAN_POINT('Ctrl Pts',(-3.85387983979557,-1.,1.38139983115075));
#63034=CARTESIAN_POINT('Ctrl Pts',(-3.85387983979557,1.,1.38139983115075));
#63035=CARTESIAN_POINT('Ctrl Pts',(-3.84616425605705,-1.,1.38187013346089));
#63036=CARTESIAN_POINT('Ctrl Pts',(-3.84616425605705,1.,1.38187013346089));
#63037=CARTESIAN_POINT('Ctrl Pts',(-3.83845502790609,-1.,1.38230274828774));
#63038=CARTESIAN_POINT('Ctrl Pts',(-3.83845502790609,1.,1.38230274828774));
#63039=CARTESIAN_POINT('Ctrl Pts',(-3.83075266982138,-1.,1.38269750245086));
#63040=CARTESIAN_POINT('Ctrl Pts',(-3.83075266982138,1.,1.38269750245086));
#63041=CARTESIAN_POINT('Ctrl Pts',(-3.82305771743715,-1.,1.38305421262724));
#63042=CARTESIAN_POINT('Ctrl Pts',(-3.82305771743715,1.,1.38305421262724));
#63043=CARTESIAN_POINT('Ctrl Pts',(-3.81537060817765,-1.,1.38337263902766));
#63044=CARTESIAN_POINT('Ctrl Pts',(-3.81537060817765,1.,1.38337263902766));
#63045=CARTESIAN_POINT('Ctrl Pts',(-3.80769156398429,-1.,1.38365244046226));
#63046=CARTESIAN_POINT('Ctrl Pts',(-3.80769156398429,1.,1.38365244046226));
#63047=CARTESIAN_POINT('Ctrl Pts',(-3.80002044322169,-1.,1.38389311766701));
#63048=CARTESIAN_POINT('Ctrl Pts',(-3.80002044322169,1.,1.38389311766701));
#63049=CARTESIAN_POINT('Ctrl Pts',(-3.79235669640907,-1.,1.38409399694588));
#63050=CARTESIAN_POINT('Ctrl Pts',(-3.79235669640907,1.,1.38409399694588));
#63051=CARTESIAN_POINT('Ctrl Pts',(-3.78469969805134,-1.,1.38425435883773));
#63052=CARTESIAN_POINT('Ctrl Pts',(-3.78469969805134,1.,1.38425435883773));
#63053=CARTESIAN_POINT('Ctrl Pts',(-3.77704902230441,-1.,1.38437354551435));
#63054=CARTESIAN_POINT('Ctrl Pts',(-3.77704902230441,1.,1.38437354551435));
#63055=CARTESIAN_POINT('Ctrl Pts',(-3.76940473185775,-1.,1.38445107339517));
#63056=CARTESIAN_POINT('Ctrl Pts',(-3.76940473185775,1.,1.38445107339517));
#63057=CARTESIAN_POINT('Ctrl Pts',(-3.76176768271347,-1.,1.38448675253343));
#63058=CARTESIAN_POINT('Ctrl Pts',(-3.76176768271347,1.,1.38448675253343));
#63059=CARTESIAN_POINT('Ctrl Pts',(-3.75413976318727,-1.,1.38448077997155));
#63060=CARTESIAN_POINT('Ctrl Pts',(-3.75413976318727,1.,1.38448077997155));
#63061=CARTESIAN_POINT('Ctrl Pts',(-3.7465231716786,-1.,1.38443344984389));
#63062=CARTESIAN_POINT('Ctrl Pts',(-3.7465231716786,1.,1.38443344984389));
#63063=CARTESIAN_POINT('Ctrl Pts',(-3.73891976418099,-1.,1.38434489156456));
#63064=CARTESIAN_POINT('Ctrl Pts',(-3.73891976418099,1.,1.38434489156456));
#63065=CARTESIAN_POINT('Ctrl Pts',(-3.73133035859283,-1.,1.38421479111531));
#63066=CARTESIAN_POINT('Ctrl Pts',(-3.73133035859283,1.,1.38421479111531));
#63067=CARTESIAN_POINT('Ctrl Pts',(-3.72375409358805,-1.,1.3840421342895));
#63068=CARTESIAN_POINT('Ctrl Pts',(-3.72375409358805,1.,1.3840421342895));
#63069=CARTESIAN_POINT('Ctrl Pts',(-3.7161876605181,-1.,1.38382489984585));
#63070=CARTESIAN_POINT('Ctrl Pts',(-3.7161876605181,1.,1.38382489984585));
#63071=CARTESIAN_POINT('Ctrl Pts',(-3.70862680753343,-1.,1.38356065402122));
#63072=CARTESIAN_POINT('Ctrl Pts',(-3.70862680753343,1.,1.38356065402122));
#63073=CARTESIAN_POINT('Ctrl Pts',(-3.70106792167894,-1.,1.38324717612862));
#63074=CARTESIAN_POINT('Ctrl Pts',(-3.70106792167894,1.,1.38324717612862));
#63075=CARTESIAN_POINT('Ctrl Pts',(-3.69350967899523,-1.,1.38288311171649));
#63076=CARTESIAN_POINT('Ctrl Pts',(-3.69350967899523,1.,1.38288311171649));
#63077=CARTESIAN_POINT('Ctrl Pts',(-3.68595444983844,-1.,1.38246852827185));
#63078=CARTESIAN_POINT('Ctrl Pts',(-3.68595444983844,1.,1.38246852827185));
#63079=CARTESIAN_POINT('Ctrl Pts',(-3.6784103848243,-1.,1.38200574290626));
#63080=CARTESIAN_POINT('Ctrl Pts',(-3.6784103848243,1.,1.38200574290626));
#63081=CARTESIAN_POINT('Ctrl Pts',(-3.67088843112282,-1.,1.38149812653876));
#63082=CARTESIAN_POINT('Ctrl Pts',(-3.67088843112282,1.,1.38149812653876));
#63083=CARTESIAN_POINT('Ctrl Pts',(-3.66339848520874,-1.,1.38094856333558));
#63084=CARTESIAN_POINT('Ctrl Pts',(-3.66339848520874,1.,1.38094856333558));
#63085=CARTESIAN_POINT('Ctrl Pts',(-3.65594554404396,-1.,1.38035791051215));
#63086=CARTESIAN_POINT('Ctrl Pts',(-3.65594554404396,1.,1.38035791051215));
#63087=CARTESIAN_POINT('Ctrl Pts',(-3.64852652756444,-1.,1.37972372481598));
#63088=CARTESIAN_POINT('Ctrl Pts',(-3.64852652756444,1.,1.37972372481598));
#63089=CARTESIAN_POINT('Ctrl Pts',(-3.64112507791112,-1.,1.37903818567347));
#63090=CARTESIAN_POINT('Ctrl Pts',(-3.64112507791112,1.,1.37903818567347));
#63091=CARTESIAN_POINT('Ctrl Pts',(-3.63371727442448,-1.,1.37829035457324));
#63092=CARTESIAN_POINT('Ctrl Pts',(-3.63371727442448,1.,1.37829035457324));
#63093=CARTESIAN_POINT('Ctrl Pts',(-3.62628098665112,-1.,1.37746987919868));
#63094=CARTESIAN_POINT('Ctrl Pts',(-3.62628098665112,1.,1.37746987919868));
#63095=CARTESIAN_POINT('Ctrl Pts',(-3.61880481160408,-1.,1.37657053403102));
#63096=CARTESIAN_POINT('Ctrl Pts',(-3.61880481160408,1.,1.37657053403102));
#63097=CARTESIAN_POINT('Ctrl Pts',(-3.61129546591082,-1.,1.37559314436641));
#63098=CARTESIAN_POINT('Ctrl Pts',(-3.61129546591082,1.,1.37559314436641));
#63099=CARTESIAN_POINT('Ctrl Pts',(-3.60379020124038,-1.,1.37455051379642));
#63100=CARTESIAN_POINT('Ctrl Pts',(-3.60379020124038,1.,1.37455051379642));
#63101=CARTESIAN_POINT('Ctrl Pts',(-3.59634627869117,-1.,1.37346320103184));
#63102=CARTESIAN_POINT('Ctrl Pts',(-3.59634627869117,1.,1.37346320103184));
#63103=CARTESIAN_POINT('Ctrl Pts',(-3.5890185384643,-1.,1.37235053661));
#63104=CARTESIAN_POINT('Ctrl Pts',(-3.5890185384643,1.,1.37235053661));
#63105=CARTESIAN_POINT('Ctrl Pts',(-3.58183885982745,-1.,1.37122241663073));
#63106=CARTESIAN_POINT('Ctrl Pts',(-3.58183885982745,1.,1.37122241663073));
#63107=CARTESIAN_POINT('Ctrl Pts',(-3.57479875549453,-1.,1.37007229485646));
#63108=CARTESIAN_POINT('Ctrl Pts',(-3.57479875549453,1.,1.37007229485646));
#63109=CARTESIAN_POINT('Ctrl Pts',(-3.56782080304554,-1.,1.36886584973349));
#63110=CARTESIAN_POINT('Ctrl Pts',(-3.56782080304554,1.,1.36886584973349));
#63111=CARTESIAN_POINT('Ctrl Pts',(-3.56077662028492,-1.,1.36754771771174));
#63112=CARTESIAN_POINT('Ctrl Pts',(-3.56077662028492,1.,1.36754771771174));
#63113=CARTESIAN_POINT('Ctrl Pts',(-3.55353883995793,-1.,1.36606145456711));
#63114=CARTESIAN_POINT('Ctrl Pts',(-3.55353883995793,1.,1.36606145456711));
#63115=CARTESIAN_POINT('Ctrl Pts',(-3.54602591832893,-1.,1.36436666257567));
#63116=CARTESIAN_POINT('Ctrl Pts',(-3.54602591832893,1.,1.36436666257567));
#63117=CARTESIAN_POINT('Ctrl Pts',(-3.53824396425032,-1.,1.36245507339334));
#63118=CARTESIAN_POINT('Ctrl Pts',(-3.53824396425032,1.,1.36245507339334));
#63119=CARTESIAN_POINT('Ctrl Pts',(-3.53034464961849,-1.,1.36037259643827));
#63120=CARTESIAN_POINT('Ctrl Pts',(-3.53034464961849,1.,1.36037259643827));
#63121=CARTESIAN_POINT('Ctrl Pts',(-3.52261776117121,-1.,1.35821701528975));
#63122=CARTESIAN_POINT('Ctrl Pts',(-3.52261776117121,1.,1.35821701528975));
#63123=CARTESIAN_POINT('Ctrl Pts',(-3.51542230699919,-1.,1.35611275237288));
#63124=CARTESIAN_POINT('Ctrl Pts',(-3.51542230699919,1.,1.35611275237288));
#63125=CARTESIAN_POINT('Ctrl Pts',(-3.50913227060177,-1.,1.35419113576022));
#63126=CARTESIAN_POINT('Ctrl Pts',(-3.50913227060177,1.,1.35419113576022));
#63127=CARTESIAN_POINT('Ctrl Pts',(-3.50408168106113,-1.,1.3525703284343));
#63128=CARTESIAN_POINT('Ctrl Pts',(-3.50408168106113,1.,1.3525703284343));
#63129=CARTESIAN_POINT('Ctrl Pts',(-3.50049707063673,-1.,1.35133076331065));
#63130=CARTESIAN_POINT('Ctrl Pts',(-3.50049707063673,1.,1.35133076331065));
#63131=CARTESIAN_POINT('Ctrl Pts',(-3.49888720256612,-1.,1.35067437417289));
#63132=CARTESIAN_POINT('Ctrl Pts',(-3.49888720256612,1.,1.35067437417289));
#63133=CARTESIAN_POINT('Ctrl Pts',(-3.49840357193384,-1.,1.35037650302887));
#63134=CARTESIAN_POINT('Ctrl Pts',(-3.49840357193384,1.,1.35037650302887));
#63135=CARTESIAN_POINT('Ctrl Pts',(-3.49840260053616,-1.,1.35026426118351));
#63136=CARTESIAN_POINT('Ctrl Pts',(-3.49840260053616,1.,1.35026426118351));
#63137=CARTESIAN_POINT('Ctrl Pts',(-3.49848248301936,-1.,1.35022972712301));
#63138=CARTESIAN_POINT('Ctrl Pts',(-3.49848248301936,1.,1.35022972712301));
#63139=CARTESIAN_POINT('',(-3.97027773754922,1.,1.36999806084572));
#63140=CARTESIAN_POINT('Ctrl Pts',(-3.97027773754922,1.,1.36999806084572));
#63141=CARTESIAN_POINT('Ctrl Pts',(-3.9687184694173,1.,1.37020239094758));
#63142=CARTESIAN_POINT('Ctrl Pts',(-3.96560037975788,1.,1.37060761746027));
#63143=CARTESIAN_POINT('Ctrl Pts',(-3.96092458508407,1.,1.37120515615663));
#63144=CARTESIAN_POINT('Ctrl Pts',(-3.95469287283105,1.,1.37198126433139));
#63145=CARTESIAN_POINT('Ctrl Pts',(-3.94690771786926,1.,1.37291699203423));
#63146=CARTESIAN_POINT('Ctrl Pts',(-3.93912709041791,1.,1.37381821967499));
#63147=CARTESIAN_POINT('Ctrl Pts',(-3.93135106761941,1.,1.37468482215784));
#63148=CARTESIAN_POINT('Ctrl Pts',(-3.92357976987132,1.,1.37551664448057));
#63149=CARTESIAN_POINT('Ctrl Pts',(-3.91581337461825,1.,1.37631350505516));
#63150=CARTESIAN_POINT('Ctrl Pts',(-3.90805209522729,1.,1.3770751963376));
#63151=CARTESIAN_POINT('Ctrl Pts',(-3.90029615196255,1.,1.3778014851263));
#63152=CARTESIAN_POINT('Ctrl Pts',(-3.89254574338385,1.,1.37849211287981));
#63153=CARTESIAN_POINT('Ctrl Pts',(-3.88480102249461,1.,1.37914679719446));
#63154=CARTESIAN_POINT('Ctrl Pts',(-3.87706205830865,1.,1.37976523097187));
#63155=CARTESIAN_POINT('Ctrl Pts',(-3.86932885813403,1.,1.38034709213129));
#63156=CARTESIAN_POINT('Ctrl Pts',(-3.86160143044187,1.,1.38089205993067));
#63157=CARTESIAN_POINT('Ctrl Pts',(-3.85387983979557,1.,1.38139983115075));
#63158=CARTESIAN_POINT('Ctrl Pts',(-3.84616425605705,1.,1.38187013346089));
#63159=CARTESIAN_POINT('Ctrl Pts',(-3.83845502790609,1.,1.38230274828774));
#63160=CARTESIAN_POINT('Ctrl Pts',(-3.83075266982138,1.,1.38269750245086));
#63161=CARTESIAN_POINT('Ctrl Pts',(-3.82305771743715,1.,1.38305421262724));
#63162=CARTESIAN_POINT('Ctrl Pts',(-3.81537060817765,1.,1.38337263902766));
#63163=CARTESIAN_POINT('Ctrl Pts',(-3.80769156398429,1.,1.38365244046226));
#63164=CARTESIAN_POINT('Ctrl Pts',(-3.80002044322169,1.,1.38389311766701));
#63165=CARTESIAN_POINT('Ctrl Pts',(-3.79235669640907,1.,1.38409399694588));
#63166=CARTESIAN_POINT('Ctrl Pts',(-3.78469969805134,1.,1.38425435883773));
#63167=CARTESIAN_POINT('Ctrl Pts',(-3.77704902230441,1.,1.38437354551435));
#63168=CARTESIAN_POINT('Ctrl Pts',(-3.76940473185775,1.,1.38445107339517));
#63169=CARTESIAN_POINT('Ctrl Pts',(-3.76176768271347,1.,1.38448675253343));
#63170=CARTESIAN_POINT('Ctrl Pts',(-3.75413976318727,1.,1.38448077997155));
#63171=CARTESIAN_POINT('Ctrl Pts',(-3.7465231716786,1.,1.38443344984389));
#63172=CARTESIAN_POINT('Ctrl Pts',(-3.73891976418099,1.,1.38434489156456));
#63173=CARTESIAN_POINT('Ctrl Pts',(-3.73133035859283,1.,1.38421479111531));
#63174=CARTESIAN_POINT('Ctrl Pts',(-3.72375409358805,1.,1.3840421342895));
#63175=CARTESIAN_POINT('Ctrl Pts',(-3.7161876605181,1.,1.38382489984585));
#63176=CARTESIAN_POINT('Ctrl Pts',(-3.70862680753343,1.,1.38356065402122));
#63177=CARTESIAN_POINT('Ctrl Pts',(-3.70106792167894,1.,1.38324717612862));
#63178=CARTESIAN_POINT('Ctrl Pts',(-3.69350967899523,1.,1.38288311171649));
#63179=CARTESIAN_POINT('Ctrl Pts',(-3.68595444983844,1.,1.38246852827185));
#63180=CARTESIAN_POINT('Ctrl Pts',(-3.6784103848243,1.,1.38200574290626));
#63181=CARTESIAN_POINT('Ctrl Pts',(-3.67088843112282,1.,1.38149812653876));
#63182=CARTESIAN_POINT('Ctrl Pts',(-3.66339848520874,1.,1.38094856333558));
#63183=CARTESIAN_POINT('Ctrl Pts',(-3.65594554404396,1.,1.38035791051215));
#63184=CARTESIAN_POINT('Ctrl Pts',(-3.64852652756444,1.,1.37972372481598));
#63185=CARTESIAN_POINT('Ctrl Pts',(-3.64112507791112,1.,1.37903818567347));
#63186=CARTESIAN_POINT('Ctrl Pts',(-3.63371727442448,1.,1.37829035457324));
#63187=CARTESIAN_POINT('Ctrl Pts',(-3.62628098665112,1.,1.37746987919868));
#63188=CARTESIAN_POINT('Ctrl Pts',(-3.61880481160408,1.,1.37657053403102));
#63189=CARTESIAN_POINT('Ctrl Pts',(-3.61129546591082,1.,1.37559314436641));
#63190=CARTESIAN_POINT('Ctrl Pts',(-3.60379020124038,1.,1.37455051379642));
#63191=CARTESIAN_POINT('Ctrl Pts',(-3.59634627869117,1.,1.37346320103184));
#63192=CARTESIAN_POINT('Ctrl Pts',(-3.5890185384643,1.,1.37235053661));
#63193=CARTESIAN_POINT('Ctrl Pts',(-3.58183885982745,1.,1.37122241663073));
#63194=CARTESIAN_POINT('Ctrl Pts',(-3.57479875549453,1.,1.37007229485646));
#63195=CARTESIAN_POINT('Ctrl Pts',(-3.56782080304554,1.,1.36886584973349));
#63196=CARTESIAN_POINT('Ctrl Pts',(-3.56077662028492,1.,1.36754771771174));
#63197=CARTESIAN_POINT('Ctrl Pts',(-3.55353883995793,1.,1.36606145456711));
#63198=CARTESIAN_POINT('Ctrl Pts',(-3.54602591832893,1.,1.36436666257567));
#63199=CARTESIAN_POINT('Ctrl Pts',(-3.53824396425032,1.,1.36245507339334));
#63200=CARTESIAN_POINT('Ctrl Pts',(-3.53034464961849,1.,1.36037259643827));
#63201=CARTESIAN_POINT('Ctrl Pts',(-3.52261776117121,1.,1.35821701528975));
#63202=CARTESIAN_POINT('Ctrl Pts',(-3.51542230699919,1.,1.35611275237288));
#63203=CARTESIAN_POINT('Ctrl Pts',(-3.50913227060177,1.,1.35419113576022));
#63204=CARTESIAN_POINT('Ctrl Pts',(-3.50408168106113,1.,1.3525703284343));
#63205=CARTESIAN_POINT('Ctrl Pts',(-3.5007660381658,1.,1.35142377279535));
#63206=CARTESIAN_POINT('Ctrl Pts',(-3.49920025459856,1.,1.35080045218652));
#63207=CARTESIAN_POINT('Ctrl Pts',(-3.49861894124915,1.,1.35049736560633));
#63208=CARTESIAN_POINT('Ctrl Pts',(-3.49847119623841,1.,1.35036670893102));
#63209=CARTESIAN_POINT('Ctrl Pts',(-3.49844575334386,1.,1.35032489087269));
#63210=CARTESIAN_POINT('',(-3.97027773754922,0.,1.36999806084572));
#63211=CARTESIAN_POINT('Ctrl Pts',(-3.62397690409552,-1.,0.96399761336957));
#63212=CARTESIAN_POINT('Ctrl Pts',(-3.62397690409552,1.,0.96399761336957));
#63213=CARTESIAN_POINT('Ctrl Pts',(-3.62393257642191,-1.,0.963922720982576));
#63214=CARTESIAN_POINT('Ctrl Pts',(-3.62393257642191,1.,0.963922720982576));
#63215=CARTESIAN_POINT('Ctrl Pts',(-3.62399933640277,-1.,0.963832486396055));
#63216=CARTESIAN_POINT('Ctrl Pts',(-3.62399933640277,1.,0.963832486396055));
#63217=CARTESIAN_POINT('Ctrl Pts',(-3.62456568607055,-1.,0.963875774532102));
#63218=CARTESIAN_POINT('Ctrl Pts',(-3.62456568607055,1.,0.963875774532102));
#63219=CARTESIAN_POINT('Ctrl Pts',(-3.62625391255277,-1.,0.964291001274618));
#63220=CARTESIAN_POINT('Ctrl Pts',(-3.62625391255277,1.,0.964291001274618));
#63221=CARTESIAN_POINT('Ctrl Pts',(-3.62988252139998,-1.,0.965395153165716));
#63222=CARTESIAN_POINT('Ctrl Pts',(-3.62988252139998,1.,0.965395153165716));
#63223=CARTESIAN_POINT('Ctrl Pts',(-3.6349212208096,-1.,0.967052554540877));
#63224=CARTESIAN_POINT('Ctrl Pts',(-3.6349212208096,1.,0.967052554540877));
#63225=CARTESIAN_POINT('Ctrl Pts',(-3.64113946505393,-1.,0.969195124674829));
#63226=CARTESIAN_POINT('Ctrl Pts',(-3.64113946505393,1.,0.969195124674829));
#63227=CARTESIAN_POINT('Ctrl Pts',(-3.64819756447072,-1.,0.971722122060277));
#63228=CARTESIAN_POINT('Ctrl Pts',(-3.64819756447072,1.,0.971722122060277));
#63229=CARTESIAN_POINT('Ctrl Pts',(-3.6557157673487,-1.,0.974519971354138));
#63230=CARTESIAN_POINT('Ctrl Pts',(-3.6557157673487,1.,0.974519971354138));
#63231=CARTESIAN_POINT('Ctrl Pts',(-3.66333049637403,-1.,0.977478312751416));
#63232=CARTESIAN_POINT('Ctrl Pts',(-3.66333049637403,1.,0.977478312751416));
#63233=CARTESIAN_POINT('Ctrl Pts',(-3.67074983340444,-1.,0.980505922458494));
#63234=CARTESIAN_POINT('Ctrl Pts',(-3.67074983340444,1.,0.980505922458494));
#63235=CARTESIAN_POINT('Ctrl Pts',(-3.67782408841876,-1.,0.983550791470864));
#63236=CARTESIAN_POINT('Ctrl Pts',(-3.67782408841876,1.,0.983550791470864));
#63237=CARTESIAN_POINT('Ctrl Pts',(-3.6845531792623,-1.,0.986602639864285));
#63238=CARTESIAN_POINT('Ctrl Pts',(-3.6845531792623,1.,0.986602639864285));
#63239=CARTESIAN_POINT('Ctrl Pts',(-3.69102682138955,-1.,0.989676715398858));
#63240=CARTESIAN_POINT('Ctrl Pts',(-3.69102682138955,1.,0.989676715398858));
#63241=CARTESIAN_POINT('Ctrl Pts',(-3.69738123415696,-1.,0.992802218332103));
#63242=CARTESIAN_POINT('Ctrl Pts',(-3.69738123415696,1.,0.992802218332103));
#63243=CARTESIAN_POINT('Ctrl Pts',(-3.70375282282107,-1.,0.996009819772431));
#63244=CARTESIAN_POINT('Ctrl Pts',(-3.70375282282107,1.,0.996009819772431));
#63245=CARTESIAN_POINT('Ctrl Pts',(-3.7102243971387,-1.,0.999317260756344));
#63246=CARTESIAN_POINT('Ctrl Pts',(-3.7102243971387,1.,0.999317260756344));
#63247=CARTESIAN_POINT('Ctrl Pts',(-3.71680667125047,-1.,1.00272423396802));
#63248=CARTESIAN_POINT('Ctrl Pts',(-3.71680667125047,1.,1.00272423396802));
#63249=CARTESIAN_POINT('Ctrl Pts',(-3.72346803750544,-1.,1.00622000735696));
#63250=CARTESIAN_POINT('Ctrl Pts',(-3.72346803750544,1.,1.00622000735696));
#63251=CARTESIAN_POINT('Ctrl Pts',(-3.73015276704407,-1.,1.00978798539491));
#63252=CARTESIAN_POINT('Ctrl Pts',(-3.73015276704407,1.,1.00978798539491));
#63253=CARTESIAN_POINT('Ctrl Pts',(-3.73680245055747,-1.,1.01341114319906));
#63254=CARTESIAN_POINT('Ctrl Pts',(-3.73680245055747,1.,1.01341114319906));
#63255=CARTESIAN_POINT('Ctrl Pts',(-3.74337942504993,-1.,1.01707794311088));
#63256=CARTESIAN_POINT('Ctrl Pts',(-3.74337942504993,1.,1.01707794311088));
#63257=CARTESIAN_POINT('Ctrl Pts',(-3.74987777155873,-1.,1.02078510487439));
#63258=CARTESIAN_POINT('Ctrl Pts',(-3.74987777155873,1.,1.02078510487439));
#63259=CARTESIAN_POINT('Ctrl Pts',(-3.75631037456224,-1.,1.02453429444668));
#63260=CARTESIAN_POINT('Ctrl Pts',(-3.75631037456224,1.,1.02453429444668));
#63261=CARTESIAN_POINT('Ctrl Pts',(-3.76270122291245,-1.,1.02833014458184));
#63262=CARTESIAN_POINT('Ctrl Pts',(-3.76270122291245,1.,1.02833014458184));
#63263=CARTESIAN_POINT('Ctrl Pts',(-3.76907609832516,-1.,1.03217786604919));
#63264=CARTESIAN_POINT('Ctrl Pts',(-3.76907609832516,1.,1.03217786604919));
#63265=CARTESIAN_POINT('Ctrl Pts',(-3.77545283140427,-1.,1.03608074678008));
#63266=CARTESIAN_POINT('Ctrl Pts',(-3.77545283140427,1.,1.03608074678008));
#63267=CARTESIAN_POINT('Ctrl Pts',(-3.7818353500817,-1.,1.04003862055798));
#63268=CARTESIAN_POINT('Ctrl Pts',(-3.7818353500817,1.,1.04003862055798));
#63269=CARTESIAN_POINT('Ctrl Pts',(-3.78821910787179,-1.,1.04404924374422));
#63270=CARTESIAN_POINT('Ctrl Pts',(-3.78821910787179,1.,1.04404924374422));
#63271=CARTESIAN_POINT('Ctrl Pts',(-3.79459440308786,-1.,1.04810913267639));
#63272=CARTESIAN_POINT('Ctrl Pts',(-3.79459440308786,1.,1.04810913267639));
#63273=CARTESIAN_POINT('Ctrl Pts',(-3.80095039790681,-1.,1.05221457990016));
#63274=CARTESIAN_POINT('Ctrl Pts',(-3.80095039790681,1.,1.05221457990016));
#63275=CARTESIAN_POINT('Ctrl Pts',(-3.80727913637791,-1.,1.05636266918644));
#63276=CARTESIAN_POINT('Ctrl Pts',(-3.80727913637791,1.,1.05636266918644));
#63277=CARTESIAN_POINT('Ctrl Pts',(-3.8135786611749,-1.,1.06055206187299));
#63278=CARTESIAN_POINT('Ctrl Pts',(-3.8135786611749,1.,1.06055206187299));
#63279=CARTESIAN_POINT('Ctrl Pts',(-3.81985083953012,-1.,1.0647824403893));
#63280=CARTESIAN_POINT('Ctrl Pts',(-3.81985083953012,1.,1.0647824403893));
#63281=CARTESIAN_POINT('Ctrl Pts',(-3.82609989967276,-1.,1.06905413180359));
#63282=CARTESIAN_POINT('Ctrl Pts',(-3.82609989967276,1.,1.06905413180359));
#63283=CARTESIAN_POINT('Ctrl Pts',(-3.83233071195144,-1.,1.07336766633459));
#63284=CARTESIAN_POINT('Ctrl Pts',(-3.83233071195144,1.,1.07336766633459));
#63285=CARTESIAN_POINT('Ctrl Pts',(-3.83854714117491,-1.,1.07772335353858));
#63286=CARTESIAN_POINT('Ctrl Pts',(-3.83854714117491,1.,1.07772335353858));
#63287=CARTESIAN_POINT('Ctrl Pts',(-3.8447504803063,-1.,1.08212087917991));
#63288=CARTESIAN_POINT('Ctrl Pts',(-3.8447504803063,1.,1.08212087917991));
#63289=CARTESIAN_POINT('Ctrl Pts',(-3.85094025222713,-1.,1.08655950846384));
#63290=CARTESIAN_POINT('Ctrl Pts',(-3.85094025222713,1.,1.08655950846384));
#63291=CARTESIAN_POINT('Ctrl Pts',(-3.85711487933931,-1.,1.09103825516294));
#63292=CARTESIAN_POINT('Ctrl Pts',(-3.85711487933931,1.,1.09103825516294));
#63293=CARTESIAN_POINT('Ctrl Pts',(-3.86327241021247,-1.,1.09555606505013));
#63294=CARTESIAN_POINT('Ctrl Pts',(-3.86327241021247,1.,1.09555606505013));
#63295=CARTESIAN_POINT('Ctrl Pts',(-3.86941120134849,-1.,1.10011198761195));
#63296=CARTESIAN_POINT('Ctrl Pts',(-3.86941120134849,1.,1.10011198761195));
#63297=CARTESIAN_POINT('Ctrl Pts',(-3.87553067187514,-1.,1.10470536603287));
#63298=CARTESIAN_POINT('Ctrl Pts',(-3.87553067187514,1.,1.10470536603287));
#63299=CARTESIAN_POINT('Ctrl Pts',(-3.88163105531724,-1.,1.10933577224008));
#63300=CARTESIAN_POINT('Ctrl Pts',(-3.88163105531724,1.,1.10933577224008));
#63301=CARTESIAN_POINT('Ctrl Pts',(-3.88771308285171,-1.,1.11400292434429));
#63302=CARTESIAN_POINT('Ctrl Pts',(-3.88771308285171,1.,1.11400292434429));
#63303=CARTESIAN_POINT('Ctrl Pts',(-3.89377768340344,-1.,1.11870660794603));
#63304=CARTESIAN_POINT('Ctrl Pts',(-3.89377768340344,1.,1.11870660794603));
#63305=CARTESIAN_POINT('Ctrl Pts',(-3.89982569750025,-1.,1.12344660099043));
#63306=CARTESIAN_POINT('Ctrl Pts',(-3.89982569750025,1.,1.12344660099043));
#63307=CARTESIAN_POINT('Ctrl Pts',(-3.90585753318737,-1.,1.12822258281553));
#63308=CARTESIAN_POINT('Ctrl Pts',(-3.90585753318737,1.,1.12822258281553));
#63309=CARTESIAN_POINT('Ctrl Pts',(-3.91187321145649,-1.,1.13303414693896));
#63310=CARTESIAN_POINT('Ctrl Pts',(-3.91187321145649,1.,1.13303414693896));
#63311=CARTESIAN_POINT('Ctrl Pts',(-3.91787251936827,-1.,1.13788084225554));
#63312=CARTESIAN_POINT('Ctrl Pts',(-3.91787251936827,1.,1.13788084225554));
#63313=CARTESIAN_POINT('Ctrl Pts',(-3.92385513133997,-1.,1.14276220561593));
#63314=CARTESIAN_POINT('Ctrl Pts',(-3.92385513133997,1.,1.14276220561593));
#63315=CARTESIAN_POINT('Ctrl Pts',(-3.92982073294257,-1.,1.14767779451123));
#63316=CARTESIAN_POINT('Ctrl Pts',(-3.92982073294257,1.,1.14767779451123));
#63317=CARTESIAN_POINT('Ctrl Pts',(-3.9357691705628,-1.,1.1526272271632));
#63318=CARTESIAN_POINT('Ctrl Pts',(-3.9357691705628,1.,1.1526272271632));
#63319=CARTESIAN_POINT('Ctrl Pts',(-3.94170046685203,-1.,1.15761018340956));
#63320=CARTESIAN_POINT('Ctrl Pts',(-3.94170046685203,1.,1.15761018340956));
#63321=CARTESIAN_POINT('Ctrl Pts',(-3.94761474780583,-1.,1.16262637999157));
#63322=CARTESIAN_POINT('Ctrl Pts',(-3.94761474780583,1.,1.16262637999157));
#63323=CARTESIAN_POINT('Ctrl Pts',(-3.95351219509876,-1.,1.16767555244438));
#63324=CARTESIAN_POINT('Ctrl Pts',(-3.95351219509876,1.,1.16767555244438));
#63325=CARTESIAN_POINT('Ctrl Pts',(-3.95939299213276,-1.,1.17275743590361));
#63326=CARTESIAN_POINT('Ctrl Pts',(-3.95939299213276,1.,1.17275743590361));
#63327=CARTESIAN_POINT('Ctrl Pts',(-3.96525726358159,-1.,1.17787174135592));
#63328=CARTESIAN_POINT('Ctrl Pts',(-3.96525726358159,1.,1.17787174135592));
#63329=CARTESIAN_POINT('Ctrl Pts',(-3.97110505165415,-1.,1.18301815039831));
#63330=CARTESIAN_POINT('Ctrl Pts',(-3.97110505165415,1.,1.18301815039831));
#63331=CARTESIAN_POINT('Ctrl Pts',(-3.97693634767754,-1.,1.18819633715539));
#63332=CARTESIAN_POINT('Ctrl Pts',(-3.97693634767754,1.,1.18819633715539));
#63333=CARTESIAN_POINT('Ctrl Pts',(-3.98275111052561,-1.,1.19340598349475));
#63334=CARTESIAN_POINT('Ctrl Pts',(-3.98275111052561,1.,1.19340598349475));
#63335=CARTESIAN_POINT('Ctrl Pts',(-3.98854928957189,-1.,1.19864679609566));
#63336=CARTESIAN_POINT('Ctrl Pts',(-3.98854928957189,1.,1.19864679609566));
#63337=CARTESIAN_POINT('Ctrl Pts',(-3.99433084799666,-1.,1.20391852375139));
#63338=CARTESIAN_POINT('Ctrl Pts',(-3.99433084799666,1.,1.20391852375139));
#63339=CARTESIAN_POINT('Ctrl Pts',(-4.00009577950721,-1.,1.20922097029551));
#63340=CARTESIAN_POINT('Ctrl Pts',(-4.00009577950721,1.,1.20922097029551));
#63341=CARTESIAN_POINT('Ctrl Pts',(-4.00584409522722,-1.,1.21455398918133));
#63342=CARTESIAN_POINT('Ctrl Pts',(-4.00584409522722,1.,1.21455398918133));
#63343=CARTESIAN_POINT('Ctrl Pts',(-4.01042947140789,-1.,1.21884478244403));
#63344=CARTESIAN_POINT('Ctrl Pts',(-4.01042947140789,1.,1.21884478244403));
#63345=CARTESIAN_POINT('Ctrl Pts',(-4.01386104433519,-1.,1.22207656455845));
#63346=CARTESIAN_POINT('Ctrl Pts',(-4.01386104433519,1.,1.22207656455845));
#63347=CARTESIAN_POINT('Ctrl Pts',(-4.01614544569895,-1.,1.22423716681317));
#63348=CARTESIAN_POINT('Ctrl Pts',(-4.01614544569895,1.,1.22423716681317));
#63349=CARTESIAN_POINT('Ctrl Pts',(-4.01728681790024,-1.,1.22531898815164));
#63350=CARTESIAN_POINT('Ctrl Pts',(-4.01728681790024,1.,1.22531898815164));
#63351=CARTESIAN_POINT('',(-3.62400312501199,1.,0.963899035118986));
#63352=CARTESIAN_POINT('Ctrl Pts',(-3.62400312501199,-1.,0.963899035118986));
#63353=CARTESIAN_POINT('Ctrl Pts',(-3.62400312501199,-0.666666666666667,
0.963899035118986));
#63354=CARTESIAN_POINT('Ctrl Pts',(-3.62400312501199,-0.333333333333333,
0.963899035118986));
#63355=CARTESIAN_POINT('Ctrl Pts',(-3.62400312501199,0.333333333333333,
0.963899035118986));
#63356=CARTESIAN_POINT('Ctrl Pts',(-3.62400312501199,0.666666666666667,
0.963899035118985));
#63357=CARTESIAN_POINT('Ctrl Pts',(-3.62400312501199,1.,0.963899035118985));
#63358=CARTESIAN_POINT('',(-4.01728681790024,1.,1.22531898815164));
#63359=CARTESIAN_POINT('',(-4.01728681790024,0.,1.22531898815164));
#63360=CARTESIAN_POINT('Ctrl Pts',(-3.62400312501199,1.,0.963899035118985));
#63361=CARTESIAN_POINT('Ctrl Pts',(-3.62404828878374,1.,0.963880158556713));
#63362=CARTESIAN_POINT('Ctrl Pts',(-3.62424461507455,1.,0.963861297423579));
#63363=CARTESIAN_POINT('Ctrl Pts',(-3.62489305727516,1.,0.963957782642589));
#63364=CARTESIAN_POINT('Ctrl Pts',(-3.62652618145252,1.,0.964373850166081));
#63365=CARTESIAN_POINT('Ctrl Pts',(-3.62988252139998,1.,0.965395153165716));
#63366=CARTESIAN_POINT('Ctrl Pts',(-3.6349212208096,1.,0.967052554540877));
#63367=CARTESIAN_POINT('Ctrl Pts',(-3.64113946505393,1.,0.969195124674829));
#63368=CARTESIAN_POINT('Ctrl Pts',(-3.64819756447072,1.,0.971722122060277));
#63369=CARTESIAN_POINT('Ctrl Pts',(-3.6557157673487,1.,0.974519971354138));
#63370=CARTESIAN_POINT('Ctrl Pts',(-3.66333049637403,1.,0.977478312751416));
#63371=CARTESIAN_POINT('Ctrl Pts',(-3.67074983340444,1.,0.980505922458494));
#63372=CARTESIAN_POINT('Ctrl Pts',(-3.67782408841876,1.,0.983550791470864));
#63373=CARTESIAN_POINT('Ctrl Pts',(-3.6845531792623,1.,0.986602639864285));
#63374=CARTESIAN_POINT('Ctrl Pts',(-3.69102682138955,1.,0.989676715398858));
#63375=CARTESIAN_POINT('Ctrl Pts',(-3.69738123415696,1.,0.992802218332103));
#63376=CARTESIAN_POINT('Ctrl Pts',(-3.70375282282107,1.,0.996009819772431));
#63377=CARTESIAN_POINT('Ctrl Pts',(-3.7102243971387,1.,0.999317260756344));
#63378=CARTESIAN_POINT('Ctrl Pts',(-3.71680667125047,1.,1.00272423396802));
#63379=CARTESIAN_POINT('Ctrl Pts',(-3.72346803750544,1.,1.00622000735696));
#63380=CARTESIAN_POINT('Ctrl Pts',(-3.73015276704407,1.,1.00978798539491));
#63381=CARTESIAN_POINT('Ctrl Pts',(-3.73680245055747,1.,1.01341114319906));
#63382=CARTESIAN_POINT('Ctrl Pts',(-3.74337942504993,1.,1.01707794311088));
#63383=CARTESIAN_POINT('Ctrl Pts',(-3.74987777155873,1.,1.02078510487439));
#63384=CARTESIAN_POINT('Ctrl Pts',(-3.75631037456224,1.,1.02453429444668));
#63385=CARTESIAN_POINT('Ctrl Pts',(-3.76270122291245,1.,1.02833014458184));
#63386=CARTESIAN_POINT('Ctrl Pts',(-3.76907609832516,1.,1.03217786604919));
#63387=CARTESIAN_POINT('Ctrl Pts',(-3.77545283140427,1.,1.03608074678008));
#63388=CARTESIAN_POINT('Ctrl Pts',(-3.7818353500817,1.,1.04003862055798));
#63389=CARTESIAN_POINT('Ctrl Pts',(-3.78821910787179,1.,1.04404924374422));
#63390=CARTESIAN_POINT('Ctrl Pts',(-3.79459440308786,1.,1.04810913267639));
#63391=CARTESIAN_POINT('Ctrl Pts',(-3.80095039790681,1.,1.05221457990016));
#63392=CARTESIAN_POINT('Ctrl Pts',(-3.80727913637791,1.,1.05636266918644));
#63393=CARTESIAN_POINT('Ctrl Pts',(-3.8135786611749,1.,1.06055206187299));
#63394=CARTESIAN_POINT('Ctrl Pts',(-3.81985083953012,1.,1.0647824403893));
#63395=CARTESIAN_POINT('Ctrl Pts',(-3.82609989967276,1.,1.06905413180359));
#63396=CARTESIAN_POINT('Ctrl Pts',(-3.83233071195144,1.,1.07336766633459));
#63397=CARTESIAN_POINT('Ctrl Pts',(-3.83854714117491,1.,1.07772335353858));
#63398=CARTESIAN_POINT('Ctrl Pts',(-3.8447504803063,1.,1.08212087917991));
#63399=CARTESIAN_POINT('Ctrl Pts',(-3.85094025222713,1.,1.08655950846384));
#63400=CARTESIAN_POINT('Ctrl Pts',(-3.85711487933931,1.,1.09103825516294));
#63401=CARTESIAN_POINT('Ctrl Pts',(-3.86327241021247,1.,1.09555606505013));
#63402=CARTESIAN_POINT('Ctrl Pts',(-3.86941120134849,1.,1.10011198761195));
#63403=CARTESIAN_POINT('Ctrl Pts',(-3.87553067187514,1.,1.10470536603287));
#63404=CARTESIAN_POINT('Ctrl Pts',(-3.88163105531724,1.,1.10933577224008));
#63405=CARTESIAN_POINT('Ctrl Pts',(-3.88771308285171,1.,1.11400292434429));
#63406=CARTESIAN_POINT('Ctrl Pts',(-3.89377768340344,1.,1.11870660794603));
#63407=CARTESIAN_POINT('Ctrl Pts',(-3.89982569750025,1.,1.12344660099043));
#63408=CARTESIAN_POINT('Ctrl Pts',(-3.90585753318737,1.,1.12822258281553));
#63409=CARTESIAN_POINT('Ctrl Pts',(-3.91187321145649,1.,1.13303414693896));
#63410=CARTESIAN_POINT('Ctrl Pts',(-3.91787251936827,1.,1.13788084225554));
#63411=CARTESIAN_POINT('Ctrl Pts',(-3.92385513133997,1.,1.14276220561593));
#63412=CARTESIAN_POINT('Ctrl Pts',(-3.92982073294257,1.,1.14767779451123));
#63413=CARTESIAN_POINT('Ctrl Pts',(-3.9357691705628,1.,1.1526272271632));
#63414=CARTESIAN_POINT('Ctrl Pts',(-3.94170046685203,1.,1.15761018340956));
#63415=CARTESIAN_POINT('Ctrl Pts',(-3.94761474780583,1.,1.16262637999157));
#63416=CARTESIAN_POINT('Ctrl Pts',(-3.95351219509876,1.,1.16767555244438));
#63417=CARTESIAN_POINT('Ctrl Pts',(-3.95939299213276,1.,1.17275743590361));
#63418=CARTESIAN_POINT('Ctrl Pts',(-3.96525726358159,1.,1.17787174135592));
#63419=CARTESIAN_POINT('Ctrl Pts',(-3.97110505165415,1.,1.18301815039831));
#63420=CARTESIAN_POINT('Ctrl Pts',(-3.97693634767754,1.,1.18819633715539));
#63421=CARTESIAN_POINT('Ctrl Pts',(-3.98275111052561,1.,1.19340598349475));
#63422=CARTESIAN_POINT('Ctrl Pts',(-3.98854928957189,1.,1.19864679609566));
#63423=CARTESIAN_POINT('Ctrl Pts',(-3.99433084799666,1.,1.20391852375139));
#63424=CARTESIAN_POINT('Ctrl Pts',(-4.00009577950721,1.,1.20922097029551));
#63425=CARTESIAN_POINT('Ctrl Pts',(-4.00584409522722,1.,1.21455398918133));
#63426=CARTESIAN_POINT('Ctrl Pts',(-4.01042947140789,1.,1.21884478244403));
#63427=CARTESIAN_POINT('Ctrl Pts',(-4.01386104433519,1.,1.22207656455845));
#63428=CARTESIAN_POINT('Ctrl Pts',(-4.01614544569895,1.,1.22423716681317));
#63429=CARTESIAN_POINT('Ctrl Pts',(-4.01728681790024,1.,1.22531898815164));
#63430=CARTESIAN_POINT('Origin',(-4.01728681790024,0.,1.22531898815164));
#63431=CARTESIAN_POINT('',(-3.97027773754922,1.,1.36999806084572));
#63432=CARTESIAN_POINT('Origin',(0.,0.,0.));
#63433=CARTESIAN_POINT('',(-3.66661143271648,1.,0.786422660833743));
#63434=CARTESIAN_POINT('Origin',(0.,1.,0.));
#63435=CARTESIAN_POINT('Ctrl Pts',(-3.66661143271648,1.,0.786422660833743));
#63436=CARTESIAN_POINT('Ctrl Pts',(-3.66661143271648,0.666666666666667,
0.786422660833743));
#63437=CARTESIAN_POINT('Ctrl Pts',(-3.66661143271648,0.333333333333333,
0.786422660833743));
#63438=CARTESIAN_POINT('Ctrl Pts',(-3.66661143271648,-0.333333333333333,
0.786422660833743));
#63439=CARTESIAN_POINT('Ctrl Pts',(-3.66661143271648,-0.666666666666667,
0.786422660833743));
#63440=CARTESIAN_POINT('Ctrl Pts',(-3.66661143271648,-1.,0.786422660833743));
#63441=CARTESIAN_POINT('Ctrl Pts',(-4.13571194405636,-1.,0.732042837400619));
#63442=CARTESIAN_POINT('Ctrl Pts',(-4.13571194405636,1.,0.732042837400619));
#63443=CARTESIAN_POINT('Ctrl Pts',(-4.13420383737278,-1.,0.732488575135926));
#63444=CARTESIAN_POINT('Ctrl Pts',(-4.13420383737278,1.,0.732488575135926));
#63445=CARTESIAN_POINT('Ctrl Pts',(-4.13118752796397,-1.,0.733376589325634));
#63446=CARTESIAN_POINT('Ctrl Pts',(-4.13118752796397,1.,0.733376589325634));
#63447=CARTESIAN_POINT('Ctrl Pts',(-4.12666277572794,-1.,0.734698226767512));
#63448=CARTESIAN_POINT('Ctrl Pts',(-4.12666277572794,1.,0.734698226767512));
#63449=CARTESIAN_POINT('Ctrl Pts',(-4.12062919626082,-1.,0.736439634335347));
#63450=CARTESIAN_POINT('Ctrl Pts',(-4.12062919626082,1.,0.736439634335347));
#63451=CARTESIAN_POINT('Ctrl Pts',(-4.11308626953795,-1.,0.738581708229118));
#63452=CARTESIAN_POINT('Ctrl Pts',(-4.11308626953795,1.,0.738581708229118));
#63453=CARTESIAN_POINT('Ctrl Pts',(-4.1055424175856,-1.,0.740688998555151));
#63454=CARTESIAN_POINT('Ctrl Pts',(-4.1055424175856,1.,0.740688998555151));
#63455=CARTESIAN_POINT('Ctrl Pts',(-4.09799769702712,-1.,0.742761369690017));
#63456=CARTESIAN_POINT('Ctrl Pts',(-4.09799769702712,1.,0.742761369690017));
#63457=CARTESIAN_POINT('Ctrl Pts',(-4.09045220253011,-1.,0.744798649705514));
#63458=CARTESIAN_POINT('Ctrl Pts',(-4.09045220253011,1.,0.744798649705514));
#63459=CARTESIAN_POINT('Ctrl Pts',(-4.08290608094789,-1.,0.746800631490821));
#63460=CARTESIAN_POINT('Ctrl Pts',(-4.08290608094789,1.,0.746800631490821));
#63461=CARTESIAN_POINT('Ctrl Pts',(-4.07535951055363,-1.,0.748767076679177));
#63462=CARTESIAN_POINT('Ctrl Pts',(-4.07535951055363,1.,0.748767076679177));
#63463=CARTESIAN_POINT('Ctrl Pts',(-4.06781267241886,-1.,0.750697720483175));
#63464=CARTESIAN_POINT('Ctrl Pts',(-4.06781267241886,1.,0.750697720483175));
#63465=CARTESIAN_POINT('Ctrl Pts',(-4.06026572221399,-1.,0.752592276482869));
#63466=CARTESIAN_POINT('Ctrl Pts',(-4.06026572221399,1.,0.752592276482869));
#63467=CARTESIAN_POINT('Ctrl Pts',(-4.05271876688106,-1.,0.754450441816411));
#63468=CARTESIAN_POINT('Ctrl Pts',(-4.05271876688106,1.,0.754450441816411));
#63469=CARTESIAN_POINT('Ctrl Pts',(-4.04517182654344,-1.,0.756271902370186));
#63470=CARTESIAN_POINT('Ctrl Pts',(-4.04517182654344,1.,0.756271902370186));
#63471=CARTESIAN_POINT('Ctrl Pts',(-4.03762485803468,-1.,0.758056338885553));
#63472=CARTESIAN_POINT('Ctrl Pts',(-4.03762485803468,1.,0.758056338885553));
#63473=CARTESIAN_POINT('Ctrl Pts',(-4.0300778195465,-1.,0.759803433244166));
#63474=CARTESIAN_POINT('Ctrl Pts',(-4.0300778195465,1.,0.759803433244166));
#63475=CARTESIAN_POINT('Ctrl Pts',(-4.02253072741347,-1.,0.761512875859941));
#63476=CARTESIAN_POINT('Ctrl Pts',(-4.02253072741347,1.,0.761512875859941));
#63477=CARTESIAN_POINT('Ctrl Pts',(-4.01498370680434,-1.,0.763184371182826));
#63478=CARTESIAN_POINT('Ctrl Pts',(-4.01498370680434,1.,0.763184371182826));
#63479=CARTESIAN_POINT('Ctrl Pts',(-4.00743706791366,-1.,0.764817648784946));
#63480=CARTESIAN_POINT('Ctrl Pts',(-4.00743706791366,1.,0.764817648784946));
#63481=CARTESIAN_POINT('Ctrl Pts',(-3.99989129179464,-1.,0.766412457135785));
#63482=CARTESIAN_POINT('Ctrl Pts',(-3.99989129179464,1.,0.766412457135785));
#63483=CARTESIAN_POINT('Ctrl Pts',(-3.99234687880892,-1.,0.767968531377708));
#63484=CARTESIAN_POINT('Ctrl Pts',(-3.99234687880892,1.,0.767968531377708));
#63485=CARTESIAN_POINT('Ctrl Pts',(-3.98480422348403,-1.,0.769485566245459));
#63486=CARTESIAN_POINT('Ctrl Pts',(-3.98480422348403,1.,0.769485566245459));
#63487=CARTESIAN_POINT('Ctrl Pts',(-3.97726349165507,-1.,0.770963190030503));
#63488=CARTESIAN_POINT('Ctrl Pts',(-3.97726349165507,1.,0.770963190030503));
#63489=CARTESIAN_POINT('Ctrl Pts',(-3.96972446532832,-1.,0.772400931772238));
#63490=CARTESIAN_POINT('Ctrl Pts',(-3.96972446532832,1.,0.772400931772238));
#63491=CARTESIAN_POINT('Ctrl Pts',(-3.96218649639876,-1.,0.773798212026682));
#63492=CARTESIAN_POINT('Ctrl Pts',(-3.96218649639876,1.,0.773798212026682));
#63493=CARTESIAN_POINT('Ctrl Pts',(-3.95464885452364,-1.,0.775154418039441));
#63494=CARTESIAN_POINT('Ctrl Pts',(-3.95464885452364,1.,0.775154418039441));
#63495=CARTESIAN_POINT('Ctrl Pts',(-3.94711101619471,-1.,0.77646896669796));
#63496=CARTESIAN_POINT('Ctrl Pts',(-3.94711101619471,1.,0.77646896669796));
#63497=CARTESIAN_POINT('Ctrl Pts',(-3.93957296768098,-1.,0.777741370568549));
#63498=CARTESIAN_POINT('Ctrl Pts',(-3.93957296768098,1.,0.777741370568549));
#63499=CARTESIAN_POINT('Ctrl Pts',(-3.93203552473153,-1.,0.778971308134786));
#63500=CARTESIAN_POINT('Ctrl Pts',(-3.93203552473153,1.,0.778971308134786));
#63501=CARTESIAN_POINT('Ctrl Pts',(-3.92450058323799,-1.,0.780158678615506));
#63502=CARTESIAN_POINT('Ctrl Pts',(-3.92450058323799,1.,0.780158678615506));
#63503=CARTESIAN_POINT('Ctrl Pts',(-3.9169703605466,-1.,0.781303428618343));
#63504=CARTESIAN_POINT('Ctrl Pts',(-3.9169703605466,1.,0.781303428618343));
#63505=CARTESIAN_POINT('Ctrl Pts',(-3.90944671004536,-1.,0.782405395622758));
#63506=CARTESIAN_POINT('Ctrl Pts',(-3.90944671004536,1.,0.782405395622758));
#63507=CARTESIAN_POINT('Ctrl Pts',(-3.90193039043971,-1.,0.783464141529082));
#63508=CARTESIAN_POINT('Ctrl Pts',(-3.90193039043971,1.,0.783464141529082));
#63509=CARTESIAN_POINT('Ctrl Pts',(-3.89442039235105,-1.,0.784478799358335));
#63510=CARTESIAN_POINT('Ctrl Pts',(-3.89442039235105,1.,0.784478799358335));
#63511=CARTESIAN_POINT('Ctrl Pts',(-3.88691313167399,-1.,0.785447890340723));
#63512=CARTESIAN_POINT('Ctrl Pts',(-3.88691313167399,1.,0.785447890340723));
#63513=CARTESIAN_POINT('Ctrl Pts',(-3.87940402818186,-1.,0.786369675812592));
#63514=CARTESIAN_POINT('Ctrl Pts',(-3.87940402818186,1.,0.786369675812592));
#63515=CARTESIAN_POINT('Ctrl Pts',(-3.87188916600905,-1.,0.78724252761798));
#63516=CARTESIAN_POINT('Ctrl Pts',(-3.87188916600905,1.,0.78724252761798));
#63517=CARTESIAN_POINT('Ctrl Pts',(-3.86436702561342,-1.,0.788065315093771));
#63518=CARTESIAN_POINT('Ctrl Pts',(-3.86436702561342,1.,0.788065315093771));
#63519=CARTESIAN_POINT('Ctrl Pts',(-3.85683995872536,-1.,0.788837734090688));
#63520=CARTESIAN_POINT('Ctrl Pts',(-3.85683995872536,1.,0.788837734090688));
#63521=CARTESIAN_POINT('Ctrl Pts',(-3.8493163780891,-1.,0.789560798155618));
#63522=CARTESIAN_POINT('Ctrl Pts',(-3.8493163780891,1.,0.789560798155618));
#63523=CARTESIAN_POINT('Ctrl Pts',(-3.84180762342476,-1.,0.790236124191289));
#63524=CARTESIAN_POINT('Ctrl Pts',(-3.84180762342476,1.,0.790236124191289));
#63525=CARTESIAN_POINT('Ctrl Pts',(-3.83432392054804,-1.,0.79086501270534));
#63526=CARTESIAN_POINT('Ctrl Pts',(-3.83432392054804,1.,0.79086501270534));
#63527=CARTESIAN_POINT('Ctrl Pts',(-3.82687033899799,-1.,0.791447528662381));
#63528=CARTESIAN_POINT('Ctrl Pts',(-3.82687033899799,1.,0.791447528662381));
#63529=CARTESIAN_POINT('Ctrl Pts',(-3.81944345442237,-1.,0.791981740718606));
#63530=CARTESIAN_POINT('Ctrl Pts',(-3.81944345442237,1.,0.791981740718606));
#63531=CARTESIAN_POINT('Ctrl Pts',(-3.81202588694726,-1.,0.792462483517568));
#63532=CARTESIAN_POINT('Ctrl Pts',(-3.81202588694726,1.,0.792462483517568));
#63533=CARTESIAN_POINT('Ctrl Pts',(-3.80459229925598,-1.,0.792882695234693));
#63534=CARTESIAN_POINT('Ctrl Pts',(-3.80459229925598,1.,0.792882695234693));
#63535=CARTESIAN_POINT('Ctrl Pts',(-3.79711921389862,-1.,0.7932356129732));
#63536=CARTESIAN_POINT('Ctrl Pts',(-3.79711921389862,1.,0.7932356129732));
#63537=CARTESIAN_POINT('Ctrl Pts',(-3.78959439439222,-1.,0.793516871680966));
#63538=CARTESIAN_POINT('Ctrl Pts',(-3.78959439439222,1.,0.793516871680966));
#63539=CARTESIAN_POINT('Ctrl Pts',(-3.78202460377617,-1.,0.793726235781339));
#63540=CARTESIAN_POINT('Ctrl Pts',(-3.78202460377617,1.,0.793726235781339));
#63541=CARTESIAN_POINT('Ctrl Pts',(-3.77444863801264,-1.,0.793870523787515));
#63542=CARTESIAN_POINT('Ctrl Pts',(-3.77444863801264,1.,0.793870523787515));
#63543=CARTESIAN_POINT('Ctrl Pts',(-3.76692626931184,-1.,0.793961083689141));
#63544=CARTESIAN_POINT('Ctrl Pts',(-3.76692626931184,1.,0.793961083689141));
#63545=CARTESIAN_POINT('Ctrl Pts',(-3.75951468666325,-1.,0.794008429135047));
#63546=CARTESIAN_POINT('Ctrl Pts',(-3.75951468666325,1.,0.794008429135047));
#63547=CARTESIAN_POINT('Ctrl Pts',(-3.75224692493895,-1.,0.79401734737144));
#63548=CARTESIAN_POINT('Ctrl Pts',(-3.75224692493895,1.,0.79401734737144));
#63549=CARTESIAN_POINT('Ctrl Pts',(-3.74511357728827,-1.,0.79398270045988));
#63550=CARTESIAN_POINT('Ctrl Pts',(-3.74511357728827,1.,0.79398270045988));
#63551=CARTESIAN_POINT('Ctrl Pts',(-3.73803280541576,-1.,0.79388270093679));
#63552=CARTESIAN_POINT('Ctrl Pts',(-3.73803280541576,1.,0.79388270093679));
#63553=CARTESIAN_POINT('Ctrl Pts',(-3.7308691469564,-1.,0.793682750269347));
#63554=CARTESIAN_POINT('Ctrl Pts',(-3.7308691469564,1.,0.793682750269347));
#63555=CARTESIAN_POINT('Ctrl Pts',(-3.7234879729357,-1.,0.79334702378387));
#63556=CARTESIAN_POINT('Ctrl Pts',(-3.7234879729357,1.,0.79334702378387));
#63557=CARTESIAN_POINT('Ctrl Pts',(-3.7158024239604,-1.,0.792848377370115));
#63558=CARTESIAN_POINT('Ctrl Pts',(-3.7158024239604,1.,0.792848377370115));
#63559=CARTESIAN_POINT('Ctrl Pts',(-3.70781724021879,-1.,0.792177688845967));
#63560=CARTESIAN_POINT('Ctrl Pts',(-3.70781724021879,1.,0.792177688845967));
#63561=CARTESIAN_POINT('Ctrl Pts',(-3.69968940808982,-1.,0.791356575696509));
#63562=CARTESIAN_POINT('Ctrl Pts',(-3.69968940808982,1.,0.791356575696509));
#63563=CARTESIAN_POINT('Ctrl Pts',(-3.69172044327754,-1.,0.79043628498958));
#63564=CARTESIAN_POINT('Ctrl Pts',(-3.69172044327754,1.,0.79043628498958));
#63565=CARTESIAN_POINT('Ctrl Pts',(-3.68428439784285,-1.,0.789483546065158));
#63566=CARTESIAN_POINT('Ctrl Pts',(-3.68428439784285,1.,0.789483546065158));
#63567=CARTESIAN_POINT('Ctrl Pts',(-3.67777119516438,-1.,0.788569566220662));
#63568=CARTESIAN_POINT('Ctrl Pts',(-3.67777119516438,1.,0.788569566220662));
#63569=CARTESIAN_POINT('Ctrl Pts',(-3.672529236635,-1.,0.787758799995426));
#63570=CARTESIAN_POINT('Ctrl Pts',(-3.672529236635,1.,0.787758799995426));
#63571=CARTESIAN_POINT('Ctrl Pts',(-3.66879484800625,-1.,0.787095252589507));
#63572=CARTESIAN_POINT('Ctrl Pts',(-3.66879484800625,1.,0.787095252589507));
#63573=CARTESIAN_POINT('Ctrl Pts',(-3.66710211819938,-1.,0.786698783541657));
#63574=CARTESIAN_POINT('Ctrl Pts',(-3.66710211819938,1.,0.786698783541657));
#63575=CARTESIAN_POINT('Ctrl Pts',(-3.66657784454965,-1.,0.786480236184947));
#63576=CARTESIAN_POINT('Ctrl Pts',(-3.66657784454965,1.,0.786480236184947));
#63577=CARTESIAN_POINT('Ctrl Pts',(-3.66655932661846,-1.,0.786369528183039));
#63578=CARTESIAN_POINT('Ctrl Pts',(-3.66655932661846,1.,0.786369528183039));
#63579=CARTESIAN_POINT('Ctrl Pts',(-3.66663282329846,-1.,0.786322922920599));
#63580=CARTESIAN_POINT('Ctrl Pts',(-3.66663282329846,1.,0.786322922920599));
#63581=CARTESIAN_POINT('',(-4.13571194405636,1.,0.732042837400619));
#63582=CARTESIAN_POINT('Ctrl Pts',(-4.13571194405636,1.,0.732042837400619));
#63583=CARTESIAN_POINT('Ctrl Pts',(-4.13420383737278,1.,0.732488575135926));
#63584=CARTESIAN_POINT('Ctrl Pts',(-4.13118752796397,1.,0.733376589325634));
#63585=CARTESIAN_POINT('Ctrl Pts',(-4.12666277572794,1.,0.734698226767512));
#63586=CARTESIAN_POINT('Ctrl Pts',(-4.12062919626082,1.,0.736439634335347));
#63587=CARTESIAN_POINT('Ctrl Pts',(-4.11308626953795,1.,0.738581708229118));
#63588=CARTESIAN_POINT('Ctrl Pts',(-4.1055424175856,1.,0.740688998555151));
#63589=CARTESIAN_POINT('Ctrl Pts',(-4.09799769702712,1.,0.742761369690017));
#63590=CARTESIAN_POINT('Ctrl Pts',(-4.09045220253011,1.,0.744798649705514));
#63591=CARTESIAN_POINT('Ctrl Pts',(-4.08290608094789,1.,0.746800631490821));
#63592=CARTESIAN_POINT('Ctrl Pts',(-4.07535951055363,1.,0.748767076679177));
#63593=CARTESIAN_POINT('Ctrl Pts',(-4.06781267241886,1.,0.750697720483175));
#63594=CARTESIAN_POINT('Ctrl Pts',(-4.06026572221399,1.,0.752592276482869));
#63595=CARTESIAN_POINT('Ctrl Pts',(-4.05271876688106,1.,0.754450441816411));
#63596=CARTESIAN_POINT('Ctrl Pts',(-4.04517182654344,1.,0.756271902370186));
#63597=CARTESIAN_POINT('Ctrl Pts',(-4.03762485803468,1.,0.758056338885553));
#63598=CARTESIAN_POINT('Ctrl Pts',(-4.0300778195465,1.,0.759803433244166));
#63599=CARTESIAN_POINT('Ctrl Pts',(-4.02253072741347,1.,0.761512875859941));
#63600=CARTESIAN_POINT('Ctrl Pts',(-4.01498370680434,1.,0.763184371182826));
#63601=CARTESIAN_POINT('Ctrl Pts',(-4.00743706791366,1.,0.764817648784946));
#63602=CARTESIAN_POINT('Ctrl Pts',(-3.99989129179464,1.,0.766412457135785));
#63603=CARTESIAN_POINT('Ctrl Pts',(-3.99234687880892,1.,0.767968531377708));
#63604=CARTESIAN_POINT('Ctrl Pts',(-3.98480422348403,1.,0.769485566245459));
#63605=CARTESIAN_POINT('Ctrl Pts',(-3.97726349165507,1.,0.770963190030503));
#63606=CARTESIAN_POINT('Ctrl Pts',(-3.96972446532832,1.,0.772400931772238));
#63607=CARTESIAN_POINT('Ctrl Pts',(-3.96218649639876,1.,0.773798212026682));
#63608=CARTESIAN_POINT('Ctrl Pts',(-3.95464885452364,1.,0.775154418039441));
#63609=CARTESIAN_POINT('Ctrl Pts',(-3.94711101619471,1.,0.77646896669796));
#63610=CARTESIAN_POINT('Ctrl Pts',(-3.93957296768098,1.,0.777741370568549));
#63611=CARTESIAN_POINT('Ctrl Pts',(-3.93203552473153,1.,0.778971308134786));
#63612=CARTESIAN_POINT('Ctrl Pts',(-3.92450058323799,1.,0.780158678615506));
#63613=CARTESIAN_POINT('Ctrl Pts',(-3.9169703605466,1.,0.781303428618343));
#63614=CARTESIAN_POINT('Ctrl Pts',(-3.90944671004536,1.,0.782405395622758));
#63615=CARTESIAN_POINT('Ctrl Pts',(-3.90193039043971,1.,0.783464141529082));
#63616=CARTESIAN_POINT('Ctrl Pts',(-3.89442039235105,1.,0.784478799358335));
#63617=CARTESIAN_POINT('Ctrl Pts',(-3.88691313167399,1.,0.785447890340723));
#63618=CARTESIAN_POINT('Ctrl Pts',(-3.87940402818186,1.,0.786369675812592));
#63619=CARTESIAN_POINT('Ctrl Pts',(-3.87188916600905,1.,0.78724252761798));
#63620=CARTESIAN_POINT('Ctrl Pts',(-3.86436702561342,1.,0.788065315093771));
#63621=CARTESIAN_POINT('Ctrl Pts',(-3.85683995872536,1.,0.788837734090688));
#63622=CARTESIAN_POINT('Ctrl Pts',(-3.8493163780891,1.,0.789560798155618));
#63623=CARTESIAN_POINT('Ctrl Pts',(-3.84180762342476,1.,0.790236124191289));
#63624=CARTESIAN_POINT('Ctrl Pts',(-3.83432392054804,1.,0.79086501270534));
#63625=CARTESIAN_POINT('Ctrl Pts',(-3.82687033899799,1.,0.791447528662381));
#63626=CARTESIAN_POINT('Ctrl Pts',(-3.81944345442237,1.,0.791981740718606));
#63627=CARTESIAN_POINT('Ctrl Pts',(-3.81202588694726,1.,0.792462483517568));
#63628=CARTESIAN_POINT('Ctrl Pts',(-3.80459229925598,1.,0.792882695234693));
#63629=CARTESIAN_POINT('Ctrl Pts',(-3.79711921389862,1.,0.7932356129732));
#63630=CARTESIAN_POINT('Ctrl Pts',(-3.78959439439222,1.,0.793516871680966));
#63631=CARTESIAN_POINT('Ctrl Pts',(-3.78202460377617,1.,0.793726235781339));
#63632=CARTESIAN_POINT('Ctrl Pts',(-3.77444863801264,1.,0.793870523787515));
#63633=CARTESIAN_POINT('Ctrl Pts',(-3.76692626931184,1.,0.793961083689141));
#63634=CARTESIAN_POINT('Ctrl Pts',(-3.75951468666325,1.,0.794008429135047));
#63635=CARTESIAN_POINT('Ctrl Pts',(-3.75224692493895,1.,0.79401734737144));
#63636=CARTESIAN_POINT('Ctrl Pts',(-3.74511357728827,1.,0.79398270045988));
#63637=CARTESIAN_POINT('Ctrl Pts',(-3.73803280541576,1.,0.79388270093679));
#63638=CARTESIAN_POINT('Ctrl Pts',(-3.7308691469564,1.,0.793682750269347));
#63639=CARTESIAN_POINT('Ctrl Pts',(-3.7234879729357,1.,0.79334702378387));
#63640=CARTESIAN_POINT('Ctrl Pts',(-3.7158024239604,1.,0.792848377370115));
#63641=CARTESIAN_POINT('Ctrl Pts',(-3.70781724021879,1.,0.792177688845967));
#63642=CARTESIAN_POINT('Ctrl Pts',(-3.69968940808982,1.,0.791356575696509));
#63643=CARTESIAN_POINT('Ctrl Pts',(-3.69172044327754,1.,0.79043628498958));
#63644=CARTESIAN_POINT('Ctrl Pts',(-3.68428439784285,1.,0.789483546065158));
#63645=CARTESIAN_POINT('Ctrl Pts',(-3.67777119516438,1.,0.788569566220662));
#63646=CARTESIAN_POINT('Ctrl Pts',(-3.672529236635,1.,0.787758799995426));
#63647=CARTESIAN_POINT('Ctrl Pts',(-3.66907505398769,1.,0.787145041181588));
#63648=CARTESIAN_POINT('Ctrl Pts',(-3.66743103898844,1.,0.786774337198499));
#63649=CARTESIAN_POINT('Ctrl Pts',(-3.66680946938396,1.,0.786565919559889));
#63650=CARTESIAN_POINT('Ctrl Pts',(-3.66664310415236,1.,0.786459983896781));
#63651=CARTESIAN_POINT('Ctrl Pts',(-3.66661143271648,1.,0.786422660833743));
#63652=CARTESIAN_POINT('',(-4.13571194405636,0.,0.732042837400619));
#63653=CARTESIAN_POINT('Ctrl Pts',(-3.73016218570874,-1.,0.385214314776329));
#63654=CARTESIAN_POINT('Ctrl Pts',(-3.73016218570874,1.,0.385214314776329));
#63655=CARTESIAN_POINT('Ctrl Pts',(-3.73010668803185,-1.,0.385147278814804));
#63656=CARTESIAN_POINT('Ctrl Pts',(-3.73010668803185,1.,0.385147278814804));
#63657=CARTESIAN_POINT('Ctrl Pts',(-3.73015851028729,-1.,0.385047711603887));
#63658=CARTESIAN_POINT('Ctrl Pts',(-3.73015851028729,1.,0.385047711603887));
#63659=CARTESIAN_POINT('Ctrl Pts',(-3.73072465900727,-1.,0.385001870183841));
#63660=CARTESIAN_POINT('Ctrl Pts',(-3.73072465900727,1.,0.385001870183841));
#63661=CARTESIAN_POINT('Ctrl Pts',(-3.73245705639337,-1.,0.385147887989514));
#63662=CARTESIAN_POINT('Ctrl Pts',(-3.73245705639337,1.,0.385147887989514));
#63663=CARTESIAN_POINT('Ctrl Pts',(-3.73621371845475,-1.,0.385670806454744));
#63664=CARTESIAN_POINT('Ctrl Pts',(-3.73621371845475,1.,0.385670806454744));
#63665=CARTESIAN_POINT('Ctrl Pts',(-3.74144965781088,-1.,0.386519576222035));
#63666=CARTESIAN_POINT('Ctrl Pts',(-3.74144965781088,1.,0.386519576222035));
#63667=CARTESIAN_POINT('Ctrl Pts',(-3.74792651696269,-1.,0.387663020050396));
#63668=CARTESIAN_POINT('Ctrl Pts',(-3.74792651696269,1.,0.387663020050396));
#63669=CARTESIAN_POINT('Ctrl Pts',(-3.75529302894757,-1.,0.389054775898251));
#63670=CARTESIAN_POINT('Ctrl Pts',(-3.75529302894757,1.,0.389054775898251));
#63671=CARTESIAN_POINT('Ctrl Pts',(-3.76315635032993,-1.,0.390642072979259));
#63672=CARTESIAN_POINT('Ctrl Pts',(-3.76315635032993,1.,0.390642072979259));
#63673=CARTESIAN_POINT('Ctrl Pts',(-3.77114011595892,-1.,0.392372786223346));
#63674=CARTESIAN_POINT('Ctrl Pts',(-3.77114011595892,1.,0.392372786223346));
#63675=CARTESIAN_POINT('Ctrl Pts',(-3.77894173114368,-1.,0.394202481011595));
#63676=CARTESIAN_POINT('Ctrl Pts',(-3.77894173114368,1.,0.394202481011595));
#63677=CARTESIAN_POINT('Ctrl Pts',(-3.78640521279479,-1.,0.396103205335028));
#63678=CARTESIAN_POINT('Ctrl Pts',(-3.78640521279479,1.,0.396103205335028));
#63679=CARTESIAN_POINT('Ctrl Pts',(-3.79352887163457,-1.,0.398064818684158));
#63680=CARTESIAN_POINT('Ctrl Pts',(-3.79352887163457,1.,0.398064818684158));
#63681=CARTESIAN_POINT('Ctrl Pts',(-3.80040370384659,-1.,0.400088346504726));
#63682=CARTESIAN_POINT('Ctrl Pts',(-3.80040370384659,1.,0.400088346504726));
#63683=CARTESIAN_POINT('Ctrl Pts',(-3.80716881962763,-1.,0.402181320148474));
#63684=CARTESIAN_POINT('Ctrl Pts',(-3.80716881962763,1.,0.402181320148474));
#63685=CARTESIAN_POINT('Ctrl Pts',(-3.81396374287762,-1.,0.404352694628236));
#63686=CARTESIAN_POINT('Ctrl Pts',(-3.81396374287762,1.,0.404352694628236));
#63687=CARTESIAN_POINT('Ctrl Pts',(-3.82087303913741,-1.,0.406607038258906));
#63688=CARTESIAN_POINT('Ctrl Pts',(-3.82087303913741,1.,0.406607038258906));
#63689=CARTESIAN_POINT('Ctrl Pts',(-3.82790724256397,-1.,0.408942371447377));
#63690=CARTESIAN_POINT('Ctrl Pts',(-3.82790724256397,1.,0.408942371447377));
#63691=CARTESIAN_POINT('Ctrl Pts',(-3.83503345578645,-1.,0.411353038798459));
#63692=CARTESIAN_POINT('Ctrl Pts',(-3.83503345578645,1.,0.411353038798459));
#63693=CARTESIAN_POINT('Ctrl Pts',(-3.84219403994742,-1.,0.413831367016726));
#63694=CARTESIAN_POINT('Ctrl Pts',(-3.84219403994742,1.,0.413831367016726));
#63695=CARTESIAN_POINT('Ctrl Pts',(-3.8493286415751,-1.,0.41636967805292));
#63696=CARTESIAN_POINT('Ctrl Pts',(-3.8493286415751,1.,0.41636967805292));
#63697=CARTESIAN_POINT('Ctrl Pts',(-3.85639825648031,-1.,0.418962468086809));
#63698=CARTESIAN_POINT('Ctrl Pts',(-3.85639825648031,1.,0.418962468086809));
#63699=CARTESIAN_POINT('Ctrl Pts',(-3.86339652542749,-1.,0.421607423177575));
#63700=CARTESIAN_POINT('Ctrl Pts',(-3.86339652542749,1.,0.421607423177575));
#63701=CARTESIAN_POINT('Ctrl Pts',(-3.87033643487882,-1.,0.424304173195142));
#63702=CARTESIAN_POINT('Ctrl Pts',(-3.87033643487882,1.,0.424304173195142));
#63703=CARTESIAN_POINT('Ctrl Pts',(-3.87724240306609,-1.,0.427053541173469));
#63704=CARTESIAN_POINT('Ctrl Pts',(-3.87724240306609,1.,0.427053541173469));
#63705=CARTESIAN_POINT('Ctrl Pts',(-3.88414070943334,-1.,0.429856640579733));
#63706=CARTESIAN_POINT('Ctrl Pts',(-3.88414070943334,1.,0.429856640579733));
#63707=CARTESIAN_POINT('Ctrl Pts',(-3.89104947940592,-1.,0.432713929544439));
#63708=CARTESIAN_POINT('Ctrl Pts',(-3.89104947940592,1.,0.432713929544439));
#63709=CARTESIAN_POINT('Ctrl Pts',(-3.8979725665544,-1.,0.435624629433505));
#63710=CARTESIAN_POINT('Ctrl Pts',(-3.8979725665544,1.,0.435624629433505));
#63711=CARTESIAN_POINT('Ctrl Pts',(-3.90490512938546,-1.,0.438587235458233));
#63712=CARTESIAN_POINT('Ctrl Pts',(-3.90490512938546,1.,0.438587235458233));
#63713=CARTESIAN_POINT('Ctrl Pts',(-3.91183704069146,-1.,0.441599824524047));
#63714=CARTESIAN_POINT('Ctrl Pts',(-3.91183704069146,1.,0.441599824524047));
#63715=CARTESIAN_POINT('Ctrl Pts',(-3.91875701610721,-1.,0.444660430230592));
#63716=CARTESIAN_POINT('Ctrl Pts',(-3.91875701610721,1.,0.444660430230592));
#63717=CARTESIAN_POINT('Ctrl Pts',(-3.92565674143424,-1.,0.447767416837296));
#63718=CARTESIAN_POINT('Ctrl Pts',(-3.92565674143424,1.,0.447767416837296));
#63719=CARTESIAN_POINT('Ctrl Pts',(-3.93253407403128,-1.,0.450919768356347));
#63720=CARTESIAN_POINT('Ctrl Pts',(-3.93253407403128,1.,0.450919768356347));
#63721=CARTESIAN_POINT('Ctrl Pts',(-3.93939080846298,-1.,0.454116879027576));
#63722=CARTESIAN_POINT('Ctrl Pts',(-3.93939080846298,1.,0.454116879027576));
#63723=CARTESIAN_POINT('Ctrl Pts',(-3.94623117206675,-1.,0.457358410451674));
#63724=CARTESIAN_POINT('Ctrl Pts',(-3.94623117206675,1.,0.457358410451674));
#63725=CARTESIAN_POINT('Ctrl Pts',(-3.95306005817363,-1.,0.460644124429119));
#63726=CARTESIAN_POINT('Ctrl Pts',(-3.95306005817363,1.,0.460644124429119));
#63727=CARTESIAN_POINT('Ctrl Pts',(-3.95988133243543,-1.,0.463973722115744));
#63728=CARTESIAN_POINT('Ctrl Pts',(-3.95988133243543,1.,0.463973722115744));
#63729=CARTESIAN_POINT('Ctrl Pts',(-3.96669622273946,-1.,0.467346690880671));
#63730=CARTESIAN_POINT('Ctrl Pts',(-3.96669622273946,1.,0.467346690880671));
#63731=CARTESIAN_POINT('Ctrl Pts',(-3.97350414289415,-1.,0.470762379613477));
#63732=CARTESIAN_POINT('Ctrl Pts',(-3.97350414289415,1.,0.470762379613477));
#63733=CARTESIAN_POINT('Ctrl Pts',(-3.9803033804443,-1.,0.474220061019542));
#63734=CARTESIAN_POINT('Ctrl Pts',(-3.9803033804443,1.,0.474220061019542));
#63735=CARTESIAN_POINT('Ctrl Pts',(-3.98709184306743,-1.,0.477718999122033));
#63736=CARTESIAN_POINT('Ctrl Pts',(-3.98709184306743,1.,0.477718999122033));
#63737=CARTESIAN_POINT('Ctrl Pts',(-3.99386775880655,-1.,0.481258512209638));
#63738=CARTESIAN_POINT('Ctrl Pts',(-3.99386775880655,1.,0.481258512209638));
#63739=CARTESIAN_POINT('Ctrl Pts',(-4.00063045119234,-1.,0.484838042421754));
#63740=CARTESIAN_POINT('Ctrl Pts',(-4.00063045119234,1.,0.484838042421754));
#63741=CARTESIAN_POINT('Ctrl Pts',(-4.0073800839092,-1.,0.48845713042453));
#63742=CARTESIAN_POINT('Ctrl Pts',(-4.0073800839092,1.,0.48845713042453));
#63743=CARTESIAN_POINT('Ctrl Pts',(-4.01411733503486,-1.,0.49211538341793));
#63744=CARTESIAN_POINT('Ctrl Pts',(-4.01411733503486,1.,0.49211538341793));
#63745=CARTESIAN_POINT('Ctrl Pts',(-4.02084308851813,-1.,0.495812444326223));
#63746=CARTESIAN_POINT('Ctrl Pts',(-4.02084308851813,1.,0.495812444326223));
#63747=CARTESIAN_POINT('Ctrl Pts',(-4.0275581398015,-1.,0.499547962340889));
#63748=CARTESIAN_POINT('Ctrl Pts',(-4.0275581398015,1.,0.499547962340889));
#63749=CARTESIAN_POINT('Ctrl Pts',(-4.0342628417439,-1.,0.503321556915513));
#63750=CARTESIAN_POINT('Ctrl Pts',(-4.0342628417439,1.,0.503321556915513));
#63751=CARTESIAN_POINT('Ctrl Pts',(-4.04095715149074,-1.,0.507132823288361));
#63752=CARTESIAN_POINT('Ctrl Pts',(-4.04095715149074,1.,0.507132823288361));
#63753=CARTESIAN_POINT('Ctrl Pts',(-4.04764078815591,-1.,0.510981349219173));
#63754=CARTESIAN_POINT('Ctrl Pts',(-4.04764078815591,1.,0.510981349219173));
#63755=CARTESIAN_POINT('Ctrl Pts',(-4.05431335771261,-1.,0.514866728193104));
#63756=CARTESIAN_POINT('Ctrl Pts',(-4.05431335771261,1.,0.514866728193104));
#63757=CARTESIAN_POINT('Ctrl Pts',(-4.06097448037934,-1.,0.518788572336809));
#63758=CARTESIAN_POINT('Ctrl Pts',(-4.06097448037934,1.,0.518788572336809));
#63759=CARTESIAN_POINT('Ctrl Pts',(-4.06762394471075,-1.,0.522746528602767));
#63760=CARTESIAN_POINT('Ctrl Pts',(-4.06762394471075,1.,0.522746528602767));
#63761=CARTESIAN_POINT('Ctrl Pts',(-4.07426172299496,-1.,0.526740277226999));
#63762=CARTESIAN_POINT('Ctrl Pts',(-4.07426172299496,1.,0.526740277226999));
#63763=CARTESIAN_POINT('Ctrl Pts',(-4.08088789536488,-1.,0.530769518728075));
#63764=CARTESIAN_POINT('Ctrl Pts',(-4.08088789536488,1.,0.530769518728075));
#63765=CARTESIAN_POINT('Ctrl Pts',(-4.08750259988693,-1.,0.534833963476999));
#63766=CARTESIAN_POINT('Ctrl Pts',(-4.08750259988693,1.,0.534833963476999));
#63767=CARTESIAN_POINT('Ctrl Pts',(-4.09410597627116,-1.,0.53893332117992));
#63768=CARTESIAN_POINT('Ctrl Pts',(-4.09410597627116,1.,0.53893332117992));
#63769=CARTESIAN_POINT('Ctrl Pts',(-4.10069810244473,-1.,0.543067286878457));
#63770=CARTESIAN_POINT('Ctrl Pts',(-4.10069810244473,1.,0.543067286878457));
#63771=CARTESIAN_POINT('Ctrl Pts',(-4.1072789702877,-1.,0.547235539486759));
#63772=CARTESIAN_POINT('Ctrl Pts',(-4.1072789702877,1.,0.547235539486759));
#63773=CARTESIAN_POINT('Ctrl Pts',(-4.11384852025578,-1.,0.551437758498246));
#63774=CARTESIAN_POINT('Ctrl Pts',(-4.11384852025578,1.,0.551437758498246));
#63775=CARTESIAN_POINT('Ctrl Pts',(-4.1204066619623,-1.,0.555673636130778));
#63776=CARTESIAN_POINT('Ctrl Pts',(-4.1204066619623,1.,0.555673636130778));
#63777=CARTESIAN_POINT('Ctrl Pts',(-4.12695329951859,-1.,0.559942890594628));
#63778=CARTESIAN_POINT('Ctrl Pts',(-4.12695329951859,1.,0.559942890594628));
#63779=CARTESIAN_POINT('Ctrl Pts',(-4.13348835726086,-1.,0.564245279535705));
#63780=CARTESIAN_POINT('Ctrl Pts',(-4.13348835726086,1.,0.564245279535705));
#63781=CARTESIAN_POINT('Ctrl Pts',(-4.14001179828669,-1.,0.568580610187116));
#63782=CARTESIAN_POINT('Ctrl Pts',(-4.14001179828669,1.,0.568580610187116));
#63783=CARTESIAN_POINT('Ctrl Pts',(-4.14652361065787,-1.,0.572948736066276));
#63784=CARTESIAN_POINT('Ctrl Pts',(-4.14652361065787,1.,0.572948736066276));
#63785=CARTESIAN_POINT('Ctrl Pts',(-4.1517237611974,-1.,0.576469391673916));
#63786=CARTESIAN_POINT('Ctrl Pts',(-4.1517237611974,1.,0.576469391673916));
#63787=CARTESIAN_POINT('Ctrl Pts',(-4.15561864787379,-1.,0.579124568912543));
#63788=CARTESIAN_POINT('Ctrl Pts',(-4.15561864787379,1.,0.579124568912543));
#63789=CARTESIAN_POINT('Ctrl Pts',(-4.15821291712391,-1.,0.580901211462913));
#63790=CARTESIAN_POINT('Ctrl Pts',(-4.15821291712391,1.,0.580901211462913));
#63791=CARTESIAN_POINT('Ctrl Pts',(-4.15950947128175,-1.,0.581791163835814));
#63792=CARTESIAN_POINT('Ctrl Pts',(-4.15950947128175,1.,0.581791163835814));
#63793=CARTESIAN_POINT('',(-3.73017266276632,1.,0.385112848332549));
#63794=CARTESIAN_POINT('Ctrl Pts',(-3.73017266276632,-1.,0.385112848332549));
#63795=CARTESIAN_POINT('Ctrl Pts',(-3.73017266276632,-0.666666666666667,
0.385112848332549));
#63796=CARTESIAN_POINT('Ctrl Pts',(-3.73017266276632,-0.333333333333333,
0.385112848332549));
#63797=CARTESIAN_POINT('Ctrl Pts',(-3.73017266276632,0.333333333333333,
0.385112848332549));
#63798=CARTESIAN_POINT('Ctrl Pts',(-3.73017266276632,0.666666666666667,
0.385112848332549));
#63799=CARTESIAN_POINT('Ctrl Pts',(-3.73017266276632,1.,0.385112848332549));
#63800=CARTESIAN_POINT('',(-4.15950947128175,1.,0.581791163835814));
#63801=CARTESIAN_POINT('',(-4.15950947128175,0.,0.581791163835814));
#63802=CARTESIAN_POINT('Ctrl Pts',(-3.73017266276632,1.,0.385112848332549));
#63803=CARTESIAN_POINT('Ctrl Pts',(-3.73021431755218,1.,0.385087139001609));
#63804=CARTESIAN_POINT('Ctrl Pts',(-3.73040527620929,1.,0.385037797882046));
#63805=CARTESIAN_POINT('Ctrl Pts',(-3.73106082862399,1.,0.385031656499141));
#63806=CARTESIAN_POINT('Ctrl Pts',(-3.73273893363318,1.,0.385187124633964));
#63807=CARTESIAN_POINT('Ctrl Pts',(-3.73621371845475,1.,0.385670806454744));
#63808=CARTESIAN_POINT('Ctrl Pts',(-3.74144965781088,1.,0.386519576222035));
#63809=CARTESIAN_POINT('Ctrl Pts',(-3.74792651696269,1.,0.387663020050396));
#63810=CARTESIAN_POINT('Ctrl Pts',(-3.75529302894757,1.,0.389054775898251));
#63811=CARTESIAN_POINT('Ctrl Pts',(-3.76315635032993,1.,0.390642072979259));
#63812=CARTESIAN_POINT('Ctrl Pts',(-3.77114011595892,1.,0.392372786223346));
#63813=CARTESIAN_POINT('Ctrl Pts',(-3.77894173114368,1.,0.394202481011595));
#63814=CARTESIAN_POINT('Ctrl Pts',(-3.78640521279479,1.,0.396103205335028));
#63815=CARTESIAN_POINT('Ctrl Pts',(-3.79352887163457,1.,0.398064818684158));
#63816=CARTESIAN_POINT('Ctrl Pts',(-3.80040370384659,1.,0.400088346504726));
#63817=CARTESIAN_POINT('Ctrl Pts',(-3.80716881962763,1.,0.402181320148474));
#63818=CARTESIAN_POINT('Ctrl Pts',(-3.81396374287762,1.,0.404352694628236));
#63819=CARTESIAN_POINT('Ctrl Pts',(-3.82087303913741,1.,0.406607038258906));
#63820=CARTESIAN_POINT('Ctrl Pts',(-3.82790724256397,1.,0.408942371447377));
#63821=CARTESIAN_POINT('Ctrl Pts',(-3.83503345578645,1.,0.411353038798459));
#63822=CARTESIAN_POINT('Ctrl Pts',(-3.84219403994742,1.,0.413831367016726));
#63823=CARTESIAN_POINT('Ctrl Pts',(-3.8493286415751,1.,0.41636967805292));
#63824=CARTESIAN_POINT('Ctrl Pts',(-3.85639825648031,1.,0.418962468086809));
#63825=CARTESIAN_POINT('Ctrl Pts',(-3.86339652542749,1.,0.421607423177575));
#63826=CARTESIAN_POINT('Ctrl Pts',(-3.87033643487882,1.,0.424304173195142));
#63827=CARTESIAN_POINT('Ctrl Pts',(-3.87724240306609,1.,0.427053541173469));
#63828=CARTESIAN_POINT('Ctrl Pts',(-3.88414070943334,1.,0.429856640579733));
#63829=CARTESIAN_POINT('Ctrl Pts',(-3.89104947940592,1.,0.432713929544439));
#63830=CARTESIAN_POINT('Ctrl Pts',(-3.8979725665544,1.,0.435624629433505));
#63831=CARTESIAN_POINT('Ctrl Pts',(-3.90490512938546,1.,0.438587235458233));
#63832=CARTESIAN_POINT('Ctrl Pts',(-3.91183704069146,1.,0.441599824524047));
#63833=CARTESIAN_POINT('Ctrl Pts',(-3.91875701610721,1.,0.444660430230592));
#63834=CARTESIAN_POINT('Ctrl Pts',(-3.92565674143424,1.,0.447767416837296));
#63835=CARTESIAN_POINT('Ctrl Pts',(-3.93253407403128,1.,0.450919768356347));
#63836=CARTESIAN_POINT('Ctrl Pts',(-3.93939080846298,1.,0.454116879027576));
#63837=CARTESIAN_POINT('Ctrl Pts',(-3.94623117206675,1.,0.457358410451674));
#63838=CARTESIAN_POINT('Ctrl Pts',(-3.95306005817363,1.,0.460644124429119));
#63839=CARTESIAN_POINT('Ctrl Pts',(-3.95988133243543,1.,0.463973722115744));
#63840=CARTESIAN_POINT('Ctrl Pts',(-3.96669622273946,1.,0.467346690880671));
#63841=CARTESIAN_POINT('Ctrl Pts',(-3.97350414289415,1.,0.470762379613477));
#63842=CARTESIAN_POINT('Ctrl Pts',(-3.9803033804443,1.,0.474220061019542));
#63843=CARTESIAN_POINT('Ctrl Pts',(-3.98709184306743,1.,0.477718999122033));
#63844=CARTESIAN_POINT('Ctrl Pts',(-3.99386775880655,1.,0.481258512209638));
#63845=CARTESIAN_POINT('Ctrl Pts',(-4.00063045119234,1.,0.484838042421754));
#63846=CARTESIAN_POINT('Ctrl Pts',(-4.0073800839092,1.,0.48845713042453));
#63847=CARTESIAN_POINT('Ctrl Pts',(-4.01411733503486,1.,0.49211538341793));
#63848=CARTESIAN_POINT('Ctrl Pts',(-4.02084308851813,1.,0.495812444326223));
#63849=CARTESIAN_POINT('Ctrl Pts',(-4.0275581398015,1.,0.499547962340889));
#63850=CARTESIAN_POINT('Ctrl Pts',(-4.0342628417439,1.,0.503321556915513));
#63851=CARTESIAN_POINT('Ctrl Pts',(-4.04095715149074,1.,0.507132823288361));
#63852=CARTESIAN_POINT('Ctrl Pts',(-4.04764078815591,1.,0.510981349219173));
#63853=CARTESIAN_POINT('Ctrl Pts',(-4.05431335771261,1.,0.514866728193104));
#63854=CARTESIAN_POINT('Ctrl Pts',(-4.06097448037934,1.,0.518788572336809));
#63855=CARTESIAN_POINT('Ctrl Pts',(-4.06762394471075,1.,0.522746528602767));
#63856=CARTESIAN_POINT('Ctrl Pts',(-4.07426172299496,1.,0.526740277226999));
#63857=CARTESIAN_POINT('Ctrl Pts',(-4.08088789536488,1.,0.530769518728075));
#63858=CARTESIAN_POINT('Ctrl Pts',(-4.08750259988693,1.,0.534833963476999));
#63859=CARTESIAN_POINT('Ctrl Pts',(-4.09410597627116,1.,0.53893332117992));
#63860=CARTESIAN_POINT('Ctrl Pts',(-4.10069810244473,1.,0.543067286878457));
#63861=CARTESIAN_POINT('Ctrl Pts',(-4.1072789702877,1.,0.547235539486759));
#63862=CARTESIAN_POINT('Ctrl Pts',(-4.11384852025578,1.,0.551437758498246));
#63863=CARTESIAN_POINT('Ctrl Pts',(-4.1204066619623,1.,0.555673636130778));
#63864=CARTESIAN_POINT('Ctrl Pts',(-4.12695329951859,1.,0.559942890594628));
#63865=CARTESIAN_POINT('Ctrl Pts',(-4.13348835726086,1.,0.564245279535705));
#63866=CARTESIAN_POINT('Ctrl Pts',(-4.14001179828669,1.,0.568580610187116));
#63867=CARTESIAN_POINT('Ctrl Pts',(-4.14652361065787,1.,0.572948736066276));
#63868=CARTESIAN_POINT('Ctrl Pts',(-4.1517237611974,1.,0.576469391673916));
#63869=CARTESIAN_POINT('Ctrl Pts',(-4.15561864787379,1.,0.579124568912543));
#63870=CARTESIAN_POINT('Ctrl Pts',(-4.15821291712391,1.,0.580901211462913));
#63871=CARTESIAN_POINT('Ctrl Pts',(-4.15950947128175,1.,0.581791163835814));
#63872=CARTESIAN_POINT('Origin',(-4.15950947128175,0.,0.581791163835814));
#63873=CARTESIAN_POINT('',(-4.13571194405636,1.,0.732042837400619));
#63874=CARTESIAN_POINT('Origin',(0.,0.,0.));
#63875=CARTESIAN_POINT('',(-3.74449296982994,1.,0.203156094897896));
#63876=CARTESIAN_POINT('Origin',(0.,1.,0.));
#63877=CARTESIAN_POINT('Ctrl Pts',(-3.74449296982994,1.,0.203156094897896));
#63878=CARTESIAN_POINT('Ctrl Pts',(-3.74449296982994,0.666666666666667,
0.203156094897896));
#63879=CARTESIAN_POINT('Ctrl Pts',(-3.74449296982994,0.333333333333333,
0.203156094897896));
#63880=CARTESIAN_POINT('Ctrl Pts',(-3.74449296982994,-0.333333333333333,
0.203156094897896));
#63881=CARTESIAN_POINT('Ctrl Pts',(-3.74449296982994,-0.666666666666667,
0.203156094897896));
#63882=CARTESIAN_POINT('Ctrl Pts',(-3.74449296982994,-1.,0.203156094897896));
#63883=CARTESIAN_POINT('Ctrl Pts',(-4.19931119685982,-1.,0.0760622897878236));
#63884=CARTESIAN_POINT('Ctrl Pts',(-4.19931119685982,1.,0.0760622897878236));
#63885=CARTESIAN_POINT('Ctrl Pts',(-4.19789138621624,-1.,0.0767384596142195));
#63886=CARTESIAN_POINT('Ctrl Pts',(-4.19789138621624,1.,0.0767384596142195));
#63887=CARTESIAN_POINT('Ctrl Pts',(-4.19505112860624,-1.,0.0780873956244402));
#63888=CARTESIAN_POINT('Ctrl Pts',(-4.19505112860624,1.,0.0780873956244402));
#63889=CARTESIAN_POINT('Ctrl Pts',(-4.19078883322483,-1.,0.0801005887117603));
#63890=CARTESIAN_POINT('Ctrl Pts',(-4.19078883322483,1.,0.0801005887117603));
#63891=CARTESIAN_POINT('Ctrl Pts',(-4.1851019532944,-1.,0.082764416438951));
#63892=CARTESIAN_POINT('Ctrl Pts',(-4.1851019532944,1.,0.082764416438951));
#63893=CARTESIAN_POINT('Ctrl Pts',(-4.17798698669991,-1.,0.0860600915552515));
#63894=CARTESIAN_POINT('Ctrl Pts',(-4.17798698669991,1.,0.0860600915552515));
#63895=CARTESIAN_POINT('Ctrl Pts',(-4.17086566491823,-1.,0.0893215560850327));
#63896=CARTESIAN_POINT('Ctrl Pts',(-4.17086566491823,1.,0.0893215560850327));
#63897=CARTESIAN_POINT('Ctrl Pts',(-4.16373802265942,-1.,0.092548667216769));
#63898=CARTESIAN_POINT('Ctrl Pts',(-4.16373802265942,1.,0.092548667216769));
#63899=CARTESIAN_POINT('Ctrl Pts',(-4.15660412653006,-1.,0.0957412403297067));
#63900=CARTESIAN_POINT('Ctrl Pts',(-4.15660412653006,1.,0.0957412403297067));
#63901=CARTESIAN_POINT('Ctrl Pts',(-4.1494640891762,-1.,0.0988990478899811));
#63902=CARTESIAN_POINT('Ctrl Pts',(-4.1494640891762,1.,0.0988990478899811));
#63903=CARTESIAN_POINT('Ctrl Pts',(-4.14231804938737,-1.,0.102021826577454));
#63904=CARTESIAN_POINT('Ctrl Pts',(-4.14231804938737,1.,0.102021826577454));
#63905=CARTESIAN_POINT('Ctrl Pts',(-4.13516614458396,-1.,0.105109286538864));
#63906=CARTESIAN_POINT('Ctrl Pts',(-4.13516614458396,1.,0.105109286538864));
#63907=CARTESIAN_POINT('Ctrl Pts',(-4.12800848371386,-1.,0.10816112052835));
#63908=CARTESIAN_POINT('Ctrl Pts',(-4.12800848371386,1.,0.10816112052835));
#63909=CARTESIAN_POINT('Ctrl Pts',(-4.12084512502444,-1.,0.111177012683377));
#63910=CARTESIAN_POINT('Ctrl Pts',(-4.12084512502444,1.,0.111177012683377));
#63911=CARTESIAN_POINT('Ctrl Pts',(-4.11367603925313,-1.,0.114156649609601));
#63912=CARTESIAN_POINT('Ctrl Pts',(-4.11367603925313,1.,0.114156649609601));
#63913=CARTESIAN_POINT('Ctrl Pts',(-4.10650113382187,-1.,0.117099722731704));
#63914=CARTESIAN_POINT('Ctrl Pts',(-4.10650113382187,1.,0.117099722731704));
#63915=CARTESIAN_POINT('Ctrl Pts',(-4.09932031767243,-1.,0.120005924388162));
#63916=CARTESIAN_POINT('Ctrl Pts',(-4.09932031767243,1.,0.120005924388162));
#63917=CARTESIAN_POINT('Ctrl Pts',(-4.09213355850836,-1.,0.122874946249119));
#63918=CARTESIAN_POINT('Ctrl Pts',(-4.09213355850836,1.,0.122874946249119));
#63919=CARTESIAN_POINT('Ctrl Pts',(-4.08494093372315,-1.,0.125706476822529));
#63920=CARTESIAN_POINT('Ctrl Pts',(-4.08494093372315,1.,0.125706476822529));
#63921=CARTESIAN_POINT('Ctrl Pts',(-4.07774270738809,-1.,0.128500200484814));
#63922=CARTESIAN_POINT('Ctrl Pts',(-4.07774270738809,1.,0.128500200484814));
#63923=CARTESIAN_POINT('Ctrl Pts',(-4.07053931528579,-1.,0.131255793548914));
#63924=CARTESIAN_POINT('Ctrl Pts',(-4.07053931528579,1.,0.131255793548914));
#63925=CARTESIAN_POINT('Ctrl Pts',(-4.06333121018476,-1.,0.133972916144225));
#63926=CARTESIAN_POINT('Ctrl Pts',(-4.06333121018476,1.,0.133972916144225));
#63927=CARTESIAN_POINT('Ctrl Pts',(-4.05611873400122,-1.,0.136651205046111));
#63928=CARTESIAN_POINT('Ctrl Pts',(-4.05611873400122,1.,0.136651205046111));
#63929=CARTESIAN_POINT('Ctrl Pts',(-4.04890199238056,-1.,0.139290267180059));
#63930=CARTESIAN_POINT('Ctrl Pts',(-4.04890199238056,1.,0.139290267180059));
#63931=CARTESIAN_POINT('Ctrl Pts',(-4.04168069633842,-1.,0.141889671485508));
#63932=CARTESIAN_POINT('Ctrl Pts',(-4.04168069633842,1.,0.141889671485508));
#63933=CARTESIAN_POINT('Ctrl Pts',(-4.03445411510403,-1.,0.144448947038352));
#63934=CARTESIAN_POINT('Ctrl Pts',(-4.03445411510403,1.,0.144448947038352));
#63935=CARTESIAN_POINT('Ctrl Pts',(-4.02722143147048,-1.,0.146967602878998));
#63936=CARTESIAN_POINT('Ctrl Pts',(-4.02722143147048,1.,0.146967602878998));
#63937=CARTESIAN_POINT('Ctrl Pts',(-4.01998203715588,-1.,0.149445144968707));
#63938=CARTESIAN_POINT('Ctrl Pts',(-4.01998203715588,1.,0.149445144968707));
#63939=CARTESIAN_POINT('Ctrl Pts',(-4.01273584234684,-1.,0.151881094022909));
#63940=CARTESIAN_POINT('Ctrl Pts',(-4.01273584234684,1.,0.151881094022909));
#63941=CARTESIAN_POINT('Ctrl Pts',(-4.00548360245297,-1.,0.15427500487231));
#63942=CARTESIAN_POINT('Ctrl Pts',(-4.00548360245297,1.,0.15427500487231));
#63943=CARTESIAN_POINT('Ctrl Pts',(-3.99822717425869,-1.,0.156626481393735));
#63944=CARTESIAN_POINT('Ctrl Pts',(-3.99822717425869,1.,0.156626481393735));
#63945=CARTESIAN_POINT('Ctrl Pts',(-3.99096873945862,-1.,0.158935123982796));
#63946=CARTESIAN_POINT('Ctrl Pts',(-3.99096873945862,1.,0.158935123982796));
#63947=CARTESIAN_POINT('Ctrl Pts',(-3.98371010319866,-1.,0.161200482186087));
#63948=CARTESIAN_POINT('Ctrl Pts',(-3.98371010319866,1.,0.161200482186087));
#63949=CARTESIAN_POINT('Ctrl Pts',(-3.97645194630944,-1.,0.163422004609999));
#63950=CARTESIAN_POINT('Ctrl Pts',(-3.97645194630944,1.,0.163422004609999));
#63951=CARTESIAN_POINT('Ctrl Pts',(-3.9691931362141,-1.,0.165598992851097));
#63952=CARTESIAN_POINT('Ctrl Pts',(-3.9691931362141,1.,0.165598992851097));
#63953=CARTESIAN_POINT('Ctrl Pts',(-3.96192990160296,-1.,0.167730547023312));
#63954=CARTESIAN_POINT('Ctrl Pts',(-3.96192990160296,1.,0.167730547023312));
#63955=CARTESIAN_POINT('Ctrl Pts',(-3.95465744665263,-1.,0.16981566637413));
#63956=CARTESIAN_POINT('Ctrl Pts',(-3.95465744665263,1.,0.16981566637413));
#63957=CARTESIAN_POINT('Ctrl Pts',(-3.94737164900861,-1.,0.171853355369233));
#63958=CARTESIAN_POINT('Ctrl Pts',(-3.94737164900861,1.,0.171853355369233));
#63959=CARTESIAN_POINT('Ctrl Pts',(-3.94007083096214,-1.,0.173842734974607));
#63960=CARTESIAN_POINT('Ctrl Pts',(-3.94007083096214,1.,0.173842734974607));
#63961=CARTESIAN_POINT('Ctrl Pts',(-3.93275726771049,-1.,0.175783136893872));
#63962=CARTESIAN_POINT('Ctrl Pts',(-3.93275726771049,1.,0.175783136893872));
#63963=CARTESIAN_POINT('Ctrl Pts',(-3.92543942697672,-1.,0.177674246152328));
#63964=CARTESIAN_POINT('Ctrl Pts',(-3.92543942697672,1.,0.177674246152328));
#63965=CARTESIAN_POINT('Ctrl Pts',(-3.91812876180948,-1.,0.179515885822894));
#63966=CARTESIAN_POINT('Ctrl Pts',(-3.91812876180948,1.,0.179515885822894));
#63967=CARTESIAN_POINT('Ctrl Pts',(-3.91083557557193,-1.,0.181307740731796));
#63968=CARTESIAN_POINT('Ctrl Pts',(-3.91083557557193,1.,0.181307740731796));
#63969=CARTESIAN_POINT('Ctrl Pts',(-3.90356488555138,-1.,0.183049081993193));
#63970=CARTESIAN_POINT('Ctrl Pts',(-3.90356488555138,1.,0.183049081993193));
#63971=CARTESIAN_POINT('Ctrl Pts',(-3.89631300742633,-1.,0.184738537728035));
#63972=CARTESIAN_POINT('Ctrl Pts',(-3.89631300742633,1.,0.184738537728035));
#63973=CARTESIAN_POINT('Ctrl Pts',(-3.88906196725817,-1.,0.186373724985263));
#63974=CARTESIAN_POINT('Ctrl Pts',(-3.88906196725817,1.,0.186373724985263));
#63975=CARTESIAN_POINT('Ctrl Pts',(-3.88178563496187,-1.,0.187951632512663));
#63976=CARTESIAN_POINT('Ctrl Pts',(-3.88178563496187,1.,0.187951632512663));
#63977=CARTESIAN_POINT('Ctrl Pts',(-3.87445976418377,-1.,0.189469253358254));
#63978=CARTESIAN_POINT('Ctrl Pts',(-3.87445976418377,1.,0.189469253358254));
#63979=CARTESIAN_POINT('Ctrl Pts',(-3.8670715862477,-1.,0.190924190418613));
#63980=CARTESIAN_POINT('Ctrl Pts',(-3.8670715862477,1.,0.190924190418613));
#63981=CARTESIAN_POINT('Ctrl Pts',(-3.85962774407652,-1.,0.192315153044979));
#63982=CARTESIAN_POINT('Ctrl Pts',(-3.85962774407652,1.,0.192315153044979));
#63983=CARTESIAN_POINT('Ctrl Pts',(-3.85216762264019,-1.,0.193642806777747));
#63984=CARTESIAN_POINT('Ctrl Pts',(-3.85216762264019,1.,0.193642806777747));
#63985=CARTESIAN_POINT('Ctrl Pts',(-3.84475203347052,-1.,0.194909009460254));
#63986=CARTESIAN_POINT('Ctrl Pts',(-3.84475203347052,1.,0.194909009460254));
#63987=CARTESIAN_POINT('Ctrl Pts',(-3.83743910616265,-1.,0.196115198971889));
#63988=CARTESIAN_POINT('Ctrl Pts',(-3.83743910616265,1.,0.196115198971889));
#63989=CARTESIAN_POINT('Ctrl Pts',(-3.83026221776488,-1.,0.197260935827375));
#63990=CARTESIAN_POINT('Ctrl Pts',(-3.83026221776488,1.,0.197260935827375));
#63991=CARTESIAN_POINT('Ctrl Pts',(-3.82321127348981,-1.,0.19834261690047));
#63992=CARTESIAN_POINT('Ctrl Pts',(-3.82321127348981,1.,0.19834261690047));
#63993=CARTESIAN_POINT('Ctrl Pts',(-3.81620203429702,-1.,0.199351525297396));
#63994=CARTESIAN_POINT('Ctrl Pts',(-3.81620203429702,1.,0.199351525297396));
#63995=CARTESIAN_POINT('Ctrl Pts',(-3.80909529318501,-1.,0.20027467943329));
#63996=CARTESIAN_POINT('Ctrl Pts',(-3.80909529318501,1.,0.20027467943329));
#63997=CARTESIAN_POINT('Ctrl Pts',(-3.80175247447171,-1.,0.201097756307252));
#63998=CARTESIAN_POINT('Ctrl Pts',(-3.80175247447171,1.,0.201097756307252));
#63999=CARTESIAN_POINT('Ctrl Pts',(-3.79408354187274,-1.,0.201807533800799));
#64000=CARTESIAN_POINT('Ctrl Pts',(-3.79408354187274,1.,0.201807533800799));
#64001=CARTESIAN_POINT('Ctrl Pts',(-3.78609175019317,-1.,0.202394260512193));
#64002=CARTESIAN_POINT('Ctrl Pts',(-3.78609175019317,1.,0.202394260512193));
#64003=CARTESIAN_POINT('Ctrl Pts',(-3.77793553476879,-1.,0.202854729699196));
#64004=CARTESIAN_POINT('Ctrl Pts',(-3.77793553476879,1.,0.202854729699196));
#64005=CARTESIAN_POINT('Ctrl Pts',(-3.76992071595267,-1.,0.203192390045337));
#64006=CARTESIAN_POINT('Ctrl Pts',(-3.76992071595267,1.,0.203192390045337));
#64007=CARTESIAN_POINT('Ctrl Pts',(-3.76242717937273,-1.,0.203414634707646));
#64008=CARTESIAN_POINT('Ctrl Pts',(-3.76242717937273,1.,0.203414634707646));
#64009=CARTESIAN_POINT('Ctrl Pts',(-3.75585118707924,-1.,0.203530796848403));
#64010=CARTESIAN_POINT('Ctrl Pts',(-3.75585118707924,1.,0.203530796848403));
#64011=CARTESIAN_POINT('Ctrl Pts',(-3.75054693397716,-1.,0.203550035479097));
#64012=CARTESIAN_POINT('Ctrl Pts',(-3.75054693397716,1.,0.203550035479097));
#64013=CARTESIAN_POINT('Ctrl Pts',(-3.74675472018582,-1.,0.203478844530229));
#64014=CARTESIAN_POINT('Ctrl Pts',(-3.74675472018582,1.,0.203478844530229));
#64015=CARTESIAN_POINT('Ctrl Pts',(-3.7450208092684,-1.,0.203352057956055));
#64016=CARTESIAN_POINT('Ctrl Pts',(-3.7450208092684,1.,0.203352057956055));
#64017=CARTESIAN_POINT('Ctrl Pts',(-3.74446880195845,-1.,0.203218215747894));
#64018=CARTESIAN_POINT('Ctrl Pts',(-3.74446880195845,1.,0.203218215747894));
#64019=CARTESIAN_POINT('Ctrl Pts',(-3.74443319346666,-1.,0.20311176758786));
#64020=CARTESIAN_POINT('Ctrl Pts',(-3.74443319346666,1.,0.20311176758786));
#64021=CARTESIAN_POINT('Ctrl Pts',(-3.74449849461127,-1.,0.203054238699719));
#64022=CARTESIAN_POINT('Ctrl Pts',(-3.74449849461127,1.,0.203054238699719));
#64023=CARTESIAN_POINT('',(-4.19931119685982,1.,0.0760622897878236));
#64024=CARTESIAN_POINT('Ctrl Pts',(-4.19931119685982,1.,0.0760622897878236));
#64025=CARTESIAN_POINT('Ctrl Pts',(-4.19789138621624,1.,0.0767384596142195));
#64026=CARTESIAN_POINT('Ctrl Pts',(-4.19505112860624,1.,0.0780873956244402));
#64027=CARTESIAN_POINT('Ctrl Pts',(-4.19078883322483,1.,0.0801005887117603));
#64028=CARTESIAN_POINT('Ctrl Pts',(-4.1851019532944,1.,0.082764416438951));
#64029=CARTESIAN_POINT('Ctrl Pts',(-4.17798698669991,1.,0.0860600915552515));
#64030=CARTESIAN_POINT('Ctrl Pts',(-4.17086566491823,1.,0.0893215560850327));
#64031=CARTESIAN_POINT('Ctrl Pts',(-4.16373802265942,1.,0.092548667216769));
#64032=CARTESIAN_POINT('Ctrl Pts',(-4.15660412653006,1.,0.0957412403297067));
#64033=CARTESIAN_POINT('Ctrl Pts',(-4.1494640891762,1.,0.0988990478899811));
#64034=CARTESIAN_POINT('Ctrl Pts',(-4.14231804938737,1.,0.102021826577454));
#64035=CARTESIAN_POINT('Ctrl Pts',(-4.13516614458396,1.,0.105109286538864));
#64036=CARTESIAN_POINT('Ctrl Pts',(-4.12800848371386,1.,0.10816112052835));
#64037=CARTESIAN_POINT('Ctrl Pts',(-4.12084512502444,1.,0.111177012683377));
#64038=CARTESIAN_POINT('Ctrl Pts',(-4.11367603925313,1.,0.114156649609601));
#64039=CARTESIAN_POINT('Ctrl Pts',(-4.10650113382187,1.,0.117099722731704));
#64040=CARTESIAN_POINT('Ctrl Pts',(-4.09932031767243,1.,0.120005924388162));
#64041=CARTESIAN_POINT('Ctrl Pts',(-4.09213355850836,1.,0.122874946249119));
#64042=CARTESIAN_POINT('Ctrl Pts',(-4.08494093372315,1.,0.125706476822529));
#64043=CARTESIAN_POINT('Ctrl Pts',(-4.07774270738809,1.,0.128500200484814));
#64044=CARTESIAN_POINT('Ctrl Pts',(-4.07053931528579,1.,0.131255793548914));
#64045=CARTESIAN_POINT('Ctrl Pts',(-4.06333121018476,1.,0.133972916144225));
#64046=CARTESIAN_POINT('Ctrl Pts',(-4.05611873400122,1.,0.136651205046111));
#64047=CARTESIAN_POINT('Ctrl Pts',(-4.04890199238056,1.,0.139290267180059));
#64048=CARTESIAN_POINT('Ctrl Pts',(-4.04168069633842,1.,0.141889671485508));
#64049=CARTESIAN_POINT('Ctrl Pts',(-4.03445411510403,1.,0.144448947038352));
#64050=CARTESIAN_POINT('Ctrl Pts',(-4.02722143147048,1.,0.146967602878998));
#64051=CARTESIAN_POINT('Ctrl Pts',(-4.01998203715588,1.,0.149445144968707));
#64052=CARTESIAN_POINT('Ctrl Pts',(-4.01273584234684,1.,0.151881094022909));
#64053=CARTESIAN_POINT('Ctrl Pts',(-4.00548360245297,1.,0.15427500487231));
#64054=CARTESIAN_POINT('Ctrl Pts',(-3.99822717425869,1.,0.156626481393735));
#64055=CARTESIAN_POINT('Ctrl Pts',(-3.99096873945862,1.,0.158935123982796));
#64056=CARTESIAN_POINT('Ctrl Pts',(-3.98371010319866,1.,0.161200482186087));
#64057=CARTESIAN_POINT('Ctrl Pts',(-3.97645194630944,1.,0.163422004609999));
#64058=CARTESIAN_POINT('Ctrl Pts',(-3.9691931362141,1.,0.165598992851097));
#64059=CARTESIAN_POINT('Ctrl Pts',(-3.96192990160296,1.,0.167730547023312));
#64060=CARTESIAN_POINT('Ctrl Pts',(-3.95465744665263,1.,0.16981566637413));
#64061=CARTESIAN_POINT('Ctrl Pts',(-3.94737164900861,1.,0.171853355369233));
#64062=CARTESIAN_POINT('Ctrl Pts',(-3.94007083096214,1.,0.173842734974607));
#64063=CARTESIAN_POINT('Ctrl Pts',(-3.93275726771049,1.,0.175783136893872));
#64064=CARTESIAN_POINT('Ctrl Pts',(-3.92543942697672,1.,0.177674246152328));
#64065=CARTESIAN_POINT('Ctrl Pts',(-3.91812876180948,1.,0.179515885822894));
#64066=CARTESIAN_POINT('Ctrl Pts',(-3.91083557557193,1.,0.181307740731796));
#64067=CARTESIAN_POINT('Ctrl Pts',(-3.90356488555138,1.,0.183049081993193));
#64068=CARTESIAN_POINT('Ctrl Pts',(-3.89631300742633,1.,0.184738537728035));
#64069=CARTESIAN_POINT('Ctrl Pts',(-3.88906196725817,1.,0.186373724985263));
#64070=CARTESIAN_POINT('Ctrl Pts',(-3.88178563496187,1.,0.187951632512663));
#64071=CARTESIAN_POINT('Ctrl Pts',(-3.87445976418377,1.,0.189469253358254));
#64072=CARTESIAN_POINT('Ctrl Pts',(-3.8670715862477,1.,0.190924190418613));
#64073=CARTESIAN_POINT('Ctrl Pts',(-3.85962774407652,1.,0.192315153044979));
#64074=CARTESIAN_POINT('Ctrl Pts',(-3.85216762264019,1.,0.193642806777747));
#64075=CARTESIAN_POINT('Ctrl Pts',(-3.84475203347052,1.,0.194909009460254));
#64076=CARTESIAN_POINT('Ctrl Pts',(-3.83743910616265,1.,0.196115198971889));
#64077=CARTESIAN_POINT('Ctrl Pts',(-3.83026221776488,1.,0.197260935827375));
#64078=CARTESIAN_POINT('Ctrl Pts',(-3.82321127348981,1.,0.19834261690047));
#64079=CARTESIAN_POINT('Ctrl Pts',(-3.81620203429702,1.,0.199351525297396));
#64080=CARTESIAN_POINT('Ctrl Pts',(-3.80909529318501,1.,0.20027467943329));
#64081=CARTESIAN_POINT('Ctrl Pts',(-3.80175247447171,1.,0.201097756307252));
#64082=CARTESIAN_POINT('Ctrl Pts',(-3.79408354187274,1.,0.201807533800799));
#64083=CARTESIAN_POINT('Ctrl Pts',(-3.78609175019317,1.,0.202394260512193));
#64084=CARTESIAN_POINT('Ctrl Pts',(-3.77793553476879,1.,0.202854729699196));
#64085=CARTESIAN_POINT('Ctrl Pts',(-3.76992071595267,1.,0.203192390045337));
#64086=CARTESIAN_POINT('Ctrl Pts',(-3.76242717937273,1.,0.203414634707646));
#64087=CARTESIAN_POINT('Ctrl Pts',(-3.75585118707924,1.,0.203530796848403));
#64088=CARTESIAN_POINT('Ctrl Pts',(-3.75054693397716,1.,0.203550035479097));
#64089=CARTESIAN_POINT('Ctrl Pts',(-3.74703926501843,1.,0.203484186269314));
#64090=CARTESIAN_POINT('Ctrl Pts',(-3.74535749969262,1.,0.203375226874331));
#64091=CARTESIAN_POINT('Ctrl Pts',(-3.74471097893961,1.,0.203266610111264));
#64092=CARTESIAN_POINT('Ctrl Pts',(-3.74453008995129,1.,0.203188003947965));
#64093=CARTESIAN_POINT('Ctrl Pts',(-3.74449296982994,1.,0.203156094897896));
#64094=CARTESIAN_POINT('',(-4.19931119685982,0.,0.0760622897878236));
#64095=CARTESIAN_POINT('Ctrl Pts',(-3.74449849461127,-1.,-0.20305423869972));
#64096=CARTESIAN_POINT('Ctrl Pts',(-3.74449849461127,1.,-0.20305423869972));
#64097=CARTESIAN_POINT('Ctrl Pts',(-3.7444331934681,-1.,-0.203111767587923));
#64098=CARTESIAN_POINT('Ctrl Pts',(-3.7444331934681,1.,-0.203111767587923));
#64099=CARTESIAN_POINT('Ctrl Pts',(-3.7444688019622,-1.,-0.203218215748059));
#64100=CARTESIAN_POINT('Ctrl Pts',(-3.7444688019622,1.,-0.203218215748059));
#64101=CARTESIAN_POINT('Ctrl Pts',(-3.74502080927395,-1.,-0.203352057956297));
#64102=CARTESIAN_POINT('Ctrl Pts',(-3.74502080927395,1.,-0.203352057956297));
#64103=CARTESIAN_POINT('Ctrl Pts',(-3.7467547201908,-1.,-0.203478844530447));
#64104=CARTESIAN_POINT('Ctrl Pts',(-3.7467547201908,1.,-0.203478844530447));
#64105=CARTESIAN_POINT('Ctrl Pts',(-3.75054693397875,-1.,-0.203550035479166));
#64106=CARTESIAN_POINT('Ctrl Pts',(-3.75054693397875,1.,-0.203550035479166));
#64107=CARTESIAN_POINT('Ctrl Pts',(-3.75585118707734,-1.,-0.203530796848322));
#64108=CARTESIAN_POINT('Ctrl Pts',(-3.75585118707734,1.,-0.203530796848322));
#64109=CARTESIAN_POINT('Ctrl Pts',(-3.76242717936885,-1.,-0.203414634707478));
#64110=CARTESIAN_POINT('Ctrl Pts',(-3.76242717936885,1.,-0.203414634707478));
#64111=CARTESIAN_POINT('Ctrl Pts',(-3.7699207159487,-1.,-0.203192390045164));
#64112=CARTESIAN_POINT('Ctrl Pts',(-3.7699207159487,1.,-0.203192390045164));
#64113=CARTESIAN_POINT('Ctrl Pts',(-3.77793553476614,-1.,-0.202854729699081));
#64114=CARTESIAN_POINT('Ctrl Pts',(-3.77793553476614,1.,-0.202854729699081));
#64115=CARTESIAN_POINT('Ctrl Pts',(-3.78609175019242,-1.,-0.20239426051216));
#64116=CARTESIAN_POINT('Ctrl Pts',(-3.78609175019242,1.,-0.20239426051216));
#64117=CARTESIAN_POINT('Ctrl Pts',(-3.7940835418736,-1.,-0.201807533800837));
#64118=CARTESIAN_POINT('Ctrl Pts',(-3.7940835418736,1.,-0.201807533800837));
#64119=CARTESIAN_POINT('Ctrl Pts',(-3.80175247447337,-1.,-0.201097756307326));
#64120=CARTESIAN_POINT('Ctrl Pts',(-3.80175247447337,1.,-0.201097756307326));
#64121=CARTESIAN_POINT('Ctrl Pts',(-3.80909529318669,-1.,-0.200274679433364));
#64122=CARTESIAN_POINT('Ctrl Pts',(-3.80909529318669,1.,-0.200274679433364));
#64123=CARTESIAN_POINT('Ctrl Pts',(-3.81620203429815,-1.,-0.199351525297447));
#64124=CARTESIAN_POINT('Ctrl Pts',(-3.81620203429815,1.,-0.199351525297447));
#64125=CARTESIAN_POINT('Ctrl Pts',(-3.82321127349016,-1.,-0.198342616900486));
#64126=CARTESIAN_POINT('Ctrl Pts',(-3.82321127349016,1.,-0.198342616900486));
#64127=CARTESIAN_POINT('Ctrl Pts',(-3.83026221776456,-1.,-0.197260935827361));
#64128=CARTESIAN_POINT('Ctrl Pts',(-3.83026221776456,1.,-0.197260935827361));
#64129=CARTESIAN_POINT('Ctrl Pts',(-3.83743910616195,-1.,-0.196115198971859));
#64130=CARTESIAN_POINT('Ctrl Pts',(-3.83743910616195,1.,-0.196115198971859));
#64131=CARTESIAN_POINT('Ctrl Pts',(-3.84475203346977,-1.,-0.194909009460221));
#64132=CARTESIAN_POINT('Ctrl Pts',(-3.84475203346977,1.,-0.194909009460221));
#64133=CARTESIAN_POINT('Ctrl Pts',(-3.85216762263966,-1.,-0.193642806777723));
#64134=CARTESIAN_POINT('Ctrl Pts',(-3.85216762263966,1.,-0.193642806777723));
#64135=CARTESIAN_POINT('Ctrl Pts',(-3.85962774407633,-1.,-0.192315153044971));
#64136=CARTESIAN_POINT('Ctrl Pts',(-3.85962774407633,1.,-0.192315153044971));
#64137=CARTESIAN_POINT('Ctrl Pts',(-3.86707158624783,-1.,-0.19092419041862));
#64138=CARTESIAN_POINT('Ctrl Pts',(-3.86707158624783,1.,-0.19092419041862));
#64139=CARTESIAN_POINT('Ctrl Pts',(-3.87445976418412,-1.,-0.189469253358272));
#64140=CARTESIAN_POINT('Ctrl Pts',(-3.87445976418412,1.,-0.189469253358272));
#64141=CARTESIAN_POINT('Ctrl Pts',(-3.88178563496228,-1.,-0.187951632512685));
#64142=CARTESIAN_POINT('Ctrl Pts',(-3.88178563496228,1.,-0.187951632512685));
#64143=CARTESIAN_POINT('Ctrl Pts',(-3.88906196725848,-1.,-0.18637372498528));
#64144=CARTESIAN_POINT('Ctrl Pts',(-3.88906196725848,1.,-0.18637372498528));
#64145=CARTESIAN_POINT('Ctrl Pts',(-3.89631300742646,-1.,-0.184738537728043));
#64146=CARTESIAN_POINT('Ctrl Pts',(-3.89631300742646,1.,-0.184738537728043));
#64147=CARTESIAN_POINT('Ctrl Pts',(-3.90356488555132,-1.,-0.183049081993191));
#64148=CARTESIAN_POINT('Ctrl Pts',(-3.90356488555132,1.,-0.183049081993191));
#64149=CARTESIAN_POINT('Ctrl Pts',(-3.91083557557175,-1.,-0.181307740731786));
#64150=CARTESIAN_POINT('Ctrl Pts',(-3.91083557557175,1.,-0.181307740731786));
#64151=CARTESIAN_POINT('Ctrl Pts',(-3.91812876180926,-1.,-0.179515885822882));
#64152=CARTESIAN_POINT('Ctrl Pts',(-3.91812876180926,1.,-0.179515885822882));
#64153=CARTESIAN_POINT('Ctrl Pts',(-3.92543942697655,-1.,-0.177674246152317));
#64154=CARTESIAN_POINT('Ctrl Pts',(-3.92543942697655,1.,-0.177674246152317));
#64155=CARTESIAN_POINT('Ctrl Pts',(-3.93275726771042,-1.,-0.175783136893868));
#64156=CARTESIAN_POINT('Ctrl Pts',(-3.93275726771042,1.,-0.175783136893868));
#64157=CARTESIAN_POINT('Ctrl Pts',(-3.94007083096217,-1.,-0.17384273497461));
#64158=CARTESIAN_POINT('Ctrl Pts',(-3.94007083096217,1.,-0.17384273497461));
#64159=CARTESIAN_POINT('Ctrl Pts',(-3.94737164900868,-1.,-0.17185335536924));
#64160=CARTESIAN_POINT('Ctrl Pts',(-3.94737164900868,1.,-0.17185335536924));
#64161=CARTESIAN_POINT('Ctrl Pts',(-3.95465744665268,-1.,-0.169815666374139));
#64162=CARTESIAN_POINT('Ctrl Pts',(-3.95465744665268,1.,-0.169815666374139));
#64163=CARTESIAN_POINT('Ctrl Pts',(-3.96192990160296,-1.,-0.167730547023319));
#64164=CARTESIAN_POINT('Ctrl Pts',(-3.96192990160296,1.,-0.167730547023319));
#64165=CARTESIAN_POINT('Ctrl Pts',(-3.96919313621407,-1.,-0.165598992851102));
#64166=CARTESIAN_POINT('Ctrl Pts',(-3.96919313621407,1.,-0.165598992851102));
#64167=CARTESIAN_POINT('Ctrl Pts',(-3.97645194630943,-1.,-0.163422004609999));
#64168=CARTESIAN_POINT('Ctrl Pts',(-3.97645194630943,1.,-0.163422004609999));
#64169=CARTESIAN_POINT('Ctrl Pts',(-3.98371010319872,-1.,-0.161200482186085));
#64170=CARTESIAN_POINT('Ctrl Pts',(-3.98371010319872,1.,-0.161200482186085));
#64171=CARTESIAN_POINT('Ctrl Pts',(-3.99096873945878,-1.,-0.158935123982793));
#64172=CARTESIAN_POINT('Ctrl Pts',(-3.99096873945878,1.,-0.158935123982793));
#64173=CARTESIAN_POINT('Ctrl Pts',(-3.99822717425893,-1.,-0.156626481393734));
#64174=CARTESIAN_POINT('Ctrl Pts',(-3.99822717425893,1.,-0.156626481393734));
#64175=CARTESIAN_POINT('Ctrl Pts',(-4.00548360245319,-1.,-0.154275004872311));
#64176=CARTESIAN_POINT('Ctrl Pts',(-4.00548360245319,1.,-0.154275004872311));
#64177=CARTESIAN_POINT('Ctrl Pts',(-4.01273584234689,-1.,-0.151881094022911));
#64178=CARTESIAN_POINT('Ctrl Pts',(-4.01273584234689,1.,-0.151881094022911));
#64179=CARTESIAN_POINT('Ctrl Pts',(-4.01998203715564,-1.,-0.149445144968707));
#64180=CARTESIAN_POINT('Ctrl Pts',(-4.01998203715564,1.,-0.149445144968707));
#64181=CARTESIAN_POINT('Ctrl Pts',(-4.02722143146994,-1.,-0.146967602878994));
#64182=CARTESIAN_POINT('Ctrl Pts',(-4.02722143146994,1.,-0.146967602878994));
#64183=CARTESIAN_POINT('Ctrl Pts',(-4.03445411510333,-1.,-0.144448947038345));
#64184=CARTESIAN_POINT('Ctrl Pts',(-4.03445411510333,1.,-0.144448947038345));
#64185=CARTESIAN_POINT('Ctrl Pts',(-4.04168069633781,-1.,-0.1418896714855));
#64186=CARTESIAN_POINT('Ctrl Pts',(-4.04168069633781,1.,-0.1418896714855));
#64187=CARTESIAN_POINT('Ctrl Pts',(-4.04890199238036,-1.,-0.139290267180057));
#64188=CARTESIAN_POINT('Ctrl Pts',(-4.04890199238036,1.,-0.139290267180057));
#64189=CARTESIAN_POINT('Ctrl Pts',(-4.05611873400172,-1.,-0.136651205046119));
#64190=CARTESIAN_POINT('Ctrl Pts',(-4.05611873400172,1.,-0.136651205046119));
#64191=CARTESIAN_POINT('Ctrl Pts',(-4.06333121018596,-1.,-0.133972916144245));
#64192=CARTESIAN_POINT('Ctrl Pts',(-4.06333121018596,1.,-0.133972916144245));
#64193=CARTESIAN_POINT('Ctrl Pts',(-4.0705393152874,-1.,-0.13125579354894));
#64194=CARTESIAN_POINT('Ctrl Pts',(-4.0705393152874,1.,-0.13125579354894));
#64195=CARTESIAN_POINT('Ctrl Pts',(-4.07774270738954,-1.,-0.128500200484838));
#64196=CARTESIAN_POINT('Ctrl Pts',(-4.07774270738954,1.,-0.128500200484838));
#64197=CARTESIAN_POINT('Ctrl Pts',(-4.08494093372377,-1.,-0.12570647682254));
#64198=CARTESIAN_POINT('Ctrl Pts',(-4.08494093372377,1.,-0.12570647682254));
#64199=CARTESIAN_POINT('Ctrl Pts',(-4.09213355850756,-1.,-0.122874946249107));
#64200=CARTESIAN_POINT('Ctrl Pts',(-4.09213355850756,1.,-0.122874946249107));
#64201=CARTESIAN_POINT('Ctrl Pts',(-4.09932031767002,-1.,-0.120005924388124));
#64202=CARTESIAN_POINT('Ctrl Pts',(-4.09932031767002,1.,-0.120005924388124));
#64203=CARTESIAN_POINT('Ctrl Pts',(-4.10650113381833,-1.,-0.117099722731648));
#64204=CARTESIAN_POINT('Ctrl Pts',(-4.10650113381833,1.,-0.117099722731648));
#64205=CARTESIAN_POINT('Ctrl Pts',(-4.11367603924961,-1.,-0.114156649609546));
#64206=CARTESIAN_POINT('Ctrl Pts',(-4.11367603924961,1.,-0.114156649609546));
#64207=CARTESIAN_POINT('Ctrl Pts',(-4.1208451250225,-1.,-0.111177012683347));
#64208=CARTESIAN_POINT('Ctrl Pts',(-4.1208451250225,1.,-0.111177012683347));
#64209=CARTESIAN_POINT('Ctrl Pts',(-4.12800848371504,-1.,-0.108161120528369));
#64210=CARTESIAN_POINT('Ctrl Pts',(-4.12800848371504,1.,-0.108161120528369));
#64211=CARTESIAN_POINT('Ctrl Pts',(-4.13516614458895,-1.,-0.105109286538945));
#64212=CARTESIAN_POINT('Ctrl Pts',(-4.13516614458895,1.,-0.105109286538945));
#64213=CARTESIAN_POINT('Ctrl Pts',(-4.14231804939538,-1.,-0.102021826577584));
#64214=CARTESIAN_POINT('Ctrl Pts',(-4.14231804939538,1.,-0.102021826577584));
#64215=CARTESIAN_POINT('Ctrl Pts',(-4.14946408918485,-1.,-0.0988990478901226));
#64216=CARTESIAN_POINT('Ctrl Pts',(-4.14946408918485,1.,-0.0988990478901226));
#64217=CARTESIAN_POINT('Ctrl Pts',(-4.15660412653577,-1.,-0.0957412403298007));
#64218=CARTESIAN_POINT('Ctrl Pts',(-4.15660412653577,1.,-0.0957412403298007));
#64219=CARTESIAN_POINT('Ctrl Pts',(-4.16373802265839,-1.,-0.0925486672167531));
#64220=CARTESIAN_POINT('Ctrl Pts',(-4.16373802265839,1.,-0.0925486672167531));
#64221=CARTESIAN_POINT('Ctrl Pts',(-4.17086566490794,-1.,-0.0893215560848649));
#64222=CARTESIAN_POINT('Ctrl Pts',(-4.17086566490794,1.,-0.0893215560848649));
#64223=CARTESIAN_POINT('Ctrl Pts',(-4.17798698668094,-1.,-0.0860600915549397));
#64224=CARTESIAN_POINT('Ctrl Pts',(-4.17798698668094,1.,-0.0860600915549397));
#64225=CARTESIAN_POINT('Ctrl Pts',(-4.18510195327123,-1.,-0.0827644164385679));
#64226=CARTESIAN_POINT('Ctrl Pts',(-4.18510195327123,1.,-0.0827644164385679));
#64227=CARTESIAN_POINT('Ctrl Pts',(-4.19078883320504,-1.,-0.080100588711432));
#64228=CARTESIAN_POINT('Ctrl Pts',(-4.19078883320504,1.,-0.080100588711432));
#64229=CARTESIAN_POINT('Ctrl Pts',(-4.19505112859416,-1.,-0.0780873956242397));
#64230=CARTESIAN_POINT('Ctrl Pts',(-4.19505112859416,1.,-0.0780873956242397));
#64231=CARTESIAN_POINT('Ctrl Pts',(-4.1978913862118,-1.,-0.0767384596141464));
#64232=CARTESIAN_POINT('Ctrl Pts',(-4.1978913862118,1.,-0.0767384596141464));
#64233=CARTESIAN_POINT('Ctrl Pts',(-4.19931119685982,-1.,-0.0760622897878246));
#64234=CARTESIAN_POINT('Ctrl Pts',(-4.19931119685982,1.,-0.0760622897878246));
#64235=CARTESIAN_POINT('',(-3.74449296983004,1.,-0.2031560948961));
#64236=CARTESIAN_POINT('Ctrl Pts',(-3.74449296983004,-1.,-0.203156094896101));
#64237=CARTESIAN_POINT('Ctrl Pts',(-3.74449296983004,-0.666666666666667,
-0.203156094896101));
#64238=CARTESIAN_POINT('Ctrl Pts',(-3.74449296983004,-0.333333333333333,
-0.203156094896101));
#64239=CARTESIAN_POINT('Ctrl Pts',(-3.74449296983004,0.333333333333333,
-0.203156094896101));
#64240=CARTESIAN_POINT('Ctrl Pts',(-3.74449296983004,0.666666666666667,
-0.203156094896101));
#64241=CARTESIAN_POINT('Ctrl Pts',(-3.74449296983004,1.,-0.203156094896101));
#64242=CARTESIAN_POINT('',(-4.19931119685982,1.,-0.0760622897878246));
#64243=CARTESIAN_POINT('',(-4.19931119685982,0.,-0.0760622897878246));
#64244=CARTESIAN_POINT('Ctrl Pts',(-3.74449296983004,1.,-0.203156094896101));
#64245=CARTESIAN_POINT('Ctrl Pts',(-3.74453008995092,1.,-0.203188003946657));
#64246=CARTESIAN_POINT('Ctrl Pts',(-3.74471097893844,1.,-0.203266610110531));
#64247=CARTESIAN_POINT('Ctrl Pts',(-3.74535749969115,1.,-0.203375226874121));
#64248=CARTESIAN_POINT('Ctrl Pts',(-3.74703926501752,1.,-0.203484186269415));
#64249=CARTESIAN_POINT('Ctrl Pts',(-3.75054693397875,1.,-0.203550035479166));
#64250=CARTESIAN_POINT('Ctrl Pts',(-3.75585118707734,1.,-0.203530796848322));
#64251=CARTESIAN_POINT('Ctrl Pts',(-3.76242717936885,1.,-0.203414634707478));
#64252=CARTESIAN_POINT('Ctrl Pts',(-3.7699207159487,1.,-0.203192390045164));
#64253=CARTESIAN_POINT('Ctrl Pts',(-3.77793553476614,1.,-0.202854729699081));
#64254=CARTESIAN_POINT('Ctrl Pts',(-3.78609175019242,1.,-0.20239426051216));
#64255=CARTESIAN_POINT('Ctrl Pts',(-3.7940835418736,1.,-0.201807533800837));
#64256=CARTESIAN_POINT('Ctrl Pts',(-3.80175247447337,1.,-0.201097756307326));
#64257=CARTESIAN_POINT('Ctrl Pts',(-3.80909529318669,1.,-0.200274679433364));
#64258=CARTESIAN_POINT('Ctrl Pts',(-3.81620203429815,1.,-0.199351525297447));
#64259=CARTESIAN_POINT('Ctrl Pts',(-3.82321127349016,1.,-0.198342616900486));
#64260=CARTESIAN_POINT('Ctrl Pts',(-3.83026221776456,1.,-0.197260935827361));
#64261=CARTESIAN_POINT('Ctrl Pts',(-3.83743910616195,1.,-0.196115198971859));
#64262=CARTESIAN_POINT('Ctrl Pts',(-3.84475203346977,1.,-0.194909009460221));
#64263=CARTESIAN_POINT('Ctrl Pts',(-3.85216762263966,1.,-0.193642806777723));
#64264=CARTESIAN_POINT('Ctrl Pts',(-3.85962774407633,1.,-0.192315153044971));
#64265=CARTESIAN_POINT('Ctrl Pts',(-3.86707158624783,1.,-0.19092419041862));
#64266=CARTESIAN_POINT('Ctrl Pts',(-3.87445976418412,1.,-0.189469253358272));
#64267=CARTESIAN_POINT('Ctrl Pts',(-3.88178563496228,1.,-0.187951632512685));
#64268=CARTESIAN_POINT('Ctrl Pts',(-3.88906196725848,1.,-0.18637372498528));
#64269=CARTESIAN_POINT('Ctrl Pts',(-3.89631300742646,1.,-0.184738537728043));
#64270=CARTESIAN_POINT('Ctrl Pts',(-3.90356488555132,1.,-0.183049081993191));
#64271=CARTESIAN_POINT('Ctrl Pts',(-3.91083557557175,1.,-0.181307740731786));
#64272=CARTESIAN_POINT('Ctrl Pts',(-3.91812876180926,1.,-0.179515885822882));
#64273=CARTESIAN_POINT('Ctrl Pts',(-3.92543942697655,1.,-0.177674246152317));
#64274=CARTESIAN_POINT('Ctrl Pts',(-3.93275726771042,1.,-0.175783136893868));
#64275=CARTESIAN_POINT('Ctrl Pts',(-3.94007083096217,1.,-0.17384273497461));
#64276=CARTESIAN_POINT('Ctrl Pts',(-3.94737164900868,1.,-0.17185335536924));
#64277=CARTESIAN_POINT('Ctrl Pts',(-3.95465744665268,1.,-0.169815666374139));
#64278=CARTESIAN_POINT('Ctrl Pts',(-3.96192990160296,1.,-0.167730547023319));
#64279=CARTESIAN_POINT('Ctrl Pts',(-3.96919313621407,1.,-0.165598992851102));
#64280=CARTESIAN_POINT('Ctrl Pts',(-3.97645194630943,1.,-0.163422004609999));
#64281=CARTESIAN_POINT('Ctrl Pts',(-3.98371010319872,1.,-0.161200482186085));
#64282=CARTESIAN_POINT('Ctrl Pts',(-3.99096873945878,1.,-0.158935123982793));
#64283=CARTESIAN_POINT('Ctrl Pts',(-3.99822717425893,1.,-0.156626481393734));
#64284=CARTESIAN_POINT('Ctrl Pts',(-4.00548360245319,1.,-0.154275004872311));
#64285=CARTESIAN_POINT('Ctrl Pts',(-4.01273584234689,1.,-0.151881094022911));
#64286=CARTESIAN_POINT('Ctrl Pts',(-4.01998203715564,1.,-0.149445144968707));
#64287=CARTESIAN_POINT('Ctrl Pts',(-4.02722143146994,1.,-0.146967602878994));
#64288=CARTESIAN_POINT('Ctrl Pts',(-4.03445411510333,1.,-0.144448947038345));
#64289=CARTESIAN_POINT('Ctrl Pts',(-4.04168069633781,1.,-0.1418896714855));
#64290=CARTESIAN_POINT('Ctrl Pts',(-4.04890199238036,1.,-0.139290267180057));
#64291=CARTESIAN_POINT('Ctrl Pts',(-4.05611873400172,1.,-0.136651205046119));
#64292=CARTESIAN_POINT('Ctrl Pts',(-4.06333121018596,1.,-0.133972916144245));
#64293=CARTESIAN_POINT('Ctrl Pts',(-4.0705393152874,1.,-0.13125579354894));
#64294=CARTESIAN_POINT('Ctrl Pts',(-4.07774270738954,1.,-0.128500200484838));
#64295=CARTESIAN_POINT('Ctrl Pts',(-4.08494093372377,1.,-0.12570647682254));
#64296=CARTESIAN_POINT('Ctrl Pts',(-4.09213355850756,1.,-0.122874946249107));
#64297=CARTESIAN_POINT('Ctrl Pts',(-4.09932031767002,1.,-0.120005924388124));
#64298=CARTESIAN_POINT('Ctrl Pts',(-4.10650113381833,1.,-0.117099722731648));
#64299=CARTESIAN_POINT('Ctrl Pts',(-4.11367603924961,1.,-0.114156649609546));
#64300=CARTESIAN_POINT('Ctrl Pts',(-4.1208451250225,1.,-0.111177012683347));
#64301=CARTESIAN_POINT('Ctrl Pts',(-4.12800848371504,1.,-0.108161120528369));
#64302=CARTESIAN_POINT('Ctrl Pts',(-4.13516614458895,1.,-0.105109286538945));
#64303=CARTESIAN_POINT('Ctrl Pts',(-4.14231804939538,1.,-0.102021826577584));
#64304=CARTESIAN_POINT('Ctrl Pts',(-4.14946408918485,1.,-0.0988990478901226));
#64305=CARTESIAN_POINT('Ctrl Pts',(-4.15660412653577,1.,-0.0957412403298007));
#64306=CARTESIAN_POINT('Ctrl Pts',(-4.16373802265839,1.,-0.0925486672167531));
#64307=CARTESIAN_POINT('Ctrl Pts',(-4.17086566490794,1.,-0.0893215560848649));
#64308=CARTESIAN_POINT('Ctrl Pts',(-4.17798698668094,1.,-0.0860600915549397));
#64309=CARTESIAN_POINT('Ctrl Pts',(-4.18510195327123,1.,-0.0827644164385679));
#64310=CARTESIAN_POINT('Ctrl Pts',(-4.19078883320504,1.,-0.080100588711432));
#64311=CARTESIAN_POINT('Ctrl Pts',(-4.19505112859416,1.,-0.0780873956242397));
#64312=CARTESIAN_POINT('Ctrl Pts',(-4.1978913862118,1.,-0.0767384596141464));
#64313=CARTESIAN_POINT('Ctrl Pts',(-4.19931119685982,1.,-0.0760622897878246));
#64314=CARTESIAN_POINT('Origin',(-4.19931119685982,0.,-0.0760622897878246));
#64315=CARTESIAN_POINT('',(-4.19931119685982,1.,0.0760622897878236));
#64316=CARTESIAN_POINT('Origin',(0.,0.,0.));
#64317=CARTESIAN_POINT('',(-3.73017266276651,1.,-0.385112848330761));
#64318=CARTESIAN_POINT('Origin',(0.,1.,0.));
#64319=CARTESIAN_POINT('Ctrl Pts',(-3.73017266276651,1.,-0.385112848330762));
#64320=CARTESIAN_POINT('Ctrl Pts',(-3.73017266276651,0.666666666666667,
-0.385112848330762));
#64321=CARTESIAN_POINT('Ctrl Pts',(-3.73017266276651,0.333333333333333,
-0.385112848330762));
#64322=CARTESIAN_POINT('Ctrl Pts',(-3.73017266276651,-0.333333333333333,
-0.385112848330762));
#64323=CARTESIAN_POINT('Ctrl Pts',(-3.73017266276651,-0.666666666666667,
-0.385112848330762));
#64324=CARTESIAN_POINT('Ctrl Pts',(-3.73017266276651,-1.,-0.385112848330762));
#64325=CARTESIAN_POINT('Ctrl Pts',(-4.15950947128175,-1.,-0.581791163835815));
#64326=CARTESIAN_POINT('Ctrl Pts',(-4.15950947128175,1.,-0.581791163835815));
#64327=CARTESIAN_POINT('Ctrl Pts',(-4.1582129171283,-1.,-0.580901211463535));
#64328=CARTESIAN_POINT('Ctrl Pts',(-4.1582129171283,1.,-0.580901211463535));
#64329=CARTESIAN_POINT('Ctrl Pts',(-4.15561864788576,-1.,-0.579124568914235));
#64330=CARTESIAN_POINT('Ctrl Pts',(-4.15561864788576,1.,-0.579124568914235));
#64331=CARTESIAN_POINT('Ctrl Pts',(-4.151723761217,-1.,-0.576469391676688));
#64332=CARTESIAN_POINT('Ctrl Pts',(-4.151723761217,1.,-0.576469391676688));
#64333=CARTESIAN_POINT('Ctrl Pts',(-4.14652361068081,-1.,-0.572948736069522));
#64334=CARTESIAN_POINT('Ctrl Pts',(-4.14652361068081,1.,-0.572948736069522));
#64335=CARTESIAN_POINT('Ctrl Pts',(-4.14001179830547,-1.,-0.568580610189774));
#64336=CARTESIAN_POINT('Ctrl Pts',(-4.14001179830547,1.,-0.568580610189774));
#64337=CARTESIAN_POINT('Ctrl Pts',(-4.13348835727104,-1.,-0.564245279537148));
#64338=CARTESIAN_POINT('Ctrl Pts',(-4.13348835727104,1.,-0.564245279537148));
#64339=CARTESIAN_POINT('Ctrl Pts',(-4.12695329951961,-1.,-0.559942890594773));
#64340=CARTESIAN_POINT('Ctrl Pts',(-4.12695329951961,1.,-0.559942890594773));
#64341=CARTESIAN_POINT('Ctrl Pts',(-4.12040666195664,-1.,-0.555673636129977));
#64342=CARTESIAN_POINT('Ctrl Pts',(-4.12040666195664,1.,-0.555673636129977));
#64343=CARTESIAN_POINT('Ctrl Pts',(-4.11384852024721,-1.,-0.551437758497032));
#64344=CARTESIAN_POINT('Ctrl Pts',(-4.11384852024721,1.,-0.551437758497032));
#64345=CARTESIAN_POINT('Ctrl Pts',(-4.10727897027977,-1.,-0.547235539485637));
#64346=CARTESIAN_POINT('Ctrl Pts',(-4.10727897027977,1.,-0.547235539485637));
#64347=CARTESIAN_POINT('Ctrl Pts',(-4.10069810243979,-1.,-0.543067286877757));
#64348=CARTESIAN_POINT('Ctrl Pts',(-4.10069810243979,1.,-0.543067286877757));
#64349=CARTESIAN_POINT('Ctrl Pts',(-4.09410597627,-1.,-0.538933321179756));
#64350=CARTESIAN_POINT('Ctrl Pts',(-4.09410597627,1.,-0.538933321179756));
#64351=CARTESIAN_POINT('Ctrl Pts',(-4.08750259988885,-1.,-0.534833963477273));
#64352=CARTESIAN_POINT('Ctrl Pts',(-4.08750259988885,1.,-0.534833963477273));
#64353=CARTESIAN_POINT('Ctrl Pts',(-4.08088789536836,-1.,-0.530769518728571));
#64354=CARTESIAN_POINT('Ctrl Pts',(-4.08088789536836,1.,-0.530769518728571));
#64355=CARTESIAN_POINT('Ctrl Pts',(-4.07426172299847,-1.,-0.526740277227498));
#64356=CARTESIAN_POINT('Ctrl Pts',(-4.07426172299847,1.,-0.526740277227498));
#64357=CARTESIAN_POINT('Ctrl Pts',(-4.06762394471314,-1.,-0.522746528603107));
#64358=CARTESIAN_POINT('Ctrl Pts',(-4.06762394471314,1.,-0.522746528603107));
#64359=CARTESIAN_POINT('Ctrl Pts',(-4.06097448038013,-1.,-0.518788572336923));
#64360=CARTESIAN_POINT('Ctrl Pts',(-4.06097448038013,1.,-0.518788572336923));
#64361=CARTESIAN_POINT('Ctrl Pts',(-4.05431335771199,-1.,-0.514866728193017));
#64362=CARTESIAN_POINT('Ctrl Pts',(-4.05431335771199,1.,-0.514866728193017));
#64363=CARTESIAN_POINT('Ctrl Pts',(-4.04764078815447,-1.,-0.51098134921897));
#64364=CARTESIAN_POINT('Ctrl Pts',(-4.04764078815447,1.,-0.51098134921897));
#64365=CARTESIAN_POINT('Ctrl Pts',(-4.04095715148915,-1.,-0.507132823288136));
#64366=CARTESIAN_POINT('Ctrl Pts',(-4.04095715148915,1.,-0.507132823288136));
#64367=CARTESIAN_POINT('Ctrl Pts',(-4.03426284174272,-1.,-0.503321556915346));
#64368=CARTESIAN_POINT('Ctrl Pts',(-4.03426284174272,1.,-0.503321556915346));
#64369=CARTESIAN_POINT('Ctrl Pts',(-4.02755813980101,-1.,-0.499547962340821));
#64370=CARTESIAN_POINT('Ctrl Pts',(-4.02755813980101,1.,-0.499547962340821));
#64371=CARTESIAN_POINT('Ctrl Pts',(-4.02084308851832,-1.,-0.495812444326251));
#64372=CARTESIAN_POINT('Ctrl Pts',(-4.02084308851832,1.,-0.495812444326251));
#64373=CARTESIAN_POINT('Ctrl Pts',(-4.01411733503546,-1.,-0.492115383418018));
#64374=CARTESIAN_POINT('Ctrl Pts',(-4.01411733503546,1.,-0.492115383418018));
#64375=CARTESIAN_POINT('Ctrl Pts',(-4.0073800839099,-1.,-0.488457130424633));
#64376=CARTESIAN_POINT('Ctrl Pts',(-4.0073800839099,1.,-0.488457130424633));
#64377=CARTESIAN_POINT('Ctrl Pts',(-4.00063045119288,-1.,-0.484838042421835));
#64378=CARTESIAN_POINT('Ctrl Pts',(-4.00063045119288,1.,-0.484838042421835));
#64379=CARTESIAN_POINT('Ctrl Pts',(-3.99386775880679,-1.,-0.481258512209675));
#64380=CARTESIAN_POINT('Ctrl Pts',(-3.99386775880679,1.,-0.481258512209675));
#64381=CARTESIAN_POINT('Ctrl Pts',(-3.98709184306738,-1.,-0.477718999122027));
#64382=CARTESIAN_POINT('Ctrl Pts',(-3.98709184306738,1.,-0.477718999122027));
#64383=CARTESIAN_POINT('Ctrl Pts',(-3.98030338044409,-1.,-0.47422006101951));
#64384=CARTESIAN_POINT('Ctrl Pts',(-3.98030338044409,1.,-0.47422006101951));
#64385=CARTESIAN_POINT('Ctrl Pts',(-3.97350414289392,-1.,-0.470762379613439));
#64386=CARTESIAN_POINT('Ctrl Pts',(-3.97350414289392,1.,-0.470762379613439));
#64387=CARTESIAN_POINT('Ctrl Pts',(-3.9666962227393,-1.,-0.467346690880643));
#64388=CARTESIAN_POINT('Ctrl Pts',(-3.9666962227393,1.,-0.467346690880643));
#64389=CARTESIAN_POINT('Ctrl Pts',(-3.95988133243538,-1.,-0.463973722115733));
#64390=CARTESIAN_POINT('Ctrl Pts',(-3.95988133243538,1.,-0.463973722115733));
#64391=CARTESIAN_POINT('Ctrl Pts',(-3.95306005817364,-1.,-0.460644124429121));
#64392=CARTESIAN_POINT('Ctrl Pts',(-3.95306005817364,1.,-0.460644124429121));
#64393=CARTESIAN_POINT('Ctrl Pts',(-3.94623117206678,-1.,-0.457358410451683));
#64394=CARTESIAN_POINT('Ctrl Pts',(-3.94623117206678,1.,-0.457358410451683));
#64395=CARTESIAN_POINT('Ctrl Pts',(-3.93939080846298,-1.,-0.454116879027584));
#64396=CARTESIAN_POINT('Ctrl Pts',(-3.93939080846298,1.,-0.454116879027584));
#64397=CARTESIAN_POINT('Ctrl Pts',(-3.93253407403123,-1.,-0.450919768356348));
#64398=CARTESIAN_POINT('Ctrl Pts',(-3.93253407403123,1.,-0.450919768356348));
#64399=CARTESIAN_POINT('Ctrl Pts',(-3.92565674143416,-1.,-0.447767416837292));
#64400=CARTESIAN_POINT('Ctrl Pts',(-3.92565674143416,1.,-0.447767416837292));
#64401=CARTESIAN_POINT('Ctrl Pts',(-3.91875701610719,-1.,-0.444660430230591));
#64402=CARTESIAN_POINT('Ctrl Pts',(-3.91875701610719,1.,-0.444660430230591));
#64403=CARTESIAN_POINT('Ctrl Pts',(-3.91183704069153,-1.,-0.441599824524054));
#64404=CARTESIAN_POINT('Ctrl Pts',(-3.91183704069153,1.,-0.441599824524054));
#64405=CARTESIAN_POINT('Ctrl Pts',(-3.90490512938563,-1.,-0.438587235458249));
#64406=CARTESIAN_POINT('Ctrl Pts',(-3.90490512938563,1.,-0.438587235458249));
#64407=CARTESIAN_POINT('Ctrl Pts',(-3.89797256655462,-1.,-0.435624629433527));
#64408=CARTESIAN_POINT('Ctrl Pts',(-3.89797256655462,1.,-0.435624629433527));
#64409=CARTESIAN_POINT('Ctrl Pts',(-3.89104947940611,-1.,-0.432713929544458));
#64410=CARTESIAN_POINT('Ctrl Pts',(-3.89104947940611,1.,-0.432713929544458));
#64411=CARTESIAN_POINT('Ctrl Pts',(-3.88414070943341,-1.,-0.429856640579741));
#64412=CARTESIAN_POINT('Ctrl Pts',(-3.88414070943341,1.,-0.429856640579741));
#64413=CARTESIAN_POINT('Ctrl Pts',(-3.87724240306597,-1.,-0.427053541173457));
#64414=CARTESIAN_POINT('Ctrl Pts',(-3.87724240306597,1.,-0.427053541173457));
#64415=CARTESIAN_POINT('Ctrl Pts',(-3.87033643487851,-1.,-0.424304173195111));
#64416=CARTESIAN_POINT('Ctrl Pts',(-3.87033643487851,1.,-0.424304173195111));
#64417=CARTESIAN_POINT('Ctrl Pts',(-3.86339652542709,-1.,-0.421607423177534));
#64418=CARTESIAN_POINT('Ctrl Pts',(-3.86339652542709,1.,-0.421607423177534));
#64419=CARTESIAN_POINT('Ctrl Pts',(-3.85639825647996,-1.,-0.418962468086773));
#64420=CARTESIAN_POINT('Ctrl Pts',(-3.85639825647996,1.,-0.418962468086773));
#64421=CARTESIAN_POINT('Ctrl Pts',(-3.84932864157497,-1.,-0.416369678052907));
#64422=CARTESIAN_POINT('Ctrl Pts',(-3.84932864157497,1.,-0.416369678052907));
#64423=CARTESIAN_POINT('Ctrl Pts',(-3.84219403994762,-1.,-0.413831367016748));
#64424=CARTESIAN_POINT('Ctrl Pts',(-3.84219403994762,1.,-0.413831367016748));
#64425=CARTESIAN_POINT('Ctrl Pts',(-3.83503345578698,-1.,-0.411353038798518));
#64426=CARTESIAN_POINT('Ctrl Pts',(-3.83503345578698,1.,-0.411353038798518));
#64427=CARTESIAN_POINT('Ctrl Pts',(-3.82790724256471,-1.,-0.40894237144746));
#64428=CARTESIAN_POINT('Ctrl Pts',(-3.82790724256471,1.,-0.40894237144746));
#64429=CARTESIAN_POINT('Ctrl Pts',(-3.8208730391381,-1.,-0.406607038258985));
#64430=CARTESIAN_POINT('Ctrl Pts',(-3.8208730391381,1.,-0.406607038258985));
#64431=CARTESIAN_POINT('Ctrl Pts',(-3.81396374287793,-1.,-0.404352694628273));
#64432=CARTESIAN_POINT('Ctrl Pts',(-3.81396374287793,1.,-0.404352694628273));
#64433=CARTESIAN_POINT('Ctrl Pts',(-3.80716881962728,-1.,-0.402181320148436));
#64434=CARTESIAN_POINT('Ctrl Pts',(-3.80716881962728,1.,-0.402181320148436));
#64435=CARTESIAN_POINT('Ctrl Pts',(-3.80040370384546,-1.,-0.4000883465046));
#64436=CARTESIAN_POINT('Ctrl Pts',(-3.80040370384546,1.,-0.4000883465046));
#64437=CARTESIAN_POINT('Ctrl Pts',(-3.7935288716329,-1.,-0.398064818683969));
#64438=CARTESIAN_POINT('Ctrl Pts',(-3.7935288716329,1.,-0.398064818683969));
#64439=CARTESIAN_POINT('Ctrl Pts',(-3.78640521279313,-1.,-0.396103205334841));
#64440=CARTESIAN_POINT('Ctrl Pts',(-3.78640521279313,1.,-0.396103205334841));
#64441=CARTESIAN_POINT('Ctrl Pts',(-3.77894173114283,-1.,-0.394202481011499));
#64442=CARTESIAN_POINT('Ctrl Pts',(-3.77894173114283,1.,-0.394202481011499));
#64443=CARTESIAN_POINT('Ctrl Pts',(-3.77114011595967,-1.,-0.392372786223432));
#64444=CARTESIAN_POINT('Ctrl Pts',(-3.77114011595967,1.,-0.392372786223432));
#64445=CARTESIAN_POINT('Ctrl Pts',(-3.76315635033257,-1.,-0.39064207297956));
#64446=CARTESIAN_POINT('Ctrl Pts',(-3.76315635033257,1.,-0.39064207297956));
#64447=CARTESIAN_POINT('Ctrl Pts',(-3.75529302895152,-1.,-0.389054775898702));
#64448=CARTESIAN_POINT('Ctrl Pts',(-3.75529302895152,1.,-0.389054775898702));
#64449=CARTESIAN_POINT('Ctrl Pts',(-3.74792651696654,-1.,-0.387663020050836));
#64450=CARTESIAN_POINT('Ctrl Pts',(-3.74792651696654,1.,-0.387663020050836));
#64451=CARTESIAN_POINT('Ctrl Pts',(-3.74144965781276,-1.,-0.386519576222251));
#64452=CARTESIAN_POINT('Ctrl Pts',(-3.74144965781276,1.,-0.386519576222251));
#64453=CARTESIAN_POINT('Ctrl Pts',(-3.73621371845318,-1.,-0.385670806454566));
#64454=CARTESIAN_POINT('Ctrl Pts',(-3.73621371845318,1.,-0.385670806454566));
#64455=CARTESIAN_POINT('Ctrl Pts',(-3.73245705638843,-1.,-0.385147887988951));
#64456=CARTESIAN_POINT('Ctrl Pts',(-3.73245705638843,1.,-0.385147887988951));
#64457=CARTESIAN_POINT('Ctrl Pts',(-3.73072465900175,-1.,-0.385001870183213));
#64458=CARTESIAN_POINT('Ctrl Pts',(-3.73072465900175,1.,-0.385001870183213));
#64459=CARTESIAN_POINT('Ctrl Pts',(-3.73015851028356,-1.,-0.385047711603462));
#64460=CARTESIAN_POINT('Ctrl Pts',(-3.73015851028356,1.,-0.385047711603462));
#64461=CARTESIAN_POINT('Ctrl Pts',(-3.73010668803042,-1.,-0.385147278814642));
#64462=CARTESIAN_POINT('Ctrl Pts',(-3.73010668803042,1.,-0.385147278814642));
#64463=CARTESIAN_POINT('Ctrl Pts',(-3.73016218570874,-1.,-0.38521431477633));
#64464=CARTESIAN_POINT('Ctrl Pts',(-3.73016218570874,1.,-0.38521431477633));
#64465=CARTESIAN_POINT('',(-4.15950947128175,1.,-0.581791163835815));
#64466=CARTESIAN_POINT('Ctrl Pts',(-4.15950947128175,1.,-0.581791163835815));
#64467=CARTESIAN_POINT('Ctrl Pts',(-4.1582129171283,1.,-0.580901211463535));
#64468=CARTESIAN_POINT('Ctrl Pts',(-4.15561864788576,1.,-0.579124568914235));
#64469=CARTESIAN_POINT('Ctrl Pts',(-4.151723761217,1.,-0.576469391676688));
#64470=CARTESIAN_POINT('Ctrl Pts',(-4.14652361068081,1.,-0.572948736069522));
#64471=CARTESIAN_POINT('Ctrl Pts',(-4.14001179830547,1.,-0.568580610189774));
#64472=CARTESIAN_POINT('Ctrl Pts',(-4.13348835727104,1.,-0.564245279537148));
#64473=CARTESIAN_POINT('Ctrl Pts',(-4.12695329951961,1.,-0.559942890594773));
#64474=CARTESIAN_POINT('Ctrl Pts',(-4.12040666195664,1.,-0.555673636129977));
#64475=CARTESIAN_POINT('Ctrl Pts',(-4.11384852024721,1.,-0.551437758497032));
#64476=CARTESIAN_POINT('Ctrl Pts',(-4.10727897027977,1.,-0.547235539485637));
#64477=CARTESIAN_POINT('Ctrl Pts',(-4.10069810243979,1.,-0.543067286877757));
#64478=CARTESIAN_POINT('Ctrl Pts',(-4.09410597627,1.,-0.538933321179756));
#64479=CARTESIAN_POINT('Ctrl Pts',(-4.08750259988885,1.,-0.534833963477273));
#64480=CARTESIAN_POINT('Ctrl Pts',(-4.08088789536836,1.,-0.530769518728571));
#64481=CARTESIAN_POINT('Ctrl Pts',(-4.07426172299847,1.,-0.526740277227498));
#64482=CARTESIAN_POINT('Ctrl Pts',(-4.06762394471314,1.,-0.522746528603107));
#64483=CARTESIAN_POINT('Ctrl Pts',(-4.06097448038013,1.,-0.518788572336923));
#64484=CARTESIAN_POINT('Ctrl Pts',(-4.05431335771199,1.,-0.514866728193017));
#64485=CARTESIAN_POINT('Ctrl Pts',(-4.04764078815447,1.,-0.51098134921897));
#64486=CARTESIAN_POINT('Ctrl Pts',(-4.04095715148915,1.,-0.507132823288136));
#64487=CARTESIAN_POINT('Ctrl Pts',(-4.03426284174272,1.,-0.503321556915346));
#64488=CARTESIAN_POINT('Ctrl Pts',(-4.02755813980101,1.,-0.499547962340821));
#64489=CARTESIAN_POINT('Ctrl Pts',(-4.02084308851832,1.,-0.495812444326251));
#64490=CARTESIAN_POINT('Ctrl Pts',(-4.01411733503546,1.,-0.492115383418018));
#64491=CARTESIAN_POINT('Ctrl Pts',(-4.0073800839099,1.,-0.488457130424633));
#64492=CARTESIAN_POINT('Ctrl Pts',(-4.00063045119288,1.,-0.484838042421835));
#64493=CARTESIAN_POINT('Ctrl Pts',(-3.99386775880679,1.,-0.481258512209675));
#64494=CARTESIAN_POINT('Ctrl Pts',(-3.98709184306738,1.,-0.477718999122027));
#64495=CARTESIAN_POINT('Ctrl Pts',(-3.98030338044409,1.,-0.47422006101951));
#64496=CARTESIAN_POINT('Ctrl Pts',(-3.97350414289392,1.,-0.470762379613439));
#64497=CARTESIAN_POINT('Ctrl Pts',(-3.9666962227393,1.,-0.467346690880643));
#64498=CARTESIAN_POINT('Ctrl Pts',(-3.95988133243538,1.,-0.463973722115733));
#64499=CARTESIAN_POINT('Ctrl Pts',(-3.95306005817364,1.,-0.460644124429121));
#64500=CARTESIAN_POINT('Ctrl Pts',(-3.94623117206678,1.,-0.457358410451683));
#64501=CARTESIAN_POINT('Ctrl Pts',(-3.93939080846298,1.,-0.454116879027584));
#64502=CARTESIAN_POINT('Ctrl Pts',(-3.93253407403123,1.,-0.450919768356348));
#64503=CARTESIAN_POINT('Ctrl Pts',(-3.92565674143416,1.,-0.447767416837292));
#64504=CARTESIAN_POINT('Ctrl Pts',(-3.91875701610719,1.,-0.444660430230591));
#64505=CARTESIAN_POINT('Ctrl Pts',(-3.91183704069153,1.,-0.441599824524054));
#64506=CARTESIAN_POINT('Ctrl Pts',(-3.90490512938563,1.,-0.438587235458249));
#64507=CARTESIAN_POINT('Ctrl Pts',(-3.89797256655462,1.,-0.435624629433527));
#64508=CARTESIAN_POINT('Ctrl Pts',(-3.89104947940611,1.,-0.432713929544458));
#64509=CARTESIAN_POINT('Ctrl Pts',(-3.88414070943341,1.,-0.429856640579741));
#64510=CARTESIAN_POINT('Ctrl Pts',(-3.87724240306597,1.,-0.427053541173457));
#64511=CARTESIAN_POINT('Ctrl Pts',(-3.87033643487851,1.,-0.424304173195111));
#64512=CARTESIAN_POINT('Ctrl Pts',(-3.86339652542709,1.,-0.421607423177534));
#64513=CARTESIAN_POINT('Ctrl Pts',(-3.85639825647996,1.,-0.418962468086773));
#64514=CARTESIAN_POINT('Ctrl Pts',(-3.84932864157497,1.,-0.416369678052907));
#64515=CARTESIAN_POINT('Ctrl Pts',(-3.84219403994762,1.,-0.413831367016748));
#64516=CARTESIAN_POINT('Ctrl Pts',(-3.83503345578698,1.,-0.411353038798518));
#64517=CARTESIAN_POINT('Ctrl Pts',(-3.82790724256471,1.,-0.40894237144746));
#64518=CARTESIAN_POINT('Ctrl Pts',(-3.8208730391381,1.,-0.406607038258985));
#64519=CARTESIAN_POINT('Ctrl Pts',(-3.81396374287793,1.,-0.404352694628273));
#64520=CARTESIAN_POINT('Ctrl Pts',(-3.80716881962728,1.,-0.402181320148436));
#64521=CARTESIAN_POINT('Ctrl Pts',(-3.80040370384546,1.,-0.4000883465046));
#64522=CARTESIAN_POINT('Ctrl Pts',(-3.7935288716329,1.,-0.398064818683969));
#64523=CARTESIAN_POINT('Ctrl Pts',(-3.78640521279313,1.,-0.396103205334841));
#64524=CARTESIAN_POINT('Ctrl Pts',(-3.77894173114283,1.,-0.394202481011499));
#64525=CARTESIAN_POINT('Ctrl Pts',(-3.77114011595967,1.,-0.392372786223432));
#64526=CARTESIAN_POINT('Ctrl Pts',(-3.76315635033257,1.,-0.39064207297956));
#64527=CARTESIAN_POINT('Ctrl Pts',(-3.75529302895152,1.,-0.389054775898702));
#64528=CARTESIAN_POINT('Ctrl Pts',(-3.74792651696654,1.,-0.387663020050836));
#64529=CARTESIAN_POINT('Ctrl Pts',(-3.74144965781276,1.,-0.386519576222251));
#64530=CARTESIAN_POINT('Ctrl Pts',(-3.73621371845318,1.,-0.385670806454566));
#64531=CARTESIAN_POINT('Ctrl Pts',(-3.73273893363406,1.,-0.385187124634206));
#64532=CARTESIAN_POINT('Ctrl Pts',(-3.73106082862548,1.,-0.385031656499164));
#64533=CARTESIAN_POINT('Ctrl Pts',(-3.73040527621055,1.,-0.385037797881504));
#64534=CARTESIAN_POINT('Ctrl Pts',(-3.73021431755274,1.,-0.385087139000374));
#64535=CARTESIAN_POINT('Ctrl Pts',(-3.73017266276651,1.,-0.385112848330762));
#64536=CARTESIAN_POINT('',(-4.15950947128175,0.,-0.581791163835815));
#64537=CARTESIAN_POINT('Ctrl Pts',(-3.66663282329846,-1.,-0.7863229229206));
#64538=CARTESIAN_POINT('Ctrl Pts',(-3.66663282329846,1.,-0.7863229229206));
#64539=CARTESIAN_POINT('Ctrl Pts',(-3.66655932661986,-1.,-0.786369528183326));
#64540=CARTESIAN_POINT('Ctrl Pts',(-3.66655932661986,1.,-0.786369528183326));
#64541=CARTESIAN_POINT('Ctrl Pts',(-3.66657784455334,-1.,-0.786480236185696));
#64542=CARTESIAN_POINT('Ctrl Pts',(-3.66657784455334,1.,-0.786480236185696));
#64543=CARTESIAN_POINT('Ctrl Pts',(-3.66710211820482,-1.,-0.786698783542764));
#64544=CARTESIAN_POINT('Ctrl Pts',(-3.66710211820482,1.,-0.786698783542764));
#64545=CARTESIAN_POINT('Ctrl Pts',(-3.66879484801113,-1.,-0.787095252590501));
#64546=CARTESIAN_POINT('Ctrl Pts',(-3.66879484801113,1.,-0.787095252590501));
#64547=CARTESIAN_POINT('Ctrl Pts',(-3.67252923663655,-1.,-0.787758799995742));
#64548=CARTESIAN_POINT('Ctrl Pts',(-3.67252923663655,1.,-0.787758799995742));
#64549=CARTESIAN_POINT('Ctrl Pts',(-3.67777119516252,-1.,-0.788569566220285));
#64550=CARTESIAN_POINT('Ctrl Pts',(-3.67777119516252,1.,-0.788569566220285));
#64551=CARTESIAN_POINT('Ctrl Pts',(-3.68428439783905,-1.,-0.789483546064387));
#64552=CARTESIAN_POINT('Ctrl Pts',(-3.68428439783905,1.,-0.789483546064387));
#64553=CARTESIAN_POINT('Ctrl Pts',(-3.69172044327364,-1.,-0.790436284988787));
#64554=CARTESIAN_POINT('Ctrl Pts',(-3.69172044327364,1.,-0.790436284988787));
#64555=CARTESIAN_POINT('Ctrl Pts',(-3.69968940808721,-1.,-0.79135657569598));
#64556=CARTESIAN_POINT('Ctrl Pts',(-3.69968940808721,1.,-0.79135657569598));
#64557=CARTESIAN_POINT('Ctrl Pts',(-3.70781724021806,-1.,-0.792177688845818));
#64558=CARTESIAN_POINT('Ctrl Pts',(-3.70781724021806,1.,-0.792177688845818));
#64559=CARTESIAN_POINT('Ctrl Pts',(-3.71580242396124,-1.,-0.792848377370287));
#64560=CARTESIAN_POINT('Ctrl Pts',(-3.71580242396124,1.,-0.792848377370287));
#64561=CARTESIAN_POINT('Ctrl Pts',(-3.72348797293734,-1.,-0.793347023784205));
#64562=CARTESIAN_POINT('Ctrl Pts',(-3.72348797293734,1.,-0.793347023784205));
#64563=CARTESIAN_POINT('Ctrl Pts',(-3.73086914695805,-1.,-0.793682750269684));
#64564=CARTESIAN_POINT('Ctrl Pts',(-3.73086914695805,1.,-0.793682750269684));
#64565=CARTESIAN_POINT('Ctrl Pts',(-3.73803280541687,-1.,-0.793882700937017));
#64566=CARTESIAN_POINT('Ctrl Pts',(-3.73803280541687,1.,-0.793882700937017));
#64567=CARTESIAN_POINT('Ctrl Pts',(-3.74511357728861,-1.,-0.793982700459952));
#64568=CARTESIAN_POINT('Ctrl Pts',(-3.74511357728861,1.,-0.793982700459952));
#64569=CARTESIAN_POINT('Ctrl Pts',(-3.75224692493864,-1.,-0.794017347371377));
#64570=CARTESIAN_POINT('Ctrl Pts',(-3.75224692493864,1.,-0.794017347371377));
#64571=CARTESIAN_POINT('Ctrl Pts',(-3.75951468666257,-1.,-0.794008429134907));
#64572=CARTESIAN_POINT('Ctrl Pts',(-3.75951468666257,1.,-0.794008429134907));
#64573=CARTESIAN_POINT('Ctrl Pts',(-3.76692626931111,-1.,-0.793961083688991));
#64574=CARTESIAN_POINT('Ctrl Pts',(-3.76692626931111,1.,-0.793961083688991));
#64575=CARTESIAN_POINT('Ctrl Pts',(-3.77444863801212,-1.,-0.793870523787408));
#64576=CARTESIAN_POINT('Ctrl Pts',(-3.77444863801212,1.,-0.793870523787408));
#64577=CARTESIAN_POINT('Ctrl Pts',(-3.78202460377598,-1.,-0.7937262357813));
#64578=CARTESIAN_POINT('Ctrl Pts',(-3.78202460377598,1.,-0.7937262357813));
#64579=CARTESIAN_POINT('Ctrl Pts',(-3.78959439439235,-1.,-0.793516871680993));
#64580=CARTESIAN_POINT('Ctrl Pts',(-3.78959439439235,1.,-0.793516871680993));
#64581=CARTESIAN_POINT('Ctrl Pts',(-3.79711921389897,-1.,-0.793235612973273));
#64582=CARTESIAN_POINT('Ctrl Pts',(-3.79711921389897,1.,-0.793235612973273));
#64583=CARTESIAN_POINT('Ctrl Pts',(-3.80459229925637,-1.,-0.792882695234778));
#64584=CARTESIAN_POINT('Ctrl Pts',(-3.80459229925637,1.,-0.792882695234778));
#64585=CARTESIAN_POINT('Ctrl Pts',(-3.81202588694756,-1.,-0.792462483517634));
#64586=CARTESIAN_POINT('Ctrl Pts',(-3.81202588694756,1.,-0.792462483517634));
#64587=CARTESIAN_POINT('Ctrl Pts',(-3.81944345442249,-1.,-0.791981740718635));
#64588=CARTESIAN_POINT('Ctrl Pts',(-3.81944345442249,1.,-0.791981740718635));
#64589=CARTESIAN_POINT('Ctrl Pts',(-3.82687033899792,-1.,-0.791447528662369));
#64590=CARTESIAN_POINT('Ctrl Pts',(-3.82687033899792,1.,-0.791447528662369));
#64591=CARTESIAN_POINT('Ctrl Pts',(-3.83432392054786,-1.,-0.790865012705301));
#64592=CARTESIAN_POINT('Ctrl Pts',(-3.83432392054786,1.,-0.790865012705301));
#64593=CARTESIAN_POINT('Ctrl Pts',(-3.84180762342454,-1.,-0.790236124191242));
#64594=CARTESIAN_POINT('Ctrl Pts',(-3.84180762342454,1.,-0.790236124191242));
#64595=CARTESIAN_POINT('Ctrl Pts',(-3.84931637808894,-1.,-0.789560798155582));
#64596=CARTESIAN_POINT('Ctrl Pts',(-3.84931637808894,1.,-0.789560798155582));
#64597=CARTESIAN_POINT('Ctrl Pts',(-3.85683995872529,-1.,-0.788837734090672));
#64598=CARTESIAN_POINT('Ctrl Pts',(-3.85683995872529,1.,-0.788837734090672));
#64599=CARTESIAN_POINT('Ctrl Pts',(-3.86436702561345,-1.,-0.788065315093777));
#64600=CARTESIAN_POINT('Ctrl Pts',(-3.86436702561345,1.,-0.788065315093777));
#64601=CARTESIAN_POINT('Ctrl Pts',(-3.87188916600912,-1.,-0.787242527617999));
#64602=CARTESIAN_POINT('Ctrl Pts',(-3.87188916600912,1.,-0.787242527617999));
#64603=CARTESIAN_POINT('Ctrl Pts',(-3.8794040281819,-1.,-0.786369675812608));
#64604=CARTESIAN_POINT('Ctrl Pts',(-3.8794040281819,1.,-0.786369675812608));
#64605=CARTESIAN_POINT('Ctrl Pts',(-3.88691313167398,-1.,-0.78544789034073));
#64606=CARTESIAN_POINT('Ctrl Pts',(-3.88691313167398,1.,-0.78544789034073));
#64607=CARTESIAN_POINT('Ctrl Pts',(-3.89442039235103,-1.,-0.784478799358336));
#64608=CARTESIAN_POINT('Ctrl Pts',(-3.89442039235103,1.,-0.784478799358336));
#64609=CARTESIAN_POINT('Ctrl Pts',(-3.9019303904397,-1.,-0.783464141529081));
#64610=CARTESIAN_POINT('Ctrl Pts',(-3.9019303904397,1.,-0.783464141529081));
#64611=CARTESIAN_POINT('Ctrl Pts',(-3.90944671004542,-1.,-0.782405395622764));
#64612=CARTESIAN_POINT('Ctrl Pts',(-3.90944671004542,1.,-0.782405395622764));
#64613=CARTESIAN_POINT('Ctrl Pts',(-3.91697036054676,-1.,-0.781303428618366));
#64614=CARTESIAN_POINT('Ctrl Pts',(-3.91697036054676,1.,-0.781303428618366));
#64615=CARTESIAN_POINT('Ctrl Pts',(-3.92450058323823,-1.,-0.780158678615542));
#64616=CARTESIAN_POINT('Ctrl Pts',(-3.92450058323823,1.,-0.780158678615542));
#64617=CARTESIAN_POINT('Ctrl Pts',(-3.93203552473174,-1.,-0.778971308134821));
#64618=CARTESIAN_POINT('Ctrl Pts',(-3.93203552473174,1.,-0.778971308134821));
#64619=CARTESIAN_POINT('Ctrl Pts',(-3.93957296768103,-1.,-0.777741370568558));
#64620=CARTESIAN_POINT('Ctrl Pts',(-3.93957296768103,1.,-0.777741370568558));
#64621=CARTESIAN_POINT('Ctrl Pts',(-3.94711101619447,-1.,-0.776468966697921));
#64622=CARTESIAN_POINT('Ctrl Pts',(-3.94711101619447,1.,-0.776468966697921));
#64623=CARTESIAN_POINT('Ctrl Pts',(-3.9546488545231,-1.,-0.775154418039351));
#64624=CARTESIAN_POINT('Ctrl Pts',(-3.9546488545231,1.,-0.775154418039351));
#64625=CARTESIAN_POINT('Ctrl Pts',(-3.96218649639807,-1.,-0.773798212026565));
#64626=CARTESIAN_POINT('Ctrl Pts',(-3.96218649639807,1.,-0.773798212026565));
#64627=CARTESIAN_POINT('Ctrl Pts',(-3.96972446532772,-1.,-0.772400931772136));
#64628=CARTESIAN_POINT('Ctrl Pts',(-3.96972446532772,1.,-0.772400931772136));
#64629=CARTESIAN_POINT('Ctrl Pts',(-3.97726349165488,-1.,-0.770963190030471));
#64630=CARTESIAN_POINT('Ctrl Pts',(-3.97726349165488,1.,-0.770963190030471));
#64631=CARTESIAN_POINT('Ctrl Pts',(-3.98480422348451,-1.,-0.769485566245544));
#64632=CARTESIAN_POINT('Ctrl Pts',(-3.98480422348451,1.,-0.769485566245544));
#64633=CARTESIAN_POINT('Ctrl Pts',(-3.9923468788101,-1.,-0.767968531377915));
#64634=CARTESIAN_POINT('Ctrl Pts',(-3.9923468788101,1.,-0.767968531377915));
#64635=CARTESIAN_POINT('Ctrl Pts',(-3.99989129179622,-1.,-0.766412457136064));
#64636=CARTESIAN_POINT('Ctrl Pts',(-3.99989129179622,1.,-0.766412457136064));
#64637=CARTESIAN_POINT('Ctrl Pts',(-4.00743706791509,-1.,-0.764817648785197));
#64638=CARTESIAN_POINT('Ctrl Pts',(-4.00743706791509,1.,-0.764817648785197));
#64639=CARTESIAN_POINT('Ctrl Pts',(-4.01498370680496,-1.,-0.763184371182935));
#64640=CARTESIAN_POINT('Ctrl Pts',(-4.01498370680496,1.,-0.763184371182935));
#64641=CARTESIAN_POINT('Ctrl Pts',(-4.02253072741268,-1.,-0.761512875859804));
#64642=CARTESIAN_POINT('Ctrl Pts',(-4.02253072741268,1.,-0.761512875859804));
#64643=CARTESIAN_POINT('Ctrl Pts',(-4.03007781954412,-1.,-0.759803433243752));
#64644=CARTESIAN_POINT('Ctrl Pts',(-4.03007781954412,1.,-0.759803433243752));
#64645=CARTESIAN_POINT('Ctrl Pts',(-4.03762485803119,-1.,-0.758056338884944));
#64646=CARTESIAN_POINT('Ctrl Pts',(-4.03762485803119,1.,-0.758056338884944));
#64647=CARTESIAN_POINT('Ctrl Pts',(-4.04517182653997,-1.,-0.756271902369581));
#64648=CARTESIAN_POINT('Ctrl Pts',(-4.04517182653997,1.,-0.756271902369581));
#64649=CARTESIAN_POINT('Ctrl Pts',(-4.05271876687915,-1.,-0.754450441816078));
#64650=CARTESIAN_POINT('Ctrl Pts',(-4.05271876687915,1.,-0.754450441816078));
#64651=CARTESIAN_POINT('Ctrl Pts',(-4.06026572221515,-1.,-0.752592276483072));
#64652=CARTESIAN_POINT('Ctrl Pts',(-4.06026572221515,1.,-0.752592276483072));
#64653=CARTESIAN_POINT('Ctrl Pts',(-4.06781267242378,-1.,-0.750697720484036));
#64654=CARTESIAN_POINT('Ctrl Pts',(-4.06781267242378,1.,-0.750697720484036));
#64655=CARTESIAN_POINT('Ctrl Pts',(-4.07535951056152,-1.,-0.748767076680557));
#64656=CARTESIAN_POINT('Ctrl Pts',(-4.07535951056152,1.,-0.748767076680557));
#64657=CARTESIAN_POINT('Ctrl Pts',(-4.08290608095642,-1.,-0.746800631492315));
#64658=CARTESIAN_POINT('Ctrl Pts',(-4.08290608095642,1.,-0.746800631492315));
#64659=CARTESIAN_POINT('Ctrl Pts',(-4.09045220253573,-1.,-0.7447986497065));
#64660=CARTESIAN_POINT('Ctrl Pts',(-4.09045220253573,1.,-0.7447986497065));
#64661=CARTESIAN_POINT('Ctrl Pts',(-4.09799769702611,-1.,-0.742761369689841));
#64662=CARTESIAN_POINT('Ctrl Pts',(-4.09799769702611,1.,-0.742761369689841));
#64663=CARTESIAN_POINT('Ctrl Pts',(-4.10554241757547,-1.,-0.740688998553377));
#64664=CARTESIAN_POINT('Ctrl Pts',(-4.10554241757547,1.,-0.740688998553377));
#64665=CARTESIAN_POINT('Ctrl Pts',(-4.11308626951927,-1.,-0.738581708225844));
#64666=CARTESIAN_POINT('Ctrl Pts',(-4.11308626951927,1.,-0.738581708225844));
#64667=CARTESIAN_POINT('Ctrl Pts',(-4.120629196238,-1.,-0.736439634331345));
#64668=CARTESIAN_POINT('Ctrl Pts',(-4.120629196238,1.,-0.736439634331345));
#64669=CARTESIAN_POINT('Ctrl Pts',(-4.12666277570844,-1.,-0.734698226764092));
#64670=CARTESIAN_POINT('Ctrl Pts',(-4.12666277570844,1.,-0.734698226764092));
#64671=CARTESIAN_POINT('Ctrl Pts',(-4.13118752795207,-1.,-0.733376589323546));
#64672=CARTESIAN_POINT('Ctrl Pts',(-4.13118752795207,1.,-0.733376589323546));
#64673=CARTESIAN_POINT('Ctrl Pts',(-4.1342038373684,-1.,-0.732488575135159));
#64674=CARTESIAN_POINT('Ctrl Pts',(-4.1342038373684,1.,-0.732488575135159));
#64675=CARTESIAN_POINT('Ctrl Pts',(-4.13571194405636,-1.,-0.73204283740062));
#64676=CARTESIAN_POINT('Ctrl Pts',(-4.13571194405636,1.,-0.73204283740062));
#64677=CARTESIAN_POINT('',(-3.66661143271685,1.,-0.786422660831985));
#64678=CARTESIAN_POINT('Ctrl Pts',(-3.66661143271685,-1.,-0.786422660831985));
#64679=CARTESIAN_POINT('Ctrl Pts',(-3.66661143271685,-0.666666666666667,
-0.786422660831985));
#64680=CARTESIAN_POINT('Ctrl Pts',(-3.66661143271685,-0.333333333333333,
-0.786422660831985));
#64681=CARTESIAN_POINT('Ctrl Pts',(-3.66661143271685,0.333333333333333,
-0.786422660831985));
#64682=CARTESIAN_POINT('Ctrl Pts',(-3.66661143271685,0.666666666666667,
-0.786422660831985));
#64683=CARTESIAN_POINT('Ctrl Pts',(-3.66661143271685,1.,-0.786422660831985));
#64684=CARTESIAN_POINT('',(-4.13571194405636,1.,-0.73204283740062));
#64685=CARTESIAN_POINT('',(-4.13571194405636,0.,-0.73204283740062));
#64686=CARTESIAN_POINT('Ctrl Pts',(-3.66661143271685,1.,-0.786422660831985));
#64687=CARTESIAN_POINT('Ctrl Pts',(-3.6666431041522,1.,-0.786459983895432));
#64688=CARTESIAN_POINT('Ctrl Pts',(-3.66680946938292,1.,-0.786565919558984));
#64689=CARTESIAN_POINT('Ctrl Pts',(-3.66743103898702,1.,-0.786774337198062));
#64690=CARTESIAN_POINT('Ctrl Pts',(-3.66907505398677,1.,-0.787145041181545));
#64691=CARTESIAN_POINT('Ctrl Pts',(-3.67252923663655,1.,-0.787758799995742));
#64692=CARTESIAN_POINT('Ctrl Pts',(-3.67777119516252,1.,-0.788569566220285));
#64693=CARTESIAN_POINT('Ctrl Pts',(-3.68428439783905,1.,-0.789483546064387));
#64694=CARTESIAN_POINT('Ctrl Pts',(-3.69172044327364,1.,-0.790436284988787));
#64695=CARTESIAN_POINT('Ctrl Pts',(-3.69968940808721,1.,-0.79135657569598));
#64696=CARTESIAN_POINT('Ctrl Pts',(-3.70781724021806,1.,-0.792177688845818));
#64697=CARTESIAN_POINT('Ctrl Pts',(-3.71580242396124,1.,-0.792848377370287));
#64698=CARTESIAN_POINT('Ctrl Pts',(-3.72348797293734,1.,-0.793347023784205));
#64699=CARTESIAN_POINT('Ctrl Pts',(-3.73086914695805,1.,-0.793682750269684));
#64700=CARTESIAN_POINT('Ctrl Pts',(-3.73803280541687,1.,-0.793882700937017));
#64701=CARTESIAN_POINT('Ctrl Pts',(-3.74511357728861,1.,-0.793982700459952));
#64702=CARTESIAN_POINT('Ctrl Pts',(-3.75224692493864,1.,-0.794017347371377));
#64703=CARTESIAN_POINT('Ctrl Pts',(-3.75951468666257,1.,-0.794008429134907));
#64704=CARTESIAN_POINT('Ctrl Pts',(-3.76692626931111,1.,-0.793961083688991));
#64705=CARTESIAN_POINT('Ctrl Pts',(-3.77444863801212,1.,-0.793870523787408));
#64706=CARTESIAN_POINT('Ctrl Pts',(-3.78202460377598,1.,-0.7937262357813));
#64707=CARTESIAN_POINT('Ctrl Pts',(-3.78959439439235,1.,-0.793516871680993));
#64708=CARTESIAN_POINT('Ctrl Pts',(-3.79711921389897,1.,-0.793235612973273));
#64709=CARTESIAN_POINT('Ctrl Pts',(-3.80459229925637,1.,-0.792882695234778));
#64710=CARTESIAN_POINT('Ctrl Pts',(-3.81202588694756,1.,-0.792462483517634));
#64711=CARTESIAN_POINT('Ctrl Pts',(-3.81944345442249,1.,-0.791981740718635));
#64712=CARTESIAN_POINT('Ctrl Pts',(-3.82687033899792,1.,-0.791447528662369));
#64713=CARTESIAN_POINT('Ctrl Pts',(-3.83432392054786,1.,-0.790865012705301));
#64714=CARTESIAN_POINT('Ctrl Pts',(-3.84180762342454,1.,-0.790236124191242));
#64715=CARTESIAN_POINT('Ctrl Pts',(-3.84931637808894,1.,-0.789560798155582));
#64716=CARTESIAN_POINT('Ctrl Pts',(-3.85683995872529,1.,-0.788837734090672));
#64717=CARTESIAN_POINT('Ctrl Pts',(-3.86436702561345,1.,-0.788065315093777));
#64718=CARTESIAN_POINT('Ctrl Pts',(-3.87188916600912,1.,-0.787242527617999));
#64719=CARTESIAN_POINT('Ctrl Pts',(-3.8794040281819,1.,-0.786369675812608));
#64720=CARTESIAN_POINT('Ctrl Pts',(-3.88691313167398,1.,-0.78544789034073));
#64721=CARTESIAN_POINT('Ctrl Pts',(-3.89442039235103,1.,-0.784478799358336));
#64722=CARTESIAN_POINT('Ctrl Pts',(-3.9019303904397,1.,-0.783464141529081));
#64723=CARTESIAN_POINT('Ctrl Pts',(-3.90944671004542,1.,-0.782405395622764));
#64724=CARTESIAN_POINT('Ctrl Pts',(-3.91697036054676,1.,-0.781303428618366));
#64725=CARTESIAN_POINT('Ctrl Pts',(-3.92450058323823,1.,-0.780158678615542));
#64726=CARTESIAN_POINT('Ctrl Pts',(-3.93203552473174,1.,-0.778971308134821));
#64727=CARTESIAN_POINT('Ctrl Pts',(-3.93957296768103,1.,-0.777741370568558));
#64728=CARTESIAN_POINT('Ctrl Pts',(-3.94711101619447,1.,-0.776468966697921));
#64729=CARTESIAN_POINT('Ctrl Pts',(-3.9546488545231,1.,-0.775154418039351));
#64730=CARTESIAN_POINT('Ctrl Pts',(-3.96218649639807,1.,-0.773798212026565));
#64731=CARTESIAN_POINT('Ctrl Pts',(-3.96972446532772,1.,-0.772400931772136));
#64732=CARTESIAN_POINT('Ctrl Pts',(-3.97726349165488,1.,-0.770963190030471));
#64733=CARTESIAN_POINT('Ctrl Pts',(-3.98480422348451,1.,-0.769485566245544));
#64734=CARTESIAN_POINT('Ctrl Pts',(-3.9923468788101,1.,-0.767968531377915));
#64735=CARTESIAN_POINT('Ctrl Pts',(-3.99989129179622,1.,-0.766412457136064));
#64736=CARTESIAN_POINT('Ctrl Pts',(-4.00743706791509,1.,-0.764817648785197));
#64737=CARTESIAN_POINT('Ctrl Pts',(-4.01498370680496,1.,-0.763184371182935));
#64738=CARTESIAN_POINT('Ctrl Pts',(-4.02253072741268,1.,-0.761512875859804));
#64739=CARTESIAN_POINT('Ctrl Pts',(-4.03007781954412,1.,-0.759803433243752));
#64740=CARTESIAN_POINT('Ctrl Pts',(-4.03762485803119,1.,-0.758056338884944));
#64741=CARTESIAN_POINT('Ctrl Pts',(-4.04517182653997,1.,-0.756271902369581));
#64742=CARTESIAN_POINT('Ctrl Pts',(-4.05271876687915,1.,-0.754450441816078));
#64743=CARTESIAN_POINT('Ctrl Pts',(-4.06026572221515,1.,-0.752592276483072));
#64744=CARTESIAN_POINT('Ctrl Pts',(-4.06781267242378,1.,-0.750697720484036));
#64745=CARTESIAN_POINT('Ctrl Pts',(-4.07535951056152,1.,-0.748767076680557));
#64746=CARTESIAN_POINT('Ctrl Pts',(-4.08290608095642,1.,-0.746800631492315));
#64747=CARTESIAN_POINT('Ctrl Pts',(-4.09045220253573,1.,-0.7447986497065));
#64748=CARTESIAN_POINT('Ctrl Pts',(-4.09799769702611,1.,-0.742761369689841));
#64749=CARTESIAN_POINT('Ctrl Pts',(-4.10554241757547,1.,-0.740688998553377));
#64750=CARTESIAN_POINT('Ctrl Pts',(-4.11308626951927,1.,-0.738581708225844));
#64751=CARTESIAN_POINT('Ctrl Pts',(-4.120629196238,1.,-0.736439634331345));
#64752=CARTESIAN_POINT('Ctrl Pts',(-4.12666277570844,1.,-0.734698226764092));
#64753=CARTESIAN_POINT('Ctrl Pts',(-4.13118752795207,1.,-0.733376589323546));
#64754=CARTESIAN_POINT('Ctrl Pts',(-4.1342038373684,1.,-0.732488575135159));
#64755=CARTESIAN_POINT('Ctrl Pts',(-4.13571194405636,1.,-0.73204283740062));
#64756=CARTESIAN_POINT('Origin',(-4.13571194405636,0.,-0.73204283740062));
#64757=CARTESIAN_POINT('',(-4.15950947128175,1.,-0.581791163835815));
#64758=CARTESIAN_POINT('Origin',(0.,0.,0.));
#64759=CARTESIAN_POINT('',(-3.62400312501245,1.,-0.963899035117248));
#64760=CARTESIAN_POINT('Origin',(0.,1.,0.));
#64761=CARTESIAN_POINT('Ctrl Pts',(-3.62400312501245,1.,-0.963899035117249));
#64762=CARTESIAN_POINT('Ctrl Pts',(-3.62400312501245,0.666666666666667,
-0.963899035117249));
#64763=CARTESIAN_POINT('Ctrl Pts',(-3.62400312501245,0.333333333333333,
-0.963899035117249));
#64764=CARTESIAN_POINT('Ctrl Pts',(-3.62400312501245,-0.333333333333333,
-0.963899035117249));
#64765=CARTESIAN_POINT('Ctrl Pts',(-3.62400312501246,-0.666666666666667,
-0.963899035117249));
#64766=CARTESIAN_POINT('Ctrl Pts',(-3.62400312501246,-1.,-0.963899035117249));
#64767=CARTESIAN_POINT('Ctrl Pts',(-4.01728681790024,-1.,-1.22531898815164));
#64768=CARTESIAN_POINT('Ctrl Pts',(-4.01728681790024,1.,-1.22531898815164));
#64769=CARTESIAN_POINT('Ctrl Pts',(-4.0161454457032,-1.,-1.22423716681447));
#64770=CARTESIAN_POINT('Ctrl Pts',(-4.0161454457032,1.,-1.22423716681447));
#64771=CARTESIAN_POINT('Ctrl Pts',(-4.01386104434674,-1.,-1.22207656456199));
#64772=CARTESIAN_POINT('Ctrl Pts',(-4.01386104434674,1.,-1.22207656456199));
#64773=CARTESIAN_POINT('Ctrl Pts',(-4.01042947142681,-1.,-1.21884478244983));
#64774=CARTESIAN_POINT('Ctrl Pts',(-4.01042947142681,1.,-1.21884478244983));
#64775=CARTESIAN_POINT('Ctrl Pts',(-4.00584409524937,-1.,-1.21455398918813));
#64776=CARTESIAN_POINT('Ctrl Pts',(-4.00584409524937,1.,-1.21455398918813));
#64777=CARTESIAN_POINT('Ctrl Pts',(-4.00009577952534,-1.,-1.20922097030107));
#64778=CARTESIAN_POINT('Ctrl Pts',(-4.00009577952534,1.,-1.20922097030107));
#64779=CARTESIAN_POINT('Ctrl Pts',(-3.99433084800649,-1.,-1.2039185237544));
#64780=CARTESIAN_POINT('Ctrl Pts',(-3.99433084800649,1.,-1.2039185237544));
#64781=CARTESIAN_POINT('Ctrl Pts',(-3.98854928957287,-1.,-1.19864679609596));
#64782=CARTESIAN_POINT('Ctrl Pts',(-3.98854928957287,1.,-1.19864679609596));
#64783=CARTESIAN_POINT('Ctrl Pts',(-3.98275111052015,-1.,-1.19340598349307));
#64784=CARTESIAN_POINT('Ctrl Pts',(-3.98275111052015,1.,-1.19340598349307));
#64785=CARTESIAN_POINT('Ctrl Pts',(-3.97693634766926,-1.,-1.18819633715285));
#64786=CARTESIAN_POINT('Ctrl Pts',(-3.97693634766926,1.,-1.18819633715285));
#64787=CARTESIAN_POINT('Ctrl Pts',(-3.9711050516465,-1.,-1.18301815039596));
#64788=CARTESIAN_POINT('Ctrl Pts',(-3.9711050516465,1.,-1.18301815039596));
#64789=CARTESIAN_POINT('Ctrl Pts',(-3.96525726357682,-1.,-1.17787174135445));
#64790=CARTESIAN_POINT('Ctrl Pts',(-3.96525726357682,1.,-1.17787174135445));
#64791=CARTESIAN_POINT('Ctrl Pts',(-3.95939299213164,-1.,-1.17275743590327));
#64792=CARTESIAN_POINT('Ctrl Pts',(-3.95939299213164,1.,-1.17275743590327));
#64793=CARTESIAN_POINT('Ctrl Pts',(-3.95351219510062,-1.,-1.16767555244495));
#64794=CARTESIAN_POINT('Ctrl Pts',(-3.95351219510062,1.,-1.16767555244495));
#64795=CARTESIAN_POINT('Ctrl Pts',(-3.9476147478092,-1.,-1.16262637999261));
#64796=CARTESIAN_POINT('Ctrl Pts',(-3.9476147478092,1.,-1.16262637999261));
#64797=CARTESIAN_POINT('Ctrl Pts',(-3.94170046685542,-1.,-1.1576101834106));
#64798=CARTESIAN_POINT('Ctrl Pts',(-3.94170046685542,1.,-1.1576101834106));
#64799=CARTESIAN_POINT('Ctrl Pts',(-3.9357691705651,-1.,-1.1526272271639));
#64800=CARTESIAN_POINT('Ctrl Pts',(-3.9357691705651,1.,-1.1526272271639));
#64801=CARTESIAN_POINT('Ctrl Pts',(-3.92982073294334,-1.,-1.14767779451147));
#64802=CARTESIAN_POINT('Ctrl Pts',(-3.92982073294334,1.,-1.14767779451147));
#64803=CARTESIAN_POINT('Ctrl Pts',(-3.92385513133937,-1.,-1.14276220561575));
#64804=CARTESIAN_POINT('Ctrl Pts',(-3.92385513133937,1.,-1.14276220561575));
#64805=CARTESIAN_POINT('Ctrl Pts',(-3.91787251936688,-1.,-1.13788084225511));
#64806=CARTESIAN_POINT('Ctrl Pts',(-3.91787251936688,1.,-1.13788084225511));
#64807=CARTESIAN_POINT('Ctrl Pts',(-3.91187321145495,-1.,-1.13303414693849));
#64808=CARTESIAN_POINT('Ctrl Pts',(-3.91187321145495,1.,-1.13303414693849));
#64809=CARTESIAN_POINT('Ctrl Pts',(-3.90585753318622,-1.,-1.12822258281518));
#64810=CARTESIAN_POINT('Ctrl Pts',(-3.90585753318622,1.,-1.12822258281518));
#64811=CARTESIAN_POINT('Ctrl Pts',(-3.89982569749978,-1.,-1.12344660099029));
#64812=CARTESIAN_POINT('Ctrl Pts',(-3.89982569749978,1.,-1.12344660099029));
#64813=CARTESIAN_POINT('Ctrl Pts',(-3.89377768340362,-1.,-1.11870660794609));
#64814=CARTESIAN_POINT('Ctrl Pts',(-3.89377768340362,1.,-1.11870660794609));
#64815=CARTESIAN_POINT('Ctrl Pts',(-3.88771308285229,-1.,-1.11400292434447));
#64816=CARTESIAN_POINT('Ctrl Pts',(-3.88771308285229,1.,-1.11400292434447));
#64817=CARTESIAN_POINT('Ctrl Pts',(-3.88163105531791,-1.,-1.10933577224029));
#64818=CARTESIAN_POINT('Ctrl Pts',(-3.88163105531791,1.,-1.10933577224029));
#64819=CARTESIAN_POINT('Ctrl Pts',(-3.87553067187566,-1.,-1.10470536603303));
#64820=CARTESIAN_POINT('Ctrl Pts',(-3.87553067187566,1.,-1.10470536603303));
#64821=CARTESIAN_POINT('Ctrl Pts',(-3.86941120134872,-1.,-1.10011198761202));
#64822=CARTESIAN_POINT('Ctrl Pts',(-3.86941120134872,1.,-1.10011198761202));
#64823=CARTESIAN_POINT('Ctrl Pts',(-3.86327241021242,-1.,-1.09555606505012));
#64824=CARTESIAN_POINT('Ctrl Pts',(-3.86327241021242,1.,-1.09555606505012));
#64825=CARTESIAN_POINT('Ctrl Pts',(-3.85711487933911,-1.,-1.09103825516288));
#64826=CARTESIAN_POINT('Ctrl Pts',(-3.85711487933911,1.,-1.09103825516288));
#64827=CARTESIAN_POINT('Ctrl Pts',(-3.8509402522269,-1.,-1.08655950846377));
#64828=CARTESIAN_POINT('Ctrl Pts',(-3.8509402522269,1.,-1.08655950846377));
#64829=CARTESIAN_POINT('Ctrl Pts',(-3.84475048030615,-1.,-1.08212087917986));
#64830=CARTESIAN_POINT('Ctrl Pts',(-3.84475048030615,1.,-1.08212087917986));
#64831=CARTESIAN_POINT('Ctrl Pts',(-3.83854714117486,-1.,-1.07772335353856));
#64832=CARTESIAN_POINT('Ctrl Pts',(-3.83854714117486,1.,-1.07772335353856));
#64833=CARTESIAN_POINT('Ctrl Pts',(-3.83233071195145,-1.,-1.0733676663346));
#64834=CARTESIAN_POINT('Ctrl Pts',(-3.83233071195145,1.,-1.0733676663346));
#64835=CARTESIAN_POINT('Ctrl Pts',(-3.82609989967278,-1.,-1.0690541318036));
#64836=CARTESIAN_POINT('Ctrl Pts',(-3.82609989967278,1.,-1.0690541318036));
#64837=CARTESIAN_POINT('Ctrl Pts',(-3.81985083953012,-1.,-1.06478244038931));
#64838=CARTESIAN_POINT('Ctrl Pts',(-3.81985083953012,1.,-1.06478244038931));
#64839=CARTESIAN_POINT('Ctrl Pts',(-3.81357866117485,-1.,-1.06055206187298));
#64840=CARTESIAN_POINT('Ctrl Pts',(-3.81357866117485,1.,-1.06055206187298));
#64841=CARTESIAN_POINT('Ctrl Pts',(-3.80727913637784,-1.,-1.05636266918643));
#64842=CARTESIAN_POINT('Ctrl Pts',(-3.80727913637784,1.,-1.05636266918643));
#64843=CARTESIAN_POINT('Ctrl Pts',(-3.80095039790678,-1.,-1.05221457990015));
#64844=CARTESIAN_POINT('Ctrl Pts',(-3.80095039790678,1.,-1.05221457990015));
#64845=CARTESIAN_POINT('Ctrl Pts',(-3.79459440308793,-1.,-1.04810913267641));
#64846=CARTESIAN_POINT('Ctrl Pts',(-3.79459440308793,1.,-1.04810913267641));
#64847=CARTESIAN_POINT('Ctrl Pts',(-3.78821910787195,-1.,-1.04404924374426));
#64848=CARTESIAN_POINT('Ctrl Pts',(-3.78821910787195,1.,-1.04404924374426));
#64849=CARTESIAN_POINT('Ctrl Pts',(-3.78183535008192,-1.,-1.04003862055804));
#64850=CARTESIAN_POINT('Ctrl Pts',(-3.78183535008192,1.,-1.04003862055804));
#64851=CARTESIAN_POINT('Ctrl Pts',(-3.77545283140445,-1.,-1.03608074678013));
#64852=CARTESIAN_POINT('Ctrl Pts',(-3.77545283140445,1.,-1.03608074678013));
#64853=CARTESIAN_POINT('Ctrl Pts',(-3.76907609832522,-1.,-1.0321778660492));
#64854=CARTESIAN_POINT('Ctrl Pts',(-3.76907609832522,1.,-1.0321778660492));
#64855=CARTESIAN_POINT('Ctrl Pts',(-3.76270122291232,-1.,-1.02833014458181));
#64856=CARTESIAN_POINT('Ctrl Pts',(-3.76270122291232,1.,-1.02833014458181));
#64857=CARTESIAN_POINT('Ctrl Pts',(-3.75631037456194,-1.,-1.0245342944466));
#64858=CARTESIAN_POINT('Ctrl Pts',(-3.75631037456194,1.,-1.0245342944466));
#64859=CARTESIAN_POINT('Ctrl Pts',(-3.74987777155834,-1.,-1.02078510487428));
#64860=CARTESIAN_POINT('Ctrl Pts',(-3.74987777155834,1.,-1.02078510487428));
#64861=CARTESIAN_POINT('Ctrl Pts',(-3.74337942504959,-1.,-1.01707794311079));
#64862=CARTESIAN_POINT('Ctrl Pts',(-3.74337942504959,1.,-1.01707794311079));
#64863=CARTESIAN_POINT('Ctrl Pts',(-3.73680245055734,-1.,-1.01341114319903));
#64864=CARTESIAN_POINT('Ctrl Pts',(-3.73680245055734,1.,-1.01341114319903));
#64865=CARTESIAN_POINT('Ctrl Pts',(-3.73015276704426,-1.,-1.00978798539496));
#64866=CARTESIAN_POINT('Ctrl Pts',(-3.73015276704426,1.,-1.00978798539496));
#64867=CARTESIAN_POINT('Ctrl Pts',(-3.72346803750595,-1.,-1.0062200073571));
#64868=CARTESIAN_POINT('Ctrl Pts',(-3.72346803750595,1.,-1.0062200073571));
#64869=CARTESIAN_POINT('Ctrl Pts',(-3.71680667125118,-1.,-1.00272423396822));
#64870=CARTESIAN_POINT('Ctrl Pts',(-3.71680667125118,1.,-1.00272423396822));
#64871=CARTESIAN_POINT('Ctrl Pts',(-3.71022439713938,-1.,-0.99931726075653));
#64872=CARTESIAN_POINT('Ctrl Pts',(-3.71022439713938,1.,-0.99931726075653));
#64873=CARTESIAN_POINT('Ctrl Pts',(-3.70375282282138,-1.,-0.996009819772518));
#64874=CARTESIAN_POINT('Ctrl Pts',(-3.70375282282138,1.,-0.996009819772518));
#64875=CARTESIAN_POINT('Ctrl Pts',(-3.69738123415662,-1.,-0.99280221833201));
#64876=CARTESIAN_POINT('Ctrl Pts',(-3.69738123415662,1.,-0.99280221833201));
#64877=CARTESIAN_POINT('Ctrl Pts',(-3.69102682138846,-1.,-0.989676715398558));
#64878=CARTESIAN_POINT('Ctrl Pts',(-3.69102682138846,1.,-0.989676715398558));
#64879=CARTESIAN_POINT('Ctrl Pts',(-3.68455317926068,-1.,-0.986602639863837));
#64880=CARTESIAN_POINT('Ctrl Pts',(-3.68455317926068,1.,-0.986602639863837));
#64881=CARTESIAN_POINT('Ctrl Pts',(-3.67782408841715,-1.,-0.983550791470419));
#64882=CARTESIAN_POINT('Ctrl Pts',(-3.67782408841715,1.,-0.983550791470419));
#64883=CARTESIAN_POINT('Ctrl Pts',(-3.67074983340361,-1.,-0.980505922458267));
#64884=CARTESIAN_POINT('Ctrl Pts',(-3.67074983340361,1.,-0.980505922458267));
#64885=CARTESIAN_POINT('Ctrl Pts',(-3.66333049637475,-1.,-0.977478312751618));
#64886=CARTESIAN_POINT('Ctrl Pts',(-3.66333049637475,1.,-0.977478312751618));
#64887=CARTESIAN_POINT('Ctrl Pts',(-3.65571576735126,-1.,-0.974519971354848));
#64888=CARTESIAN_POINT('Ctrl Pts',(-3.65571576735126,1.,-0.974519971354848));
#64889=CARTESIAN_POINT('Ctrl Pts',(-3.64819756447455,-1.,-0.971722122061341));
#64890=CARTESIAN_POINT('Ctrl Pts',(-3.64819756447455,1.,-0.971722122061341));
#64891=CARTESIAN_POINT('Ctrl Pts',(-3.64113946505766,-1.,-0.969195124675865));
#64892=CARTESIAN_POINT('Ctrl Pts',(-3.64113946505766,1.,-0.969195124675865));
#64893=CARTESIAN_POINT('Ctrl Pts',(-3.63492122081143,-1.,-0.967052554541385));
#64894=CARTESIAN_POINT('Ctrl Pts',(-3.63492122081143,1.,-0.967052554541385));
#64895=CARTESIAN_POINT('Ctrl Pts',(-3.62988252139846,-1.,-0.965395153165293));
#64896=CARTESIAN_POINT('Ctrl Pts',(-3.62988252139846,1.,-0.965395153165293));
#64897=CARTESIAN_POINT('Ctrl Pts',(-3.62625391254797,-1.,-0.964291001273287));
#64898=CARTESIAN_POINT('Ctrl Pts',(-3.62625391254797,1.,-0.964291001273287));
#64899=CARTESIAN_POINT('Ctrl Pts',(-3.6245656860652,-1.,-0.963875774530619));
#64900=CARTESIAN_POINT('Ctrl Pts',(-3.6245656860652,1.,-0.963875774530619));
#64901=CARTESIAN_POINT('Ctrl Pts',(-3.62399933639914,-1.,-0.963832486395051));
#64902=CARTESIAN_POINT('Ctrl Pts',(-3.62399933639914,1.,-0.963832486395051));
#64903=CARTESIAN_POINT('Ctrl Pts',(-3.62393257642052,-1.,-0.963922720982193));
#64904=CARTESIAN_POINT('Ctrl Pts',(-3.62393257642052,1.,-0.963922720982193));
#64905=CARTESIAN_POINT('Ctrl Pts',(-3.62397690409552,-1.,-0.963997613369571));
#64906=CARTESIAN_POINT('Ctrl Pts',(-3.62397690409552,1.,-0.963997613369571));
#64907=CARTESIAN_POINT('',(-4.01728681790024,1.,-1.22531898815164));
#64908=CARTESIAN_POINT('Ctrl Pts',(-4.01728681790024,1.,-1.22531898815164));
#64909=CARTESIAN_POINT('Ctrl Pts',(-4.0161454457032,1.,-1.22423716681447));
#64910=CARTESIAN_POINT('Ctrl Pts',(-4.01386104434674,1.,-1.22207656456199));
#64911=CARTESIAN_POINT('Ctrl Pts',(-4.01042947142681,1.,-1.21884478244983));
#64912=CARTESIAN_POINT('Ctrl Pts',(-4.00584409524937,1.,-1.21455398918813));
#64913=CARTESIAN_POINT('Ctrl Pts',(-4.00009577952534,1.,-1.20922097030107));
#64914=CARTESIAN_POINT('Ctrl Pts',(-3.99433084800649,1.,-1.2039185237544));
#64915=CARTESIAN_POINT('Ctrl Pts',(-3.98854928957287,1.,-1.19864679609596));
#64916=CARTESIAN_POINT('Ctrl Pts',(-3.98275111052015,1.,-1.19340598349307));
#64917=CARTESIAN_POINT('Ctrl Pts',(-3.97693634766926,1.,-1.18819633715285));
#64918=CARTESIAN_POINT('Ctrl Pts',(-3.9711050516465,1.,-1.18301815039596));
#64919=CARTESIAN_POINT('Ctrl Pts',(-3.96525726357682,1.,-1.17787174135445));
#64920=CARTESIAN_POINT('Ctrl Pts',(-3.95939299213164,1.,-1.17275743590327));
#64921=CARTESIAN_POINT('Ctrl Pts',(-3.95351219510062,1.,-1.16767555244495));
#64922=CARTESIAN_POINT('Ctrl Pts',(-3.9476147478092,1.,-1.16262637999261));
#64923=CARTESIAN_POINT('Ctrl Pts',(-3.94170046685542,1.,-1.1576101834106));
#64924=CARTESIAN_POINT('Ctrl Pts',(-3.9357691705651,1.,-1.1526272271639));
#64925=CARTESIAN_POINT('Ctrl Pts',(-3.92982073294334,1.,-1.14767779451147));
#64926=CARTESIAN_POINT('Ctrl Pts',(-3.92385513133937,1.,-1.14276220561575));
#64927=CARTESIAN_POINT('Ctrl Pts',(-3.91787251936688,1.,-1.13788084225511));
#64928=CARTESIAN_POINT('Ctrl Pts',(-3.91187321145495,1.,-1.13303414693849));
#64929=CARTESIAN_POINT('Ctrl Pts',(-3.90585753318622,1.,-1.12822258281518));
#64930=CARTESIAN_POINT('Ctrl Pts',(-3.89982569749978,1.,-1.12344660099029));
#64931=CARTESIAN_POINT('Ctrl Pts',(-3.89377768340362,1.,-1.11870660794609));
#64932=CARTESIAN_POINT('Ctrl Pts',(-3.88771308285229,1.,-1.11400292434447));
#64933=CARTESIAN_POINT('Ctrl Pts',(-3.88163105531791,1.,-1.10933577224029));
#64934=CARTESIAN_POINT('Ctrl Pts',(-3.87553067187566,1.,-1.10470536603303));
#64935=CARTESIAN_POINT('Ctrl Pts',(-3.86941120134872,1.,-1.10011198761202));
#64936=CARTESIAN_POINT('Ctrl Pts',(-3.86327241021242,1.,-1.09555606505012));
#64937=CARTESIAN_POINT('Ctrl Pts',(-3.85711487933911,1.,-1.09103825516288));
#64938=CARTESIAN_POINT('Ctrl Pts',(-3.8509402522269,1.,-1.08655950846377));
#64939=CARTESIAN_POINT('Ctrl Pts',(-3.84475048030615,1.,-1.08212087917986));
#64940=CARTESIAN_POINT('Ctrl Pts',(-3.83854714117486,1.,-1.07772335353856));
#64941=CARTESIAN_POINT('Ctrl Pts',(-3.83233071195145,1.,-1.0733676663346));
#64942=CARTESIAN_POINT('Ctrl Pts',(-3.82609989967278,1.,-1.0690541318036));
#64943=CARTESIAN_POINT('Ctrl Pts',(-3.81985083953012,1.,-1.06478244038931));
#64944=CARTESIAN_POINT('Ctrl Pts',(-3.81357866117485,1.,-1.06055206187298));
#64945=CARTESIAN_POINT('Ctrl Pts',(-3.80727913637784,1.,-1.05636266918643));
#64946=CARTESIAN_POINT('Ctrl Pts',(-3.80095039790678,1.,-1.05221457990015));
#64947=CARTESIAN_POINT('Ctrl Pts',(-3.79459440308793,1.,-1.04810913267641));
#64948=CARTESIAN_POINT('Ctrl Pts',(-3.78821910787195,1.,-1.04404924374426));
#64949=CARTESIAN_POINT('Ctrl Pts',(-3.78183535008192,1.,-1.04003862055804));
#64950=CARTESIAN_POINT('Ctrl Pts',(-3.77545283140445,1.,-1.03608074678013));
#64951=CARTESIAN_POINT('Ctrl Pts',(-3.76907609832522,1.,-1.0321778660492));
#64952=CARTESIAN_POINT('Ctrl Pts',(-3.76270122291232,1.,-1.02833014458181));
#64953=CARTESIAN_POINT('Ctrl Pts',(-3.75631037456194,1.,-1.0245342944466));
#64954=CARTESIAN_POINT('Ctrl Pts',(-3.74987777155834,1.,-1.02078510487428));
#64955=CARTESIAN_POINT('Ctrl Pts',(-3.74337942504959,1.,-1.01707794311079));
#64956=CARTESIAN_POINT('Ctrl Pts',(-3.73680245055734,1.,-1.01341114319903));
#64957=CARTESIAN_POINT('Ctrl Pts',(-3.73015276704426,1.,-1.00978798539496));
#64958=CARTESIAN_POINT('Ctrl Pts',(-3.72346803750595,1.,-1.0062200073571));
#64959=CARTESIAN_POINT('Ctrl Pts',(-3.71680667125118,1.,-1.00272423396822));
#64960=CARTESIAN_POINT('Ctrl Pts',(-3.71022439713938,1.,-0.99931726075653));
#64961=CARTESIAN_POINT('Ctrl Pts',(-3.70375282282138,1.,-0.996009819772518));
#64962=CARTESIAN_POINT('Ctrl Pts',(-3.69738123415662,1.,-0.99280221833201));
#64963=CARTESIAN_POINT('Ctrl Pts',(-3.69102682138846,1.,-0.989676715398558));
#64964=CARTESIAN_POINT('Ctrl Pts',(-3.68455317926068,1.,-0.986602639863837));
#64965=CARTESIAN_POINT('Ctrl Pts',(-3.67782408841715,1.,-0.983550791470419));
#64966=CARTESIAN_POINT('Ctrl Pts',(-3.67074983340361,1.,-0.980505922458267));
#64967=CARTESIAN_POINT('Ctrl Pts',(-3.66333049637475,1.,-0.977478312751618));
#64968=CARTESIAN_POINT('Ctrl Pts',(-3.65571576735126,1.,-0.974519971354848));
#64969=CARTESIAN_POINT('Ctrl Pts',(-3.64819756447455,1.,-0.971722122061341));
#64970=CARTESIAN_POINT('Ctrl Pts',(-3.64113946505766,1.,-0.969195124675865));
#64971=CARTESIAN_POINT('Ctrl Pts',(-3.63492122081143,1.,-0.967052554541385));
#64972=CARTESIAN_POINT('Ctrl Pts',(-3.62988252139846,1.,-0.965395153165293));
#64973=CARTESIAN_POINT('Ctrl Pts',(-3.62652618145335,1.,-0.964373850166458));
#64974=CARTESIAN_POINT('Ctrl Pts',(-3.62489305727662,1.,-0.963957782642843));
#64975=CARTESIAN_POINT('Ctrl Pts',(-3.62424461507588,1.,-0.963861297423241));
#64976=CARTESIAN_POINT('Ctrl Pts',(-3.6240482887845,1.,-0.963880158555582));
#64977=CARTESIAN_POINT('Ctrl Pts',(-3.62400312501245,1.,-0.963899035117249));
#64978=CARTESIAN_POINT('',(-4.01728681790024,0.,-1.22531898815164));
#64979=CARTESIAN_POINT('Ctrl Pts',(-3.49848248301936,-1.,-1.35022972712301));
#64980=CARTESIAN_POINT('Ctrl Pts',(-3.49848248301936,1.,-1.35022972712301));
#64981=CARTESIAN_POINT('Ctrl Pts',(-3.4984026005375,-1.,-1.35026426118402));
#64982=CARTESIAN_POINT('Ctrl Pts',(-3.4984026005375,1.,-1.35026426118402));
#64983=CARTESIAN_POINT('Ctrl Pts',(-3.49840357193736,-1.,-1.35037650303019));
#64984=CARTESIAN_POINT('Ctrl Pts',(-3.49840357193736,1.,-1.35037650303019));
#64985=CARTESIAN_POINT('Ctrl Pts',(-3.49888720257132,-1.,-1.35067437417483));
#64986=CARTESIAN_POINT('Ctrl Pts',(-3.49888720257132,1.,-1.35067437417483));
#64987=CARTESIAN_POINT('Ctrl Pts',(-3.5004970706414,-1.,-1.3513307633124));
#64988=CARTESIAN_POINT('Ctrl Pts',(-3.5004970706414,1.,-1.3513307633124));
#64989=CARTESIAN_POINT('Ctrl Pts',(-3.50408168106261,-1.,-1.35257032843486));
#64990=CARTESIAN_POINT('Ctrl Pts',(-3.50408168106261,1.,-1.35257032843486));
#64991=CARTESIAN_POINT('Ctrl Pts',(-3.50913227059999,-1.,-1.35419113575956));
#64992=CARTESIAN_POINT('Ctrl Pts',(-3.50913227059999,1.,-1.35419113575956));
#64993=CARTESIAN_POINT('Ctrl Pts',(-3.51542230699556,-1.,-1.35611275237152));
#64994=CARTESIAN_POINT('Ctrl Pts',(-3.51542230699556,1.,-1.35611275237152));
#64995=CARTESIAN_POINT('Ctrl Pts',(-3.52261776116748,-1.,-1.35821701528836));
#64996=CARTESIAN_POINT('Ctrl Pts',(-3.52261776116748,1.,-1.35821701528836));
#64997=CARTESIAN_POINT('Ctrl Pts',(-3.530344649616,-1.,-1.36037259643734));
#64998=CARTESIAN_POINT('Ctrl Pts',(-3.530344649616,1.,-1.36037259643734));
#64999=CARTESIAN_POINT('Ctrl Pts',(-3.53824396424961,-1.,-1.36245507339307));
#65000=CARTESIAN_POINT('Ctrl Pts',(-3.53824396424961,1.,-1.36245507339307));
#65001=CARTESIAN_POINT('Ctrl Pts',(-3.54602591832973,-1.,-1.36436666257597));
#65002=CARTESIAN_POINT('Ctrl Pts',(-3.54602591832973,1.,-1.36436666257597));
#65003=CARTESIAN_POINT('Ctrl Pts',(-3.55353883995949,-1.,-1.3660614545677));
#65004=CARTESIAN_POINT('Ctrl Pts',(-3.55353883995949,1.,-1.3660614545677));
#65005=CARTESIAN_POINT('Ctrl Pts',(-3.56077662028649,-1.,-1.36754771771233));
#65006=CARTESIAN_POINT('Ctrl Pts',(-3.56077662028649,1.,-1.36754771771233));
#65007=CARTESIAN_POINT('Ctrl Pts',(-3.5678208030466,-1.,-1.36886584973389));
#65008=CARTESIAN_POINT('Ctrl Pts',(-3.5678208030466,1.,-1.36886584973389));
#65009=CARTESIAN_POINT('Ctrl Pts',(-3.57479875549486,-1.,-1.37007229485659));
#65010=CARTESIAN_POINT('Ctrl Pts',(-3.57479875549486,1.,-1.37007229485659));
#65011=CARTESIAN_POINT('Ctrl Pts',(-3.58183885982715,-1.,-1.37122241663062));
#65012=CARTESIAN_POINT('Ctrl Pts',(-3.58183885982715,1.,-1.37122241663062));
#65013=CARTESIAN_POINT('Ctrl Pts',(-3.58901853846365,-1.,-1.37235053660976));
#65014=CARTESIAN_POINT('Ctrl Pts',(-3.58901853846365,1.,-1.37235053660976));
#65015=CARTESIAN_POINT('Ctrl Pts',(-3.59634627869048,-1.,-1.37346320103157));
#65016=CARTESIAN_POINT('Ctrl Pts',(-3.59634627869048,1.,-1.37346320103157));
#65017=CARTESIAN_POINT('Ctrl Pts',(-3.60379020123988,-1.,-1.37455051379623));
#65018=CARTESIAN_POINT('Ctrl Pts',(-3.60379020123988,1.,-1.37455051379623));
#65019=CARTESIAN_POINT('Ctrl Pts',(-3.61129546591064,-1.,-1.37559314436634));
#65020=CARTESIAN_POINT('Ctrl Pts',(-3.61129546591064,1.,-1.37559314436634));
#65021=CARTESIAN_POINT('Ctrl Pts',(-3.6188048116042,-1.,-1.37657053403107));
#65022=CARTESIAN_POINT('Ctrl Pts',(-3.6188048116042,1.,-1.37657053403107));
#65023=CARTESIAN_POINT('Ctrl Pts',(-3.62628098665145,-1.,-1.37746987919881));
#65024=CARTESIAN_POINT('Ctrl Pts',(-3.62628098665145,1.,-1.37746987919881));
#65025=CARTESIAN_POINT('Ctrl Pts',(-3.63371727442486,-1.,-1.37829035457339));
#65026=CARTESIAN_POINT('Ctrl Pts',(-3.63371727442486,1.,-1.37829035457339));
#65027=CARTESIAN_POINT('Ctrl Pts',(-3.64112507791141,-1.,-1.37903818567359));
#65028=CARTESIAN_POINT('Ctrl Pts',(-3.64112507791141,1.,-1.37903818567359));
#65029=CARTESIAN_POINT('Ctrl Pts',(-3.64852652756456,-1.,-1.37972372481603));
#65030=CARTESIAN_POINT('Ctrl Pts',(-3.64852652756456,1.,-1.37972372481603));
#65031=CARTESIAN_POINT('Ctrl Pts',(-3.6559455440439,-1.,-1.38035791051212));
#65032=CARTESIAN_POINT('Ctrl Pts',(-3.6559455440439,1.,-1.38035791051212));
#65033=CARTESIAN_POINT('Ctrl Pts',(-3.66339848520857,-1.,-1.38094856333552));
#65034=CARTESIAN_POINT('Ctrl Pts',(-3.66339848520857,1.,-1.38094856333552));
#65035=CARTESIAN_POINT('Ctrl Pts',(-3.67088843112262,-1.,-1.38149812653868));
#65036=CARTESIAN_POINT('Ctrl Pts',(-3.67088843112262,1.,-1.38149812653868));
#65037=CARTESIAN_POINT('Ctrl Pts',(-3.67841038482414,-1.,-1.3820057429062));
#65038=CARTESIAN_POINT('Ctrl Pts',(-3.67841038482414,1.,-1.3820057429062));
#65039=CARTESIAN_POINT('Ctrl Pts',(-3.68595444983837,-1.,-1.38246852827182));
#65040=CARTESIAN_POINT('Ctrl Pts',(-3.68595444983837,1.,-1.38246852827182));
#65041=CARTESIAN_POINT('Ctrl Pts',(-3.69350967899526,-1.,-1.3828831117165));
#65042=CARTESIAN_POINT('Ctrl Pts',(-3.69350967899526,1.,-1.3828831117165));
#65043=CARTESIAN_POINT('Ctrl Pts',(-3.701067921679,-1.,-1.38324717612865));
#65044=CARTESIAN_POINT('Ctrl Pts',(-3.701067921679,1.,-1.38324717612865));
#65045=CARTESIAN_POINT('Ctrl Pts',(-3.70862680753347,-1.,-1.38356065402124));
#65046=CARTESIAN_POINT('Ctrl Pts',(-3.70862680753347,1.,-1.38356065402124));
#65047=CARTESIAN_POINT('Ctrl Pts',(-3.7161876605181,-1.,-1.38382489984586));
#65048=CARTESIAN_POINT('Ctrl Pts',(-3.7161876605181,1.,-1.38382489984586));
#65049=CARTESIAN_POINT('Ctrl Pts',(-3.72375409358803,-1.,-1.3840421342895));
#65050=CARTESIAN_POINT('Ctrl Pts',(-3.72375409358803,1.,-1.3840421342895));
#65051=CARTESIAN_POINT('Ctrl Pts',(-3.73133035859282,-1.,-1.38421479111531));
#65052=CARTESIAN_POINT('Ctrl Pts',(-3.73133035859282,1.,-1.38421479111531));
#65053=CARTESIAN_POINT('Ctrl Pts',(-3.73891976418104,-1.,-1.38434489156458));
#65054=CARTESIAN_POINT('Ctrl Pts',(-3.73891976418104,1.,-1.38434489156458));
#65055=CARTESIAN_POINT('Ctrl Pts',(-3.74652317167876,-1.,-1.38443344984394));
#65056=CARTESIAN_POINT('Ctrl Pts',(-3.74652317167876,1.,-1.38443344984394));
#65057=CARTESIAN_POINT('Ctrl Pts',(-3.7541397631875,-1.,-1.38448077997163));
#65058=CARTESIAN_POINT('Ctrl Pts',(-3.7541397631875,1.,-1.38448077997163));
#65059=CARTESIAN_POINT('Ctrl Pts',(-3.76176768271367,-1.,-1.3844867525335));
#65060=CARTESIAN_POINT('Ctrl Pts',(-3.76176768271367,1.,-1.3844867525335));
#65061=CARTESIAN_POINT('Ctrl Pts',(-3.76940473185779,-1.,-1.38445107339518));
#65062=CARTESIAN_POINT('Ctrl Pts',(-3.76940473185779,1.,-1.38445107339518));
#65063=CARTESIAN_POINT('Ctrl Pts',(-3.77704902230418,-1.,-1.38437354551428));
#65064=CARTESIAN_POINT('Ctrl Pts',(-3.77704902230418,1.,-1.38437354551428));
#65065=CARTESIAN_POINT('Ctrl Pts',(-3.78469969805082,-1.,-1.38425435883756));
#65066=CARTESIAN_POINT('Ctrl Pts',(-3.78469969805082,1.,-1.38425435883756));
#65067=CARTESIAN_POINT('Ctrl Pts',(-3.79235669640841,-1.,-1.38409399694566));
#65068=CARTESIAN_POINT('Ctrl Pts',(-3.79235669640841,1.,-1.38409399694566));
#65069=CARTESIAN_POINT('Ctrl Pts',(-3.80002044322111,-1.,-1.38389311766682));
#65070=CARTESIAN_POINT('Ctrl Pts',(-3.80002044322111,1.,-1.38389311766682));
#65071=CARTESIAN_POINT('Ctrl Pts',(-3.80769156398411,-1.,-1.3836524404622));
#65072=CARTESIAN_POINT('Ctrl Pts',(-3.80769156398411,1.,-1.3836524404622));
#65073=CARTESIAN_POINT('Ctrl Pts',(-3.81537060817811,-1.,-1.38337263902782));
#65074=CARTESIAN_POINT('Ctrl Pts',(-3.81537060817811,1.,-1.38337263902782));
#65075=CARTESIAN_POINT('Ctrl Pts',(-3.82305771743829,-1.,-1.38305421262763));
#65076=CARTESIAN_POINT('Ctrl Pts',(-3.82305771743829,1.,-1.38305421262763));
#65077=CARTESIAN_POINT('Ctrl Pts',(-3.8307526698229,-1.,-1.38269750245138));
#65078=CARTESIAN_POINT('Ctrl Pts',(-3.8307526698229,1.,-1.38269750245138));
#65079=CARTESIAN_POINT('Ctrl Pts',(-3.83845502790746,-1.,-1.38230274828821));
#65080=CARTESIAN_POINT('Ctrl Pts',(-3.83845502790746,1.,-1.38230274828821));
#65081=CARTESIAN_POINT('Ctrl Pts',(-3.84616425605764,-1.,-1.38187013346109));
#65082=CARTESIAN_POINT('Ctrl Pts',(-3.84616425605764,1.,-1.38187013346109));
#65083=CARTESIAN_POINT('Ctrl Pts',(-3.85387983979481,-1.,-1.38139983115049));
#65084=CARTESIAN_POINT('Ctrl Pts',(-3.85387983979481,1.,-1.38139983115049));
#65085=CARTESIAN_POINT('Ctrl Pts',(-3.86160143043959,-1.,-1.38089205992989));
#65086=CARTESIAN_POINT('Ctrl Pts',(-3.86160143043959,1.,-1.38089205992989));
#65087=CARTESIAN_POINT('Ctrl Pts',(-3.86932885813068,-1.,-1.38034709213014));
#65088=CARTESIAN_POINT('Ctrl Pts',(-3.86932885813068,1.,-1.38034709213014));
#65089=CARTESIAN_POINT('Ctrl Pts',(-3.87706205830532,-1.,-1.37976523097073));
#65090=CARTESIAN_POINT('Ctrl Pts',(-3.87706205830532,1.,-1.37976523097073));
#65091=CARTESIAN_POINT('Ctrl Pts',(-3.88480102249277,-1.,-1.37914679719383));
#65092=CARTESIAN_POINT('Ctrl Pts',(-3.88480102249277,1.,-1.37914679719383));
#65093=CARTESIAN_POINT('Ctrl Pts',(-3.89254574338496,-1.,-1.3784921128802));
#65094=CARTESIAN_POINT('Ctrl Pts',(-3.89254574338496,1.,-1.3784921128802));
#65095=CARTESIAN_POINT('Ctrl Pts',(-3.90029615196727,-1.,-1.37780148512792));
#65096=CARTESIAN_POINT('Ctrl Pts',(-3.90029615196727,1.,-1.37780148512792));
#65097=CARTESIAN_POINT('Ctrl Pts',(-3.90805209523486,-1.,-1.3770751963402));
#65098=CARTESIAN_POINT('Ctrl Pts',(-3.90805209523486,1.,-1.3770751963402));
#65099=CARTESIAN_POINT('Ctrl Pts',(-3.91581337462644,-1.,-1.37631350505797));
#65100=CARTESIAN_POINT('Ctrl Pts',(-3.91581337462644,1.,-1.37631350505797));
#65101=CARTESIAN_POINT('Ctrl Pts',(-3.92357976987672,-1.,-1.37551664448242));
#65102=CARTESIAN_POINT('Ctrl Pts',(-3.92357976987672,1.,-1.37551664448242));
#65103=CARTESIAN_POINT('Ctrl Pts',(-3.93135106761844,-1.,-1.37468482215751));
#65104=CARTESIAN_POINT('Ctrl Pts',(-3.93135106761844,1.,-1.37468482215751));
#65105=CARTESIAN_POINT('Ctrl Pts',(-3.93912709040818,-1.,-1.37381821967165));
#65106=CARTESIAN_POINT('Ctrl Pts',(-3.93912709040818,1.,-1.37381821967165));
#65107=CARTESIAN_POINT('Ctrl Pts',(-3.94690771785133,-1.,-1.37291699202807));
#65108=CARTESIAN_POINT('Ctrl Pts',(-3.94690771785133,1.,-1.37291699202807));
#65109=CARTESIAN_POINT('Ctrl Pts',(-3.95469287280914,-1.,-1.37198126432386));
#65110=CARTESIAN_POINT('Ctrl Pts',(-3.95469287280914,1.,-1.37198126432386));
#65111=CARTESIAN_POINT('Ctrl Pts',(-3.96092458506535,-1.,-1.3712051561502));
#65112=CARTESIAN_POINT('Ctrl Pts',(-3.96092458506535,1.,-1.3712051561502));
#65113=CARTESIAN_POINT('Ctrl Pts',(-3.96560037974645,-1.,-1.37060761745635));
#65114=CARTESIAN_POINT('Ctrl Pts',(-3.96560037974645,1.,-1.37060761745635));
#65115=CARTESIAN_POINT('Ctrl Pts',(-3.9687184694131,-1.,-1.37020239094614));
#65116=CARTESIAN_POINT('Ctrl Pts',(-3.9687184694131,1.,-1.37020239094614));
#65117=CARTESIAN_POINT('Ctrl Pts',(-3.97027773754922,-1.,-1.36999806084572));
#65118=CARTESIAN_POINT('Ctrl Pts',(-3.97027773754922,1.,-1.36999806084572));
#65119=CARTESIAN_POINT('',(-3.4984457533445,1.,-1.35032489087101));
#65120=CARTESIAN_POINT('Ctrl Pts',(-3.4984457533445,-1.,-1.35032489087101));
#65121=CARTESIAN_POINT('Ctrl Pts',(-3.4984457533445,-0.666666666666667,
-1.35032489087101));
#65122=CARTESIAN_POINT('Ctrl Pts',(-3.4984457533445,-0.333333333333333,
-1.35032489087101));
#65123=CARTESIAN_POINT('Ctrl Pts',(-3.4984457533445,0.333333333333333,-1.35032489087101));
#65124=CARTESIAN_POINT('Ctrl Pts',(-3.4984457533445,0.666666666666667,-1.35032489087101));
#65125=CARTESIAN_POINT('Ctrl Pts',(-3.4984457533445,1.,-1.35032489087101));
#65126=CARTESIAN_POINT('',(-3.97027773754922,1.,-1.36999806084572));
#65127=CARTESIAN_POINT('',(-3.97027773754922,0.,-1.36999806084572));
#65128=CARTESIAN_POINT('Ctrl Pts',(-3.4984457533445,1.,-1.35032489087101));
#65129=CARTESIAN_POINT('Ctrl Pts',(-3.49847119623846,1.,-1.35036670892966));
#65130=CARTESIAN_POINT('Ctrl Pts',(-3.49861894124827,1.,-1.35049736560527));
#65131=CARTESIAN_POINT('Ctrl Pts',(-3.49920025459723,1.,-1.35080045218587));
#65132=CARTESIAN_POINT('Ctrl Pts',(-3.5007660381649,1.,-1.35142377279517));
#65133=CARTESIAN_POINT('Ctrl Pts',(-3.50408168106261,1.,-1.35257032843486));
#65134=CARTESIAN_POINT('Ctrl Pts',(-3.50913227059999,1.,-1.35419113575956));
#65135=CARTESIAN_POINT('Ctrl Pts',(-3.51542230699556,1.,-1.35611275237152));
#65136=CARTESIAN_POINT('Ctrl Pts',(-3.52261776116748,1.,-1.35821701528836));
#65137=CARTESIAN_POINT('Ctrl Pts',(-3.530344649616,1.,-1.36037259643734));
#65138=CARTESIAN_POINT('Ctrl Pts',(-3.53824396424961,1.,-1.36245507339307));
#65139=CARTESIAN_POINT('Ctrl Pts',(-3.54602591832973,1.,-1.36436666257597));
#65140=CARTESIAN_POINT('Ctrl Pts',(-3.55353883995949,1.,-1.3660614545677));
#65141=CARTESIAN_POINT('Ctrl Pts',(-3.56077662028649,1.,-1.36754771771233));
#65142=CARTESIAN_POINT('Ctrl Pts',(-3.5678208030466,1.,-1.36886584973389));
#65143=CARTESIAN_POINT('Ctrl Pts',(-3.57479875549486,1.,-1.37007229485659));
#65144=CARTESIAN_POINT('Ctrl Pts',(-3.58183885982715,1.,-1.37122241663062));
#65145=CARTESIAN_POINT('Ctrl Pts',(-3.58901853846365,1.,-1.37235053660976));
#65146=CARTESIAN_POINT('Ctrl Pts',(-3.59634627869048,1.,-1.37346320103157));
#65147=CARTESIAN_POINT('Ctrl Pts',(-3.60379020123988,1.,-1.37455051379623));
#65148=CARTESIAN_POINT('Ctrl Pts',(-3.61129546591064,1.,-1.37559314436634));
#65149=CARTESIAN_POINT('Ctrl Pts',(-3.6188048116042,1.,-1.37657053403107));
#65150=CARTESIAN_POINT('Ctrl Pts',(-3.62628098665145,1.,-1.37746987919881));
#65151=CARTESIAN_POINT('Ctrl Pts',(-3.63371727442486,1.,-1.37829035457339));
#65152=CARTESIAN_POINT('Ctrl Pts',(-3.64112507791141,1.,-1.37903818567359));
#65153=CARTESIAN_POINT('Ctrl Pts',(-3.64852652756456,1.,-1.37972372481603));
#65154=CARTESIAN_POINT('Ctrl Pts',(-3.6559455440439,1.,-1.38035791051212));
#65155=CARTESIAN_POINT('Ctrl Pts',(-3.66339848520857,1.,-1.38094856333552));
#65156=CARTESIAN_POINT('Ctrl Pts',(-3.67088843112262,1.,-1.38149812653868));
#65157=CARTESIAN_POINT('Ctrl Pts',(-3.67841038482414,1.,-1.3820057429062));
#65158=CARTESIAN_POINT('Ctrl Pts',(-3.68595444983837,1.,-1.38246852827182));
#65159=CARTESIAN_POINT('Ctrl Pts',(-3.69350967899526,1.,-1.3828831117165));
#65160=CARTESIAN_POINT('Ctrl Pts',(-3.701067921679,1.,-1.38324717612865));
#65161=CARTESIAN_POINT('Ctrl Pts',(-3.70862680753347,1.,-1.38356065402124));
#65162=CARTESIAN_POINT('Ctrl Pts',(-3.7161876605181,1.,-1.38382489984586));
#65163=CARTESIAN_POINT('Ctrl Pts',(-3.72375409358803,1.,-1.3840421342895));
#65164=CARTESIAN_POINT('Ctrl Pts',(-3.73133035859282,1.,-1.38421479111531));
#65165=CARTESIAN_POINT('Ctrl Pts',(-3.73891976418104,1.,-1.38434489156458));
#65166=CARTESIAN_POINT('Ctrl Pts',(-3.74652317167876,1.,-1.38443344984394));
#65167=CARTESIAN_POINT('Ctrl Pts',(-3.7541397631875,1.,-1.38448077997163));
#65168=CARTESIAN_POINT('Ctrl Pts',(-3.76176768271367,1.,-1.3844867525335));
#65169=CARTESIAN_POINT('Ctrl Pts',(-3.76940473185779,1.,-1.38445107339518));
#65170=CARTESIAN_POINT('Ctrl Pts',(-3.77704902230418,1.,-1.38437354551428));
#65171=CARTESIAN_POINT('Ctrl Pts',(-3.78469969805082,1.,-1.38425435883756));
#65172=CARTESIAN_POINT('Ctrl Pts',(-3.79235669640841,1.,-1.38409399694566));
#65173=CARTESIAN_POINT('Ctrl Pts',(-3.80002044322111,1.,-1.38389311766682));
#65174=CARTESIAN_POINT('Ctrl Pts',(-3.80769156398411,1.,-1.3836524404622));
#65175=CARTESIAN_POINT('Ctrl Pts',(-3.81537060817811,1.,-1.38337263902782));
#65176=CARTESIAN_POINT('Ctrl Pts',(-3.82305771743829,1.,-1.38305421262763));
#65177=CARTESIAN_POINT('Ctrl Pts',(-3.8307526698229,1.,-1.38269750245138));
#65178=CARTESIAN_POINT('Ctrl Pts',(-3.83845502790746,1.,-1.38230274828821));
#65179=CARTESIAN_POINT('Ctrl Pts',(-3.84616425605764,1.,-1.38187013346109));
#65180=CARTESIAN_POINT('Ctrl Pts',(-3.85387983979481,1.,-1.38139983115049));
#65181=CARTESIAN_POINT('Ctrl Pts',(-3.86160143043959,1.,-1.38089205992989));
#65182=CARTESIAN_POINT('Ctrl Pts',(-3.86932885813068,1.,-1.38034709213014));
#65183=CARTESIAN_POINT('Ctrl Pts',(-3.87706205830532,1.,-1.37976523097073));
#65184=CARTESIAN_POINT('Ctrl Pts',(-3.88480102249277,1.,-1.37914679719383));
#65185=CARTESIAN_POINT('Ctrl Pts',(-3.89254574338496,1.,-1.3784921128802));
#65186=CARTESIAN_POINT('Ctrl Pts',(-3.90029615196727,1.,-1.37780148512792));
#65187=CARTESIAN_POINT('Ctrl Pts',(-3.90805209523486,1.,-1.3770751963402));
#65188=CARTESIAN_POINT('Ctrl Pts',(-3.91581337462644,1.,-1.37631350505797));
#65189=CARTESIAN_POINT('Ctrl Pts',(-3.92357976987672,1.,-1.37551664448242));
#65190=CARTESIAN_POINT('Ctrl Pts',(-3.93135106761844,1.,-1.37468482215751));
#65191=CARTESIAN_POINT('Ctrl Pts',(-3.93912709040818,1.,-1.37381821967165));
#65192=CARTESIAN_POINT('Ctrl Pts',(-3.94690771785133,1.,-1.37291699202807));
#65193=CARTESIAN_POINT('Ctrl Pts',(-3.95469287280914,1.,-1.37198126432386));
#65194=CARTESIAN_POINT('Ctrl Pts',(-3.96092458506535,1.,-1.3712051561502));
#65195=CARTESIAN_POINT('Ctrl Pts',(-3.96560037974645,1.,-1.37060761745635));
#65196=CARTESIAN_POINT('Ctrl Pts',(-3.9687184694131,1.,-1.37020239094614));
#65197=CARTESIAN_POINT('Ctrl Pts',(-3.97027773754922,1.,-1.36999806084572));
#65198=CARTESIAN_POINT('Origin',(-3.97027773754922,0.,-1.36999806084572));
#65199=CARTESIAN_POINT('',(-4.01728681790024,1.,-1.22531898815164));
#65200=CARTESIAN_POINT('Origin',(0.,0.,0.));
#65201=CARTESIAN_POINT('',(-3.42859860294378,1.,-1.51895082866166));
#65202=CARTESIAN_POINT('Origin',(0.,1.,0.));
#65203=CARTESIAN_POINT('Ctrl Pts',(-3.42859860294378,1.,-1.51895082866166));
#65204=CARTESIAN_POINT('Ctrl Pts',(-3.42859860294378,0.666666666666667,
-1.51895082866166));
#65205=CARTESIAN_POINT('Ctrl Pts',(-3.42859860294378,0.333333333333333,
-1.51895082866166));
#65206=CARTESIAN_POINT('Ctrl Pts',(-3.42859860294378,-0.333333333333333,
-1.51895082866166));
#65207=CARTESIAN_POINT('Ctrl Pts',(-3.42859860294378,-0.666666666666667,
-1.51895082866166));
#65208=CARTESIAN_POINT('Ctrl Pts',(-3.42859860294378,-1.,-1.51895082866166));
#65209=CARTESIAN_POINT('Ctrl Pts',(-3.77614523045147,-1.,-1.83867539237861));
#65210=CARTESIAN_POINT('Ctrl Pts',(-3.77614523045147,1.,-1.83867539237861));
#65211=CARTESIAN_POINT('Ctrl Pts',(-3.77518714458232,-1.,-1.83742834010821));
#65212=CARTESIAN_POINT('Ctrl Pts',(-3.77518714458232,1.,-1.83742834010821));
#65213=CARTESIAN_POINT('Ctrl Pts',(-3.77326886065484,-1.,-1.83493697935064));
#65214=CARTESIAN_POINT('Ctrl Pts',(-3.77326886065484,1.,-1.83493697935064));
#65215=CARTESIAN_POINT('Ctrl Pts',(-3.77038509819777,-1.,-1.83120816956515));
#65216=CARTESIAN_POINT('Ctrl Pts',(-3.77038509819777,1.,-1.83120816956515));
#65217=CARTESIAN_POINT('Ctrl Pts',(-3.76652740355856,-1.,-1.82625289221933));
#65218=CARTESIAN_POINT('Ctrl Pts',(-3.76652740355856,1.,-1.82625289221933));
#65219=CARTESIAN_POINT('Ctrl Pts',(-3.76168412709652,-1.,-1.82008629694924));
#65220=CARTESIAN_POINT('Ctrl Pts',(-3.76168412709652,1.,-1.82008629694924));
#65221=CARTESIAN_POINT('Ctrl Pts',(-3.75681965683995,-1.,-1.81394729834032));
#65222=CARTESIAN_POINT('Ctrl Pts',(-3.75681965683995,1.,-1.81394729834032));
#65223=CARTESIAN_POINT('Ctrl Pts',(-3.75193395888069,-1.,-1.80783603939662));
#65224=CARTESIAN_POINT('Ctrl Pts',(-3.75193395888069,1.,-1.80783603939662));
#65225=CARTESIAN_POINT('Ctrl Pts',(-3.74702700874954,-1.,-1.80175271485519));
#65226=CARTESIAN_POINT('Ctrl Pts',(-3.74702700874954,1.,-1.80175271485519));
#65227=CARTESIAN_POINT('Ctrl Pts',(-3.74209880351667,-1.,-1.79569757859041));
#65228=CARTESIAN_POINT('Ctrl Pts',(-3.74209880351667,1.,-1.79569757859041));
#65229=CARTESIAN_POINT('Ctrl Pts',(-3.73714934729962,-1.,-1.78967092823139));
#65230=CARTESIAN_POINT('Ctrl Pts',(-3.73714934729962,1.,-1.78967092823139));
#65231=CARTESIAN_POINT('Ctrl Pts',(-3.73217863095022,-1.,-1.78367308442682));
#65232=CARTESIAN_POINT('Ctrl Pts',(-3.73217863095022,1.,-1.78367308442682));
#65233=CARTESIAN_POINT('Ctrl Pts',(-3.72718661205504,-1.,-1.77770437039606));
#65234=CARTESIAN_POINT('Ctrl Pts',(-3.72718661205504,1.,-1.77770437039606));
#65235=CARTESIAN_POINT('Ctrl Pts',(-3.72217319911429,-1.,-1.77176509401846));
#65236=CARTESIAN_POINT('Ctrl Pts',(-3.72217319911429,1.,-1.77176509401846));
#65237=CARTESIAN_POINT('Ctrl Pts',(-3.71713822377675,-1.,-1.76585552124549));
#65238=CARTESIAN_POINT('Ctrl Pts',(-3.71713822377675,1.,-1.76585552124549));
#65239=CARTESIAN_POINT('Ctrl Pts',(-3.71208146346454,-1.,-1.75997588499021));
#65240=CARTESIAN_POINT('Ctrl Pts',(-3.71208146346454,1.,-1.75997588499021));
#65241=CARTESIAN_POINT('Ctrl Pts',(-3.70700269736876,-1.,-1.75412641804148));
#65242=CARTESIAN_POINT('Ctrl Pts',(-3.70700269736876,1.,-1.75412641804148));
#65243=CARTESIAN_POINT('Ctrl Pts',(-3.70190175673422,-1.,-1.74830738046092));
#65244=CARTESIAN_POINT('Ctrl Pts',(-3.70190175673422,1.,-1.74830738046092));
#65245=CARTESIAN_POINT('Ctrl Pts',(-3.6967785691046,-1.,-1.74251908492589));
#65246=CARTESIAN_POINT('Ctrl Pts',(-3.6967785691046,1.,-1.74251908492589));
#65247=CARTESIAN_POINT('Ctrl Pts',(-3.69163322647906,-1.,-1.73676193254493));
#65248=CARTESIAN_POINT('Ctrl Pts',(-3.69163322647906,1.,-1.73676193254493));
#65249=CARTESIAN_POINT('Ctrl Pts',(-3.68646597019188,-1.,-1.73103640956647));
#65250=CARTESIAN_POINT('Ctrl Pts',(-3.68646597019188,1.,-1.73103640956647));
#65251=CARTESIAN_POINT('Ctrl Pts',(-3.68127704936472,-1.,-1.72534302437003));
#65252=CARTESIAN_POINT('Ctrl Pts',(-3.68127704936472,1.,-1.72534302437003));
#65253=CARTESIAN_POINT('Ctrl Pts',(-3.67606660374665,-1.,-1.71968225581787));
#65254=CARTESIAN_POINT('Ctrl Pts',(-3.67606660374665,1.,-1.71968225581787));
#65255=CARTESIAN_POINT('Ctrl Pts',(-3.67083454901629,-1.,-1.71405450210392));
#65256=CARTESIAN_POINT('Ctrl Pts',(-3.67083454901629,1.,-1.71405450210392));
#65257=CARTESIAN_POINT('Ctrl Pts',(-3.6655804319893,-1.,-1.70846001610983));
#65258=CARTESIAN_POINT('Ctrl Pts',(-3.6655804319893,1.,-1.70846001610983));
#65259=CARTESIAN_POINT('Ctrl Pts',(-3.6603033877491,-1.,-1.70289888566904));
#65260=CARTESIAN_POINT('Ctrl Pts',(-3.6603033877491,1.,-1.70289888566904));
#65261=CARTESIAN_POINT('Ctrl Pts',(-3.65500246526798,-1.,-1.69737117722558));
#65262=CARTESIAN_POINT('Ctrl Pts',(-3.65500246526798,1.,-1.69737117722558));
#65263=CARTESIAN_POINT('Ctrl Pts',(-3.64967689827393,-1.,-1.691877054817));
#65264=CARTESIAN_POINT('Ctrl Pts',(-3.64967689827393,1.,-1.691877054817));
#65265=CARTESIAN_POINT('Ctrl Pts',(-3.64432638915199,-1.,-1.68641690471455));
#65266=CARTESIAN_POINT('Ctrl Pts',(-3.64432638915199,1.,-1.68641690471455));
#65267=CARTESIAN_POINT('Ctrl Pts',(-3.63895140887443,-1.,-1.68099146651577));
#65268=CARTESIAN_POINT('Ctrl Pts',(-3.63895140887443,1.,-1.68099146651577));
#65269=CARTESIAN_POINT('Ctrl Pts',(-3.63355343201211,-1.,-1.67560193613145));
#65270=CARTESIAN_POINT('Ctrl Pts',(-3.63355343201211,1.,-1.67560193613145));
#65271=CARTESIAN_POINT('Ctrl Pts',(-3.62813422105257,-1.,-1.67024966008037));
#65272=CARTESIAN_POINT('Ctrl Pts',(-3.62813422105257,1.,-1.67024966008037));
#65273=CARTESIAN_POINT('Ctrl Pts',(-3.62269517989104,-1.,-1.66493585923853));
#65274=CARTESIAN_POINT('Ctrl Pts',(-3.62269517989104,1.,-1.66493585923853));
#65275=CARTESIAN_POINT('Ctrl Pts',(-3.61723666482457,-1.,-1.65966133399186));
#65276=CARTESIAN_POINT('Ctrl Pts',(-3.61723666482457,1.,-1.65966133399186));
#65277=CARTESIAN_POINT('Ctrl Pts',(-3.61175734965129,-1.,-1.65442619244327));
#65278=CARTESIAN_POINT('Ctrl Pts',(-3.61175734965129,1.,-1.65442619244327));
#65279=CARTESIAN_POINT('Ctrl Pts',(-3.60625346556992,-1.,-1.64922952425833));
#65280=CARTESIAN_POINT('Ctrl Pts',(-3.60625346556992,1.,-1.64922952425833));
#65281=CARTESIAN_POINT('Ctrl Pts',(-3.6007202851384,-1.,-1.6440700438558));
#65282=CARTESIAN_POINT('Ctrl Pts',(-3.6007202851384,1.,-1.6440700438558));
#65283=CARTESIAN_POINT('Ctrl Pts',(-3.59515368334887,-1.,-1.63894676675349));
#65284=CARTESIAN_POINT('Ctrl Pts',(-3.59515368334887,1.,-1.63894676675349));
#65285=CARTESIAN_POINT('Ctrl Pts',(-3.58955176627876,-1.,-1.63385971451259));
#65286=CARTESIAN_POINT('Ctrl Pts',(-3.58955176627876,1.,-1.63385971451259));
#65287=CARTESIAN_POINT('Ctrl Pts',(-3.5839162577435,-1.,-1.62881051550748));
#65288=CARTESIAN_POINT('Ctrl Pts',(-3.5839162577435,1.,-1.62881051550748));
#65289=CARTESIAN_POINT('Ctrl Pts',(-3.57825455954405,-1.,-1.62380329464851));
#65290=CARTESIAN_POINT('Ctrl Pts',(-3.57825455954405,1.,-1.62380329464851));
#65291=CARTESIAN_POINT('Ctrl Pts',(-3.57257679609826,-1.,-1.61884340915412));
#65292=CARTESIAN_POINT('Ctrl Pts',(-3.57257679609826,1.,-1.61884340915412));
#65293=CARTESIAN_POINT('Ctrl Pts',(-3.56689200468404,-1.,-1.61393581747522));
#65294=CARTESIAN_POINT('Ctrl Pts',(-3.56689200468404,1.,-1.61393581747522));
#65295=CARTESIAN_POINT('Ctrl Pts',(-3.56120432482986,-1.,-1.60908344685459));
#65296=CARTESIAN_POINT('Ctrl Pts',(-3.56120432482986,1.,-1.60908344685459));
#65297=CARTESIAN_POINT('Ctrl Pts',(-3.55550985096117,-1.,-1.60428584699848));
#65298=CARTESIAN_POINT('Ctrl Pts',(-3.55550985096117,1.,-1.60428584699848));
#65299=CARTESIAN_POINT('Ctrl Pts',(-3.54979148634426,-1.,-1.59953698113444));
#65300=CARTESIAN_POINT('Ctrl Pts',(-3.54979148634426,1.,-1.59953698113444));
#65301=CARTESIAN_POINT('Ctrl Pts',(-3.544024581823,-1.,-1.5948276694975));
#65302=CARTESIAN_POINT('Ctrl Pts',(-3.544024581823,1.,-1.5948276694975));
#65303=CARTESIAN_POINT('Ctrl Pts',(-3.53818616861045,-1.,-1.59014958368725));
#65304=CARTESIAN_POINT('Ctrl Pts',(-3.53818616861045,1.,-1.59014958368725));
#65305=CARTESIAN_POINT('Ctrl Pts',(-3.53226378147068,-1.,-1.58549906268083));
#65306=CARTESIAN_POINT('Ctrl Pts',(-3.53226378147068,1.,-1.58549906268083));
#65307=CARTESIAN_POINT('Ctrl Pts',(-3.52626275334899,-1.,-1.58088027227856));
#65308=CARTESIAN_POINT('Ctrl Pts',(-3.52626275334899,1.,-1.58088027227856));
#65309=CARTESIAN_POINT('Ctrl Pts',(-3.52021847865961,-1.,-1.5763104998818));
#65310=CARTESIAN_POINT('Ctrl Pts',(-3.52021847865961,1.,-1.5763104998818));
#65311=CARTESIAN_POINT('Ctrl Pts',(-3.51418598431733,-1.,-1.57181569799774));
#65312=CARTESIAN_POINT('Ctrl Pts',(-3.51418598431733,1.,-1.57181569799774));
#65313=CARTESIAN_POINT('Ctrl Pts',(-3.50821771695427,-1.,-1.56742097575041));
#65314=CARTESIAN_POINT('Ctrl Pts',(-3.50821771695427,1.,-1.56742097575041));
#65315=CARTESIAN_POINT('Ctrl Pts',(-3.50234321621607,-1.,-1.56314187758689));
#65316=CARTESIAN_POINT('Ctrl Pts',(-3.50234321621607,1.,-1.56314187758689));
#65317=CARTESIAN_POINT('Ctrl Pts',(-3.49655185179623,-1.,-1.55897703097859));
#65318=CARTESIAN_POINT('Ctrl Pts',(-3.49655185179623,1.,-1.55897703097859));
#65319=CARTESIAN_POINT('Ctrl Pts',(-3.49076460877317,-1.,-1.5548959590107));
#65320=CARTESIAN_POINT('Ctrl Pts',(-3.49076460877317,1.,-1.5548959590107));
#65321=CARTESIAN_POINT('Ctrl Pts',(-3.48485155928414,-1.,-1.55084702970382));
#65322=CARTESIAN_POINT('Ctrl Pts',(-3.48485155928414,1.,-1.55084702970382));
#65323=CARTESIAN_POINT('Ctrl Pts',(-3.47868272898599,-1.,-1.54678009290206));
#65324=CARTESIAN_POINT('Ctrl Pts',(-3.47868272898599,1.,-1.54678009290206));
#65325=CARTESIAN_POINT('Ctrl Pts',(-3.47217189224576,-1.,-1.54266605398152));
#65326=CARTESIAN_POINT('Ctrl Pts',(-3.47217189224576,1.,-1.54266605398152));
#65327=CARTESIAN_POINT('Ctrl Pts',(-3.46531752207222,-1.,-1.53851507915533));
#65328=CARTESIAN_POINT('Ctrl Pts',(-3.46531752207222,1.,-1.53851507915533));
#65329=CARTESIAN_POINT('Ctrl Pts',(-3.45825932955273,-1.,-1.53440195378902));
#65330=CARTESIAN_POINT('Ctrl Pts',(-3.45825932955273,1.,-1.53440195378902));
#65331=CARTESIAN_POINT('Ctrl Pts',(-3.45127136828667,-1.,-1.530462444618));
#65332=CARTESIAN_POINT('Ctrl Pts',(-3.45127136828667,1.,-1.530462444618));
#65333=CARTESIAN_POINT('Ctrl Pts',(-3.44469547527,-1.,-1.52686242875717));
#65334=CARTESIAN_POINT('Ctrl Pts',(-3.44469547527,1.,-1.52686242875717));
#65335=CARTESIAN_POINT('Ctrl Pts',(-3.43888895974182,-1.,-1.52377348950429));
#65336=CARTESIAN_POINT('Ctrl Pts',(-3.43888895974182,1.,-1.52377348950429));
#65337=CARTESIAN_POINT('Ctrl Pts',(-3.43417156977749,-1.,-1.52134826724227));
#65338=CARTESIAN_POINT('Ctrl Pts',(-3.43417156977749,1.,-1.52134826724227));
#65339=CARTESIAN_POINT('Ctrl Pts',(-3.43076036253384,-1.,-1.51969006980792));
#65340=CARTESIAN_POINT('Ctrl Pts',(-3.43076036253384,1.,-1.51969006980792));
#65341=CARTESIAN_POINT('Ctrl Pts',(-3.42915787669388,-1.,-1.51901585838879));
#65342=CARTESIAN_POINT('Ctrl Pts',(-3.42915787669388,1.,-1.51901585838879));
#65343=CARTESIAN_POINT('Ctrl Pts',(-3.42860527148835,-1.,-1.51888450659497));
#65344=CARTESIAN_POINT('Ctrl Pts',(-3.42860527148835,1.,-1.51888450659497));
#65345=CARTESIAN_POINT('Ctrl Pts',(-3.42852521763648,-1.,-1.51896318668306));
#65346=CARTESIAN_POINT('Ctrl Pts',(-3.42852521763648,1.,-1.51896318668306));
#65347=CARTESIAN_POINT('Ctrl Pts',(-3.42855728381368,-1.,-1.519044091397));
#65348=CARTESIAN_POINT('Ctrl Pts',(-3.42855728381368,1.,-1.519044091397));
#65349=CARTESIAN_POINT('',(-3.77614523045147,1.,-1.83867539237861));
#65350=CARTESIAN_POINT('Ctrl Pts',(-3.77614523045147,1.,-1.83867539237861));
#65351=CARTESIAN_POINT('Ctrl Pts',(-3.77518714458232,1.,-1.83742834010821));
#65352=CARTESIAN_POINT('Ctrl Pts',(-3.77326886065484,1.,-1.83493697935064));
#65353=CARTESIAN_POINT('Ctrl Pts',(-3.77038509819777,1.,-1.83120816956515));
#65354=CARTESIAN_POINT('Ctrl Pts',(-3.76652740355856,1.,-1.82625289221933));
#65355=CARTESIAN_POINT('Ctrl Pts',(-3.76168412709652,1.,-1.82008629694924));
#65356=CARTESIAN_POINT('Ctrl Pts',(-3.75681965683995,1.,-1.81394729834032));
#65357=CARTESIAN_POINT('Ctrl Pts',(-3.75193395888069,1.,-1.80783603939662));
#65358=CARTESIAN_POINT('Ctrl Pts',(-3.74702700874954,1.,-1.80175271485519));
#65359=CARTESIAN_POINT('Ctrl Pts',(-3.74209880351667,1.,-1.79569757859041));
#65360=CARTESIAN_POINT('Ctrl Pts',(-3.73714934729962,1.,-1.78967092823139));
#65361=CARTESIAN_POINT('Ctrl Pts',(-3.73217863095022,1.,-1.78367308442682));
#65362=CARTESIAN_POINT('Ctrl Pts',(-3.72718661205504,1.,-1.77770437039606));
#65363=CARTESIAN_POINT('Ctrl Pts',(-3.72217319911429,1.,-1.77176509401846));
#65364=CARTESIAN_POINT('Ctrl Pts',(-3.71713822377675,1.,-1.76585552124549));
#65365=CARTESIAN_POINT('Ctrl Pts',(-3.71208146346454,1.,-1.75997588499021));
#65366=CARTESIAN_POINT('Ctrl Pts',(-3.70700269736876,1.,-1.75412641804148));
#65367=CARTESIAN_POINT('Ctrl Pts',(-3.70190175673422,1.,-1.74830738046092));
#65368=CARTESIAN_POINT('Ctrl Pts',(-3.6967785691046,1.,-1.74251908492589));
#65369=CARTESIAN_POINT('Ctrl Pts',(-3.69163322647906,1.,-1.73676193254493));
#65370=CARTESIAN_POINT('Ctrl Pts',(-3.68646597019188,1.,-1.73103640956647));
#65371=CARTESIAN_POINT('Ctrl Pts',(-3.68127704936472,1.,-1.72534302437003));
#65372=CARTESIAN_POINT('Ctrl Pts',(-3.67606660374665,1.,-1.71968225581787));
#65373=CARTESIAN_POINT('Ctrl Pts',(-3.67083454901629,1.,-1.71405450210392));
#65374=CARTESIAN_POINT('Ctrl Pts',(-3.6655804319893,1.,-1.70846001610983));
#65375=CARTESIAN_POINT('Ctrl Pts',(-3.6603033877491,1.,-1.70289888566904));
#65376=CARTESIAN_POINT('Ctrl Pts',(-3.65500246526798,1.,-1.69737117722558));
#65377=CARTESIAN_POINT('Ctrl Pts',(-3.64967689827393,1.,-1.691877054817));
#65378=CARTESIAN_POINT('Ctrl Pts',(-3.64432638915199,1.,-1.68641690471455));
#65379=CARTESIAN_POINT('Ctrl Pts',(-3.63895140887443,1.,-1.68099146651577));
#65380=CARTESIAN_POINT('Ctrl Pts',(-3.63355343201211,1.,-1.67560193613145));
#65381=CARTESIAN_POINT('Ctrl Pts',(-3.62813422105257,1.,-1.67024966008037));
#65382=CARTESIAN_POINT('Ctrl Pts',(-3.62269517989104,1.,-1.66493585923853));
#65383=CARTESIAN_POINT('Ctrl Pts',(-3.61723666482457,1.,-1.65966133399186));
#65384=CARTESIAN_POINT('Ctrl Pts',(-3.61175734965129,1.,-1.65442619244327));
#65385=CARTESIAN_POINT('Ctrl Pts',(-3.60625346556992,1.,-1.64922952425833));
#65386=CARTESIAN_POINT('Ctrl Pts',(-3.6007202851384,1.,-1.6440700438558));
#65387=CARTESIAN_POINT('Ctrl Pts',(-3.59515368334887,1.,-1.63894676675349));
#65388=CARTESIAN_POINT('Ctrl Pts',(-3.58955176627876,1.,-1.63385971451259));
#65389=CARTESIAN_POINT('Ctrl Pts',(-3.5839162577435,1.,-1.62881051550748));
#65390=CARTESIAN_POINT('Ctrl Pts',(-3.57825455954405,1.,-1.62380329464851));
#65391=CARTESIAN_POINT('Ctrl Pts',(-3.57257679609826,1.,-1.61884340915412));
#65392=CARTESIAN_POINT('Ctrl Pts',(-3.56689200468404,1.,-1.61393581747522));
#65393=CARTESIAN_POINT('Ctrl Pts',(-3.56120432482986,1.,-1.60908344685459));
#65394=CARTESIAN_POINT('Ctrl Pts',(-3.55550985096117,1.,-1.60428584699848));
#65395=CARTESIAN_POINT('Ctrl Pts',(-3.54979148634426,1.,-1.59953698113444));
#65396=CARTESIAN_POINT('Ctrl Pts',(-3.544024581823,1.,-1.5948276694975));
#65397=CARTESIAN_POINT('Ctrl Pts',(-3.53818616861045,1.,-1.59014958368725));
#65398=CARTESIAN_POINT('Ctrl Pts',(-3.53226378147068,1.,-1.58549906268083));
#65399=CARTESIAN_POINT('Ctrl Pts',(-3.52626275334899,1.,-1.58088027227856));
#65400=CARTESIAN_POINT('Ctrl Pts',(-3.52021847865961,1.,-1.5763104998818));
#65401=CARTESIAN_POINT('Ctrl Pts',(-3.51418598431733,1.,-1.57181569799774));
#65402=CARTESIAN_POINT('Ctrl Pts',(-3.50821771695427,1.,-1.56742097575041));
#65403=CARTESIAN_POINT('Ctrl Pts',(-3.50234321621607,1.,-1.56314187758689));
#65404=CARTESIAN_POINT('Ctrl Pts',(-3.49655185179623,1.,-1.55897703097859));
#65405=CARTESIAN_POINT('Ctrl Pts',(-3.49076460877317,1.,-1.5548959590107));
#65406=CARTESIAN_POINT('Ctrl Pts',(-3.48485155928414,1.,-1.55084702970382));
#65407=CARTESIAN_POINT('Ctrl Pts',(-3.47868272898599,1.,-1.54678009290206));
#65408=CARTESIAN_POINT('Ctrl Pts',(-3.47217189224576,1.,-1.54266605398152));
#65409=CARTESIAN_POINT('Ctrl Pts',(-3.46531752207222,1.,-1.53851507915533));
#65410=CARTESIAN_POINT('Ctrl Pts',(-3.45825932955273,1.,-1.53440195378902));
#65411=CARTESIAN_POINT('Ctrl Pts',(-3.45127136828667,1.,-1.530462444618));
#65412=CARTESIAN_POINT('Ctrl Pts',(-3.44469547527,1.,-1.52686242875717));
#65413=CARTESIAN_POINT('Ctrl Pts',(-3.43888895974182,1.,-1.52377348950429));
#65414=CARTESIAN_POINT('Ctrl Pts',(-3.43417156977749,1.,-1.52134826724227));
#65415=CARTESIAN_POINT('Ctrl Pts',(-3.43101631893491,1.,-1.5198144909343));
#65416=CARTESIAN_POINT('Ctrl Pts',(-3.42946838852728,1.,-1.51914806898539));
#65417=CARTESIAN_POINT('Ctrl Pts',(-3.42884302333978,1.,-1.51895133295017));
#65418=CARTESIAN_POINT('Ctrl Pts',(-3.42864616361967,1.,-1.51893924967231));
#65419=CARTESIAN_POINT('Ctrl Pts',(-3.42859860294378,1.,-1.51895082866166));
#65420=CARTESIAN_POINT('',(-3.77614523045147,0.,-1.83867539237861));
#65421=CARTESIAN_POINT('Ctrl Pts',(-3.24418789321065,-1.,-1.8808893942881));
#65422=CARTESIAN_POINT('Ctrl Pts',(-3.24418789321065,1.,-1.8808893942881));
#65423=CARTESIAN_POINT('Ctrl Pts',(-3.24410359189733,-1.,-1.8809110068042));
#65424=CARTESIAN_POINT('Ctrl Pts',(-3.24410359189733,1.,-1.8809110068042));
#65425=CARTESIAN_POINT('Ctrl Pts',(-3.24408699284449,-1.,-1.8810220187274));
#65426=CARTESIAN_POINT('Ctrl Pts',(-3.24408699284449,1.,-1.8810220187274));
#65427=CARTESIAN_POINT('Ctrl Pts',(-3.24451807186964,-1.,-1.88139187908347));
#65428=CARTESIAN_POINT('Ctrl Pts',(-3.24451807186964,1.,-1.88139187908347));
#65429=CARTESIAN_POINT('Ctrl Pts',(-3.24600543790876,-1.,-1.88229202583187));
#65430=CARTESIAN_POINT('Ctrl Pts',(-3.24600543790876,1.,-1.88229202583187));
#65431=CARTESIAN_POINT('Ctrl Pts',(-3.24935200512055,-1.,-1.88407708646435));
#65432=CARTESIAN_POINT('Ctrl Pts',(-3.24935200512055,1.,-1.88407708646435));
#65433=CARTESIAN_POINT('Ctrl Pts',(-3.25408686339298,-1.,-1.88646802523372));
#65434=CARTESIAN_POINT('Ctrl Pts',(-3.25408686339298,1.,-1.88646802523372));
#65435=CARTESIAN_POINT('Ctrl Pts',(-3.2599988519361,-1.,-1.88934996203508));
#65436=CARTESIAN_POINT('Ctrl Pts',(-3.2599988519361,1.,-1.88934996203508));
#65437=CARTESIAN_POINT('Ctrl Pts',(-3.2667765388833,-1.,-1.89255393500769));
#65438=CARTESIAN_POINT('Ctrl Pts',(-3.2667765388833,1.,-1.89255393500769));
#65439=CARTESIAN_POINT('Ctrl Pts',(-3.27407108932908,-1.,-1.89589172903662));
#65440=CARTESIAN_POINT('Ctrl Pts',(-3.27407108932908,1.,-1.89589172903662));
#65441=CARTESIAN_POINT('Ctrl Pts',(-3.28154737912287,-1.,-1.89918429230424));
#65442=CARTESIAN_POINT('Ctrl Pts',(-3.28154737912287,1.,-1.89918429230424));
#65443=CARTESIAN_POINT('Ctrl Pts',(-3.28893448600364,-1.,-1.9022897124757));
#65444=CARTESIAN_POINT('Ctrl Pts',(-3.28893448600364,1.,-1.9022897124757));
#65445=CARTESIAN_POINT('Ctrl Pts',(-3.29608978722258,-1.,-1.9051389186417));
#65446=CARTESIAN_POINT('Ctrl Pts',(-3.29608978722258,1.,-1.9051389186417));
#65447=CARTESIAN_POINT('Ctrl Pts',(-3.30300595568341,-1.,-1.90773912171424));
#65448=CARTESIAN_POINT('Ctrl Pts',(-3.30300595568341,1.,-1.90773912171424));
#65449=CARTESIAN_POINT('Ctrl Pts',(-3.30975721158694,-1.,-1.91014297830502));
#65450=CARTESIAN_POINT('Ctrl Pts',(-3.30975721158694,1.,-1.91014297830502));
#65451=CARTESIAN_POINT('Ctrl Pts',(-3.31646052426395,-1.,-1.91242616234459));
#65452=CARTESIAN_POINT('Ctrl Pts',(-3.31646052426395,1.,-1.91242616234459));
#65453=CARTESIAN_POINT('Ctrl Pts',(-3.32323403454507,-1.,-1.91466343916612));
#65454=CARTESIAN_POINT('Ctrl Pts',(-3.32323403454507,1.,-1.91466343916612));
#65455=CARTESIAN_POINT('Ctrl Pts',(-3.33014884257812,-1.,-1.91690081930297));
#65456=CARTESIAN_POINT('Ctrl Pts',(-3.33014884257812,1.,-1.91690081930297));
#65457=CARTESIAN_POINT('Ctrl Pts',(-3.33721230709948,-1.,-1.91914609610173));
#65458=CARTESIAN_POINT('Ctrl Pts',(-3.33721230709948,1.,-1.91914609610173));
#65459=CARTESIAN_POINT('Ctrl Pts',(-3.34439448941915,-1.,-1.92138450828378));
#65460=CARTESIAN_POINT('Ctrl Pts',(-3.34439448941915,1.,-1.92138450828378));
#65461=CARTESIAN_POINT('Ctrl Pts',(-3.35164424847206,-1.,-1.92358838440518));
#65462=CARTESIAN_POINT('Ctrl Pts',(-3.35164424847206,1.,-1.92358838440518));
#65463=CARTESIAN_POINT('Ctrl Pts',(-3.35890824422976,-1.,-1.92572846125763));
#65464=CARTESIAN_POINT('Ctrl Pts',(-3.35890824422976,1.,-1.92572846125763));
#65465=CARTESIAN_POINT('Ctrl Pts',(-3.36615168657597,-1.,-1.92778626543803));
#65466=CARTESIAN_POINT('Ctrl Pts',(-3.36615168657597,1.,-1.92778626543803));
#65467=CARTESIAN_POINT('Ctrl Pts',(-3.37336807068078,-1.,-1.92975993109897));
#65468=CARTESIAN_POINT('Ctrl Pts',(-3.37336807068078,1.,-1.92975993109897));
#65469=CARTESIAN_POINT('Ctrl Pts',(-3.38056768525577,-1.,-1.93165739093292));
#65470=CARTESIAN_POINT('Ctrl Pts',(-3.38056768525577,1.,-1.93165739093292));
#65471=CARTESIAN_POINT('Ctrl Pts',(-3.38777076883267,-1.,-1.93349233176794));
#65472=CARTESIAN_POINT('Ctrl Pts',(-3.38777076883267,1.,-1.93349233176794));
#65473=CARTESIAN_POINT('Ctrl Pts',(-3.39499923640789,-1.,-1.93527929945982));
#65474=CARTESIAN_POINT('Ctrl Pts',(-3.39499923640789,1.,-1.93527929945982));
#65475=CARTESIAN_POINT('Ctrl Pts',(-3.40226802104093,-1.,-1.93702857723089));
#65476=CARTESIAN_POINT('Ctrl Pts',(-3.40226802104093,1.,-1.93702857723089));
#65477=CARTESIAN_POINT('Ctrl Pts',(-3.40957978266622,-1.,-1.93874306008132));
#65478=CARTESIAN_POINT('Ctrl Pts',(-3.40957978266622,1.,-1.93874306008132));
#65479=CARTESIAN_POINT('Ctrl Pts',(-3.41692971994082,-1.,-1.94042111965237));
#65480=CARTESIAN_POINT('Ctrl Pts',(-3.41692971994082,1.,-1.94042111965237));
#65481=CARTESIAN_POINT('Ctrl Pts',(-3.42430850941497,-1.,-1.94205835913692));
#65482=CARTESIAN_POINT('Ctrl Pts',(-3.42430850941497,1.,-1.94205835913692));
#65483=CARTESIAN_POINT('Ctrl Pts',(-3.43170586602436,-1.,-1.94364973660285));
#65484=CARTESIAN_POINT('Ctrl Pts',(-3.43170586602436,1.,-1.94364973660285));
#65485=CARTESIAN_POINT('Ctrl Pts',(-3.43911410197693,-1.,-1.94519168842883));
#65486=CARTESIAN_POINT('Ctrl Pts',(-3.43911410197693,1.,-1.94519168842883));
#65487=CARTESIAN_POINT('Ctrl Pts',(-3.44653088665685,-1.,-1.94668377715332));
#65488=CARTESIAN_POINT('Ctrl Pts',(-3.44653088665685,1.,-1.94668377715332));
#65489=CARTESIAN_POINT('Ctrl Pts',(-3.45395731584051,-1.,-1.94812754766524));
#65490=CARTESIAN_POINT('Ctrl Pts',(-3.45395731584051,1.,-1.94812754766524));
#65491=CARTESIAN_POINT('Ctrl Pts',(-3.46139661060959,-1.,-1.94952575850196));
#65492=CARTESIAN_POINT('Ctrl Pts',(-3.46139661060959,1.,-1.94952575850196));
#65493=CARTESIAN_POINT('Ctrl Pts',(-3.4688525897419,-1.,-1.95088147859876));
#65494=CARTESIAN_POINT('Ctrl Pts',(-3.4688525897419,1.,-1.95088147859876));
#65495=CARTESIAN_POINT('Ctrl Pts',(-3.47632820495926,-1.,-1.95219722189878));
#65496=CARTESIAN_POINT('Ctrl Pts',(-3.47632820495926,1.,-1.95219722189878));
#65497=CARTESIAN_POINT('Ctrl Pts',(-3.48382414832648,-1.,-1.95347412486316));
#65498=CARTESIAN_POINT('Ctrl Pts',(-3.48382414832648,1.,-1.95347412486316));
#65499=CARTESIAN_POINT('Ctrl Pts',(-3.49133956289154,-1.,-1.95471236969653));
#65500=CARTESIAN_POINT('Ctrl Pts',(-3.49133956289154,1.,-1.95471236969653));
#65501=CARTESIAN_POINT('Ctrl Pts',(-3.49887263575602,-1.,-1.9559115382367));
#65502=CARTESIAN_POINT('Ctrl Pts',(-3.49887263575602,1.,-1.9559115382367));
#65503=CARTESIAN_POINT('Ctrl Pts',(-3.50642124159913,-1.,-1.95707099606513));
#65504=CARTESIAN_POINT('Ctrl Pts',(-3.50642124159913,1.,-1.95707099606513));
#65505=CARTESIAN_POINT('Ctrl Pts',(-3.51398354617772,-1.,-1.95819025316768));
#65506=CARTESIAN_POINT('Ctrl Pts',(-3.51398354617772,1.,-1.95819025316768));
#65507=CARTESIAN_POINT('Ctrl Pts',(-3.52155867431438,-1.,-1.95926936324436));
#65508=CARTESIAN_POINT('Ctrl Pts',(-3.52155867431438,1.,-1.95926936324436));
#65509=CARTESIAN_POINT('Ctrl Pts',(-3.52914648844289,-1.,-1.96030879411534));
#65510=CARTESIAN_POINT('Ctrl Pts',(-3.52914648844289,1.,-1.96030879411534));
#65511=CARTESIAN_POINT('Ctrl Pts',(-3.53674730625759,-1.,-1.96130926212661));
#65512=CARTESIAN_POINT('Ctrl Pts',(-3.53674730625759,1.,-1.96130926212661));
#65513=CARTESIAN_POINT('Ctrl Pts',(-3.54436163300425,-1.,-1.96227157573058));
#65514=CARTESIAN_POINT('Ctrl Pts',(-3.54436163300425,1.,-1.96227157573058));
#65515=CARTESIAN_POINT('Ctrl Pts',(-3.55198990600929,-1.,-1.96319648628667));
#65516=CARTESIAN_POINT('Ctrl Pts',(-3.55198990600929,1.,-1.96319648628667));
#65517=CARTESIAN_POINT('Ctrl Pts',(-3.55963218706201,-1.,-1.96408450906868));
#65518=CARTESIAN_POINT('Ctrl Pts',(-3.55963218706201,1.,-1.96408450906868));
#65519=CARTESIAN_POINT('Ctrl Pts',(-3.56728820357933,-1.,-1.96493594634643));
#65520=CARTESIAN_POINT('Ctrl Pts',(-3.56728820357933,1.,-1.96493594634643));
#65521=CARTESIAN_POINT('Ctrl Pts',(-3.57495748601088,-1.,-1.96575096652857));
#65522=CARTESIAN_POINT('Ctrl Pts',(-3.57495748601088,1.,-1.96575096652857));
#65523=CARTESIAN_POINT('Ctrl Pts',(-3.58263947663884,-1.,-1.9665296668894));
#65524=CARTESIAN_POINT('Ctrl Pts',(-3.58263947663884,1.,-1.9665296668894));
#65525=CARTESIAN_POINT('Ctrl Pts',(-3.5903336402273,-1.,-1.96727213799507));
#65526=CARTESIAN_POINT('Ctrl Pts',(-3.5903336402273,1.,-1.96727213799507));
#65527=CARTESIAN_POINT('Ctrl Pts',(-3.59803959819725,-1.,-1.96797854118257));
#65528=CARTESIAN_POINT('Ctrl Pts',(-3.59803959819725,1.,-1.96797854118257));
#65529=CARTESIAN_POINT('Ctrl Pts',(-3.60575714017676,-1.,-1.96864911885775));
#65530=CARTESIAN_POINT('Ctrl Pts',(-3.60575714017676,1.,-1.96864911885775));
#65531=CARTESIAN_POINT('Ctrl Pts',(-3.61348615496393,-1.,-1.96928416040712));
#65532=CARTESIAN_POINT('Ctrl Pts',(-3.61348615496393,1.,-1.96928416040712));
#65533=CARTESIAN_POINT('Ctrl Pts',(-3.62122658401722,-1.,-1.96988398129888));
#65534=CARTESIAN_POINT('Ctrl Pts',(-3.62122658401722,1.,-1.96988398129888));
#65535=CARTESIAN_POINT('Ctrl Pts',(-3.62897836973397,-1.,-1.97044889850518));
#65536=CARTESIAN_POINT('Ctrl Pts',(-3.62897836973397,1.,-1.97044889850518));
#65537=CARTESIAN_POINT('Ctrl Pts',(-3.63674139590853,-1.,-1.97097920454698));
#65538=CARTESIAN_POINT('Ctrl Pts',(-3.63674139590853,1.,-1.97097920454698));
#65539=CARTESIAN_POINT('Ctrl Pts',(-3.64451546724221,-1.,-1.97147515441539));
#65540=CARTESIAN_POINT('Ctrl Pts',(-3.64451546724221,1.,-1.97147515441539));
#65541=CARTESIAN_POINT('Ctrl Pts',(-3.65230034717364,-1.,-1.97193697240645));
#65542=CARTESIAN_POINT('Ctrl Pts',(-3.65230034717364,1.,-1.97193697240645));
#65543=CARTESIAN_POINT('Ctrl Pts',(-3.66009578166865,-1.,-1.97236485439317));
#65544=CARTESIAN_POINT('Ctrl Pts',(-3.66009578166865,1.,-1.97236485439317));
#65545=CARTESIAN_POINT('Ctrl Pts',(-3.66790152751984,-1.,-1.9727589719863));
#65546=CARTESIAN_POINT('Ctrl Pts',(-3.66790152751984,1.,-1.9727589719863));
#65547=CARTESIAN_POINT('Ctrl Pts',(-3.67571738106175,-1.,-1.97311947678035));
#65548=CARTESIAN_POINT('Ctrl Pts',(-3.67571738106175,1.,-1.97311947678035));
#65549=CARTESIAN_POINT('Ctrl Pts',(-3.68354319913416,-1.,-1.9734465030363));
#65550=CARTESIAN_POINT('Ctrl Pts',(-3.68354319913416,1.,-1.9734465030363));
#65551=CARTESIAN_POINT('Ctrl Pts',(-3.69137888597855,-1.,-1.97374016224397));
#65552=CARTESIAN_POINT('Ctrl Pts',(-3.69137888597855,1.,-1.97374016224397));
#65553=CARTESIAN_POINT('Ctrl Pts',(-3.69765528558292,-1.,-1.97394846382288));
#65554=CARTESIAN_POINT('Ctrl Pts',(-3.69765528558292,1.,-1.97394846382288));
#65555=CARTESIAN_POINT('Ctrl Pts',(-3.70236698911837,-1.,-1.97408973726149));
#65556=CARTESIAN_POINT('Ctrl Pts',(-3.70236698911837,1.,-1.97408973726149));
#65557=CARTESIAN_POINT('Ctrl Pts',(-3.7055100813194,-1.,-1.974177276451));
#65558=CARTESIAN_POINT('Ctrl Pts',(-3.7055100813194,1.,-1.974177276451));
#65559=CARTESIAN_POINT('Ctrl Pts',(-3.70708211654725,-1.,-1.97421938526992));
#65560=CARTESIAN_POINT('Ctrl Pts',(-3.70708211654725,1.,-1.97421938526992));
#65561=CARTESIAN_POINT('',(-3.24413672884902,1.,-1.88097764062542));
#65562=CARTESIAN_POINT('Ctrl Pts',(-3.24413672884902,-1.,-1.88097764062542));
#65563=CARTESIAN_POINT('Ctrl Pts',(-3.24413672884902,-0.666666666666667,
-1.88097764062542));
#65564=CARTESIAN_POINT('Ctrl Pts',(-3.24413672884902,-0.333333333333333,
-1.88097764062542));
#65565=CARTESIAN_POINT('Ctrl Pts',(-3.24413672884902,0.333333333333333,
-1.88097764062542));
#65566=CARTESIAN_POINT('Ctrl Pts',(-3.24413672884902,0.666666666666667,
-1.88097764062542));
#65567=CARTESIAN_POINT('Ctrl Pts',(-3.24413672884902,1.,-1.88097764062542));
#65568=CARTESIAN_POINT('',(-3.70708211654725,1.,-1.97421938526992));
#65569=CARTESIAN_POINT('',(-3.70708211654725,0.,-1.97421938526992));
#65570=CARTESIAN_POINT('Ctrl Pts',(-3.24413672884902,1.,-1.88097764062542));
#65571=CARTESIAN_POINT('Ctrl Pts',(-3.24415531671311,1.,-1.88102292397987));
#65572=CARTESIAN_POINT('Ctrl Pts',(-3.24428080352952,1.,-1.88117508446657));
#65573=CARTESIAN_POINT('Ctrl Pts',(-3.24480754675942,1.,-1.88156537699118));
#65574=CARTESIAN_POINT('Ctrl Pts',(-3.24625654410705,1.,-1.88242596600422));
#65575=CARTESIAN_POINT('Ctrl Pts',(-3.24935200512055,1.,-1.88407708646435));
#65576=CARTESIAN_POINT('Ctrl Pts',(-3.25408686339298,1.,-1.88646802523372));
#65577=CARTESIAN_POINT('Ctrl Pts',(-3.2599988519361,1.,-1.88934996203508));
#65578=CARTESIAN_POINT('Ctrl Pts',(-3.2667765388833,1.,-1.89255393500769));
#65579=CARTESIAN_POINT('Ctrl Pts',(-3.27407108932908,1.,-1.89589172903662));
#65580=CARTESIAN_POINT('Ctrl Pts',(-3.28154737912287,1.,-1.89918429230424));
#65581=CARTESIAN_POINT('Ctrl Pts',(-3.28893448600364,1.,-1.9022897124757));
#65582=CARTESIAN_POINT('Ctrl Pts',(-3.29608978722258,1.,-1.9051389186417));
#65583=CARTESIAN_POINT('Ctrl Pts',(-3.30300595568341,1.,-1.90773912171424));
#65584=CARTESIAN_POINT('Ctrl Pts',(-3.30975721158694,1.,-1.91014297830502));
#65585=CARTESIAN_POINT('Ctrl Pts',(-3.31646052426395,1.,-1.91242616234459));
#65586=CARTESIAN_POINT('Ctrl Pts',(-3.32323403454507,1.,-1.91466343916612));
#65587=CARTESIAN_POINT('Ctrl Pts',(-3.33014884257812,1.,-1.91690081930297));
#65588=CARTESIAN_POINT('Ctrl Pts',(-3.33721230709948,1.,-1.91914609610173));
#65589=CARTESIAN_POINT('Ctrl Pts',(-3.34439448941915,1.,-1.92138450828378));
#65590=CARTESIAN_POINT('Ctrl Pts',(-3.35164424847206,1.,-1.92358838440518));
#65591=CARTESIAN_POINT('Ctrl Pts',(-3.35890824422976,1.,-1.92572846125763));
#65592=CARTESIAN_POINT('Ctrl Pts',(-3.36615168657597,1.,-1.92778626543803));
#65593=CARTESIAN_POINT('Ctrl Pts',(-3.37336807068078,1.,-1.92975993109897));
#65594=CARTESIAN_POINT('Ctrl Pts',(-3.38056768525577,1.,-1.93165739093292));
#65595=CARTESIAN_POINT('Ctrl Pts',(-3.38777076883267,1.,-1.93349233176794));
#65596=CARTESIAN_POINT('Ctrl Pts',(-3.39499923640789,1.,-1.93527929945982));
#65597=CARTESIAN_POINT('Ctrl Pts',(-3.40226802104093,1.,-1.93702857723089));
#65598=CARTESIAN_POINT('Ctrl Pts',(-3.40957978266622,1.,-1.93874306008132));
#65599=CARTESIAN_POINT('Ctrl Pts',(-3.41692971994082,1.,-1.94042111965237));
#65600=CARTESIAN_POINT('Ctrl Pts',(-3.42430850941497,1.,-1.94205835913692));
#65601=CARTESIAN_POINT('Ctrl Pts',(-3.43170586602436,1.,-1.94364973660285));
#65602=CARTESIAN_POINT('Ctrl Pts',(-3.43911410197693,1.,-1.94519168842883));
#65603=CARTESIAN_POINT('Ctrl Pts',(-3.44653088665685,1.,-1.94668377715332));
#65604=CARTESIAN_POINT('Ctrl Pts',(-3.45395731584051,1.,-1.94812754766524));
#65605=CARTESIAN_POINT('Ctrl Pts',(-3.46139661060959,1.,-1.94952575850196));
#65606=CARTESIAN_POINT('Ctrl Pts',(-3.4688525897419,1.,-1.95088147859876));
#65607=CARTESIAN_POINT('Ctrl Pts',(-3.47632820495926,1.,-1.95219722189878));
#65608=CARTESIAN_POINT('Ctrl Pts',(-3.48382414832648,1.,-1.95347412486316));
#65609=CARTESIAN_POINT('Ctrl Pts',(-3.49133956289154,1.,-1.95471236969653));
#65610=CARTESIAN_POINT('Ctrl Pts',(-3.49887263575602,1.,-1.9559115382367));
#65611=CARTESIAN_POINT('Ctrl Pts',(-3.50642124159913,1.,-1.95707099606513));
#65612=CARTESIAN_POINT('Ctrl Pts',(-3.51398354617772,1.,-1.95819025316768));
#65613=CARTESIAN_POINT('Ctrl Pts',(-3.52155867431438,1.,-1.95926936324436));
#65614=CARTESIAN_POINT('Ctrl Pts',(-3.52914648844289,1.,-1.96030879411534));
#65615=CARTESIAN_POINT('Ctrl Pts',(-3.53674730625759,1.,-1.96130926212661));
#65616=CARTESIAN_POINT('Ctrl Pts',(-3.54436163300425,1.,-1.96227157573058));
#65617=CARTESIAN_POINT('Ctrl Pts',(-3.55198990600929,1.,-1.96319648628667));
#65618=CARTESIAN_POINT('Ctrl Pts',(-3.55963218706201,1.,-1.96408450906868));
#65619=CARTESIAN_POINT('Ctrl Pts',(-3.56728820357933,1.,-1.96493594634643));
#65620=CARTESIAN_POINT('Ctrl Pts',(-3.57495748601088,1.,-1.96575096652857));
#65621=CARTESIAN_POINT('Ctrl Pts',(-3.58263947663884,1.,-1.9665296668894));
#65622=CARTESIAN_POINT('Ctrl Pts',(-3.5903336402273,1.,-1.96727213799507));
#65623=CARTESIAN_POINT('Ctrl Pts',(-3.59803959819725,1.,-1.96797854118257));
#65624=CARTESIAN_POINT('Ctrl Pts',(-3.60575714017676,1.,-1.96864911885775));
#65625=CARTESIAN_POINT('Ctrl Pts',(-3.61348615496393,1.,-1.96928416040712));
#65626=CARTESIAN_POINT('Ctrl Pts',(-3.62122658401722,1.,-1.96988398129888));
#65627=CARTESIAN_POINT('Ctrl Pts',(-3.62897836973397,1.,-1.97044889850518));
#65628=CARTESIAN_POINT('Ctrl Pts',(-3.63674139590853,1.,-1.97097920454698));
#65629=CARTESIAN_POINT('Ctrl Pts',(-3.64451546724221,1.,-1.97147515441539));
#65630=CARTESIAN_POINT('Ctrl Pts',(-3.65230034717364,1.,-1.97193697240645));
#65631=CARTESIAN_POINT('Ctrl Pts',(-3.66009578166865,1.,-1.97236485439317));
#65632=CARTESIAN_POINT('Ctrl Pts',(-3.66790152751984,1.,-1.9727589719863));
#65633=CARTESIAN_POINT('Ctrl Pts',(-3.67571738106175,1.,-1.97311947678035));
#65634=CARTESIAN_POINT('Ctrl Pts',(-3.68354319913416,1.,-1.9734465030363));
#65635=CARTESIAN_POINT('Ctrl Pts',(-3.69137888597855,1.,-1.97374016224397));
#65636=CARTESIAN_POINT('Ctrl Pts',(-3.69765528558292,1.,-1.97394846382288));
#65637=CARTESIAN_POINT('Ctrl Pts',(-3.70236698911837,1.,-1.97408973726149));
#65638=CARTESIAN_POINT('Ctrl Pts',(-3.7055100813194,1.,-1.974177276451));
#65639=CARTESIAN_POINT('Ctrl Pts',(-3.70708211654725,1.,-1.97421938526992));
#65640=CARTESIAN_POINT('Origin',(-3.70708211654725,0.,-1.97421938526992));
#65641=CARTESIAN_POINT('',(-3.77614523045147,1.,-1.83867539237861));
#65642=CARTESIAN_POINT('Origin',(0.,0.,0.));
#65643=CARTESIAN_POINT('',(-3.14877060440425,1.,-2.03660101169564));
#65644=CARTESIAN_POINT('Origin',(0.,1.,0.));
#65645=CARTESIAN_POINT('Ctrl Pts',(-3.14877060440425,1.,-2.03660101169564));
#65646=CARTESIAN_POINT('Ctrl Pts',(-3.14877060440425,0.666666666666667,
-2.03660101169564));
#65647=CARTESIAN_POINT('Ctrl Pts',(-3.14877060440425,0.333333333333333,
-2.03660101169564));
#65648=CARTESIAN_POINT('Ctrl Pts',(-3.14877060440425,-0.333333333333333,
-2.03660101169564));
#65649=CARTESIAN_POINT('Ctrl Pts',(-3.14877060440425,-0.666666666666667,
-2.03660101169564));
#65650=CARTESIAN_POINT('Ctrl Pts',(-3.14877060440425,-1.,-2.03660101169564));
#65651=CARTESIAN_POINT('Ctrl Pts',(-3.44202241512147,-1.,-2.40675750623143));
#65652=CARTESIAN_POINT('Ctrl Pts',(-3.44202241512147,1.,-2.40675750623143));
#65653=CARTESIAN_POINT('Ctrl Pts',(-3.44127120683402,-1.,-2.40537592959345));
#65654=CARTESIAN_POINT('Ctrl Pts',(-3.44127120683402,1.,-2.40537592959345));
#65655=CARTESIAN_POINT('Ctrl Pts',(-3.43976627485223,-1.,-2.40261515590099));
#65656=CARTESIAN_POINT('Ctrl Pts',(-3.43976627485223,1.,-2.40261515590099));
#65657=CARTESIAN_POINT('Ctrl Pts',(-3.43750133066036,-1.,-2.39848113411429));
#65658=CARTESIAN_POINT('Ctrl Pts',(-3.43750133066036,1.,-2.39848113411429));
#65659=CARTESIAN_POINT('Ctrl Pts',(-3.43446630680436,-1.,-2.39298338805823));
#65660=CARTESIAN_POINT('Ctrl Pts',(-3.43446630680436,1.,-2.39298338805823));
#65661=CARTESIAN_POINT('Ctrl Pts',(-3.43064732714472,-1.,-2.38613505844641));
#65662=CARTESIAN_POINT('Ctrl Pts',(-3.43064732714472,1.,-2.38613505844641));
#65663=CARTESIAN_POINT('Ctrl Pts',(-3.42680309755241,-1.,-2.37931067029517));
#65664=CARTESIAN_POINT('Ctrl Pts',(-3.42680309755241,1.,-2.37931067029517));
#65665=CARTESIAN_POINT('Ctrl Pts',(-3.42293356216595,-1.,-2.37251035954351));
#65666=CARTESIAN_POINT('Ctrl Pts',(-3.42293356216595,1.,-2.37251035954351));
#65667=CARTESIAN_POINT('Ctrl Pts',(-3.41903866635384,-1.,-2.36573431470314));
#65668=CARTESIAN_POINT('Ctrl Pts',(-3.41903866635384,1.,-2.36573431470314));
#65669=CARTESIAN_POINT('Ctrl Pts',(-3.4151183675076,-1.,-2.35898278606449));
#65670=CARTESIAN_POINT('Ctrl Pts',(-3.4151183675076,1.,-2.35898278606449));
#65671=CARTESIAN_POINT('Ctrl Pts',(-3.41117262313464,-1.,-2.35225606823649));
#65672=CARTESIAN_POINT('Ctrl Pts',(-3.41117262313464,1.,-2.35225606823649));
#65673=CARTESIAN_POINT('Ctrl Pts',(-3.40720137403888,-1.,-2.34555447648901));
#65674=CARTESIAN_POINT('Ctrl Pts',(-3.40720137403888,1.,-2.34555447648901));
#65675=CARTESIAN_POINT('Ctrl Pts',(-3.40320452776646,-1.,-2.33887832342715));
#65676=CARTESIAN_POINT('Ctrl Pts',(-3.40320452776646,1.,-2.33887832342715));
#65677=CARTESIAN_POINT('Ctrl Pts',(-3.39918194578115,-1.,-2.33222789882601));
#65678=CARTESIAN_POINT('Ctrl Pts',(-3.39918194578115,1.,-2.33222789882601));
#65679=CARTESIAN_POINT('Ctrl Pts',(-3.39513342020045,-1.,-2.32560343902683));
#65680=CARTESIAN_POINT('Ctrl Pts',(-3.39513342020045,1.,-2.32560343902683));
#65681=CARTESIAN_POINT('Ctrl Pts',(-3.39105869475112,-1.,-2.31900513925627));
#65682=CARTESIAN_POINT('Ctrl Pts',(-3.39105869475112,1.,-2.31900513925627));
#65683=CARTESIAN_POINT('Ctrl Pts',(-3.38695751492659,-1.,-2.31243319489505));
#65684=CARTESIAN_POINT('Ctrl Pts',(-3.38695751492659,1.,-2.31243319489505));
#65685=CARTESIAN_POINT('Ctrl Pts',(-3.38282967336676,-1.,-2.30588783640389));
#65686=CARTESIAN_POINT('Ctrl Pts',(-3.38282967336676,1.,-2.30588783640389));
#65687=CARTESIAN_POINT('Ctrl Pts',(-3.37867504959382,-1.,-2.29936936127588));
#65688=CARTESIAN_POINT('Ctrl Pts',(-3.37867504959382,1.,-2.29936936127588));
#65689=CARTESIAN_POINT('Ctrl Pts',(-3.37449367172707,-1.,-2.2928781800731));
#65690=CARTESIAN_POINT('Ctrl Pts',(-3.37449367172707,1.,-2.2928781800731));
#65691=CARTESIAN_POINT('Ctrl Pts',(-3.37028570206357,-1.,-2.28641481081045));
#65692=CARTESIAN_POINT('Ctrl Pts',(-3.37028570206357,1.,-2.28641481081045));
#65693=CARTESIAN_POINT('Ctrl Pts',(-3.36605130712978,-1.,-2.27997979457968));
#65694=CARTESIAN_POINT('Ctrl Pts',(-3.36605130712978,1.,-2.27997979457968));
#65695=CARTESIAN_POINT('Ctrl Pts',(-3.36179055004369,-1.,-2.27357362620902));
#65696=CARTESIAN_POINT('Ctrl Pts',(-3.36179055004369,1.,-2.27357362620902));
#65697=CARTESIAN_POINT('Ctrl Pts',(-3.35750328523077,-1.,-2.26719668579921));
#65698=CARTESIAN_POINT('Ctrl Pts',(-3.35750328523077,1.,-2.26719668579921));
#65699=CARTESIAN_POINT('Ctrl Pts',(-3.35318902552676,-1.,-2.26084915222484));
#65700=CARTESIAN_POINT('Ctrl Pts',(-3.35318902552676,1.,-2.26084915222484));
#65701=CARTESIAN_POINT('Ctrl Pts',(-3.34884690292342,-1.,-2.25453097693524));
#65702=CARTESIAN_POINT('Ctrl Pts',(-3.34884690292342,1.,-2.25453097693524));
#65703=CARTESIAN_POINT('Ctrl Pts',(-3.34447596770768,-1.,-2.24824207678288));
#65704=CARTESIAN_POINT('Ctrl Pts',(-3.34447596770768,1.,-2.24824207678288));
#65705=CARTESIAN_POINT('Ctrl Pts',(-3.34007543738044,-1.,-2.24198249391437));
#65706=CARTESIAN_POINT('Ctrl Pts',(-3.34007543738044,1.,-2.24198249391437));
#65707=CARTESIAN_POINT('Ctrl Pts',(-3.33564495756478,-1.,-2.2357525632881));
#65708=CARTESIAN_POINT('Ctrl Pts',(-3.33564495756478,1.,-2.2357525632881));
#65709=CARTESIAN_POINT('Ctrl Pts',(-3.33118487773593,-1.,-2.22955308907221));
#65710=CARTESIAN_POINT('Ctrl Pts',(-3.33118487773593,1.,-2.22955308907221));
#65711=CARTESIAN_POINT('Ctrl Pts',(-3.32669646722871,-1.,-2.22338548312758));
#65712=CARTESIAN_POINT('Ctrl Pts',(-3.32669646722871,1.,-2.22338548312758));
#65713=CARTESIAN_POINT('Ctrl Pts',(-3.32218125618955,-1.,-2.21725135110889));
#65714=CARTESIAN_POINT('Ctrl Pts',(-3.32218125618955,1.,-2.21725135110889));
#65715=CARTESIAN_POINT('Ctrl Pts',(-3.31764044024231,-1.,-2.21115211847872));
#65716=CARTESIAN_POINT('Ctrl Pts',(-3.31764044024231,1.,-2.21115211847872));
#65717=CARTESIAN_POINT('Ctrl Pts',(-3.3130742460895,-1.,-2.20508863150608));
#65718=CARTESIAN_POINT('Ctrl Pts',(-3.3130742460895,1.,-2.20508863150608));
#65719=CARTESIAN_POINT('Ctrl Pts',(-3.30848134694596,-1.,-2.19906078949924));
#65720=CARTESIAN_POINT('Ctrl Pts',(-3.30848134694596,1.,-2.19906078949924));
#65721=CARTESIAN_POINT('Ctrl Pts',(-3.30385816281831,-1.,-2.19306710376112));
#65722=CARTESIAN_POINT('Ctrl Pts',(-3.30385816281831,1.,-2.19306710376112));
#65723=CARTESIAN_POINT('Ctrl Pts',(-3.29920022557635,-1.,-2.18710556500325));
#65724=CARTESIAN_POINT('Ctrl Pts',(-3.29920022557635,1.,-2.18710556500325));
#65725=CARTESIAN_POINT('Ctrl Pts',(-3.29450361500484,-1.,-2.18117455557062));
#65726=CARTESIAN_POINT('Ctrl Pts',(-3.29450361500484,1.,-2.18117455557062));
#65727=CARTESIAN_POINT('Ctrl Pts',(-3.28976645712566,-1.,-2.17527380048422));
#65728=CARTESIAN_POINT('Ctrl Pts',(-3.28976645712566,1.,-2.17527380048422));
#65729=CARTESIAN_POINT('Ctrl Pts',(-3.2849901997973,-1.,-2.16940517773459));
#65730=CARTESIAN_POINT('Ctrl Pts',(-3.2849901997973,1.,-2.16940517773459));
#65731=CARTESIAN_POINT('Ctrl Pts',(-3.28018150841414,-1.,-2.16357391934434));
#65732=CARTESIAN_POINT('Ctrl Pts',(-3.28018150841414,1.,-2.16357391934434));
#65733=CARTESIAN_POINT('Ctrl Pts',(-3.27534954469206,-1.,-2.15778690038359));
#65734=CARTESIAN_POINT('Ctrl Pts',(-3.27534954469206,1.,-2.15778690038359));
#65735=CARTESIAN_POINT('Ctrl Pts',(-3.27050245897244,-1.,-2.15205043199818));
#65736=CARTESIAN_POINT('Ctrl Pts',(-3.27050245897244,1.,-2.15205043199818));
#65737=CARTESIAN_POINT('Ctrl Pts',(-3.26564388189764,-1.,-2.14636805295663));
#65738=CARTESIAN_POINT('Ctrl Pts',(-3.26564388189764,1.,-2.14636805295663));
#65739=CARTESIAN_POINT('Ctrl Pts',(-3.26077002641868,-1.,-2.14073870754257));
#65740=CARTESIAN_POINT('Ctrl Pts',(-3.26077002641868,1.,-2.14073870754257));
#65741=CARTESIAN_POINT('Ctrl Pts',(-3.25586495065027,-1.,-2.13515375878786));
#65742=CARTESIAN_POINT('Ctrl Pts',(-3.25586495065027,1.,-2.13515375878786));
#65743=CARTESIAN_POINT('Ctrl Pts',(-3.25090574493994,-1.,-2.1296002839681));
#65744=CARTESIAN_POINT('Ctrl Pts',(-3.25090574493994,1.,-2.1296002839681));
#65745=CARTESIAN_POINT('Ctrl Pts',(-3.24587102613347,-1.,-2.12406646410943));
#65746=CARTESIAN_POINT('Ctrl Pts',(-3.24587102613347,1.,-2.12406646410943));
#65747=CARTESIAN_POINT('Ctrl Pts',(-3.24074905517282,-1.,-2.11854673326972));
#65748=CARTESIAN_POINT('Ctrl Pts',(-3.24074905517282,1.,-2.11854673326972));
#65749=CARTESIAN_POINT('Ctrl Pts',(-3.23554444767115,-1.,-2.11304604021784));
#65750=CARTESIAN_POINT('Ctrl Pts',(-3.23554444767115,1.,-2.11304604021784));
#65751=CARTESIAN_POINT('Ctrl Pts',(-3.23028945793334,-1.,-2.1075869964248));
#65752=CARTESIAN_POINT('Ctrl Pts',(-3.23028945793334,1.,-2.1075869964248));
#65753=CARTESIAN_POINT('Ctrl Pts',(-3.22503437553496,-1.,-2.10220384298533));
#65754=CARTESIAN_POINT('Ctrl Pts',(-3.22503437553496,1.,-2.10220384298533));
#65755=CARTESIAN_POINT('Ctrl Pts',(-3.21982707347067,-1.,-2.09692958434933));
#65756=CARTESIAN_POINT('Ctrl Pts',(-3.21982707347067,1.,-2.09692958434933));
#65757=CARTESIAN_POINT('Ctrl Pts',(-3.2146942960168,-1.,-2.0917841946046));
#65758=CARTESIAN_POINT('Ctrl Pts',(-3.2146942960168,1.,-2.0917841946046));
#65759=CARTESIAN_POINT('Ctrl Pts',(-3.20962575845433,-1.,-2.08676465517435));
#65760=CARTESIAN_POINT('Ctrl Pts',(-3.20962575845433,1.,-2.08676465517435));
#65761=CARTESIAN_POINT('Ctrl Pts',(-3.20454818630635,-1.,-2.08182850370816));
#65762=CARTESIAN_POINT('Ctrl Pts',(-3.20454818630635,1.,-2.08182850370816));
#65763=CARTESIAN_POINT('Ctrl Pts',(-3.19934132835879,-1.,-2.0769044187063));
#65764=CARTESIAN_POINT('Ctrl Pts',(-3.19934132835879,1.,-2.0769044187063));
#65765=CARTESIAN_POINT('Ctrl Pts',(-3.19388465568113,-1.,-2.07192253497765));
#65766=CARTESIAN_POINT('Ctrl Pts',(-3.19388465568113,1.,-2.07192253497765));
#65767=CARTESIAN_POINT('Ctrl Pts',(-3.18809755562297,-1.,-2.06684062744065));
#65768=CARTESIAN_POINT('Ctrl Pts',(-3.18809755562297,1.,-2.06684062744065));
#65769=CARTESIAN_POINT('Ctrl Pts',(-3.18197692964677,-1.,-2.06166849827143));
#65770=CARTESIAN_POINT('Ctrl Pts',(-3.18197692964677,1.,-2.06166849827143));
#65771=CARTESIAN_POINT('Ctrl Pts',(-3.17564906975592,-1.,-2.05650186773279));
#65772=CARTESIAN_POINT('Ctrl Pts',(-3.17564906975592,1.,-2.05650186773279));
#65773=CARTESIAN_POINT('Ctrl Pts',(-3.16936341689859,-1.,-2.05151770247452));
#65774=CARTESIAN_POINT('Ctrl Pts',(-3.16936341689859,1.,-2.05151770247452));
#65775=CARTESIAN_POINT('Ctrl Pts',(-3.16343165059235,-1.,-2.0469333124766));
#65776=CARTESIAN_POINT('Ctrl Pts',(-3.16343165059235,1.,-2.0469333124766));
#65777=CARTESIAN_POINT('Ctrl Pts',(-3.15817983946525,-1.,-2.04297406404132));
#65778=CARTESIAN_POINT('Ctrl Pts',(-3.15817983946525,1.,-2.04297406404132));
#65779=CARTESIAN_POINT('Ctrl Pts',(-3.1538999167466,-1.,-2.03984073791432));
#65780=CARTESIAN_POINT('Ctrl Pts',(-3.1538999167466,1.,-2.03984073791432));
#65781=CARTESIAN_POINT('Ctrl Pts',(-3.15079010635326,-1.,-2.03766932526171));
#65782=CARTESIAN_POINT('Ctrl Pts',(-3.15079010635326,1.,-2.03766932526171));
#65783=CARTESIAN_POINT('Ctrl Pts',(-3.14931281967585,-1.,-2.03675273048882));
#65784=CARTESIAN_POINT('Ctrl Pts',(-3.14931281967585,1.,-2.03675273048882));
#65785=CARTESIAN_POINT('Ctrl Pts',(-3.14878756590499,-1.,-2.03653654935384));
#65786=CARTESIAN_POINT('Ctrl Pts',(-3.14878756590499,1.,-2.03653654935384));
#65787=CARTESIAN_POINT('Ctrl Pts',(-3.14869618937138,-1.,-2.036601737578));
#65788=CARTESIAN_POINT('Ctrl Pts',(-3.14869618937138,1.,-2.036601737578));
#65789=CARTESIAN_POINT('Ctrl Pts',(-3.1487152044751,-1.,-2.03668666247593));
#65790=CARTESIAN_POINT('Ctrl Pts',(-3.1487152044751,1.,-2.03668666247593));
#65791=CARTESIAN_POINT('',(-3.44202241512147,1.,-2.40675750623143));
#65792=CARTESIAN_POINT('Ctrl Pts',(-3.44202241512147,1.,-2.40675750623143));
#65793=CARTESIAN_POINT('Ctrl Pts',(-3.44127120683402,1.,-2.40537592959345));
#65794=CARTESIAN_POINT('Ctrl Pts',(-3.43976627485223,1.,-2.40261515590099));
#65795=CARTESIAN_POINT('Ctrl Pts',(-3.43750133066036,1.,-2.39848113411429));
#65796=CARTESIAN_POINT('Ctrl Pts',(-3.43446630680436,1.,-2.39298338805823));
#65797=CARTESIAN_POINT('Ctrl Pts',(-3.43064732714472,1.,-2.38613505844641));
#65798=CARTESIAN_POINT('Ctrl Pts',(-3.42680309755241,1.,-2.37931067029517));
#65799=CARTESIAN_POINT('Ctrl Pts',(-3.42293356216595,1.,-2.37251035954351));
#65800=CARTESIAN_POINT('Ctrl Pts',(-3.41903866635384,1.,-2.36573431470314));
#65801=CARTESIAN_POINT('Ctrl Pts',(-3.4151183675076,1.,-2.35898278606449));
#65802=CARTESIAN_POINT('Ctrl Pts',(-3.41117262313464,1.,-2.35225606823649));
#65803=CARTESIAN_POINT('Ctrl Pts',(-3.40720137403888,1.,-2.34555447648901));
#65804=CARTESIAN_POINT('Ctrl Pts',(-3.40320452776646,1.,-2.33887832342715));
#65805=CARTESIAN_POINT('Ctrl Pts',(-3.39918194578115,1.,-2.33222789882601));
#65806=CARTESIAN_POINT('Ctrl Pts',(-3.39513342020045,1.,-2.32560343902683));
#65807=CARTESIAN_POINT('Ctrl Pts',(-3.39105869475112,1.,-2.31900513925627));
#65808=CARTESIAN_POINT('Ctrl Pts',(-3.38695751492659,1.,-2.31243319489505));
#65809=CARTESIAN_POINT('Ctrl Pts',(-3.38282967336676,1.,-2.30588783640389));
#65810=CARTESIAN_POINT('Ctrl Pts',(-3.37867504959382,1.,-2.29936936127588));
#65811=CARTESIAN_POINT('Ctrl Pts',(-3.37449367172707,1.,-2.2928781800731));
#65812=CARTESIAN_POINT('Ctrl Pts',(-3.37028570206357,1.,-2.28641481081045));
#65813=CARTESIAN_POINT('Ctrl Pts',(-3.36605130712978,1.,-2.27997979457968));
#65814=CARTESIAN_POINT('Ctrl Pts',(-3.36179055004369,1.,-2.27357362620902));
#65815=CARTESIAN_POINT('Ctrl Pts',(-3.35750328523077,1.,-2.26719668579921));
#65816=CARTESIAN_POINT('Ctrl Pts',(-3.35318902552676,1.,-2.26084915222484));
#65817=CARTESIAN_POINT('Ctrl Pts',(-3.34884690292342,1.,-2.25453097693524));
#65818=CARTESIAN_POINT('Ctrl Pts',(-3.34447596770768,1.,-2.24824207678288));
#65819=CARTESIAN_POINT('Ctrl Pts',(-3.34007543738044,1.,-2.24198249391437));
#65820=CARTESIAN_POINT('Ctrl Pts',(-3.33564495756478,1.,-2.2357525632881));
#65821=CARTESIAN_POINT('Ctrl Pts',(-3.33118487773593,1.,-2.22955308907221));
#65822=CARTESIAN_POINT('Ctrl Pts',(-3.32669646722871,1.,-2.22338548312758));
#65823=CARTESIAN_POINT('Ctrl Pts',(-3.32218125618955,1.,-2.21725135110889));
#65824=CARTESIAN_POINT('Ctrl Pts',(-3.31764044024231,1.,-2.21115211847872));
#65825=CARTESIAN_POINT('Ctrl Pts',(-3.3130742460895,1.,-2.20508863150608));
#65826=CARTESIAN_POINT('Ctrl Pts',(-3.30848134694596,1.,-2.19906078949924));
#65827=CARTESIAN_POINT('Ctrl Pts',(-3.30385816281831,1.,-2.19306710376112));
#65828=CARTESIAN_POINT('Ctrl Pts',(-3.29920022557635,1.,-2.18710556500325));
#65829=CARTESIAN_POINT('Ctrl Pts',(-3.29450361500484,1.,-2.18117455557062));
#65830=CARTESIAN_POINT('Ctrl Pts',(-3.28976645712566,1.,-2.17527380048422));
#65831=CARTESIAN_POINT('Ctrl Pts',(-3.2849901997973,1.,-2.16940517773459));
#65832=CARTESIAN_POINT('Ctrl Pts',(-3.28018150841414,1.,-2.16357391934434));
#65833=CARTESIAN_POINT('Ctrl Pts',(-3.27534954469206,1.,-2.15778690038359));
#65834=CARTESIAN_POINT('Ctrl Pts',(-3.27050245897244,1.,-2.15205043199818));
#65835=CARTESIAN_POINT('Ctrl Pts',(-3.26564388189764,1.,-2.14636805295663));
#65836=CARTESIAN_POINT('Ctrl Pts',(-3.26077002641868,1.,-2.14073870754257));
#65837=CARTESIAN_POINT('Ctrl Pts',(-3.25586495065027,1.,-2.13515375878786));
#65838=CARTESIAN_POINT('Ctrl Pts',(-3.25090574493994,1.,-2.1296002839681));
#65839=CARTESIAN_POINT('Ctrl Pts',(-3.24587102613347,1.,-2.12406646410943));
#65840=CARTESIAN_POINT('Ctrl Pts',(-3.24074905517282,1.,-2.11854673326972));
#65841=CARTESIAN_POINT('Ctrl Pts',(-3.23554444767115,1.,-2.11304604021784));
#65842=CARTESIAN_POINT('Ctrl Pts',(-3.23028945793334,1.,-2.1075869964248));
#65843=CARTESIAN_POINT('Ctrl Pts',(-3.22503437553496,1.,-2.10220384298533));
#65844=CARTESIAN_POINT('Ctrl Pts',(-3.21982707347067,1.,-2.09692958434933));
#65845=CARTESIAN_POINT('Ctrl Pts',(-3.2146942960168,1.,-2.0917841946046));
#65846=CARTESIAN_POINT('Ctrl Pts',(-3.20962575845433,1.,-2.08676465517435));
#65847=CARTESIAN_POINT('Ctrl Pts',(-3.20454818630635,1.,-2.08182850370816));
#65848=CARTESIAN_POINT('Ctrl Pts',(-3.19934132835879,1.,-2.0769044187063));
#65849=CARTESIAN_POINT('Ctrl Pts',(-3.19388465568113,1.,-2.07192253497765));
#65850=CARTESIAN_POINT('Ctrl Pts',(-3.18809755562297,1.,-2.06684062744065));
#65851=CARTESIAN_POINT('Ctrl Pts',(-3.18197692964677,1.,-2.06166849827143));
#65852=CARTESIAN_POINT('Ctrl Pts',(-3.17564906975592,1.,-2.05650186773279));
#65853=CARTESIAN_POINT('Ctrl Pts',(-3.16936341689859,1.,-2.05151770247452));
#65854=CARTESIAN_POINT('Ctrl Pts',(-3.16343165059235,1.,-2.0469333124766));
#65855=CARTESIAN_POINT('Ctrl Pts',(-3.15817983946525,1.,-2.04297406404132));
#65856=CARTESIAN_POINT('Ctrl Pts',(-3.1538999167466,1.,-2.03984073791432));
#65857=CARTESIAN_POINT('Ctrl Pts',(-3.15102344775396,1.,-2.03783225496023));
#65858=CARTESIAN_POINT('Ctrl Pts',(-3.14959882629936,1.,-2.03693188810614));
#65859=CARTESIAN_POINT('Ctrl Pts',(-3.14901193669147,1.,-2.03663974554941));
#65860=CARTESIAN_POINT('Ctrl Pts',(-3.1488193908823,1.,-2.03659701539175));
#65861=CARTESIAN_POINT('Ctrl Pts',(-3.14877060440425,1.,-2.03660101169564));
#65862=CARTESIAN_POINT('',(-3.44202241512147,0.,-2.40675750623143));
#65863=CARTESIAN_POINT('Ctrl Pts',(-2.91001063062876,-1.,-2.36523532225181));
#65864=CARTESIAN_POINT('Ctrl Pts',(-2.91001063062876,1.,-2.36523532225181));
#65865=CARTESIAN_POINT('Ctrl Pts',(-2.90992398626211,-1.,-2.36524348105112));
#65866=CARTESIAN_POINT('Ctrl Pts',(-2.90992398626211,1.,-2.36524348105112));
#65867=CARTESIAN_POINT('Ctrl Pts',(-2.90989022548032,-1.,-2.36535052956938));
#65868=CARTESIAN_POINT('Ctrl Pts',(-2.90989022548032,1.,-2.36535052956938));
#65869=CARTESIAN_POINT('Ctrl Pts',(-2.91025813830041,-1.,-2.36578327194741));
#65870=CARTESIAN_POINT('Ctrl Pts',(-2.91025813830041,1.,-2.36578327194741));
#65871=CARTESIAN_POINT('Ctrl Pts',(-2.9115863784204,-1.,-2.36690501170627));
#65872=CARTESIAN_POINT('Ctrl Pts',(-2.9115863784204,1.,-2.36690501170627));
#65873=CARTESIAN_POINT('Ctrl Pts',(-2.9146124988314,-1.,-2.36919161373173));
#65874=CARTESIAN_POINT('Ctrl Pts',(-2.9146124988314,1.,-2.36919161373173));
#65875=CARTESIAN_POINT('Ctrl Pts',(-2.91891503791411,-1.,-2.37229381109821));
#65876=CARTESIAN_POINT('Ctrl Pts',(-2.91891503791411,1.,-2.37229381109821));
#65877=CARTESIAN_POINT('Ctrl Pts',(-2.92430340582608,-1.,-2.3760651052403));
#65878=CARTESIAN_POINT('Ctrl Pts',(-2.92430340582608,1.,-2.3760651052403));
#65879=CARTESIAN_POINT('Ctrl Pts',(-2.93049643640206,-1.,-2.38028989582073));
#65880=CARTESIAN_POINT('Ctrl Pts',(-2.93049643640206,1.,-2.38028989582073));
#65881=CARTESIAN_POINT('Ctrl Pts',(-2.93717903280391,-1.,-2.38472771516311));
#65882=CARTESIAN_POINT('Ctrl Pts',(-2.93717903280391,1.,-2.38472771516311));
#65883=CARTESIAN_POINT('Ctrl Pts',(-2.94404820669076,-1.,-2.38914929090759));
#65884=CARTESIAN_POINT('Ctrl Pts',(-2.94404820669076,1.,-2.38914929090759));
#65885=CARTESIAN_POINT('Ctrl Pts',(-2.95085857128439,-1.,-2.39337207631667));
#65886=CARTESIAN_POINT('Ctrl Pts',(-2.95085857128439,1.,-2.39337207631667));
#65887=CARTESIAN_POINT('Ctrl Pts',(-2.95748006482942,-1.,-2.39730553974517));
#65888=CARTESIAN_POINT('Ctrl Pts',(-2.95748006482942,1.,-2.39730553974517));
#65889=CARTESIAN_POINT('Ctrl Pts',(-2.96390432240312,-1.,-2.4009556571164));
#65890=CARTESIAN_POINT('Ctrl Pts',(-2.96390432240312,1.,-2.4009556571164));
#65891=CARTESIAN_POINT('Ctrl Pts',(-2.9701964131236,-1.,-2.40438604734919));
#65892=CARTESIAN_POINT('Ctrl Pts',(-2.9701964131236,1.,-2.40438604734919));
#65893=CARTESIAN_POINT('Ctrl Pts',(-2.97646002822422,-1.,-2.40768975073713));
#65894=CARTESIAN_POINT('Ctrl Pts',(-2.97646002822422,1.,-2.40768975073713));
#65895=CARTESIAN_POINT('Ctrl Pts',(-2.98280015815107,-1.,-2.41095909342571));
#65896=CARTESIAN_POINT('Ctrl Pts',(-2.98280015815107,1.,-2.41095909342571));
#65897=CARTESIAN_POINT('Ctrl Pts',(-2.98927983005796,-1.,-2.41425064199586));
#65898=CARTESIAN_POINT('Ctrl Pts',(-2.98927983005796,1.,-2.41425064199586));
#65899=CARTESIAN_POINT('Ctrl Pts',(-2.99590509293503,-1.,-2.41757324500514));
#65900=CARTESIAN_POINT('Ctrl Pts',(-2.99590509293503,1.,-2.41757324500514));
#65901=CARTESIAN_POINT('Ctrl Pts',(-3.00264868585996,-1.,-2.42090763946779));
#65902=CARTESIAN_POINT('Ctrl Pts',(-3.00264868585996,1.,-2.42090763946779));
#65903=CARTESIAN_POINT('Ctrl Pts',(-3.00946442616658,-1.,-2.42421849439613));
#65904=CARTESIAN_POINT('Ctrl Pts',(-3.00946442616658,1.,-2.42421849439613));
#65905=CARTESIAN_POINT('Ctrl Pts',(-3.01630420830504,-1.,-2.42746856264168));
#65906=CARTESIAN_POINT('Ctrl Pts',(-3.01630420830504,1.,-2.42746856264168));
#65907=CARTESIAN_POINT('Ctrl Pts',(-3.02313656036004,-1.,-2.43063415586637));
#65908=CARTESIAN_POINT('Ctrl Pts',(-3.02313656036004,1.,-2.43063415586637));
#65909=CARTESIAN_POINT('Ctrl Pts',(-3.02995534946978,-1.,-2.43371241361488));
#65910=CARTESIAN_POINT('Ctrl Pts',(-3.02995534946978,1.,-2.43371241361488));
#65911=CARTESIAN_POINT('Ctrl Pts',(-3.03676949672821,-1.,-2.43671278042414));
#65912=CARTESIAN_POINT('Ctrl Pts',(-3.03676949672821,1.,-2.43671278042414));
#65913=CARTESIAN_POINT('Ctrl Pts',(-3.04359685040555,-1.,-2.43965194061857));
#65914=CARTESIAN_POINT('Ctrl Pts',(-3.04359685040555,1.,-2.43965194061857));
#65915=CARTESIAN_POINT('Ctrl Pts',(-3.05045678021504,-1.,-2.44254768923105));
#65916=CARTESIAN_POINT('Ctrl Pts',(-3.05045678021504,1.,-2.44254768923105));
#65917=CARTESIAN_POINT('Ctrl Pts',(-3.05736242671506,-1.,-2.44541251892556));
#65918=CARTESIAN_POINT('Ctrl Pts',(-3.05736242671506,1.,-2.44541251892556));
#65919=CARTESIAN_POINT('Ctrl Pts',(-3.06431596421405,-1.,-2.44824970516544));
#65920=CARTESIAN_POINT('Ctrl Pts',(-3.06431596421405,1.,-2.44824970516544));
#65921=CARTESIAN_POINT('Ctrl Pts',(-3.07131290521297,-1.,-2.45105688854422));
#65922=CARTESIAN_POINT('Ctrl Pts',(-3.07131290521297,1.,-2.45105688854422));
#65923=CARTESIAN_POINT('Ctrl Pts',(-3.07834472886139,-1.,-2.4538282678779));
#65924=CARTESIAN_POINT('Ctrl Pts',(-3.07834472886139,1.,-2.4538282678779));
#65925=CARTESIAN_POINT('Ctrl Pts',(-3.08540206545315,-1.,-2.45655725437039));
#65926=CARTESIAN_POINT('Ctrl Pts',(-3.08540206545315,1.,-2.45655725437039));
#65927=CARTESIAN_POINT('Ctrl Pts',(-3.09247787931887,-1.,-2.4592391256388));
#65928=CARTESIAN_POINT('Ctrl Pts',(-3.09247787931887,1.,-2.4592391256388));
#65929=CARTESIAN_POINT('Ctrl Pts',(-3.09956993697052,-1.,-2.46187308501884));
#65930=CARTESIAN_POINT('Ctrl Pts',(-3.09956993697052,1.,-2.46187308501884));
#65931=CARTESIAN_POINT('Ctrl Pts',(-3.1066790790198,-1.,-2.46446082979646));
#65932=CARTESIAN_POINT('Ctrl Pts',(-3.1066790790198,1.,-2.46446082979646));
#65933=CARTESIAN_POINT('Ctrl Pts',(-3.11380805536122,-1.,-2.46700558843506));
#65934=CARTESIAN_POINT('Ctrl Pts',(-3.11380805536122,1.,-2.46700558843506));
#65935=CARTESIAN_POINT('Ctrl Pts',(-3.12096015766983,-1.,-2.46951098947469));
#65936=CARTESIAN_POINT('Ctrl Pts',(-3.12096015766983,1.,-2.46951098947469));
#65937=CARTESIAN_POINT('Ctrl Pts',(-3.12813790805952,-1.,-2.47197997765871));
#65938=CARTESIAN_POINT('Ctrl Pts',(-3.12813790805952,1.,-2.47197997765871));
#65939=CARTESIAN_POINT('Ctrl Pts',(-3.13534181229295,-1.,-2.47441378371932));
#65940=CARTESIAN_POINT('Ctrl Pts',(-3.13534181229295,1.,-2.47441378371932));
#65941=CARTESIAN_POINT('Ctrl Pts',(-3.1425709954655,-1.,-2.47681245356109));
#65942=CARTESIAN_POINT('Ctrl Pts',(-3.1425709954655,1.,-2.47681245356109));
#65943=CARTESIAN_POINT('Ctrl Pts',(-3.14982373241352,-1.,-2.47917529057029));
#65944=CARTESIAN_POINT('Ctrl Pts',(-3.14982373241352,1.,-2.47917529057029));
#65945=CARTESIAN_POINT('Ctrl Pts',(-3.15709802322739,-1.,-2.48150133566571));
#65946=CARTESIAN_POINT('Ctrl Pts',(-3.15709802322739,1.,-2.48150133566571));
#65947=CARTESIAN_POINT('Ctrl Pts',(-3.16439213290161,-1.,-2.48378981792725));
#65948=CARTESIAN_POINT('Ctrl Pts',(-3.16439213290161,1.,-2.48378981792725));
#65949=CARTESIAN_POINT('Ctrl Pts',(-3.17170518863313,-1.,-2.48604065348587));
#65950=CARTESIAN_POINT('Ctrl Pts',(-3.17170518863313,1.,-2.48604065348587));
#65951=CARTESIAN_POINT('Ctrl Pts',(-3.17903698136622,-1.,-2.48825428288201));
#65952=CARTESIAN_POINT('Ctrl Pts',(-3.17903698136622,1.,-2.48825428288201));
#65953=CARTESIAN_POINT('Ctrl Pts',(-3.18638771282266,-1.,-2.49043146334059));
#65954=CARTESIAN_POINT('Ctrl Pts',(-3.18638771282266,1.,-2.49043146334059));
#65955=CARTESIAN_POINT('Ctrl Pts',(-3.19375775555798,-1.,-2.49257307239848));
#65956=CARTESIAN_POINT('Ctrl Pts',(-3.19375775555798,1.,-2.49257307239848));
#65957=CARTESIAN_POINT('Ctrl Pts',(-3.20114742397588,-1.,-2.49467992057755));
#65958=CARTESIAN_POINT('Ctrl Pts',(-3.20114742397588,1.,-2.49467992057755));
#65959=CARTESIAN_POINT('Ctrl Pts',(-3.20855669849836,-1.,-2.4967525264737));
#65960=CARTESIAN_POINT('Ctrl Pts',(-3.20855669849836,1.,-2.4967525264737));
#65961=CARTESIAN_POINT('Ctrl Pts',(-3.21598526261286,-1.,-2.4987911459939));
#65962=CARTESIAN_POINT('Ctrl Pts',(-3.21598526261286,1.,-2.4987911459939));
#65963=CARTESIAN_POINT('Ctrl Pts',(-3.22343262620503,-1.,-2.50079587201957));
#65964=CARTESIAN_POINT('Ctrl Pts',(-3.22343262620503,1.,-2.50079587201957));
#65965=CARTESIAN_POINT('Ctrl Pts',(-3.23089822320646,-1.,-2.50276671338111));
#65966=CARTESIAN_POINT('Ctrl Pts',(-3.23089822320646,1.,-2.50276671338111));
#65967=CARTESIAN_POINT('Ctrl Pts',(-3.23838151080319,-1.,-2.5047036758003));
#65968=CARTESIAN_POINT('Ctrl Pts',(-3.23838151080319,1.,-2.5047036758003));
#65969=CARTESIAN_POINT('Ctrl Pts',(-3.24588208983849,-1.,-2.506606859405));
#65970=CARTESIAN_POINT('Ctrl Pts',(-3.24588208983849,1.,-2.506606859405));
#65971=CARTESIAN_POINT('Ctrl Pts',(-3.25339971460982,-1.,-2.50847647070723));
#65972=CARTESIAN_POINT('Ctrl Pts',(-3.25339971460982,1.,-2.50847647070723));
#65973=CARTESIAN_POINT('Ctrl Pts',(-3.26093423001434,-1.,-2.51031277813486));
#65974=CARTESIAN_POINT('Ctrl Pts',(-3.26093423001434,1.,-2.51031277813486));
#65975=CARTESIAN_POINT('Ctrl Pts',(-3.26848552888115,-1.,-2.51211608411423));
#65976=CARTESIAN_POINT('Ctrl Pts',(-3.26848552888115,1.,-2.51211608411423));
#65977=CARTESIAN_POINT('Ctrl Pts',(-3.27605350473142,-1.,-2.513886692704));
#65978=CARTESIAN_POINT('Ctrl Pts',(-3.27605350473142,1.,-2.513886692704));
#65979=CARTESIAN_POINT('Ctrl Pts',(-3.28363799702982,-1.,-2.51562487464514));
#65980=CARTESIAN_POINT('Ctrl Pts',(-3.28363799702982,1.,-2.51562487464514));
#65981=CARTESIAN_POINT('Ctrl Pts',(-3.2912387729927,-1.,-2.51733085123797));
#65982=CARTESIAN_POINT('Ctrl Pts',(-3.2912387729927,1.,-2.51733085123797));
#65983=CARTESIAN_POINT('Ctrl Pts',(-3.29885556388352,-1.,-2.51900480701069));
#65984=CARTESIAN_POINT('Ctrl Pts',(-3.29885556388352,1.,-2.51900480701069));
#65985=CARTESIAN_POINT('Ctrl Pts',(-3.30648808815442,-1.,-2.52064689568511));
#65986=CARTESIAN_POINT('Ctrl Pts',(-3.30648808815442,1.,-2.52064689568511));
#65987=CARTESIAN_POINT('Ctrl Pts',(-3.31413607874645,-1.,-2.52225724871313));
#65988=CARTESIAN_POINT('Ctrl Pts',(-3.31413607874645,1.,-2.52225724871313));
#65989=CARTESIAN_POINT('Ctrl Pts',(-3.32179931078699,-1.,-2.5238359839626));
#65990=CARTESIAN_POINT('Ctrl Pts',(-3.32179931078699,1.,-2.5238359839626));
#65991=CARTESIAN_POINT('Ctrl Pts',(-3.32947762187533,-1.,-2.52538321164634));
#65992=CARTESIAN_POINT('Ctrl Pts',(-3.32947762187533,1.,-2.52538321164634));
#65993=CARTESIAN_POINT('Ctrl Pts',(-3.33717089999103,-1.,-2.52689902690158));
#65994=CARTESIAN_POINT('Ctrl Pts',(-3.33717089999103,1.,-2.52689902690158));
#65995=CARTESIAN_POINT('Ctrl Pts',(-3.34333744115511,-1.,-2.52808660915689));
#65996=CARTESIAN_POINT('Ctrl Pts',(-3.34333744115511,1.,-2.52808660915689));
#65997=CARTESIAN_POINT('Ctrl Pts',(-3.34796903576663,-1.,-2.52896321610703));
#65998=CARTESIAN_POINT('Ctrl Pts',(-3.34796903576663,1.,-2.52896321610703));
#65999=CARTESIAN_POINT('Ctrl Pts',(-3.35105973714071,-1.,-2.5295413654909));
#66000=CARTESIAN_POINT('Ctrl Pts',(-3.35105973714071,1.,-2.5295413654909));
#66001=CARTESIAN_POINT('Ctrl Pts',(-3.35260583073571,-1.,-2.52982887637028));
#66002=CARTESIAN_POINT('Ctrl Pts',(-3.35260583073571,1.,-2.52982887637028));
#66003=CARTESIAN_POINT('',(-2.90994629141676,1.,-2.36531447826073));
#66004=CARTESIAN_POINT('Ctrl Pts',(-2.90994629141676,-1.,-2.36531447826074));
#66005=CARTESIAN_POINT('Ctrl Pts',(-2.90994629141676,-0.666666666666667,
-2.36531447826074));
#66006=CARTESIAN_POINT('Ctrl Pts',(-2.90994629141676,-0.333333333333333,
-2.36531447826074));
#66007=CARTESIAN_POINT('Ctrl Pts',(-2.90994629141676,0.333333333333333,
-2.36531447826074));
#66008=CARTESIAN_POINT('Ctrl Pts',(-2.90994629141676,0.666666666666667,
-2.36531447826074));
#66009=CARTESIAN_POINT('Ctrl Pts',(-2.90994629141676,1.,-2.36531447826074));
#66010=CARTESIAN_POINT('',(-3.35260583073571,1.,-2.52982887637028));
#66011=CARTESIAN_POINT('',(-3.35260583073571,0.,-2.52982887637028));
#66012=CARTESIAN_POINT('Ctrl Pts',(-2.90994629141676,1.,-2.36531447826073));
#66013=CARTESIAN_POINT('Ctrl Pts',(-2.90995756655606,1.,-2.36536211188453));
#66014=CARTESIAN_POINT('Ctrl Pts',(-2.91005770527719,1.,-2.36553202948613));
#66015=CARTESIAN_POINT('Ctrl Pts',(-2.91051690822156,1.,-2.36599991765749));
#66016=CARTESIAN_POINT('Ctrl Pts',(-2.91181344022549,1.,-2.36707658451664));
#66017=CARTESIAN_POINT('Ctrl Pts',(-2.9146124988314,1.,-2.36919161373173));
#66018=CARTESIAN_POINT('Ctrl Pts',(-2.91891503791411,1.,-2.37229381109821));
#66019=CARTESIAN_POINT('Ctrl Pts',(-2.92430340582608,1.,-2.3760651052403));
#66020=CARTESIAN_POINT('Ctrl Pts',(-2.93049643640206,1.,-2.38028989582073));
#66021=CARTESIAN_POINT('Ctrl Pts',(-2.93717903280391,1.,-2.38472771516311));
#66022=CARTESIAN_POINT('Ctrl Pts',(-2.94404820669076,1.,-2.38914929090759));
#66023=CARTESIAN_POINT('Ctrl Pts',(-2.95085857128439,1.,-2.39337207631667));
#66024=CARTESIAN_POINT('Ctrl Pts',(-2.95748006482942,1.,-2.39730553974517));
#66025=CARTESIAN_POINT('Ctrl Pts',(-2.96390432240312,1.,-2.4009556571164));
#66026=CARTESIAN_POINT('Ctrl Pts',(-2.9701964131236,1.,-2.40438604734919));
#66027=CARTESIAN_POINT('Ctrl Pts',(-2.97646002822422,1.,-2.40768975073713));
#66028=CARTESIAN_POINT('Ctrl Pts',(-2.98280015815107,1.,-2.41095909342571));
#66029=CARTESIAN_POINT('Ctrl Pts',(-2.98927983005796,1.,-2.41425064199586));
#66030=CARTESIAN_POINT('Ctrl Pts',(-2.99590509293503,1.,-2.41757324500514));
#66031=CARTESIAN_POINT('Ctrl Pts',(-3.00264868585996,1.,-2.42090763946779));
#66032=CARTESIAN_POINT('Ctrl Pts',(-3.00946442616658,1.,-2.42421849439613));
#66033=CARTESIAN_POINT('Ctrl Pts',(-3.01630420830504,1.,-2.42746856264168));
#66034=CARTESIAN_POINT('Ctrl Pts',(-3.02313656036004,1.,-2.43063415586637));
#66035=CARTESIAN_POINT('Ctrl Pts',(-3.02995534946978,1.,-2.43371241361488));
#66036=CARTESIAN_POINT('Ctrl Pts',(-3.03676949672821,1.,-2.43671278042414));
#66037=CARTESIAN_POINT('Ctrl Pts',(-3.04359685040555,1.,-2.43965194061857));
#66038=CARTESIAN_POINT('Ctrl Pts',(-3.05045678021504,1.,-2.44254768923105));
#66039=CARTESIAN_POINT('Ctrl Pts',(-3.05736242671506,1.,-2.44541251892556));
#66040=CARTESIAN_POINT('Ctrl Pts',(-3.06431596421405,1.,-2.44824970516544));
#66041=CARTESIAN_POINT('Ctrl Pts',(-3.07131290521297,1.,-2.45105688854422));
#66042=CARTESIAN_POINT('Ctrl Pts',(-3.07834472886139,1.,-2.4538282678779));
#66043=CARTESIAN_POINT('Ctrl Pts',(-3.08540206545315,1.,-2.45655725437039));
#66044=CARTESIAN_POINT('Ctrl Pts',(-3.09247787931887,1.,-2.4592391256388));
#66045=CARTESIAN_POINT('Ctrl Pts',(-3.09956993697052,1.,-2.46187308501884));
#66046=CARTESIAN_POINT('Ctrl Pts',(-3.1066790790198,1.,-2.46446082979646));
#66047=CARTESIAN_POINT('Ctrl Pts',(-3.11380805536122,1.,-2.46700558843506));
#66048=CARTESIAN_POINT('Ctrl Pts',(-3.12096015766983,1.,-2.46951098947469));
#66049=CARTESIAN_POINT('Ctrl Pts',(-3.12813790805952,1.,-2.47197997765871));
#66050=CARTESIAN_POINT('Ctrl Pts',(-3.13534181229295,1.,-2.47441378371932));
#66051=CARTESIAN_POINT('Ctrl Pts',(-3.1425709954655,1.,-2.47681245356109));
#66052=CARTESIAN_POINT('Ctrl Pts',(-3.14982373241352,1.,-2.47917529057029));
#66053=CARTESIAN_POINT('Ctrl Pts',(-3.15709802322739,1.,-2.48150133566571));
#66054=CARTESIAN_POINT('Ctrl Pts',(-3.16439213290161,1.,-2.48378981792725));
#66055=CARTESIAN_POINT('Ctrl Pts',(-3.17170518863313,1.,-2.48604065348587));
#66056=CARTESIAN_POINT('Ctrl Pts',(-3.17903698136622,1.,-2.48825428288201));
#66057=CARTESIAN_POINT('Ctrl Pts',(-3.18638771282266,1.,-2.49043146334059));
#66058=CARTESIAN_POINT('Ctrl Pts',(-3.19375775555798,1.,-2.49257307239848));
#66059=CARTESIAN_POINT('Ctrl Pts',(-3.20114742397588,1.,-2.49467992057755));
#66060=CARTESIAN_POINT('Ctrl Pts',(-3.20855669849836,1.,-2.4967525264737));
#66061=CARTESIAN_POINT('Ctrl Pts',(-3.21598526261286,1.,-2.4987911459939));
#66062=CARTESIAN_POINT('Ctrl Pts',(-3.22343262620503,1.,-2.50079587201957));
#66063=CARTESIAN_POINT('Ctrl Pts',(-3.23089822320646,1.,-2.50276671338111));
#66064=CARTESIAN_POINT('Ctrl Pts',(-3.23838151080319,1.,-2.5047036758003));
#66065=CARTESIAN_POINT('Ctrl Pts',(-3.24588208983849,1.,-2.506606859405));
#66066=CARTESIAN_POINT('Ctrl Pts',(-3.25339971460982,1.,-2.50847647070723));
#66067=CARTESIAN_POINT('Ctrl Pts',(-3.26093423001434,1.,-2.51031277813486));
#66068=CARTESIAN_POINT('Ctrl Pts',(-3.26848552888115,1.,-2.51211608411423));
#66069=CARTESIAN_POINT('Ctrl Pts',(-3.27605350473142,1.,-2.513886692704));
#66070=CARTESIAN_POINT('Ctrl Pts',(-3.28363799702982,1.,-2.51562487464514));
#66071=CARTESIAN_POINT('Ctrl Pts',(-3.2912387729927,1.,-2.51733085123797));
#66072=CARTESIAN_POINT('Ctrl Pts',(-3.29885556388352,1.,-2.51900480701069));
#66073=CARTESIAN_POINT('Ctrl Pts',(-3.30648808815442,1.,-2.52064689568511));
#66074=CARTESIAN_POINT('Ctrl Pts',(-3.31413607874645,1.,-2.52225724871313));
#66075=CARTESIAN_POINT('Ctrl Pts',(-3.32179931078699,1.,-2.5238359839626));
#66076=CARTESIAN_POINT('Ctrl Pts',(-3.32947762187533,1.,-2.52538321164634));
#66077=CARTESIAN_POINT('Ctrl Pts',(-3.33717089999103,1.,-2.52689902690158));
#66078=CARTESIAN_POINT('Ctrl Pts',(-3.34333744115511,1.,-2.52808660915689));
#66079=CARTESIAN_POINT('Ctrl Pts',(-3.34796903576663,1.,-2.52896321610703));
#66080=CARTESIAN_POINT('Ctrl Pts',(-3.35105973714071,1.,-2.5295413654909));
#66081=CARTESIAN_POINT('Ctrl Pts',(-3.35260583073571,1.,-2.52982887637028));
#66082=CARTESIAN_POINT('Origin',(-3.35260583073571,0.,-2.52982887637028));
#66083=CARTESIAN_POINT('',(-3.44202241512147,1.,-2.40675750623143));
#66084=CARTESIAN_POINT('Origin',(0.,0.,0.));
#66085=CARTESIAN_POINT('',(-2.79140942341378,1.,-2.50410331873042));
#66086=CARTESIAN_POINT('Origin',(0.,1.,0.));
#66087=CARTESIAN_POINT('Ctrl Pts',(-2.79140942341378,1.,-2.50410331873042));
#66088=CARTESIAN_POINT('Ctrl Pts',(-2.79140942341378,0.666666666666667,
-2.50410331873042));
#66089=CARTESIAN_POINT('Ctrl Pts',(-2.79140942341378,0.333333333333333,
-2.50410331873042));
#66090=CARTESIAN_POINT('Ctrl Pts',(-2.79140942341378,-0.333333333333333,
-2.50410331873042));
#66091=CARTESIAN_POINT('Ctrl Pts',(-2.79140942341378,-0.666666666666667,
-2.50410331873042));
#66092=CARTESIAN_POINT('Ctrl Pts',(-2.79140942341378,-1.,-2.50410331873042));
#66093=CARTESIAN_POINT('Ctrl Pts',(-3.02314558451372,-1.,-2.91557726271063));
#66094=CARTESIAN_POINT('Ctrl Pts',(-3.02314558451372,1.,-2.91557726271063));
#66095=CARTESIAN_POINT('Ctrl Pts',(-3.02261975104912,-1.,-2.91409518070707));
#66096=CARTESIAN_POINT('Ctrl Pts',(-3.02261975104912,1.,-2.91409518070707));
#66097=CARTESIAN_POINT('Ctrl Pts',(-3.02156522743299,-1.,-2.91113297349052));
#66098=CARTESIAN_POINT('Ctrl Pts',(-3.02156522743299,1.,-2.91113297349052));
#66099=CARTESIAN_POINT('Ctrl Pts',(-3.01997487194926,-1.,-2.90669553303902));
#66100=CARTESIAN_POINT('Ctrl Pts',(-3.01997487194926,1.,-2.90669553303902));
#66101=CARTESIAN_POINT('Ctrl Pts',(-3.01783725123646,-1.,-2.90079069102661));
#66102=CARTESIAN_POINT('Ctrl Pts',(-3.01783725123646,1.,-2.90079069102661));
#66103=CARTESIAN_POINT('Ctrl Pts',(-3.01513660433291,-1.,-2.8934292556764));
#66104=CARTESIAN_POINT('Ctrl Pts',(-3.01513660433291,1.,-2.8934292556764));
#66105=CARTESIAN_POINT('Ctrl Pts',(-3.01240727309568,-1.,-2.88608751706796));
#66106=CARTESIAN_POINT('Ctrl Pts',(-3.01240727309568,1.,-2.88608751706796));
#66107=CARTESIAN_POINT('Ctrl Pts',(-3.0096491810855,-1.,-2.87876560072799));
#66108=CARTESIAN_POINT('Ctrl Pts',(-3.0096491810855,1.,-2.87876560072799));
#66109=CARTESIAN_POINT('Ctrl Pts',(-3.00686224485374,-1.,-2.87146368430104));
#66110=CARTESIAN_POINT('Ctrl Pts',(-3.00686224485374,1.,-2.87146368430104));
#66111=CARTESIAN_POINT('Ctrl Pts',(-3.00404638316245,-1.,-2.86418200833065));
#66112=CARTESIAN_POINT('Ctrl Pts',(-3.00404638316245,1.,-2.86418200833065));
#66113=CARTESIAN_POINT('Ctrl Pts',(-3.0012015079552,-1.,-2.85692085715129));
#66114=CARTESIAN_POINT('Ctrl Pts',(-3.0012015079552,1.,-2.85692085715129));
#66115=CARTESIAN_POINT('Ctrl Pts',(-2.99832751144566,-1.,-2.84968053289104));
#66116=CARTESIAN_POINT('Ctrl Pts',(-2.99832751144566,1.,-2.84968053289104));
#66117=CARTESIAN_POINT('Ctrl Pts',(-2.995424253416,-1.,-2.84246132984334));
#66118=CARTESIAN_POINT('Ctrl Pts',(-2.995424253416,1.,-2.84246132984334));
#66119=CARTESIAN_POINT('Ctrl Pts',(-2.99249155170479,-1.,-2.83526351254383));
#66120=CARTESIAN_POINT('Ctrl Pts',(-2.99249155170479,1.,-2.83526351254383));
#66121=CARTESIAN_POINT('Ctrl Pts',(-2.98952916401699,-1.,-2.82808728190402));
#66122=CARTESIAN_POINT('Ctrl Pts',(-2.98952916401699,1.,-2.82808728190402));
#66123=CARTESIAN_POINT('Ctrl Pts',(-2.98653680669434,-1.,-2.82093279065704));
#66124=CARTESIAN_POINT('Ctrl Pts',(-2.98653680669434,1.,-2.82093279065704));
#66125=CARTESIAN_POINT('Ctrl Pts',(-2.9835141977994,-1.,-2.81380019196454));
#66126=CARTESIAN_POINT('Ctrl Pts',(-2.9835141977994,1.,-2.81380019196454));
#66127=CARTESIAN_POINT('Ctrl Pts',(-2.98046109647299,-1.,-2.80668968101162));
#66128=CARTESIAN_POINT('Ctrl Pts',(-2.98046109647299,1.,-2.80668968101162));
#66129=CARTESIAN_POINT('Ctrl Pts',(-2.97737733718242,-1.,-2.79960153278186));
#66130=CARTESIAN_POINT('Ctrl Pts',(-2.97737733718242,1.,-2.79960153278186));
#66131=CARTESIAN_POINT('Ctrl Pts',(-2.97426288347475,-1.,-2.79253615718147));
#66132=CARTESIAN_POINT('Ctrl Pts',(-2.97426288347475,1.,-2.79253615718147));
#66133=CARTESIAN_POINT('Ctrl Pts',(-2.97111781461349,-1.,-2.78549409123657));
#66134=CARTESIAN_POINT('Ctrl Pts',(-2.97111781461349,1.,-2.78549409123657));
#66135=CARTESIAN_POINT('Ctrl Pts',(-2.9679422104295,-1.,-2.77847589542767));
#66136=CARTESIAN_POINT('Ctrl Pts',(-2.9679422104295,1.,-2.77847589542767));
#66137=CARTESIAN_POINT('Ctrl Pts',(-2.96473605585548,-1.,-2.77148206836464));
#66138=CARTESIAN_POINT('Ctrl Pts',(-2.96473605585548,1.,-2.77148206836464));
#66139=CARTESIAN_POINT('Ctrl Pts',(-2.96149914764832,-1.,-2.76451296269571));
#66140=CARTESIAN_POINT('Ctrl Pts',(-2.96149914764832,1.,-2.76451296269571));
#66141=CARTESIAN_POINT('Ctrl Pts',(-2.9582309766594,-1.,-2.75756867888393));
#66142=CARTESIAN_POINT('Ctrl Pts',(-2.9582309766594,1.,-2.75756867888393));
#66143=CARTESIAN_POINT('Ctrl Pts',(-2.95493069316211,-1.,-2.75064903318996));
#66144=CARTESIAN_POINT('Ctrl Pts',(-2.95493069316211,1.,-2.75064903318996));
#66145=CARTESIAN_POINT('Ctrl Pts',(-2.95159737214305,-1.,-2.7437537949221));
#66146=CARTESIAN_POINT('Ctrl Pts',(-2.95159737214305,1.,-2.7437537949221));
#66147=CARTESIAN_POINT('Ctrl Pts',(-2.94823023414381,-1.,-2.73688288329825));
#66148=CARTESIAN_POINT('Ctrl Pts',(-2.94823023414381,1.,-2.73688288329825));
#66149=CARTESIAN_POINT('Ctrl Pts',(-2.94482887675139,-1.,-2.73003657371613));
#66150=CARTESIAN_POINT('Ctrl Pts',(-2.94482887675139,1.,-2.73003657371613));
#66151=CARTESIAN_POINT('Ctrl Pts',(-2.94139351933882,-1.,-2.72321571511322));
#66152=CARTESIAN_POINT('Ctrl Pts',(-2.94139351933882,1.,-2.72321571511322));
#66153=CARTESIAN_POINT('Ctrl Pts',(-2.93792519474955,-1.,-2.71642190053575));
#66154=CARTESIAN_POINT('Ctrl Pts',(-2.93792519474955,1.,-2.71642190053575));
#66155=CARTESIAN_POINT('Ctrl Pts',(-2.93442516311168,-1.,-2.70965695523776));
#66156=CARTESIAN_POINT('Ctrl Pts',(-2.93442516311168,1.,-2.70965695523776));
#66157=CARTESIAN_POINT('Ctrl Pts',(-2.93089438233746,-1.,-2.70292247416881));
#66158=CARTESIAN_POINT('Ctrl Pts',(-2.93089438233746,1.,-2.70292247416881));
#66159=CARTESIAN_POINT('Ctrl Pts',(-2.92733294395268,-1.,-2.69621932864302));
#66160=CARTESIAN_POINT('Ctrl Pts',(-2.92733294395268,1.,-2.69621932864302));
#66161=CARTESIAN_POINT('Ctrl Pts',(-2.92373955325876,-1.,-2.68954721165342));
#66162=CARTESIAN_POINT('Ctrl Pts',(-2.92373955325876,1.,-2.68954721165342));
#66163=CARTESIAN_POINT('Ctrl Pts',(-2.92011090722152,-1.,-2.68290409279689));
#66164=CARTESIAN_POINT('Ctrl Pts',(-2.92011090722152,1.,-2.68290409279689));
#66165=CARTESIAN_POINT('Ctrl Pts',(-2.91644290704281,-1.,-2.67628728855309));
#66166=CARTESIAN_POINT('Ctrl Pts',(-2.91644290704281,1.,-2.67628728855309));
#66167=CARTESIAN_POINT('Ctrl Pts',(-2.91273193382876,-1.,-2.66969458792627));
#66168=CARTESIAN_POINT('Ctrl Pts',(-2.91273193382876,1.,-2.66969458792627));
#66169=CARTESIAN_POINT('Ctrl Pts',(-2.90897617968921,-1.,-2.66312542616808));
#66170=CARTESIAN_POINT('Ctrl Pts',(-2.90897617968921,1.,-2.66312542616808));
#66171=CARTESIAN_POINT('Ctrl Pts',(-2.90517678087467,-1.,-2.65658188464287));
#66172=CARTESIAN_POINT('Ctrl Pts',(-2.90517678087467,1.,-2.65658188464287));
#66173=CARTESIAN_POINT('Ctrl Pts',(-2.90133950224879,-1.,-2.65007017365576));
#66174=CARTESIAN_POINT('Ctrl Pts',(-2.90133950224879,1.,-2.65007017365576));
#66175=CARTESIAN_POINT('Ctrl Pts',(-2.89747231723361,-1.,-2.64359851684146));
#66176=CARTESIAN_POINT('Ctrl Pts',(-2.89747231723361,1.,-2.64359851684146));
#66177=CARTESIAN_POINT('Ctrl Pts',(-2.89358228854557,-1.,-2.63717442263944));
#66178=CARTESIAN_POINT('Ctrl Pts',(-2.89358228854557,1.,-2.63717442263944));
#66179=CARTESIAN_POINT('Ctrl Pts',(-2.88967244854243,-1.,-2.63080195420771));
#66180=CARTESIAN_POINT('Ctrl Pts',(-2.88967244854243,1.,-2.63080195420771));
#66181=CARTESIAN_POINT('Ctrl Pts',(-2.88573922195049,-1.,-2.62447947640253));
#66182=CARTESIAN_POINT('Ctrl Pts',(-2.88573922195049,1.,-2.62447947640253));
#66183=CARTESIAN_POINT('Ctrl Pts',(-2.88176821427502,-1.,-2.61819596473087));
#66184=CARTESIAN_POINT('Ctrl Pts',(-2.88176821427502,1.,-2.61819596473087));
#66185=CARTESIAN_POINT('Ctrl Pts',(-2.87773881947885,-1.,-2.61193507170928));
#66186=CARTESIAN_POINT('Ctrl Pts',(-2.87773881947885,1.,-2.61193507170928));
#66187=CARTESIAN_POINT('Ctrl Pts',(-2.87363176656475,-1.,-2.6056817788128));
#66188=CARTESIAN_POINT('Ctrl Pts',(-2.87363176656475,1.,-2.6056817788128));
#66189=CARTESIAN_POINT('Ctrl Pts',(-2.86943633170712,-1.,-2.59942875223202));
#66190=CARTESIAN_POINT('Ctrl Pts',(-2.86943633170712,1.,-2.59942875223202));
#66191=CARTESIAN_POINT('Ctrl Pts',(-2.86515629953528,-1.,-2.59318160184921));
#66192=CARTESIAN_POINT('Ctrl Pts',(-2.86515629953528,1.,-2.59318160184921));
#66193=CARTESIAN_POINT('Ctrl Pts',(-2.86081999003668,-1.,-2.5869677064356));
#66194=CARTESIAN_POINT('Ctrl Pts',(-2.86081999003668,1.,-2.5869677064356));
#66195=CARTESIAN_POINT('Ctrl Pts',(-2.85647171715147,-1.,-2.58082875254407));
#66196=CARTESIAN_POINT('Ctrl Pts',(-2.85647171715147,1.,-2.58082875254407));
#66197=CARTESIAN_POINT('Ctrl Pts',(-2.85215360144483,-1.,-2.57480482727128));
#66198=CARTESIAN_POINT('Ctrl Pts',(-2.85215360144483,1.,-2.57480482727128));
#66199=CARTESIAN_POINT('Ctrl Pts',(-2.84788893329091,-1.,-2.56891984251743));
#66200=CARTESIAN_POINT('Ctrl Pts',(-2.84788893329091,1.,-2.56891984251743));
#66201=CARTESIAN_POINT('Ctrl Pts',(-2.84366802680211,-1.,-2.56316920798489));
#66202=CARTESIAN_POINT('Ctrl Pts',(-2.84366802680211,1.,-2.56316920798489));
#66203=CARTESIAN_POINT('Ctrl Pts',(-2.83942515220699,-1.,-2.55749952145165));
#66204=CARTESIAN_POINT('Ctrl Pts',(-2.83942515220699,1.,-2.55749952145165));
#66205=CARTESIAN_POINT('Ctrl Pts',(-2.83505269592412,-1.,-2.55182152806964));
#66206=CARTESIAN_POINT('Ctrl Pts',(-2.83505269592412,1.,-2.55182152806964));
#66207=CARTESIAN_POINT('Ctrl Pts',(-2.83044254225794,-1.,-2.54604736792542));
#66208=CARTESIAN_POINT('Ctrl Pts',(-2.83044254225794,1.,-2.54604736792542));
#66209=CARTESIAN_POINT('Ctrl Pts',(-2.82552167649157,-1.,-2.54012272520141));
#66210=CARTESIAN_POINT('Ctrl Pts',(-2.82552167649157,1.,-2.54012272520141));
#66211=CARTESIAN_POINT('Ctrl Pts',(-2.82028550483744,-1.,-2.53405679667463));
#66212=CARTESIAN_POINT('Ctrl Pts',(-2.82028550483744,1.,-2.53405679667463));
#66213=CARTESIAN_POINT('Ctrl Pts',(-2.8148437904867,-1.,-2.52796388055457));
#66214=CARTESIAN_POINT('Ctrl Pts',(-2.8148437904867,1.,-2.52796388055457));
#66215=CARTESIAN_POINT('Ctrl Pts',(-2.80941521967234,-1.,-2.52205778589922));
#66216=CARTESIAN_POINT('Ctrl Pts',(-2.80941521967234,1.,-2.52205778589922));
#66217=CARTESIAN_POINT('Ctrl Pts',(-2.80427363984939,-1.,-2.51660190466067));
#66218=CARTESIAN_POINT('Ctrl Pts',(-2.80427363984939,1.,-2.51660190466067));
#66219=CARTESIAN_POINT('Ctrl Pts',(-2.79970585014308,-1.,-2.51186983687947));
#66220=CARTESIAN_POINT('Ctrl Pts',(-2.79970585014308,1.,-2.51186983687947));
#66221=CARTESIAN_POINT('Ctrl Pts',(-2.7959687805717,-1.,-2.50810555977564));
#66222=CARTESIAN_POINT('Ctrl Pts',(-2.7959687805717,1.,-2.50810555977564));
#66223=CARTESIAN_POINT('Ctrl Pts',(-2.79323694088143,-1.,-2.50547439929077));
#66224=CARTESIAN_POINT('Ctrl Pts',(-2.79323694088143,1.,-2.50547439929077));
#66225=CARTESIAN_POINT('Ctrl Pts',(-2.79192122906739,-1.,-2.50433799076945));
#66226=CARTESIAN_POINT('Ctrl Pts',(-2.79192122906739,1.,-2.50433799076945));
#66227=CARTESIAN_POINT('Ctrl Pts',(-2.79143626022225,-1.,-2.50404230339032));
#66228=CARTESIAN_POINT('Ctrl Pts',(-2.79143626022225,1.,-2.50404230339032));
#66229=CARTESIAN_POINT('Ctrl Pts',(-2.79133581100044,-1.,-2.50409239460011));
#66230=CARTESIAN_POINT('Ctrl Pts',(-2.79133581100044,1.,-2.50409239460011));
#66231=CARTESIAN_POINT('Ctrl Pts',(-2.79134130681569,-1.,-2.50417924854921));
#66232=CARTESIAN_POINT('Ctrl Pts',(-2.79134130681569,1.,-2.50417924854921));
#66233=CARTESIAN_POINT('',(-3.02314558451372,1.,-2.91557726271063));
#66234=CARTESIAN_POINT('Ctrl Pts',(-3.02314558451372,1.,-2.91557726271063));
#66235=CARTESIAN_POINT('Ctrl Pts',(-3.02261975104912,1.,-2.91409518070707));
#66236=CARTESIAN_POINT('Ctrl Pts',(-3.02156522743299,1.,-2.91113297349052));
#66237=CARTESIAN_POINT('Ctrl Pts',(-3.01997487194926,1.,-2.90669553303902));
#66238=CARTESIAN_POINT('Ctrl Pts',(-3.01783725123646,1.,-2.90079069102661));
#66239=CARTESIAN_POINT('Ctrl Pts',(-3.01513660433291,1.,-2.8934292556764));
#66240=CARTESIAN_POINT('Ctrl Pts',(-3.01240727309568,1.,-2.88608751706796));
#66241=CARTESIAN_POINT('Ctrl Pts',(-3.0096491810855,1.,-2.87876560072799));
#66242=CARTESIAN_POINT('Ctrl Pts',(-3.00686224485374,1.,-2.87146368430104));
#66243=CARTESIAN_POINT('Ctrl Pts',(-3.00404638316245,1.,-2.86418200833065));
#66244=CARTESIAN_POINT('Ctrl Pts',(-3.0012015079552,1.,-2.85692085715129));
#66245=CARTESIAN_POINT('Ctrl Pts',(-2.99832751144566,1.,-2.84968053289104));
#66246=CARTESIAN_POINT('Ctrl Pts',(-2.995424253416,1.,-2.84246132984334));
#66247=CARTESIAN_POINT('Ctrl Pts',(-2.99249155170479,1.,-2.83526351254383));
#66248=CARTESIAN_POINT('Ctrl Pts',(-2.98952916401699,1.,-2.82808728190402));
#66249=CARTESIAN_POINT('Ctrl Pts',(-2.98653680669434,1.,-2.82093279065704));
#66250=CARTESIAN_POINT('Ctrl Pts',(-2.9835141977994,1.,-2.81380019196454));
#66251=CARTESIAN_POINT('Ctrl Pts',(-2.98046109647299,1.,-2.80668968101162));
#66252=CARTESIAN_POINT('Ctrl Pts',(-2.97737733718242,1.,-2.79960153278186));
#66253=CARTESIAN_POINT('Ctrl Pts',(-2.97426288347475,1.,-2.79253615718147));
#66254=CARTESIAN_POINT('Ctrl Pts',(-2.97111781461349,1.,-2.78549409123657));
#66255=CARTESIAN_POINT('Ctrl Pts',(-2.9679422104295,1.,-2.77847589542767));
#66256=CARTESIAN_POINT('Ctrl Pts',(-2.96473605585548,1.,-2.77148206836464));
#66257=CARTESIAN_POINT('Ctrl Pts',(-2.96149914764832,1.,-2.76451296269571));
#66258=CARTESIAN_POINT('Ctrl Pts',(-2.9582309766594,1.,-2.75756867888393));
#66259=CARTESIAN_POINT('Ctrl Pts',(-2.95493069316211,1.,-2.75064903318996));
#66260=CARTESIAN_POINT('Ctrl Pts',(-2.95159737214305,1.,-2.7437537949221));
#66261=CARTESIAN_POINT('Ctrl Pts',(-2.94823023414381,1.,-2.73688288329825));
#66262=CARTESIAN_POINT('Ctrl Pts',(-2.94482887675139,1.,-2.73003657371613));
#66263=CARTESIAN_POINT('Ctrl Pts',(-2.94139351933882,1.,-2.72321571511322));
#66264=CARTESIAN_POINT('Ctrl Pts',(-2.93792519474955,1.,-2.71642190053575));
#66265=CARTESIAN_POINT('Ctrl Pts',(-2.93442516311168,1.,-2.70965695523776));
#66266=CARTESIAN_POINT('Ctrl Pts',(-2.93089438233746,1.,-2.70292247416881));
#66267=CARTESIAN_POINT('Ctrl Pts',(-2.92733294395268,1.,-2.69621932864302));
#66268=CARTESIAN_POINT('Ctrl Pts',(-2.92373955325876,1.,-2.68954721165342));
#66269=CARTESIAN_POINT('Ctrl Pts',(-2.92011090722152,1.,-2.68290409279689));
#66270=CARTESIAN_POINT('Ctrl Pts',(-2.91644290704281,1.,-2.67628728855309));
#66271=CARTESIAN_POINT('Ctrl Pts',(-2.91273193382876,1.,-2.66969458792627));
#66272=CARTESIAN_POINT('Ctrl Pts',(-2.90897617968921,1.,-2.66312542616808));
#66273=CARTESIAN_POINT('Ctrl Pts',(-2.90517678087467,1.,-2.65658188464287));
#66274=CARTESIAN_POINT('Ctrl Pts',(-2.90133950224879,1.,-2.65007017365576));
#66275=CARTESIAN_POINT('Ctrl Pts',(-2.89747231723361,1.,-2.64359851684146));
#66276=CARTESIAN_POINT('Ctrl Pts',(-2.89358228854557,1.,-2.63717442263944));
#66277=CARTESIAN_POINT('Ctrl Pts',(-2.88967244854243,1.,-2.63080195420771));
#66278=CARTESIAN_POINT('Ctrl Pts',(-2.88573922195049,1.,-2.62447947640253));
#66279=CARTESIAN_POINT('Ctrl Pts',(-2.88176821427502,1.,-2.61819596473087));
#66280=CARTESIAN_POINT('Ctrl Pts',(-2.87773881947885,1.,-2.61193507170928));
#66281=CARTESIAN_POINT('Ctrl Pts',(-2.87363176656475,1.,-2.6056817788128));
#66282=CARTESIAN_POINT('Ctrl Pts',(-2.86943633170712,1.,-2.59942875223202));
#66283=CARTESIAN_POINT('Ctrl Pts',(-2.86515629953528,1.,-2.59318160184921));
#66284=CARTESIAN_POINT('Ctrl Pts',(-2.86081999003668,1.,-2.5869677064356));
#66285=CARTESIAN_POINT('Ctrl Pts',(-2.85647171715147,1.,-2.58082875254407));
#66286=CARTESIAN_POINT('Ctrl Pts',(-2.85215360144483,1.,-2.57480482727128));
#66287=CARTESIAN_POINT('Ctrl Pts',(-2.84788893329091,1.,-2.56891984251743));
#66288=CARTESIAN_POINT('Ctrl Pts',(-2.84366802680211,1.,-2.56316920798489));
#66289=CARTESIAN_POINT('Ctrl Pts',(-2.83942515220699,1.,-2.55749952145165));
#66290=CARTESIAN_POINT('Ctrl Pts',(-2.83505269592412,1.,-2.55182152806964));
#66291=CARTESIAN_POINT('Ctrl Pts',(-2.83044254225794,1.,-2.54604736792542));
#66292=CARTESIAN_POINT('Ctrl Pts',(-2.82552167649157,1.,-2.54012272520141));
#66293=CARTESIAN_POINT('Ctrl Pts',(-2.82028550483744,1.,-2.53405679667463));
#66294=CARTESIAN_POINT('Ctrl Pts',(-2.8148437904867,1.,-2.52796388055457));
#66295=CARTESIAN_POINT('Ctrl Pts',(-2.80941521967234,1.,-2.52205778589922));
#66296=CARTESIAN_POINT('Ctrl Pts',(-2.80427363984939,1.,-2.51660190466067));
#66297=CARTESIAN_POINT('Ctrl Pts',(-2.79970585014308,1.,-2.51186983687947));
#66298=CARTESIAN_POINT('Ctrl Pts',(-2.7959687805717,1.,-2.50810555977564));
#66299=CARTESIAN_POINT('Ctrl Pts',(-2.79344192164204,1.,-2.50567182569153));
#66300=CARTESIAN_POINT('Ctrl Pts',(-2.79217568804874,1.,-2.50455968395235));
#66301=CARTESIAN_POINT('Ctrl Pts',(-2.79164172519039,1.,-2.50417932839344));
#66302=CARTESIAN_POINT('Ctrl Pts',(-2.79145823440899,1.,-2.50410700351427));
#66303=CARTESIAN_POINT('Ctrl Pts',(-2.79140942341378,1.,-2.50410331873043));
#66304=CARTESIAN_POINT('',(-3.02314558451372,0.,-2.91557726271063));
#66305=CARTESIAN_POINT('Ctrl Pts',(-2.50417924854921,-1.,-2.79134130681569));
#66306=CARTESIAN_POINT('Ctrl Pts',(-2.50417924854921,1.,-2.79134130681569));
#66307=CARTESIAN_POINT('Ctrl Pts',(-2.50409239460108,-1.,-2.7913358110015));
#66308=CARTESIAN_POINT('Ctrl Pts',(-2.50409239460108,1.,-2.7913358110015));
#66309=CARTESIAN_POINT('Ctrl Pts',(-2.50404230339286,-1.,-2.79143626022503));
#66310=CARTESIAN_POINT('Ctrl Pts',(-2.50404230339286,1.,-2.79143626022503));
#66311=CARTESIAN_POINT('Ctrl Pts',(-2.5043379907732,-1.,-2.79192122907148));
#66312=CARTESIAN_POINT('Ctrl Pts',(-2.5043379907732,1.,-2.79192122907148));
#66313=CARTESIAN_POINT('Ctrl Pts',(-2.50547439929414,-1.,-2.7932369408851));
#66314=CARTESIAN_POINT('Ctrl Pts',(-2.50547439929414,1.,-2.7932369408851));
#66315=CARTESIAN_POINT('Ctrl Pts',(-2.50810555977671,-1.,-2.79596878057287));
#66316=CARTESIAN_POINT('Ctrl Pts',(-2.50810555977671,1.,-2.79596878057287));
#66317=CARTESIAN_POINT('Ctrl Pts',(-2.51186983687818,-1.,-2.79970585014168));
#66318=CARTESIAN_POINT('Ctrl Pts',(-2.51186983687818,1.,-2.79970585014168));
#66319=CARTESIAN_POINT('Ctrl Pts',(-2.51660190465805,-1.,-2.80427363984653));
#66320=CARTESIAN_POINT('Ctrl Pts',(-2.51660190465805,1.,-2.80427363984653));
#66321=CARTESIAN_POINT('Ctrl Pts',(-2.52205778589653,-1.,-2.80941521966941));
#66322=CARTESIAN_POINT('Ctrl Pts',(-2.52205778589653,1.,-2.80941521966941));
#66323=CARTESIAN_POINT('Ctrl Pts',(-2.52796388055278,-1.,-2.81484379048475));
#66324=CARTESIAN_POINT('Ctrl Pts',(-2.52796388055278,1.,-2.81484379048475));
#66325=CARTESIAN_POINT('Ctrl Pts',(-2.53405679667412,-1.,-2.82028550483689));
#66326=CARTESIAN_POINT('Ctrl Pts',(-2.53405679667412,1.,-2.82028550483689));
#66327=CARTESIAN_POINT('Ctrl Pts',(-2.54012272520199,-1.,-2.8255216764922));
#66328=CARTESIAN_POINT('Ctrl Pts',(-2.54012272520199,1.,-2.8255216764922));
#66329=CARTESIAN_POINT('Ctrl Pts',(-2.54604736792655,-1.,-2.83044254225917));
#66330=CARTESIAN_POINT('Ctrl Pts',(-2.54604736792655,1.,-2.83044254225917));
#66331=CARTESIAN_POINT('Ctrl Pts',(-2.55182152807077,-1.,-2.83505269592536));
#66332=CARTESIAN_POINT('Ctrl Pts',(-2.55182152807077,1.,-2.83505269592536));
#66333=CARTESIAN_POINT('Ctrl Pts',(-2.55749952145241,-1.,-2.83942515220782));
#66334=CARTESIAN_POINT('Ctrl Pts',(-2.55749952145241,1.,-2.83942515220782));
#66335=CARTESIAN_POINT('Ctrl Pts',(-2.56316920798513,-1.,-2.84366802680237));
#66336=CARTESIAN_POINT('Ctrl Pts',(-2.56316920798513,1.,-2.84366802680237));
#66337=CARTESIAN_POINT('Ctrl Pts',(-2.56891984251721,-1.,-2.84788893329067));
#66338=CARTESIAN_POINT('Ctrl Pts',(-2.56891984251721,1.,-2.84788893329067));
#66339=CARTESIAN_POINT('Ctrl Pts',(-2.57480482727081,-1.,-2.85215360144431));
#66340=CARTESIAN_POINT('Ctrl Pts',(-2.57480482727081,1.,-2.85215360144431));
#66341=CARTESIAN_POINT('Ctrl Pts',(-2.58082875254357,-1.,-2.85647171715092));
#66342=CARTESIAN_POINT('Ctrl Pts',(-2.58082875254357,1.,-2.85647171715092));
#66343=CARTESIAN_POINT('Ctrl Pts',(-2.58696770643524,-1.,-2.86081999003629));
#66344=CARTESIAN_POINT('Ctrl Pts',(-2.58696770643524,1.,-2.86081999003629));
#66345=CARTESIAN_POINT('Ctrl Pts',(-2.59318160184908,-1.,-2.86515629953513));
#66346=CARTESIAN_POINT('Ctrl Pts',(-2.59318160184908,1.,-2.86515629953513));
#66347=CARTESIAN_POINT('Ctrl Pts',(-2.5994287522321,-1.,-2.86943633170722));
#66348=CARTESIAN_POINT('Ctrl Pts',(-2.5994287522321,1.,-2.86943633170722));
#66349=CARTESIAN_POINT('Ctrl Pts',(-2.60568177881303,-1.,-2.87363176656501));
#66350=CARTESIAN_POINT('Ctrl Pts',(-2.60568177881303,1.,-2.87363176656501));
#66351=CARTESIAN_POINT('Ctrl Pts',(-2.61193507170955,-1.,-2.87773881947915));
#66352=CARTESIAN_POINT('Ctrl Pts',(-2.61193507170955,1.,-2.87773881947915));
#66353=CARTESIAN_POINT('Ctrl Pts',(-2.61819596473108,-1.,-2.88176821427525));
#66354=CARTESIAN_POINT('Ctrl Pts',(-2.61819596473108,1.,-2.88176821427525));
#66355=CARTESIAN_POINT('Ctrl Pts',(-2.62447947640262,-1.,-2.88573922195059));
#66356=CARTESIAN_POINT('Ctrl Pts',(-2.62447947640262,1.,-2.88573922195059));
#66357=CARTESIAN_POINT('Ctrl Pts',(-2.63080195420767,-1.,-2.88967244854239));
#66358=CARTESIAN_POINT('Ctrl Pts',(-2.63080195420767,1.,-2.88967244854239));
#66359=CARTESIAN_POINT('Ctrl Pts',(-2.63717442263932,-1.,-2.89358228854544));
#66360=CARTESIAN_POINT('Ctrl Pts',(-2.63717442263932,1.,-2.89358228854544));
#66361=CARTESIAN_POINT('Ctrl Pts',(-2.64359851684131,-1.,-2.89747231723345));
#66362=CARTESIAN_POINT('Ctrl Pts',(-2.64359851684131,1.,-2.89747231723345));
#66363=CARTESIAN_POINT('Ctrl Pts',(-2.65007017365564,-1.,-2.90133950224867));
#66364=CARTESIAN_POINT('Ctrl Pts',(-2.65007017365564,1.,-2.90133950224867));
#66365=CARTESIAN_POINT('Ctrl Pts',(-2.65658188464282,-1.,-2.90517678087461));
#66366=CARTESIAN_POINT('Ctrl Pts',(-2.65658188464282,1.,-2.90517678087461));
#66367=CARTESIAN_POINT('Ctrl Pts',(-2.6631254261681,-1.,-2.90897617968923));
#66368=CARTESIAN_POINT('Ctrl Pts',(-2.6631254261681,1.,-2.90897617968923));
#66369=CARTESIAN_POINT('Ctrl Pts',(-2.66969458792631,-1.,-2.91273193382882));
#66370=CARTESIAN_POINT('Ctrl Pts',(-2.66969458792631,1.,-2.91273193382882));
#66371=CARTESIAN_POINT('Ctrl Pts',(-2.67628728855312,-1.,-2.91644290704285));
#66372=CARTESIAN_POINT('Ctrl Pts',(-2.67628728855312,1.,-2.91644290704285));
#66373=CARTESIAN_POINT('Ctrl Pts',(-2.68290409279688,-1.,-2.92011090722152));
#66374=CARTESIAN_POINT('Ctrl Pts',(-2.68290409279688,1.,-2.92011090722152));
#66375=CARTESIAN_POINT('Ctrl Pts',(-2.68954721165339,-1.,-2.92373955325875));
#66376=CARTESIAN_POINT('Ctrl Pts',(-2.68954721165339,1.,-2.92373955325875));
#66377=CARTESIAN_POINT('Ctrl Pts',(-2.69621932864301,-1.,-2.92733294395267));
#66378=CARTESIAN_POINT('Ctrl Pts',(-2.69621932864301,1.,-2.92733294395267));
#66379=CARTESIAN_POINT('Ctrl Pts',(-2.70292247416885,-1.,-2.93089438233749));
#66380=CARTESIAN_POINT('Ctrl Pts',(-2.70292247416885,1.,-2.93089438233749));
#66381=CARTESIAN_POINT('Ctrl Pts',(-2.70965695523787,-1.,-2.93442516311179));
#66382=CARTESIAN_POINT('Ctrl Pts',(-2.70965695523787,1.,-2.93442516311179));
#66383=CARTESIAN_POINT('Ctrl Pts',(-2.71642190053592,-1.,-2.93792519474972));
#66384=CARTESIAN_POINT('Ctrl Pts',(-2.71642190053592,1.,-2.93792519474972));
#66385=CARTESIAN_POINT('Ctrl Pts',(-2.72321571511337,-1.,-2.94139351933897));
#66386=CARTESIAN_POINT('Ctrl Pts',(-2.72321571511337,1.,-2.94139351933897));
#66387=CARTESIAN_POINT('Ctrl Pts',(-2.73003657371617,-1.,-2.94482887675143));
#66388=CARTESIAN_POINT('Ctrl Pts',(-2.73003657371617,1.,-2.94482887675143));
#66389=CARTESIAN_POINT('Ctrl Pts',(-2.73688288329808,-1.,-2.94823023414364));
#66390=CARTESIAN_POINT('Ctrl Pts',(-2.73688288329808,1.,-2.94823023414364));
#66391=CARTESIAN_POINT('Ctrl Pts',(-2.74375379492172,-1.,-2.95159737214266));
#66392=CARTESIAN_POINT('Ctrl Pts',(-2.74375379492172,1.,-2.95159737214266));
#66393=CARTESIAN_POINT('Ctrl Pts',(-2.75064903318947,-1.,-2.95493069316161));
#66394=CARTESIAN_POINT('Ctrl Pts',(-2.75064903318947,1.,-2.95493069316161));
#66395=CARTESIAN_POINT('Ctrl Pts',(-2.7575686788835,-1.,-2.95823097665896));
#66396=CARTESIAN_POINT('Ctrl Pts',(-2.7575686788835,1.,-2.95823097665896));
#66397=CARTESIAN_POINT('Ctrl Pts',(-2.76451296269557,-1.,-2.96149914764818));
#66398=CARTESIAN_POINT('Ctrl Pts',(-2.76451296269557,1.,-2.96149914764818));
#66399=CARTESIAN_POINT('Ctrl Pts',(-2.77148206836498,-1.,-2.96473605585583));
#66400=CARTESIAN_POINT('Ctrl Pts',(-2.77148206836498,1.,-2.96473605585583));
#66401=CARTESIAN_POINT('Ctrl Pts',(-2.7784758954285,-1.,-2.96794221043036));
#66402=CARTESIAN_POINT('Ctrl Pts',(-2.7784758954285,1.,-2.96794221043036));
#66403=CARTESIAN_POINT('Ctrl Pts',(-2.78549409123769,-1.,-2.97111781461465));
#66404=CARTESIAN_POINT('Ctrl Pts',(-2.78549409123769,1.,-2.97111781461465));
#66405=CARTESIAN_POINT('Ctrl Pts',(-2.79253615718248,-1.,-2.9742628834758));
#66406=CARTESIAN_POINT('Ctrl Pts',(-2.79253615718248,1.,-2.9742628834758));
#66407=CARTESIAN_POINT('Ctrl Pts',(-2.7996015327823,-1.,-2.97737733718287));
#66408=CARTESIAN_POINT('Ctrl Pts',(-2.7996015327823,1.,-2.97737733718287));
#66409=CARTESIAN_POINT('Ctrl Pts',(-2.80668968101106,-1.,-2.98046109647241));
#66410=CARTESIAN_POINT('Ctrl Pts',(-2.80668968101106,1.,-2.98046109647241));
#66411=CARTESIAN_POINT('Ctrl Pts',(-2.81380019196286,-1.,-2.98351419779767));
#66412=CARTESIAN_POINT('Ctrl Pts',(-2.81380019196286,1.,-2.98351419779767));
#66413=CARTESIAN_POINT('Ctrl Pts',(-2.82093279065457,-1.,-2.9865368066918));
#66414=CARTESIAN_POINT('Ctrl Pts',(-2.82093279065457,1.,-2.9865368066918));
#66415=CARTESIAN_POINT('Ctrl Pts',(-2.82808728190157,-1.,-2.98952916401446));
#66416=CARTESIAN_POINT('Ctrl Pts',(-2.82808728190157,1.,-2.98952916401446));
#66417=CARTESIAN_POINT('Ctrl Pts',(-2.83526351254248,-1.,-2.99249155170339));
#66418=CARTESIAN_POINT('Ctrl Pts',(-2.83526351254248,1.,-2.99249155170339));
#66419=CARTESIAN_POINT('Ctrl Pts',(-2.84246132984415,-1.,-2.99542425341685));
#66420=CARTESIAN_POINT('Ctrl Pts',(-2.84246132984415,1.,-2.99542425341685));
#66421=CARTESIAN_POINT('Ctrl Pts',(-2.84968053289451,-1.,-2.99832751144925));
#66422=CARTESIAN_POINT('Ctrl Pts',(-2.84968053289451,1.,-2.99832751144925));
#66423=CARTESIAN_POINT('Ctrl Pts',(-2.85692085715686,-1.,-3.00120150796095));
#66424=CARTESIAN_POINT('Ctrl Pts',(-2.85692085715686,1.,-3.00120150796095));
#66425=CARTESIAN_POINT('Ctrl Pts',(-2.86418200833667,-1.,-3.00404638316867));
#66426=CARTESIAN_POINT('Ctrl Pts',(-2.86418200833667,1.,-3.00404638316867));
#66427=CARTESIAN_POINT('Ctrl Pts',(-2.87146368430502,-1.,-3.00686224485784));
#66428=CARTESIAN_POINT('Ctrl Pts',(-2.87146368430502,1.,-3.00686224485784));
#66429=CARTESIAN_POINT('Ctrl Pts',(-2.87876560072727,-1.,-3.00964918108476));
#66430=CARTESIAN_POINT('Ctrl Pts',(-2.87876560072727,1.,-3.00964918108476));
#66431=CARTESIAN_POINT('Ctrl Pts',(-2.8860875170608,-1.,-3.01240727308829));
#66432=CARTESIAN_POINT('Ctrl Pts',(-2.8860875170608,1.,-3.01240727308829));
#66433=CARTESIAN_POINT('Ctrl Pts',(-2.89342925566321,-1.,-3.01513660431928));
#66434=CARTESIAN_POINT('Ctrl Pts',(-2.89342925566321,1.,-3.01513660431928));
#66435=CARTESIAN_POINT('Ctrl Pts',(-2.9007906910105,-1.,-3.01783725121981));
#66436=CARTESIAN_POINT('Ctrl Pts',(-2.9007906910105,1.,-3.01783725121981));
#66437=CARTESIAN_POINT('Ctrl Pts',(-2.90669553302526,-1.,-3.01997487193503));
#66438=CARTESIAN_POINT('Ctrl Pts',(-2.90669553302526,1.,-3.01997487193503));
#66439=CARTESIAN_POINT('Ctrl Pts',(-2.91113297348212,-1.,-3.02156522742431));
#66440=CARTESIAN_POINT('Ctrl Pts',(-2.91113297348212,1.,-3.02156522742431));
#66441=CARTESIAN_POINT('Ctrl Pts',(-2.91409518070399,-1.,-3.02261975104593));
#66442=CARTESIAN_POINT('Ctrl Pts',(-2.91409518070399,1.,-3.02261975104593));
#66443=CARTESIAN_POINT('Ctrl Pts',(-2.91557726271063,-1.,-3.02314558451372));
#66444=CARTESIAN_POINT('Ctrl Pts',(-2.91557726271063,1.,-3.02314558451372));
#66445=CARTESIAN_POINT('',(-2.50410331873176,1.,-2.79140942341258));
#66446=CARTESIAN_POINT('Ctrl Pts',(-2.50410331873176,-1.,-2.79140942341258));
#66447=CARTESIAN_POINT('Ctrl Pts',(-2.50410331873176,-0.666666666666667,
-2.79140942341258));
#66448=CARTESIAN_POINT('Ctrl Pts',(-2.50410331873176,-0.333333333333333,
-2.79140942341258));
#66449=CARTESIAN_POINT('Ctrl Pts',(-2.50410331873176,0.333333333333333,
-2.79140942341258));
#66450=CARTESIAN_POINT('Ctrl Pts',(-2.50410331873176,0.666666666666667,
-2.79140942341258));
#66451=CARTESIAN_POINT('Ctrl Pts',(-2.50410331873176,1.,-2.79140942341258));
#66452=CARTESIAN_POINT('',(-2.91557726271063,1.,-3.02314558451372));
#66453=CARTESIAN_POINT('',(-2.91557726271063,0.,-3.02314558451372));
#66454=CARTESIAN_POINT('Ctrl Pts',(-2.50410331873176,1.,-2.79140942341258));
#66455=CARTESIAN_POINT('Ctrl Pts',(-2.50410700351493,1.,-2.79145823440781));
#66456=CARTESIAN_POINT('Ctrl Pts',(-2.50417932839313,1.,-2.79164172518905));
#66457=CARTESIAN_POINT('Ctrl Pts',(-2.50455968395146,1.,-2.79217568804755));
#66458=CARTESIAN_POINT('Ctrl Pts',(-2.50567182569081,1.,-2.79344192164147));
#66459=CARTESIAN_POINT('Ctrl Pts',(-2.50810555977671,1.,-2.79596878057287));
#66460=CARTESIAN_POINT('Ctrl Pts',(-2.51186983687818,1.,-2.79970585014168));
#66461=CARTESIAN_POINT('Ctrl Pts',(-2.51660190465805,1.,-2.80427363984653));
#66462=CARTESIAN_POINT('Ctrl Pts',(-2.52205778589653,1.,-2.80941521966941));
#66463=CARTESIAN_POINT('Ctrl Pts',(-2.52796388055278,1.,-2.81484379048475));
#66464=CARTESIAN_POINT('Ctrl Pts',(-2.53405679667412,1.,-2.82028550483689));
#66465=CARTESIAN_POINT('Ctrl Pts',(-2.54012272520199,1.,-2.8255216764922));
#66466=CARTESIAN_POINT('Ctrl Pts',(-2.54604736792655,1.,-2.83044254225917));
#66467=CARTESIAN_POINT('Ctrl Pts',(-2.55182152807077,1.,-2.83505269592536));
#66468=CARTESIAN_POINT('Ctrl Pts',(-2.55749952145241,1.,-2.83942515220782));
#66469=CARTESIAN_POINT('Ctrl Pts',(-2.56316920798513,1.,-2.84366802680237));
#66470=CARTESIAN_POINT('Ctrl Pts',(-2.56891984251721,1.,-2.84788893329067));
#66471=CARTESIAN_POINT('Ctrl Pts',(-2.57480482727081,1.,-2.85215360144431));
#66472=CARTESIAN_POINT('Ctrl Pts',(-2.58082875254357,1.,-2.85647171715092));
#66473=CARTESIAN_POINT('Ctrl Pts',(-2.58696770643524,1.,-2.86081999003629));
#66474=CARTESIAN_POINT('Ctrl Pts',(-2.59318160184908,1.,-2.86515629953513));
#66475=CARTESIAN_POINT('Ctrl Pts',(-2.5994287522321,1.,-2.86943633170722));
#66476=CARTESIAN_POINT('Ctrl Pts',(-2.60568177881303,1.,-2.87363176656501));
#66477=CARTESIAN_POINT('Ctrl Pts',(-2.61193507170955,1.,-2.87773881947915));
#66478=CARTESIAN_POINT('Ctrl Pts',(-2.61819596473108,1.,-2.88176821427525));
#66479=CARTESIAN_POINT('Ctrl Pts',(-2.62447947640262,1.,-2.88573922195059));
#66480=CARTESIAN_POINT('Ctrl Pts',(-2.63080195420767,1.,-2.88967244854239));
#66481=CARTESIAN_POINT('Ctrl Pts',(-2.63717442263932,1.,-2.89358228854544));
#66482=CARTESIAN_POINT('Ctrl Pts',(-2.64359851684131,1.,-2.89747231723345));
#66483=CARTESIAN_POINT('Ctrl Pts',(-2.65007017365564,1.,-2.90133950224867));
#66484=CARTESIAN_POINT('Ctrl Pts',(-2.65658188464282,1.,-2.90517678087461));
#66485=CARTESIAN_POINT('Ctrl Pts',(-2.6631254261681,1.,-2.90897617968923));
#66486=CARTESIAN_POINT('Ctrl Pts',(-2.66969458792631,1.,-2.91273193382882));
#66487=CARTESIAN_POINT('Ctrl Pts',(-2.67628728855312,1.,-2.91644290704285));
#66488=CARTESIAN_POINT('Ctrl Pts',(-2.68290409279688,1.,-2.92011090722152));
#66489=CARTESIAN_POINT('Ctrl Pts',(-2.68954721165339,1.,-2.92373955325875));
#66490=CARTESIAN_POINT('Ctrl Pts',(-2.69621932864301,1.,-2.92733294395267));
#66491=CARTESIAN_POINT('Ctrl Pts',(-2.70292247416885,1.,-2.93089438233749));
#66492=CARTESIAN_POINT('Ctrl Pts',(-2.70965695523787,1.,-2.93442516311179));
#66493=CARTESIAN_POINT('Ctrl Pts',(-2.71642190053592,1.,-2.93792519474972));
#66494=CARTESIAN_POINT('Ctrl Pts',(-2.72321571511337,1.,-2.94139351933897));
#66495=CARTESIAN_POINT('Ctrl Pts',(-2.73003657371617,1.,-2.94482887675143));
#66496=CARTESIAN_POINT('Ctrl Pts',(-2.73688288329808,1.,-2.94823023414364));
#66497=CARTESIAN_POINT('Ctrl Pts',(-2.74375379492172,1.,-2.95159737214266));
#66498=CARTESIAN_POINT('Ctrl Pts',(-2.75064903318947,1.,-2.95493069316161));
#66499=CARTESIAN_POINT('Ctrl Pts',(-2.7575686788835,1.,-2.95823097665896));
#66500=CARTESIAN_POINT('Ctrl Pts',(-2.76451296269557,1.,-2.96149914764818));
#66501=CARTESIAN_POINT('Ctrl Pts',(-2.77148206836498,1.,-2.96473605585583));
#66502=CARTESIAN_POINT('Ctrl Pts',(-2.7784758954285,1.,-2.96794221043036));
#66503=CARTESIAN_POINT('Ctrl Pts',(-2.78549409123769,1.,-2.97111781461465));
#66504=CARTESIAN_POINT('Ctrl Pts',(-2.79253615718248,1.,-2.9742628834758));
#66505=CARTESIAN_POINT('Ctrl Pts',(-2.7996015327823,1.,-2.97737733718287));
#66506=CARTESIAN_POINT('Ctrl Pts',(-2.80668968101106,1.,-2.98046109647241));
#66507=CARTESIAN_POINT('Ctrl Pts',(-2.81380019196286,1.,-2.98351419779767));
#66508=CARTESIAN_POINT('Ctrl Pts',(-2.82093279065457,1.,-2.9865368066918));
#66509=CARTESIAN_POINT('Ctrl Pts',(-2.82808728190157,1.,-2.98952916401446));
#66510=CARTESIAN_POINT('Ctrl Pts',(-2.83526351254248,1.,-2.99249155170339));
#66511=CARTESIAN_POINT('Ctrl Pts',(-2.84246132984415,1.,-2.99542425341685));
#66512=CARTESIAN_POINT('Ctrl Pts',(-2.84968053289451,1.,-2.99832751144925));
#66513=CARTESIAN_POINT('Ctrl Pts',(-2.85692085715686,1.,-3.00120150796095));
#66514=CARTESIAN_POINT('Ctrl Pts',(-2.86418200833667,1.,-3.00404638316867));
#66515=CARTESIAN_POINT('Ctrl Pts',(-2.87146368430502,1.,-3.00686224485784));
#66516=CARTESIAN_POINT('Ctrl Pts',(-2.87876560072727,1.,-3.00964918108476));
#66517=CARTESIAN_POINT('Ctrl Pts',(-2.8860875170608,1.,-3.01240727308829));
#66518=CARTESIAN_POINT('Ctrl Pts',(-2.89342925566321,1.,-3.01513660431928));
#66519=CARTESIAN_POINT('Ctrl Pts',(-2.9007906910105,1.,-3.01783725121981));
#66520=CARTESIAN_POINT('Ctrl Pts',(-2.90669553302526,1.,-3.01997487193503));
#66521=CARTESIAN_POINT('Ctrl Pts',(-2.91113297348212,1.,-3.02156522742431));
#66522=CARTESIAN_POINT('Ctrl Pts',(-2.91409518070399,1.,-3.02261975104593));
#66523=CARTESIAN_POINT('Ctrl Pts',(-2.91557726271063,1.,-3.02314558451372));
#66524=CARTESIAN_POINT('Origin',(-2.91557726271063,0.,-3.02314558451372));
#66525=CARTESIAN_POINT('',(-3.02314558451372,1.,-2.91557726271063));
#66526=CARTESIAN_POINT('Origin',(0.,0.,0.));
#66527=CARTESIAN_POINT('',(-2.36531447826213,1.,-2.90994629141562));
#66528=CARTESIAN_POINT('Origin',(0.,1.,0.));
#66529=CARTESIAN_POINT('Ctrl Pts',(-2.36531447826213,1.,-2.90994629141562));
#66530=CARTESIAN_POINT('Ctrl Pts',(-2.36531447826213,0.666666666666667,
-2.90994629141562));
#66531=CARTESIAN_POINT('Ctrl Pts',(-2.36531447826213,0.333333333333333,
-2.90994629141562));
#66532=CARTESIAN_POINT('Ctrl Pts',(-2.36531447826213,-0.333333333333333,
-2.90994629141562));
#66533=CARTESIAN_POINT('Ctrl Pts',(-2.36531447826213,-0.666666666666667,
-2.90994629141562));
#66534=CARTESIAN_POINT('Ctrl Pts',(-2.36531447826213,-1.,-2.90994629141562));
#66535=CARTESIAN_POINT('Ctrl Pts',(-2.52982887637028,-1.,-3.35260583073571));
#66536=CARTESIAN_POINT('Ctrl Pts',(-2.52982887637028,1.,-3.35260583073571));
#66537=CARTESIAN_POINT('Ctrl Pts',(-2.52954136549357,-1.,-3.35105973714426));
#66538=CARTESIAN_POINT('Ctrl Pts',(-2.52954136549357,1.,-3.35105973714426));
#66539=CARTESIAN_POINT('Ctrl Pts',(-2.5289632161143,-1.,-3.34796903577628));
#66540=CARTESIAN_POINT('Ctrl Pts',(-2.5289632161143,1.,-3.34796903577628));
#66541=CARTESIAN_POINT('Ctrl Pts',(-2.52808660916879,-1.,-3.34333744117093));
#66542=CARTESIAN_POINT('Ctrl Pts',(-2.52808660916879,1.,-3.34333744117093));
#66543=CARTESIAN_POINT('Ctrl Pts',(-2.52689902691551,-1.,-3.33717090000955));
#66544=CARTESIAN_POINT('Ctrl Pts',(-2.52689902691551,1.,-3.33717090000955));
#66545=CARTESIAN_POINT('Ctrl Pts',(-2.52538321165774,-1.,-3.32947762189049));
#66546=CARTESIAN_POINT('Ctrl Pts',(-2.52538321165774,1.,-3.32947762189049));
#66547=CARTESIAN_POINT('Ctrl Pts',(-2.52383598396878,-1.,-3.32179931079521));
#66548=CARTESIAN_POINT('Ctrl Pts',(-2.52383598396878,1.,-3.32179931079521));
#66549=CARTESIAN_POINT('Ctrl Pts',(-2.52225724871375,-1.,-3.31413607874727));
#66550=CARTESIAN_POINT('Ctrl Pts',(-2.52225724871375,1.,-3.31413607874727));
#66551=CARTESIAN_POINT('Ctrl Pts',(-2.52064689568167,-1.,-3.30648808814986));
#66552=CARTESIAN_POINT('Ctrl Pts',(-2.52064689568167,1.,-3.30648808814986));
#66553=CARTESIAN_POINT('Ctrl Pts',(-2.51900480700548,-1.,-3.29885556387661));
#66554=CARTESIAN_POINT('Ctrl Pts',(-2.51900480700548,1.,-3.29885556387661));
#66555=CARTESIAN_POINT('Ctrl Pts',(-2.51733085123316,-1.,-3.2912387729863));
#66556=CARTESIAN_POINT('Ctrl Pts',(-2.51733085123316,1.,-3.2912387729863));
#66557=CARTESIAN_POINT('Ctrl Pts',(-2.51562487464215,-1.,-3.28363799702583));
#66558=CARTESIAN_POINT('Ctrl Pts',(-2.51562487464215,1.,-3.28363799702583));
#66559=CARTESIAN_POINT('Ctrl Pts',(-2.51388669270329,-1.,-3.27605350473048));
#66560=CARTESIAN_POINT('Ctrl Pts',(-2.51388669270329,1.,-3.27605350473048));
#66561=CARTESIAN_POINT('Ctrl Pts',(-2.51211608411539,-1.,-3.26848552888271));
#66562=CARTESIAN_POINT('Ctrl Pts',(-2.51211608411539,1.,-3.26848552888271));
#66563=CARTESIAN_POINT('Ctrl Pts',(-2.51031277813697,-1.,-3.26093423001716));
#66564=CARTESIAN_POINT('Ctrl Pts',(-2.51031277813697,1.,-3.26093423001716));
#66565=CARTESIAN_POINT('Ctrl Pts',(-2.50847647070936,-1.,-3.25339971461265));
#66566=CARTESIAN_POINT('Ctrl Pts',(-2.50847647070936,1.,-3.25339971461265));
#66567=CARTESIAN_POINT('Ctrl Pts',(-2.50660685940645,-1.,-3.24588208984042));
#66568=CARTESIAN_POINT('Ctrl Pts',(-2.50660685940645,1.,-3.24588208984042));
#66569=CARTESIAN_POINT('Ctrl Pts',(-2.50470367580078,-1.,-3.23838151080383));
#66570=CARTESIAN_POINT('Ctrl Pts',(-2.50470367580078,1.,-3.23838151080383));
#66571=CARTESIAN_POINT('Ctrl Pts',(-2.50276671338074,-1.,-3.23089822320596));
#66572=CARTESIAN_POINT('Ctrl Pts',(-2.50276671338074,1.,-3.23089822320596));
#66573=CARTESIAN_POINT('Ctrl Pts',(-2.5007958720187,-1.,-3.22343262620387));
#66574=CARTESIAN_POINT('Ctrl Pts',(-2.5007958720187,1.,-3.22343262620387));
#66575=CARTESIAN_POINT('Ctrl Pts',(-2.49879114599293,-1.,-3.21598526261157));
#66576=CARTESIAN_POINT('Ctrl Pts',(-2.49879114599293,1.,-3.21598526261157));
#66577=CARTESIAN_POINT('Ctrl Pts',(-2.49675252647298,-1.,-3.2085566984974));
#66578=CARTESIAN_POINT('Ctrl Pts',(-2.49675252647298,1.,-3.2085566984974));
#66579=CARTESIAN_POINT('Ctrl Pts',(-2.49467992057726,-1.,-3.20114742397549));
#66580=CARTESIAN_POINT('Ctrl Pts',(-2.49467992057726,1.,-3.20114742397549));
#66581=CARTESIAN_POINT('Ctrl Pts',(-2.4925730723986,-1.,-3.19375775555814));
#66582=CARTESIAN_POINT('Ctrl Pts',(-2.4925730723986,1.,-3.19375775555814));
#66583=CARTESIAN_POINT('Ctrl Pts',(-2.49043146334095,-1.,-3.18638771282315));
#66584=CARTESIAN_POINT('Ctrl Pts',(-2.49043146334095,1.,-3.18638771282315));
#66585=CARTESIAN_POINT('Ctrl Pts',(-2.48825428288243,-1.,-3.17903698136679));
#66586=CARTESIAN_POINT('Ctrl Pts',(-2.48825428288243,1.,-3.17903698136679));
#66587=CARTESIAN_POINT('Ctrl Pts',(-2.48604065348619,-1.,-3.17170518863357));
#66588=CARTESIAN_POINT('Ctrl Pts',(-2.48604065348619,1.,-3.17170518863357));
#66589=CARTESIAN_POINT('Ctrl Pts',(-2.48378981792739,-1.,-3.16439213290181));
#66590=CARTESIAN_POINT('Ctrl Pts',(-2.48378981792739,1.,-3.16439213290181));
#66591=CARTESIAN_POINT('Ctrl Pts',(-2.48150133566568,-1.,-3.15709802322735));
#66592=CARTESIAN_POINT('Ctrl Pts',(-2.48150133566568,1.,-3.15709802322735));
#66593=CARTESIAN_POINT('Ctrl Pts',(-2.47917529057016,-1.,-3.14982373241335));
#66594=CARTESIAN_POINT('Ctrl Pts',(-2.47917529057016,1.,-3.14982373241335));
#66595=CARTESIAN_POINT('Ctrl Pts',(-2.47681245356095,-1.,-3.14257099546531));
#66596=CARTESIAN_POINT('Ctrl Pts',(-2.47681245356095,1.,-3.14257099546531));
#66597=CARTESIAN_POINT('Ctrl Pts',(-2.47441378371923,-1.,-3.13534181229282));
#66598=CARTESIAN_POINT('Ctrl Pts',(-2.47441378371923,1.,-3.13534181229282));
#66599=CARTESIAN_POINT('Ctrl Pts',(-2.47197997765868,-1.,-3.12813790805948));
#66600=CARTESIAN_POINT('Ctrl Pts',(-2.47197997765868,1.,-3.12813790805948));
#66601=CARTESIAN_POINT('Ctrl Pts',(-2.4695109894747,-1.,-3.12096015766984));
#66602=CARTESIAN_POINT('Ctrl Pts',(-2.4695109894747,1.,-3.12096015766984));
#66603=CARTESIAN_POINT('Ctrl Pts',(-2.46700558843507,-1.,-3.11380805536124));
#66604=CARTESIAN_POINT('Ctrl Pts',(-2.46700558843507,1.,-3.11380805536124));
#66605=CARTESIAN_POINT('Ctrl Pts',(-2.46446082979645,-1.,-3.10667907901981));
#66606=CARTESIAN_POINT('Ctrl Pts',(-2.46446082979645,1.,-3.10667907901981));
#66607=CARTESIAN_POINT('Ctrl Pts',(-2.4618730850188,-1.,-3.09956993697048));
#66608=CARTESIAN_POINT('Ctrl Pts',(-2.4618730850188,1.,-3.09956993697048));
#66609=CARTESIAN_POINT('Ctrl Pts',(-2.45923912563875,-1.,-3.09247787931881));
#66610=CARTESIAN_POINT('Ctrl Pts',(-2.45923912563875,1.,-3.09247787931881));
#66611=CARTESIAN_POINT('Ctrl Pts',(-2.45655725437037,-1.,-3.08540206545313));
#66612=CARTESIAN_POINT('Ctrl Pts',(-2.45655725437037,1.,-3.08540206545313));
#66613=CARTESIAN_POINT('Ctrl Pts',(-2.45382826787795,-1.,-3.07834472886145));
#66614=CARTESIAN_POINT('Ctrl Pts',(-2.45382826787795,1.,-3.07834472886145));
#66615=CARTESIAN_POINT('Ctrl Pts',(-2.45105688854432,-1.,-3.0713129052131));
#66616=CARTESIAN_POINT('Ctrl Pts',(-2.45105688854432,1.,-3.0713129052131));
#66617=CARTESIAN_POINT('Ctrl Pts',(-2.44824970516558,-1.,-3.06431596421422));
#66618=CARTESIAN_POINT('Ctrl Pts',(-2.44824970516558,1.,-3.06431596421422));
#66619=CARTESIAN_POINT('Ctrl Pts',(-2.44541251892568,-1.,-3.05736242671521));
#66620=CARTESIAN_POINT('Ctrl Pts',(-2.44541251892568,1.,-3.05736242671521));
#66621=CARTESIAN_POINT('Ctrl Pts',(-2.44254768923109,-1.,-3.05045678021509));
#66622=CARTESIAN_POINT('Ctrl Pts',(-2.44254768923109,1.,-3.05045678021509));
#66623=CARTESIAN_POINT('Ctrl Pts',(-2.43965194061849,-1.,-3.04359685040545));
#66624=CARTESIAN_POINT('Ctrl Pts',(-2.43965194061849,1.,-3.04359685040545));
#66625=CARTESIAN_POINT('Ctrl Pts',(-2.43671278042394,-1.,-3.03676949672797));
#66626=CARTESIAN_POINT('Ctrl Pts',(-2.43671278042394,1.,-3.03676949672797));
#66627=CARTESIAN_POINT('Ctrl Pts',(-2.43371241361462,-1.,-3.02995534946946));
#66628=CARTESIAN_POINT('Ctrl Pts',(-2.43371241361462,1.,-3.02995534946946));
#66629=CARTESIAN_POINT('Ctrl Pts',(-2.43063415586615,-1.,-3.02313656035977));
#66630=CARTESIAN_POINT('Ctrl Pts',(-2.43063415586615,1.,-3.02313656035977));
#66631=CARTESIAN_POINT('Ctrl Pts',(-2.4274685626416,-1.,-3.01630420830494));
#66632=CARTESIAN_POINT('Ctrl Pts',(-2.4274685626416,1.,-3.01630420830494));
#66633=CARTESIAN_POINT('Ctrl Pts',(-2.42421849439625,-1.,-3.00946442616674));
#66634=CARTESIAN_POINT('Ctrl Pts',(-2.42421849439625,1.,-3.00946442616674));
#66635=CARTESIAN_POINT('Ctrl Pts',(-2.42090763946812,-1.,-3.00264868586038));
#66636=CARTESIAN_POINT('Ctrl Pts',(-2.42090763946812,1.,-3.00264868586038));
#66637=CARTESIAN_POINT('Ctrl Pts',(-2.4175732450056,-1.,-2.99590509293561));
#66638=CARTESIAN_POINT('Ctrl Pts',(-2.4175732450056,1.,-2.99590509293561));
#66639=CARTESIAN_POINT('Ctrl Pts',(-2.4142506419963,-1.,-2.98927983005851));
#66640=CARTESIAN_POINT('Ctrl Pts',(-2.4142506419963,1.,-2.98927983005851));
#66641=CARTESIAN_POINT('Ctrl Pts',(-2.41095909342591,-1.,-2.98280015815132));
#66642=CARTESIAN_POINT('Ctrl Pts',(-2.41095909342591,1.,-2.98280015815132));
#66643=CARTESIAN_POINT('Ctrl Pts',(-2.40768975073691,-1.,-2.97646002822395));
#66644=CARTESIAN_POINT('Ctrl Pts',(-2.40768975073691,1.,-2.97646002822395));
#66645=CARTESIAN_POINT('Ctrl Pts',(-2.40438604734848,-1.,-2.97019641312272));
#66646=CARTESIAN_POINT('Ctrl Pts',(-2.40438604734848,1.,-2.97019641312272));
#66647=CARTESIAN_POINT('Ctrl Pts',(-2.40095565711535,-1.,-2.96390432240181));
#66648=CARTESIAN_POINT('Ctrl Pts',(-2.40095565711535,1.,-2.96390432240181));
#66649=CARTESIAN_POINT('Ctrl Pts',(-2.39730553974412,-1.,-2.95748006482811));
#66650=CARTESIAN_POINT('Ctrl Pts',(-2.39730553974412,1.,-2.95748006482811));
#66651=CARTESIAN_POINT('Ctrl Pts',(-2.39337207631613,-1.,-2.95085857128372));
#66652=CARTESIAN_POINT('Ctrl Pts',(-2.39337207631613,1.,-2.95085857128372));
#66653=CARTESIAN_POINT('Ctrl Pts',(-2.38914929090806,-1.,-2.94404820669135));
#66654=CARTESIAN_POINT('Ctrl Pts',(-2.38914929090806,1.,-2.94404820669135));
#66655=CARTESIAN_POINT('Ctrl Pts',(-2.38472771516476,-1.,-2.93717903280599));
#66656=CARTESIAN_POINT('Ctrl Pts',(-2.38472771516476,1.,-2.93717903280599));
#66657=CARTESIAN_POINT('Ctrl Pts',(-2.3802898958232,-1.,-2.93049643640517));
#66658=CARTESIAN_POINT('Ctrl Pts',(-2.3802898958232,1.,-2.93049643640517));
#66659=CARTESIAN_POINT('Ctrl Pts',(-2.37606510524271,-1.,-2.92430340582912));
#66660=CARTESIAN_POINT('Ctrl Pts',(-2.37606510524271,1.,-2.92430340582912));
#66661=CARTESIAN_POINT('Ctrl Pts',(-2.37229381109939,-1.,-2.9189150379156));
#66662=CARTESIAN_POINT('Ctrl Pts',(-2.37229381109939,1.,-2.9189150379156));
#66663=CARTESIAN_POINT('Ctrl Pts',(-2.36919161373074,-1.,-2.91461249883016));
#66664=CARTESIAN_POINT('Ctrl Pts',(-2.36919161373074,1.,-2.91461249883016));
#66665=CARTESIAN_POINT('Ctrl Pts',(-2.36690501170317,-1.,-2.9115863784165));
#66666=CARTESIAN_POINT('Ctrl Pts',(-2.36690501170317,1.,-2.9115863784165));
#66667=CARTESIAN_POINT('Ctrl Pts',(-2.36578327194396,-1.,-2.91025813829606));
#66668=CARTESIAN_POINT('Ctrl Pts',(-2.36578327194396,1.,-2.91025813829606));
#66669=CARTESIAN_POINT('Ctrl Pts',(-2.36535052956704,-1.,-2.90989022547738));
#66670=CARTESIAN_POINT('Ctrl Pts',(-2.36535052956704,1.,-2.90989022547738));
#66671=CARTESIAN_POINT('Ctrl Pts',(-2.36524348105023,-1.,-2.90992398626098));
#66672=CARTESIAN_POINT('Ctrl Pts',(-2.36524348105023,1.,-2.90992398626098));
#66673=CARTESIAN_POINT('Ctrl Pts',(-2.36523532225181,-1.,-2.91001063062876));
#66674=CARTESIAN_POINT('Ctrl Pts',(-2.36523532225181,1.,-2.91001063062876));
#66675=CARTESIAN_POINT('',(-2.52982887637028,1.,-3.35260583073571));
#66676=CARTESIAN_POINT('Ctrl Pts',(-2.52982887637028,1.,-3.35260583073571));
#66677=CARTESIAN_POINT('Ctrl Pts',(-2.52954136549357,1.,-3.35105973714426));
#66678=CARTESIAN_POINT('Ctrl Pts',(-2.5289632161143,1.,-3.34796903577628));
#66679=CARTESIAN_POINT('Ctrl Pts',(-2.52808660916879,1.,-3.34333744117093));
#66680=CARTESIAN_POINT('Ctrl Pts',(-2.52689902691551,1.,-3.33717090000955));
#66681=CARTESIAN_POINT('Ctrl Pts',(-2.52538321165774,1.,-3.32947762189049));
#66682=CARTESIAN_POINT('Ctrl Pts',(-2.52383598396878,1.,-3.32179931079521));
#66683=CARTESIAN_POINT('Ctrl Pts',(-2.52225724871375,1.,-3.31413607874727));
#66684=CARTESIAN_POINT('Ctrl Pts',(-2.52064689568167,1.,-3.30648808814986));
#66685=CARTESIAN_POINT('Ctrl Pts',(-2.51900480700548,1.,-3.29885556387661));
#66686=CARTESIAN_POINT('Ctrl Pts',(-2.51733085123316,1.,-3.2912387729863));
#66687=CARTESIAN_POINT('Ctrl Pts',(-2.51562487464215,1.,-3.28363799702583));
#66688=CARTESIAN_POINT('Ctrl Pts',(-2.51388669270329,1.,-3.27605350473048));
#66689=CARTESIAN_POINT('Ctrl Pts',(-2.51211608411539,1.,-3.26848552888271));
#66690=CARTESIAN_POINT('Ctrl Pts',(-2.51031277813697,1.,-3.26093423001716));
#66691=CARTESIAN_POINT('Ctrl Pts',(-2.50847647070936,1.,-3.25339971461265));
#66692=CARTESIAN_POINT('Ctrl Pts',(-2.50660685940645,1.,-3.24588208984042));
#66693=CARTESIAN_POINT('Ctrl Pts',(-2.50470367580078,1.,-3.23838151080383));
#66694=CARTESIAN_POINT('Ctrl Pts',(-2.50276671338074,1.,-3.23089822320596));
#66695=CARTESIAN_POINT('Ctrl Pts',(-2.5007958720187,1.,-3.22343262620387));
#66696=CARTESIAN_POINT('Ctrl Pts',(-2.49879114599293,1.,-3.21598526261157));
#66697=CARTESIAN_POINT('Ctrl Pts',(-2.49675252647298,1.,-3.2085566984974));
#66698=CARTESIAN_POINT('Ctrl Pts',(-2.49467992057726,1.,-3.20114742397549));
#66699=CARTESIAN_POINT('Ctrl Pts',(-2.4925730723986,1.,-3.19375775555814));
#66700=CARTESIAN_POINT('Ctrl Pts',(-2.49043146334095,1.,-3.18638771282315));
#66701=CARTESIAN_POINT('Ctrl Pts',(-2.48825428288243,1.,-3.17903698136679));
#66702=CARTESIAN_POINT('Ctrl Pts',(-2.48604065348619,1.,-3.17170518863357));
#66703=CARTESIAN_POINT('Ctrl Pts',(-2.48378981792739,1.,-3.16439213290181));
#66704=CARTESIAN_POINT('Ctrl Pts',(-2.48150133566568,1.,-3.15709802322735));
#66705=CARTESIAN_POINT('Ctrl Pts',(-2.47917529057016,1.,-3.14982373241335));
#66706=CARTESIAN_POINT('Ctrl Pts',(-2.47681245356095,1.,-3.14257099546531));
#66707=CARTESIAN_POINT('Ctrl Pts',(-2.47441378371923,1.,-3.13534181229282));
#66708=CARTESIAN_POINT('Ctrl Pts',(-2.47197997765868,1.,-3.12813790805948));
#66709=CARTESIAN_POINT('Ctrl Pts',(-2.4695109894747,1.,-3.12096015766984));
#66710=CARTESIAN_POINT('Ctrl Pts',(-2.46700558843507,1.,-3.11380805536124));
#66711=CARTESIAN_POINT('Ctrl Pts',(-2.46446082979645,1.,-3.10667907901981));
#66712=CARTESIAN_POINT('Ctrl Pts',(-2.4618730850188,1.,-3.09956993697048));
#66713=CARTESIAN_POINT('Ctrl Pts',(-2.45923912563875,1.,-3.09247787931881));
#66714=CARTESIAN_POINT('Ctrl Pts',(-2.45655725437037,1.,-3.08540206545313));
#66715=CARTESIAN_POINT('Ctrl Pts',(-2.45382826787795,1.,-3.07834472886145));
#66716=CARTESIAN_POINT('Ctrl Pts',(-2.45105688854432,1.,-3.0713129052131));
#66717=CARTESIAN_POINT('Ctrl Pts',(-2.44824970516558,1.,-3.06431596421422));
#66718=CARTESIAN_POINT('Ctrl Pts',(-2.44541251892568,1.,-3.05736242671521));
#66719=CARTESIAN_POINT('Ctrl Pts',(-2.44254768923109,1.,-3.05045678021509));
#66720=CARTESIAN_POINT('Ctrl Pts',(-2.43965194061849,1.,-3.04359685040545));
#66721=CARTESIAN_POINT('Ctrl Pts',(-2.43671278042394,1.,-3.03676949672797));
#66722=CARTESIAN_POINT('Ctrl Pts',(-2.43371241361462,1.,-3.02995534946946));
#66723=CARTESIAN_POINT('Ctrl Pts',(-2.43063415586615,1.,-3.02313656035977));
#66724=CARTESIAN_POINT('Ctrl Pts',(-2.4274685626416,1.,-3.01630420830494));
#66725=CARTESIAN_POINT('Ctrl Pts',(-2.42421849439625,1.,-3.00946442616674));
#66726=CARTESIAN_POINT('Ctrl Pts',(-2.42090763946812,1.,-3.00264868586038));
#66727=CARTESIAN_POINT('Ctrl Pts',(-2.4175732450056,1.,-2.99590509293561));
#66728=CARTESIAN_POINT('Ctrl Pts',(-2.4142506419963,1.,-2.98927983005851));
#66729=CARTESIAN_POINT('Ctrl Pts',(-2.41095909342591,1.,-2.98280015815132));
#66730=CARTESIAN_POINT('Ctrl Pts',(-2.40768975073691,1.,-2.97646002822395));
#66731=CARTESIAN_POINT('Ctrl Pts',(-2.40438604734848,1.,-2.97019641312272));
#66732=CARTESIAN_POINT('Ctrl Pts',(-2.40095565711535,1.,-2.96390432240181));
#66733=CARTESIAN_POINT('Ctrl Pts',(-2.39730553974412,1.,-2.95748006482811));
#66734=CARTESIAN_POINT('Ctrl Pts',(-2.39337207631613,1.,-2.95085857128372));
#66735=CARTESIAN_POINT('Ctrl Pts',(-2.38914929090806,1.,-2.94404820669135));
#66736=CARTESIAN_POINT('Ctrl Pts',(-2.38472771516476,1.,-2.93717903280599));
#66737=CARTESIAN_POINT('Ctrl Pts',(-2.3802898958232,1.,-2.93049643640517));
#66738=CARTESIAN_POINT('Ctrl Pts',(-2.37606510524271,1.,-2.92430340582912));
#66739=CARTESIAN_POINT('Ctrl Pts',(-2.37229381109939,1.,-2.9189150379156));
#66740=CARTESIAN_POINT('Ctrl Pts',(-2.36919161373074,1.,-2.91461249883016));
#66741=CARTESIAN_POINT('Ctrl Pts',(-2.36707658451709,1.,-2.91181344022628));
#66742=CARTESIAN_POINT('Ctrl Pts',(-2.36599991765853,1.,-2.91051690822262));
#66743=CARTESIAN_POINT('Ctrl Pts',(-2.36553202948741,1.,-2.9100577052777));
#66744=CARTESIAN_POINT('Ctrl Pts',(-2.3653621118858,1.,-2.90995756655559));
#66745=CARTESIAN_POINT('Ctrl Pts',(-2.36531447826213,1.,-2.90994629141563));
#66746=CARTESIAN_POINT('',(-2.52982887637028,0.,-3.35260583073571));
#66747=CARTESIAN_POINT('Ctrl Pts',(-2.03668666247593,-1.,-3.1487152044751));
#66748=CARTESIAN_POINT('Ctrl Pts',(-2.03668666247593,1.,-3.1487152044751));
#66749=CARTESIAN_POINT('Ctrl Pts',(-2.03660173757879,-1.,-3.14869618937258));
#66750=CARTESIAN_POINT('Ctrl Pts',(-2.03660173757879,1.,-3.14869618937258));
#66751=CARTESIAN_POINT('Ctrl Pts',(-2.03653654935592,-1.,-3.14878756590812));
#66752=CARTESIAN_POINT('Ctrl Pts',(-2.03653654935592,1.,-3.14878756590812));
#66753=CARTESIAN_POINT('Ctrl Pts',(-2.03675273049189,-1.,-3.14931281968048));
#66754=CARTESIAN_POINT('Ctrl Pts',(-2.03675273049189,1.,-3.14931281968048));
#66755=CARTESIAN_POINT('Ctrl Pts',(-2.03766932526445,-1.,-3.15079010635742));
#66756=CARTESIAN_POINT('Ctrl Pts',(-2.03766932526445,1.,-3.15079010635742));
#66757=CARTESIAN_POINT('Ctrl Pts',(-2.03984073791519,-1.,-3.15389991674792));
#66758=CARTESIAN_POINT('Ctrl Pts',(-2.03984073791519,1.,-3.15389991674792));
#66759=CARTESIAN_POINT('Ctrl Pts',(-2.04297406404027,-1.,-3.15817983946367));
#66760=CARTESIAN_POINT('Ctrl Pts',(-2.04297406404027,1.,-3.15817983946367));
#66761=CARTESIAN_POINT('Ctrl Pts',(-2.04693331247446,-1.,-3.16343165058912));
#66762=CARTESIAN_POINT('Ctrl Pts',(-2.04693331247446,1.,-3.16343165058912));
#66763=CARTESIAN_POINT('Ctrl Pts',(-2.05151770247233,-1.,-3.16936341689527));
#66764=CARTESIAN_POINT('Ctrl Pts',(-2.05151770247233,1.,-3.16936341689527));
#66765=CARTESIAN_POINT('Ctrl Pts',(-2.05650186773132,-1.,-3.17564906975371));
#66766=CARTESIAN_POINT('Ctrl Pts',(-2.05650186773132,1.,-3.17564906975371));
#66767=CARTESIAN_POINT('Ctrl Pts',(-2.06166849827101,-1.,-3.18197692964614));
#66768=CARTESIAN_POINT('Ctrl Pts',(-2.06166849827101,1.,-3.18197692964614));
#66769=CARTESIAN_POINT('Ctrl Pts',(-2.06684062744112,-1.,-3.18809755562368));
#66770=CARTESIAN_POINT('Ctrl Pts',(-2.06684062744112,1.,-3.18809755562368));
#66771=CARTESIAN_POINT('Ctrl Pts',(-2.07192253497857,-1.,-3.19388465568252));
#66772=CARTESIAN_POINT('Ctrl Pts',(-2.07192253497857,1.,-3.19388465568252));
#66773=CARTESIAN_POINT('Ctrl Pts',(-2.07690441870722,-1.,-3.19934132836019));
#66774=CARTESIAN_POINT('Ctrl Pts',(-2.07690441870722,1.,-3.19934132836019));
#66775=CARTESIAN_POINT('Ctrl Pts',(-2.08182850370878,-1.,-3.2045481863073));
#66776=CARTESIAN_POINT('Ctrl Pts',(-2.08182850370878,1.,-3.2045481863073));
#66777=CARTESIAN_POINT('Ctrl Pts',(-2.08676465517455,-1.,-3.20962575845463));
#66778=CARTESIAN_POINT('Ctrl Pts',(-2.08676465517455,1.,-3.20962575845463));
#66779=CARTESIAN_POINT('Ctrl Pts',(-2.09178419460443,-1.,-3.21469429601654));
#66780=CARTESIAN_POINT('Ctrl Pts',(-2.09178419460443,1.,-3.21469429601654));
#66781=CARTESIAN_POINT('Ctrl Pts',(-2.09692958434895,-1.,-3.21982707347009));
#66782=CARTESIAN_POINT('Ctrl Pts',(-2.09692958434895,1.,-3.21982707347009));
#66783=CARTESIAN_POINT('Ctrl Pts',(-2.10220384298492,-1.,-3.22503437553434));
#66784=CARTESIAN_POINT('Ctrl Pts',(-2.10220384298492,1.,-3.22503437553434));
#66785=CARTESIAN_POINT('Ctrl Pts',(-2.10758699642451,-1.,-3.23028945793289));
#66786=CARTESIAN_POINT('Ctrl Pts',(-2.10758699642451,1.,-3.23028945793289));
#66787=CARTESIAN_POINT('Ctrl Pts',(-2.11304604021773,-1.,-3.23554444767099));
#66788=CARTESIAN_POINT('Ctrl Pts',(-2.11304604021773,1.,-3.23554444767099));
#66789=CARTESIAN_POINT('Ctrl Pts',(-2.11854673326979,-1.,-3.24074905517293));
#66790=CARTESIAN_POINT('Ctrl Pts',(-2.11854673326979,1.,-3.24074905517293));
#66791=CARTESIAN_POINT('Ctrl Pts',(-2.12406646410962,-1.,-3.24587102613376));
#66792=CARTESIAN_POINT('Ctrl Pts',(-2.12406646410962,1.,-3.24587102613376));
#66793=CARTESIAN_POINT('Ctrl Pts',(-2.12960028396832,-1.,-3.25090574494028));
#66794=CARTESIAN_POINT('Ctrl Pts',(-2.12960028396832,1.,-3.25090574494028));
#66795=CARTESIAN_POINT('Ctrl Pts',(-2.13515375878803,-1.,-3.25586495065054));
#66796=CARTESIAN_POINT('Ctrl Pts',(-2.13515375878803,1.,-3.25586495065054));
#66797=CARTESIAN_POINT('Ctrl Pts',(-2.14073870754264,-1.,-3.26077002641879));
#66798=CARTESIAN_POINT('Ctrl Pts',(-2.14073870754264,1.,-3.26077002641879));
#66799=CARTESIAN_POINT('Ctrl Pts',(-2.1463680529566,-1.,-3.26564388189759));
#66800=CARTESIAN_POINT('Ctrl Pts',(-2.1463680529566,1.,-3.26564388189759));
#66801=CARTESIAN_POINT('Ctrl Pts',(-2.15205043199808,-1.,-3.27050245897228));
#66802=CARTESIAN_POINT('Ctrl Pts',(-2.15205043199808,1.,-3.27050245897228));
#66803=CARTESIAN_POINT('Ctrl Pts',(-2.15778690038347,-1.,-3.27534954469187));
#66804=CARTESIAN_POINT('Ctrl Pts',(-2.15778690038347,1.,-3.27534954469187));
#66805=CARTESIAN_POINT('Ctrl Pts',(-2.16357391934425,-1.,-3.280181508414));
#66806=CARTESIAN_POINT('Ctrl Pts',(-2.16357391934425,1.,-3.280181508414));
#66807=CARTESIAN_POINT('Ctrl Pts',(-2.16940517773455,-1.,-3.28499019979724));
#66808=CARTESIAN_POINT('Ctrl Pts',(-2.16940517773455,1.,-3.28499019979724));
#66809=CARTESIAN_POINT('Ctrl Pts',(-2.17527380048423,-1.,-3.28976645712568));
#66810=CARTESIAN_POINT('Ctrl Pts',(-2.17527380048423,1.,-3.28976645712568));
#66811=CARTESIAN_POINT('Ctrl Pts',(-2.18117455557065,-1.,-3.2945036150049));
#66812=CARTESIAN_POINT('Ctrl Pts',(-2.18117455557065,1.,-3.2945036150049));
#66813=CARTESIAN_POINT('Ctrl Pts',(-2.18710556500327,-1.,-3.29920022557639));
#66814=CARTESIAN_POINT('Ctrl Pts',(-2.18710556500327,1.,-3.29920022557639));
#66815=CARTESIAN_POINT('Ctrl Pts',(-2.19306710376111,-1.,-3.30385816281831));
#66816=CARTESIAN_POINT('Ctrl Pts',(-2.19306710376111,1.,-3.30385816281831));
#66817=CARTESIAN_POINT('Ctrl Pts',(-2.19906078949923,-1.,-3.30848134694595));
#66818=CARTESIAN_POINT('Ctrl Pts',(-2.19906078949923,1.,-3.30848134694595));
#66819=CARTESIAN_POINT('Ctrl Pts',(-2.20508863150607,-1.,-3.31307424608949));
#66820=CARTESIAN_POINT('Ctrl Pts',(-2.20508863150607,1.,-3.31307424608949));
#66821=CARTESIAN_POINT('Ctrl Pts',(-2.21115211847875,-1.,-3.31764044024235));
#66822=CARTESIAN_POINT('Ctrl Pts',(-2.21115211847875,1.,-3.31764044024235));
#66823=CARTESIAN_POINT('Ctrl Pts',(-2.21725135110898,-1.,-3.32218125618968));
#66824=CARTESIAN_POINT('Ctrl Pts',(-2.21725135110898,1.,-3.32218125618968));
#66825=CARTESIAN_POINT('Ctrl Pts',(-2.22338548312772,-1.,-3.3266964672289));
#66826=CARTESIAN_POINT('Ctrl Pts',(-2.22338548312772,1.,-3.3266964672289));
#66827=CARTESIAN_POINT('Ctrl Pts',(-2.22955308907233,-1.,-3.33118487773611));
#66828=CARTESIAN_POINT('Ctrl Pts',(-2.22955308907233,1.,-3.33118487773611));
#66829=CARTESIAN_POINT('Ctrl Pts',(-2.23575256328812,-1.,-3.33564495756482));
#66830=CARTESIAN_POINT('Ctrl Pts',(-2.23575256328812,1.,-3.33564495756482));
#66831=CARTESIAN_POINT('Ctrl Pts',(-2.24198249391422,-1.,-3.34007543738025));
#66832=CARTESIAN_POINT('Ctrl Pts',(-2.24198249391422,1.,-3.34007543738025));
#66833=CARTESIAN_POINT('Ctrl Pts',(-2.24824207678256,-1.,-3.34447596770723));
#66834=CARTESIAN_POINT('Ctrl Pts',(-2.24824207678256,1.,-3.34447596770723));
#66835=CARTESIAN_POINT('Ctrl Pts',(-2.25453097693483,-1.,-3.34884690292285));
#66836=CARTESIAN_POINT('Ctrl Pts',(-2.25453097693483,1.,-3.34884690292285));
#66837=CARTESIAN_POINT('Ctrl Pts',(-2.26084915222449,-1.,-3.35318902552626));
#66838=CARTESIAN_POINT('Ctrl Pts',(-2.26084915222449,1.,-3.35318902552626));
#66839=CARTESIAN_POINT('Ctrl Pts',(-2.2671966857991,-1.,-3.35750328523061));
#66840=CARTESIAN_POINT('Ctrl Pts',(-2.2671966857991,1.,-3.35750328523061));
#66841=CARTESIAN_POINT('Ctrl Pts',(-2.2735736262093,-1.,-3.36179055004409));
#66842=CARTESIAN_POINT('Ctrl Pts',(-2.2735736262093,1.,-3.36179055004409));
#66843=CARTESIAN_POINT('Ctrl Pts',(-2.27997979458037,-1.,-3.36605130713076));
#66844=CARTESIAN_POINT('Ctrl Pts',(-2.27997979458037,1.,-3.36605130713076));
#66845=CARTESIAN_POINT('Ctrl Pts',(-2.28641481081137,-1.,-3.37028570206488));
#66846=CARTESIAN_POINT('Ctrl Pts',(-2.28641481081137,1.,-3.37028570206488));
#66847=CARTESIAN_POINT('Ctrl Pts',(-2.29287818007393,-1.,-3.37449367172826));
#66848=CARTESIAN_POINT('Ctrl Pts',(-2.29287818007393,1.,-3.37449367172826));
#66849=CARTESIAN_POINT('Ctrl Pts',(-2.29936936127624,-1.,-3.37867504959433));
#66850=CARTESIAN_POINT('Ctrl Pts',(-2.29936936127624,1.,-3.37867504959433));
#66851=CARTESIAN_POINT('Ctrl Pts',(-2.30588783640343,-1.,-3.3828296733661));
#66852=CARTESIAN_POINT('Ctrl Pts',(-2.30588783640343,1.,-3.3828296733661));
#66853=CARTESIAN_POINT('Ctrl Pts',(-2.31243319489367,-1.,-3.38695751492462));
#66854=CARTESIAN_POINT('Ctrl Pts',(-2.31243319489367,1.,-3.38695751492462));
#66855=CARTESIAN_POINT('Ctrl Pts',(-2.31900513925424,-1.,-3.39105869474822));
#66856=CARTESIAN_POINT('Ctrl Pts',(-2.31900513925424,1.,-3.39105869474822));
#66857=CARTESIAN_POINT('Ctrl Pts',(-2.3256034390248,-1.,-3.39513342019756));
#66858=CARTESIAN_POINT('Ctrl Pts',(-2.3256034390248,1.,-3.39513342019756));
#66859=CARTESIAN_POINT('Ctrl Pts',(-2.33222789882489,-1.,-3.39918194577956));
#66860=CARTESIAN_POINT('Ctrl Pts',(-2.33222789882489,1.,-3.39918194577956));
#66861=CARTESIAN_POINT('Ctrl Pts',(-2.33887832342782,-1.,-3.40320452776743));
#66862=CARTESIAN_POINT('Ctrl Pts',(-2.33887832342782,1.,-3.40320452776743));
#66863=CARTESIAN_POINT('Ctrl Pts',(-2.34555447649188,-1.,-3.40720137404297));
#66864=CARTESIAN_POINT('Ctrl Pts',(-2.34555447649188,1.,-3.40720137404297));
#66865=CARTESIAN_POINT('Ctrl Pts',(-2.35225606824109,-1.,-3.41117262314119));
#66866=CARTESIAN_POINT('Ctrl Pts',(-2.35225606824109,1.,-3.41117262314119));
#66867=CARTESIAN_POINT('Ctrl Pts',(-2.35898278606946,-1.,-3.41511836751469));
#66868=CARTESIAN_POINT('Ctrl Pts',(-2.35898278606946,1.,-3.41511836751469));
#66869=CARTESIAN_POINT('Ctrl Pts',(-2.36573431470642,-1.,-3.41903866635852));
#66870=CARTESIAN_POINT('Ctrl Pts',(-2.36573431470642,1.,-3.41903866635852));
#66871=CARTESIAN_POINT('Ctrl Pts',(-2.37251035954292,-1.,-3.42293356216511));
#66872=CARTESIAN_POINT('Ctrl Pts',(-2.37251035954292,1.,-3.42293356216511));
#66873=CARTESIAN_POINT('Ctrl Pts',(-2.37931067028926,-1.,-3.42680309754399));
#66874=CARTESIAN_POINT('Ctrl Pts',(-2.37931067028926,1.,-3.42680309754399));
#66875=CARTESIAN_POINT('Ctrl Pts',(-2.38613505843552,-1.,-3.4306473271292));
#66876=CARTESIAN_POINT('Ctrl Pts',(-2.38613505843552,1.,-3.4306473271292));
#66877=CARTESIAN_POINT('Ctrl Pts',(-2.39298338804493,-1.,-3.4344663067854));
#66878=CARTESIAN_POINT('Ctrl Pts',(-2.39298338804493,1.,-3.4344663067854));
#66879=CARTESIAN_POINT('Ctrl Pts',(-2.39848113410292,-1.,-3.43750133064416));
#66880=CARTESIAN_POINT('Ctrl Pts',(-2.39848113410292,1.,-3.43750133064416));
#66881=CARTESIAN_POINT('Ctrl Pts',(-2.40261515589405,-1.,-3.43976627484234));
#66882=CARTESIAN_POINT('Ctrl Pts',(-2.40261515589405,1.,-3.43976627484234));
#66883=CARTESIAN_POINT('Ctrl Pts',(-2.4053759295909,-1.,-3.44127120683039));
#66884=CARTESIAN_POINT('Ctrl Pts',(-2.4053759295909,1.,-3.44127120683039));
#66885=CARTESIAN_POINT('Ctrl Pts',(-2.40675750623143,-1.,-3.44202241512147));
#66886=CARTESIAN_POINT('Ctrl Pts',(-2.40675750623143,1.,-3.44202241512147));
#66887=CARTESIAN_POINT('',(-2.03660101169714,1.,-3.14877060440328));
#66888=CARTESIAN_POINT('Ctrl Pts',(-2.03660101169715,-1.,-3.14877060440327));
#66889=CARTESIAN_POINT('Ctrl Pts',(-2.03660101169715,-0.666666666666667,
-3.14877060440327));
#66890=CARTESIAN_POINT('Ctrl Pts',(-2.03660101169715,-0.333333333333333,
-3.14877060440327));
#66891=CARTESIAN_POINT('Ctrl Pts',(-2.03660101169715,0.333333333333333,
-3.14877060440327));
#66892=CARTESIAN_POINT('Ctrl Pts',(-2.03660101169715,0.666666666666667,
-3.14877060440327));
#66893=CARTESIAN_POINT('Ctrl Pts',(-2.03660101169715,1.,-3.14877060440327));
#66894=CARTESIAN_POINT('',(-2.40675750623143,1.,-3.44202241512147));
#66895=CARTESIAN_POINT('',(-2.40675750623143,0.,-3.44202241512147));
#66896=CARTESIAN_POINT('Ctrl Pts',(-2.03660101169715,1.,-3.14877060440328));
#66897=CARTESIAN_POINT('Ctrl Pts',(-2.03659701539259,1.,-3.14881939088124));
#66898=CARTESIAN_POINT('Ctrl Pts',(-2.03663974554932,1.,-3.1490119366901));
#66899=CARTESIAN_POINT('Ctrl Pts',(-2.03693188810545,1.,-3.14959882629805));
#66900=CARTESIAN_POINT('Ctrl Pts',(-2.03783225495961,1.,-3.15102344775328));
#66901=CARTESIAN_POINT('Ctrl Pts',(-2.03984073791519,1.,-3.15389991674792));
#66902=CARTESIAN_POINT('Ctrl Pts',(-2.04297406404027,1.,-3.15817983946367));
#66903=CARTESIAN_POINT('Ctrl Pts',(-2.04693331247446,1.,-3.16343165058912));
#66904=CARTESIAN_POINT('Ctrl Pts',(-2.05151770247233,1.,-3.16936341689527));
#66905=CARTESIAN_POINT('Ctrl Pts',(-2.05650186773132,1.,-3.17564906975371));
#66906=CARTESIAN_POINT('Ctrl Pts',(-2.06166849827101,1.,-3.18197692964614));
#66907=CARTESIAN_POINT('Ctrl Pts',(-2.06684062744112,1.,-3.18809755562368));
#66908=CARTESIAN_POINT('Ctrl Pts',(-2.07192253497857,1.,-3.19388465568252));
#66909=CARTESIAN_POINT('Ctrl Pts',(-2.07690441870722,1.,-3.19934132836019));
#66910=CARTESIAN_POINT('Ctrl Pts',(-2.08182850370878,1.,-3.2045481863073));
#66911=CARTESIAN_POINT('Ctrl Pts',(-2.08676465517455,1.,-3.20962575845463));
#66912=CARTESIAN_POINT('Ctrl Pts',(-2.09178419460443,1.,-3.21469429601654));
#66913=CARTESIAN_POINT('Ctrl Pts',(-2.09692958434895,1.,-3.21982707347009));
#66914=CARTESIAN_POINT('Ctrl Pts',(-2.10220384298492,1.,-3.22503437553434));
#66915=CARTESIAN_POINT('Ctrl Pts',(-2.10758699642451,1.,-3.23028945793289));
#66916=CARTESIAN_POINT('Ctrl Pts',(-2.11304604021773,1.,-3.23554444767099));
#66917=CARTESIAN_POINT('Ctrl Pts',(-2.11854673326979,1.,-3.24074905517293));
#66918=CARTESIAN_POINT('Ctrl Pts',(-2.12406646410962,1.,-3.24587102613376));
#66919=CARTESIAN_POINT('Ctrl Pts',(-2.12960028396832,1.,-3.25090574494028));
#66920=CARTESIAN_POINT('Ctrl Pts',(-2.13515375878803,1.,-3.25586495065054));
#66921=CARTESIAN_POINT('Ctrl Pts',(-2.14073870754264,1.,-3.26077002641879));
#66922=CARTESIAN_POINT('Ctrl Pts',(-2.1463680529566,1.,-3.26564388189759));
#66923=CARTESIAN_POINT('Ctrl Pts',(-2.15205043199808,1.,-3.27050245897228));
#66924=CARTESIAN_POINT('Ctrl Pts',(-2.15778690038347,1.,-3.27534954469187));
#66925=CARTESIAN_POINT('Ctrl Pts',(-2.16357391934425,1.,-3.280181508414));
#66926=CARTESIAN_POINT('Ctrl Pts',(-2.16940517773455,1.,-3.28499019979724));
#66927=CARTESIAN_POINT('Ctrl Pts',(-2.17527380048423,1.,-3.28976645712568));
#66928=CARTESIAN_POINT('Ctrl Pts',(-2.18117455557065,1.,-3.2945036150049));
#66929=CARTESIAN_POINT('Ctrl Pts',(-2.18710556500327,1.,-3.29920022557639));
#66930=CARTESIAN_POINT('Ctrl Pts',(-2.19306710376111,1.,-3.30385816281831));
#66931=CARTESIAN_POINT('Ctrl Pts',(-2.19906078949923,1.,-3.30848134694595));
#66932=CARTESIAN_POINT('Ctrl Pts',(-2.20508863150607,1.,-3.31307424608949));
#66933=CARTESIAN_POINT('Ctrl Pts',(-2.21115211847875,1.,-3.31764044024235));
#66934=CARTESIAN_POINT('Ctrl Pts',(-2.21725135110898,1.,-3.32218125618968));
#66935=CARTESIAN_POINT('Ctrl Pts',(-2.22338548312772,1.,-3.3266964672289));
#66936=CARTESIAN_POINT('Ctrl Pts',(-2.22955308907233,1.,-3.33118487773611));
#66937=CARTESIAN_POINT('Ctrl Pts',(-2.23575256328812,1.,-3.33564495756482));
#66938=CARTESIAN_POINT('Ctrl Pts',(-2.24198249391422,1.,-3.34007543738025));
#66939=CARTESIAN_POINT('Ctrl Pts',(-2.24824207678256,1.,-3.34447596770723));
#66940=CARTESIAN_POINT('Ctrl Pts',(-2.25453097693483,1.,-3.34884690292285));
#66941=CARTESIAN_POINT('Ctrl Pts',(-2.26084915222449,1.,-3.35318902552626));
#66942=CARTESIAN_POINT('Ctrl Pts',(-2.2671966857991,1.,-3.35750328523061));
#66943=CARTESIAN_POINT('Ctrl Pts',(-2.2735736262093,1.,-3.36179055004409));
#66944=CARTESIAN_POINT('Ctrl Pts',(-2.27997979458037,1.,-3.36605130713076));
#66945=CARTESIAN_POINT('Ctrl Pts',(-2.28641481081137,1.,-3.37028570206488));
#66946=CARTESIAN_POINT('Ctrl Pts',(-2.29287818007393,1.,-3.37449367172826));
#66947=CARTESIAN_POINT('Ctrl Pts',(-2.29936936127624,1.,-3.37867504959433));
#66948=CARTESIAN_POINT('Ctrl Pts',(-2.30588783640343,1.,-3.3828296733661));
#66949=CARTESIAN_POINT('Ctrl Pts',(-2.31243319489367,1.,-3.38695751492462));
#66950=CARTESIAN_POINT('Ctrl Pts',(-2.31900513925424,1.,-3.39105869474822));
#66951=CARTESIAN_POINT('Ctrl Pts',(-2.3256034390248,1.,-3.39513342019756));
#66952=CARTESIAN_POINT('Ctrl Pts',(-2.33222789882489,1.,-3.39918194577956));
#66953=CARTESIAN_POINT('Ctrl Pts',(-2.33887832342782,1.,-3.40320452776743));
#66954=CARTESIAN_POINT('Ctrl Pts',(-2.34555447649188,1.,-3.40720137404297));
#66955=CARTESIAN_POINT('Ctrl Pts',(-2.35225606824109,1.,-3.41117262314119));
#66956=CARTESIAN_POINT('Ctrl Pts',(-2.35898278606946,1.,-3.41511836751469));
#66957=CARTESIAN_POINT('Ctrl Pts',(-2.36573431470642,1.,-3.41903866635852));
#66958=CARTESIAN_POINT('Ctrl Pts',(-2.37251035954292,1.,-3.42293356216511));
#66959=CARTESIAN_POINT('Ctrl Pts',(-2.37931067028926,1.,-3.42680309754399));
#66960=CARTESIAN_POINT('Ctrl Pts',(-2.38613505843552,1.,-3.4306473271292));
#66961=CARTESIAN_POINT('Ctrl Pts',(-2.39298338804493,1.,-3.4344663067854));
#66962=CARTESIAN_POINT('Ctrl Pts',(-2.39848113410292,1.,-3.43750133064416));
#66963=CARTESIAN_POINT('Ctrl Pts',(-2.40261515589405,1.,-3.43976627484234));
#66964=CARTESIAN_POINT('Ctrl Pts',(-2.4053759295909,1.,-3.44127120683039));
#66965=CARTESIAN_POINT('Ctrl Pts',(-2.40675750623143,1.,-3.44202241512147));
#66966=CARTESIAN_POINT('Origin',(-2.40675750623143,0.,-3.44202241512147));
#66967=CARTESIAN_POINT('',(-2.52982887637028,1.,-3.35260583073571));
#66968=CARTESIAN_POINT('Origin',(0.,0.,0.));
#66969=CARTESIAN_POINT('',(-1.88097764062697,1.,-3.24413672884812));
#66970=CARTESIAN_POINT('Origin',(0.,1.,0.));
#66971=CARTESIAN_POINT('Ctrl Pts',(-1.88097764062697,1.,-3.24413672884812));
#66972=CARTESIAN_POINT('Ctrl Pts',(-1.88097764062697,0.666666666666667,
-3.24413672884812));
#66973=CARTESIAN_POINT('Ctrl Pts',(-1.88097764062697,0.333333333333333,
-3.24413672884812));
#66974=CARTESIAN_POINT('Ctrl Pts',(-1.88097764062697,-0.333333333333333,
-3.24413672884812));
#66975=CARTESIAN_POINT('Ctrl Pts',(-1.88097764062697,-0.666666666666667,
-3.24413672884812));
#66976=CARTESIAN_POINT('Ctrl Pts',(-1.88097764062697,-1.,-3.24413672884812));
#66977=CARTESIAN_POINT('Ctrl Pts',(-1.97421938526992,-1.,-3.70708211654725));
#66978=CARTESIAN_POINT('Ctrl Pts',(-1.97421938526992,1.,-3.70708211654725));
#66979=CARTESIAN_POINT('Ctrl Pts',(-1.97417727645308,-1.,-3.70551008132332));
#66980=CARTESIAN_POINT('Ctrl Pts',(-1.97417727645308,1.,-3.70551008132332));
#66981=CARTESIAN_POINT('Ctrl Pts',(-1.97408973726715,-1.,-3.70236698912904));
#66982=CARTESIAN_POINT('Ctrl Pts',(-1.97408973726715,1.,-3.70236698912904));
#66983=CARTESIAN_POINT('Ctrl Pts',(-1.97394846383216,-1.,-3.6976552856004));
#66984=CARTESIAN_POINT('Ctrl Pts',(-1.97394846383216,1.,-3.6976552856004));
#66985=CARTESIAN_POINT('Ctrl Pts',(-1.97374016225483,-1.,-3.69137888599902));
#66986=CARTESIAN_POINT('Ctrl Pts',(-1.97374016225483,1.,-3.69137888599902));
#66987=CARTESIAN_POINT('Ctrl Pts',(-1.97344650304519,-1.,-3.68354319915092));
#66988=CARTESIAN_POINT('Ctrl Pts',(-1.97344650304519,1.,-3.68354319915092));
#66989=CARTESIAN_POINT('Ctrl Pts',(-1.97311947678517,-1.,-3.67571738107084));
#66990=CARTESIAN_POINT('Ctrl Pts',(-1.97311947678517,1.,-3.67571738107084));
#66991=CARTESIAN_POINT('Ctrl Pts',(-1.97275897198678,-1.,-3.66790152752075));
#66992=CARTESIAN_POINT('Ctrl Pts',(-1.97275897198678,1.,-3.66790152752075));
#66993=CARTESIAN_POINT('Ctrl Pts',(-1.9723648543905,-1.,-3.6600957816636));
#66994=CARTESIAN_POINT('Ctrl Pts',(-1.9723648543905,1.,-3.6600957816636));
#66995=CARTESIAN_POINT('Ctrl Pts',(-1.9719369724024,-1.,-3.652300347166));
#66996=CARTESIAN_POINT('Ctrl Pts',(-1.9719369724024,1.,-3.652300347166));
#66997=CARTESIAN_POINT('Ctrl Pts',(-1.97147515441164,-1.,-3.64451546723514));
#66998=CARTESIAN_POINT('Ctrl Pts',(-1.97147515441164,1.,-3.64451546723514));
#66999=CARTESIAN_POINT('Ctrl Pts',(-1.97097920454464,-1.,-3.63674139590412));
#67000=CARTESIAN_POINT('Ctrl Pts',(-1.97097920454464,1.,-3.63674139590412));
#67001=CARTESIAN_POINT('Ctrl Pts',(-1.97044889850463,-1.,-3.62897836973293));
#67002=CARTESIAN_POINT('Ctrl Pts',(-1.97044889850463,1.,-3.62897836973293));
#67003=CARTESIAN_POINT('Ctrl Pts',(-1.96988398129978,-1.,-3.62122658401893));
#67004=CARTESIAN_POINT('Ctrl Pts',(-1.96988398129978,1.,-3.62122658401893));
#67005=CARTESIAN_POINT('Ctrl Pts',(-1.96928416040877,-1.,-3.61348615496704));
#67006=CARTESIAN_POINT('Ctrl Pts',(-1.96928416040877,1.,-3.61348615496704));
#67007=CARTESIAN_POINT('Ctrl Pts',(-1.9686491188594,-1.,-3.60575714017989));
#67008=CARTESIAN_POINT('Ctrl Pts',(-1.9686491188594,1.,-3.60575714017989));
#67009=CARTESIAN_POINT('Ctrl Pts',(-1.96797854118369,-1.,-3.59803959819938));
#67010=CARTESIAN_POINT('Ctrl Pts',(-1.96797854118369,1.,-3.59803959819938));
#67011=CARTESIAN_POINT('Ctrl Pts',(-1.96727213799544,-1.,-3.59033364022801));
#67012=CARTESIAN_POINT('Ctrl Pts',(-1.96727213799544,1.,-3.59033364022801));
#67013=CARTESIAN_POINT('Ctrl Pts',(-1.96652966688911,-1.,-3.58263947663829));
#67014=CARTESIAN_POINT('Ctrl Pts',(-1.96652966688911,1.,-3.58263947663829));
#67015=CARTESIAN_POINT('Ctrl Pts',(-1.96575096652789,-1.,-3.57495748600959));
#67016=CARTESIAN_POINT('Ctrl Pts',(-1.96575096652789,1.,-3.57495748600959));
#67017=CARTESIAN_POINT('Ctrl Pts',(-1.96493594634567,-1.,-3.56728820357791));
#67018=CARTESIAN_POINT('Ctrl Pts',(-1.96493594634567,1.,-3.56728820357791));
#67019=CARTESIAN_POINT('Ctrl Pts',(-1.96408450906812,-1.,-3.55963218706096));
#67020=CARTESIAN_POINT('Ctrl Pts',(-1.96408450906812,1.,-3.55963218706096));
#67021=CARTESIAN_POINT('Ctrl Pts',(-1.96319648628644,-1.,-3.55198990600886));
#67022=CARTESIAN_POINT('Ctrl Pts',(-1.96319648628644,1.,-3.55198990600886));
#67023=CARTESIAN_POINT('Ctrl Pts',(-1.96227157573067,-1.,-3.54436163300443));
#67024=CARTESIAN_POINT('Ctrl Pts',(-1.96227157573067,1.,-3.54436163300443));
#67025=CARTESIAN_POINT('Ctrl Pts',(-1.96130926212689,-1.,-3.53674730625813));
#67026=CARTESIAN_POINT('Ctrl Pts',(-1.96130926212689,1.,-3.53674730625813));
#67027=CARTESIAN_POINT('Ctrl Pts',(-1.96030879411566,-1.,-3.52914648844351));
#67028=CARTESIAN_POINT('Ctrl Pts',(-1.96030879411566,1.,-3.52914648844351));
#67029=CARTESIAN_POINT('Ctrl Pts',(-1.95926936324461,-1.,-3.52155867431486));
#67030=CARTESIAN_POINT('Ctrl Pts',(-1.95926936324461,1.,-3.52155867431486));
#67031=CARTESIAN_POINT('Ctrl Pts',(-1.95819025316779,-1.,-3.51398354617794));
#67032=CARTESIAN_POINT('Ctrl Pts',(-1.95819025316779,1.,-3.51398354617794));
#67033=CARTESIAN_POINT('Ctrl Pts',(-1.95707099606511,-1.,-3.50642124159909));
#67034=CARTESIAN_POINT('Ctrl Pts',(-1.95707099606511,1.,-3.50642124159909));
#67035=CARTESIAN_POINT('Ctrl Pts',(-1.95591153823661,-1.,-3.49887263575583));
#67036=CARTESIAN_POINT('Ctrl Pts',(-1.95591153823661,1.,-3.49887263575583));
#67037=CARTESIAN_POINT('Ctrl Pts',(-1.95471236969643,-1.,-3.49133956289133));
#67038=CARTESIAN_POINT('Ctrl Pts',(-1.95471236969643,1.,-3.49133956289133));
#67039=CARTESIAN_POINT('Ctrl Pts',(-1.95347412486309,-1.,-3.48382414832634));
#67040=CARTESIAN_POINT('Ctrl Pts',(-1.95347412486309,1.,-3.48382414832634));
#67041=CARTESIAN_POINT('Ctrl Pts',(-1.95219722189876,-1.,-3.47632820495921));
#67042=CARTESIAN_POINT('Ctrl Pts',(-1.95219722189876,1.,-3.47632820495921));
#67043=CARTESIAN_POINT('Ctrl Pts',(-1.95088147859877,-1.,-3.46885258974191));
#67044=CARTESIAN_POINT('Ctrl Pts',(-1.95088147859877,1.,-3.46885258974191));
#67045=CARTESIAN_POINT('Ctrl Pts',(-1.94952575850197,-1.,-3.46139661060962));
#67046=CARTESIAN_POINT('Ctrl Pts',(-1.94952575850197,1.,-3.46139661060962));
#67047=CARTESIAN_POINT('Ctrl Pts',(-1.94812754766524,-1.,-3.45395731584051));
#67048=CARTESIAN_POINT('Ctrl Pts',(-1.94812754766524,1.,-3.45395731584051));
#67049=CARTESIAN_POINT('Ctrl Pts',(-1.94668377715329,-1.,-3.44653088665681));
#67050=CARTESIAN_POINT('Ctrl Pts',(-1.94668377715329,1.,-3.44653088665681));
#67051=CARTESIAN_POINT('Ctrl Pts',(-1.94519168842879,-1.,-3.43911410197687));
#67052=CARTESIAN_POINT('Ctrl Pts',(-1.94519168842879,1.,-3.43911410197687));
#67053=CARTESIAN_POINT('Ctrl Pts',(-1.94364973660284,-1.,-3.43170586602434));
#67054=CARTESIAN_POINT('Ctrl Pts',(-1.94364973660284,1.,-3.43170586602434));
#67055=CARTESIAN_POINT('Ctrl Pts',(-1.94205835913696,-1.,-3.42430850941503));
#67056=CARTESIAN_POINT('Ctrl Pts',(-1.94205835913696,1.,-3.42430850941503));
#67057=CARTESIAN_POINT('Ctrl Pts',(-1.94042111965246,-1.,-3.41692971994096));
#67058=CARTESIAN_POINT('Ctrl Pts',(-1.94042111965246,1.,-3.41692971994096));
#67059=CARTESIAN_POINT('Ctrl Pts',(-1.93874306008143,-1.,-3.40957978266642));
#67060=CARTESIAN_POINT('Ctrl Pts',(-1.93874306008143,1.,-3.40957978266642));
#67061=CARTESIAN_POINT('Ctrl Pts',(-1.93702857723098,-1.,-3.40226802104109));
#67062=CARTESIAN_POINT('Ctrl Pts',(-1.93702857723098,1.,-3.40226802104109));
#67063=CARTESIAN_POINT('Ctrl Pts',(-1.93527929945985,-1.,-3.39499923640795));
#67064=CARTESIAN_POINT('Ctrl Pts',(-1.93527929945985,1.,-3.39499923640795));
#67065=CARTESIAN_POINT('Ctrl Pts',(-1.93349233176788,-1.,-3.38777076883256));
#67066=CARTESIAN_POINT('Ctrl Pts',(-1.93349233176788,1.,-3.38777076883256));
#67067=CARTESIAN_POINT('Ctrl Pts',(-1.93165739093276,-1.,-3.3805676852555));
#67068=CARTESIAN_POINT('Ctrl Pts',(-1.93165739093276,1.,-3.3805676852555));
#67069=CARTESIAN_POINT('Ctrl Pts',(-1.92975993109877,-1.,-3.37336807068043));
#67070=CARTESIAN_POINT('Ctrl Pts',(-1.92975993109877,1.,-3.37336807068043));
#67071=CARTESIAN_POINT('Ctrl Pts',(-1.92778626543786,-1.,-3.36615168657567));
#67072=CARTESIAN_POINT('Ctrl Pts',(-1.92778626543786,1.,-3.36615168657567));
#67073=CARTESIAN_POINT('Ctrl Pts',(-1.92572846125756,-1.,-3.35890824422965));
#67074=CARTESIAN_POINT('Ctrl Pts',(-1.92572846125756,1.,-3.35890824422965));
#67075=CARTESIAN_POINT('Ctrl Pts',(-1.92358838440528,-1.,-3.35164424847223));
#67076=CARTESIAN_POINT('Ctrl Pts',(-1.92358838440528,1.,-3.35164424847223));
#67077=CARTESIAN_POINT('Ctrl Pts',(-1.92138450828404,-1.,-3.34439448941961));
#67078=CARTESIAN_POINT('Ctrl Pts',(-1.92138450828404,1.,-3.34439448941961));
#67079=CARTESIAN_POINT('Ctrl Pts',(-1.9191460961021,-1.,-3.33721230710012));
#67080=CARTESIAN_POINT('Ctrl Pts',(-1.9191460961021,1.,-3.33721230710012));
#67081=CARTESIAN_POINT('Ctrl Pts',(-1.91690081930331,-1.,-3.33014884257873));
#67082=CARTESIAN_POINT('Ctrl Pts',(-1.91690081930331,1.,-3.33014884257873));
#67083=CARTESIAN_POINT('Ctrl Pts',(-1.91466343916628,-1.,-3.32323403454535));
#67084=CARTESIAN_POINT('Ctrl Pts',(-1.91466343916628,1.,-3.32323403454535));
#67085=CARTESIAN_POINT('Ctrl Pts',(-1.91242616234442,-1.,-3.31646052426364));
#67086=CARTESIAN_POINT('Ctrl Pts',(-1.91242616234442,1.,-3.31646052426364));
#67087=CARTESIAN_POINT('Ctrl Pts',(-1.91014297830446,-1.,-3.30975721158596));
#67088=CARTESIAN_POINT('Ctrl Pts',(-1.91014297830446,1.,-3.30975721158596));
#67089=CARTESIAN_POINT('Ctrl Pts',(-1.90773912171341,-1.,-3.30300595568195));
#67090=CARTESIAN_POINT('Ctrl Pts',(-1.90773912171341,1.,-3.30300595568195));
#67091=CARTESIAN_POINT('Ctrl Pts',(-1.90513891864087,-1.,-3.29608978722113));
#67092=CARTESIAN_POINT('Ctrl Pts',(-1.90513891864087,1.,-3.29608978722113));
#67093=CARTESIAN_POINT('Ctrl Pts',(-1.90228971247527,-1.,-3.2889344860029));
#67094=CARTESIAN_POINT('Ctrl Pts',(-1.90228971247527,1.,-3.2889344860029));
#67095=CARTESIAN_POINT('Ctrl Pts',(-1.89918429230462,-1.,-3.28154737912352));
#67096=CARTESIAN_POINT('Ctrl Pts',(-1.89918429230462,1.,-3.28154737912352));
#67097=CARTESIAN_POINT('Ctrl Pts',(-1.89589172903793,-1.,-3.27407108933139));
#67098=CARTESIAN_POINT('Ctrl Pts',(-1.89589172903793,1.,-3.27407108933139));
#67099=CARTESIAN_POINT('Ctrl Pts',(-1.89255393500965,-1.,-3.26677653888676));
#67100=CARTESIAN_POINT('Ctrl Pts',(-1.89255393500965,1.,-3.26677653888676));
#67101=CARTESIAN_POINT('Ctrl Pts',(-1.88934996203698,-1.,-3.25999885193947));
#67102=CARTESIAN_POINT('Ctrl Pts',(-1.88934996203698,1.,-3.25999885193947));
#67103=CARTESIAN_POINT('Ctrl Pts',(-1.88646802523466,-1.,-3.25408686339463));
#67104=CARTESIAN_POINT('Ctrl Pts',(-1.88646802523466,1.,-3.25408686339463));
#67105=CARTESIAN_POINT('Ctrl Pts',(-1.88407708646357,-1.,-3.24935200511918));
#67106=CARTESIAN_POINT('Ctrl Pts',(-1.88407708646357,1.,-3.24935200511918));
#67107=CARTESIAN_POINT('Ctrl Pts',(-1.88229202582941,-1.,-3.24600543790443));
#67108=CARTESIAN_POINT('Ctrl Pts',(-1.88229202582941,1.,-3.24600543790443));
#67109=CARTESIAN_POINT('Ctrl Pts',(-1.88139187908074,-1.,-3.24451807186481));
#67110=CARTESIAN_POINT('Ctrl Pts',(-1.88139187908074,1.,-3.24451807186481));
#67111=CARTESIAN_POINT('Ctrl Pts',(-1.88102201872555,-1.,-3.24408699284121));
#67112=CARTESIAN_POINT('Ctrl Pts',(-1.88102201872555,1.,-3.24408699284121));
#67113=CARTESIAN_POINT('Ctrl Pts',(-1.88091100680349,-1.,-3.24410359189609));
#67114=CARTESIAN_POINT('Ctrl Pts',(-1.88091100680349,1.,-3.24410359189609));
#67115=CARTESIAN_POINT('Ctrl Pts',(-1.8808893942881,-1.,-3.24418789321065));
#67116=CARTESIAN_POINT('Ctrl Pts',(-1.8808893942881,1.,-3.24418789321065));
#67117=CARTESIAN_POINT('',(-1.97421938526992,1.,-3.70708211654725));
#67118=CARTESIAN_POINT('Ctrl Pts',(-1.97421938526992,1.,-3.70708211654725));
#67119=CARTESIAN_POINT('Ctrl Pts',(-1.97417727645308,1.,-3.70551008132332));
#67120=CARTESIAN_POINT('Ctrl Pts',(-1.97408973726715,1.,-3.70236698912904));
#67121=CARTESIAN_POINT('Ctrl Pts',(-1.97394846383216,1.,-3.6976552856004));
#67122=CARTESIAN_POINT('Ctrl Pts',(-1.97374016225483,1.,-3.69137888599902));
#67123=CARTESIAN_POINT('Ctrl Pts',(-1.97344650304519,1.,-3.68354319915092));
#67124=CARTESIAN_POINT('Ctrl Pts',(-1.97311947678517,1.,-3.67571738107084));
#67125=CARTESIAN_POINT('Ctrl Pts',(-1.97275897198678,1.,-3.66790152752075));
#67126=CARTESIAN_POINT('Ctrl Pts',(-1.9723648543905,1.,-3.6600957816636));
#67127=CARTESIAN_POINT('Ctrl Pts',(-1.9719369724024,1.,-3.652300347166));
#67128=CARTESIAN_POINT('Ctrl Pts',(-1.97147515441164,1.,-3.64451546723514));
#67129=CARTESIAN_POINT('Ctrl Pts',(-1.97097920454464,1.,-3.63674139590412));
#67130=CARTESIAN_POINT('Ctrl Pts',(-1.97044889850463,1.,-3.62897836973293));
#67131=CARTESIAN_POINT('Ctrl Pts',(-1.96988398129978,1.,-3.62122658401893));
#67132=CARTESIAN_POINT('Ctrl Pts',(-1.96928416040877,1.,-3.61348615496704));
#67133=CARTESIAN_POINT('Ctrl Pts',(-1.9686491188594,1.,-3.60575714017989));
#67134=CARTESIAN_POINT('Ctrl Pts',(-1.96797854118369,1.,-3.59803959819938));
#67135=CARTESIAN_POINT('Ctrl Pts',(-1.96727213799544,1.,-3.59033364022801));
#67136=CARTESIAN_POINT('Ctrl Pts',(-1.96652966688911,1.,-3.58263947663829));
#67137=CARTESIAN_POINT('Ctrl Pts',(-1.96575096652789,1.,-3.57495748600959));
#67138=CARTESIAN_POINT('Ctrl Pts',(-1.96493594634567,1.,-3.56728820357791));
#67139=CARTESIAN_POINT('Ctrl Pts',(-1.96408450906812,1.,-3.55963218706096));
#67140=CARTESIAN_POINT('Ctrl Pts',(-1.96319648628644,1.,-3.55198990600886));
#67141=CARTESIAN_POINT('Ctrl Pts',(-1.96227157573067,1.,-3.54436163300443));
#67142=CARTESIAN_POINT('Ctrl Pts',(-1.96130926212689,1.,-3.53674730625813));
#67143=CARTESIAN_POINT('Ctrl Pts',(-1.96030879411566,1.,-3.52914648844351));
#67144=CARTESIAN_POINT('Ctrl Pts',(-1.95926936324461,1.,-3.52155867431486));
#67145=CARTESIAN_POINT('Ctrl Pts',(-1.95819025316779,1.,-3.51398354617794));
#67146=CARTESIAN_POINT('Ctrl Pts',(-1.95707099606511,1.,-3.50642124159909));
#67147=CARTESIAN_POINT('Ctrl Pts',(-1.95591153823661,1.,-3.49887263575583));
#67148=CARTESIAN_POINT('Ctrl Pts',(-1.95471236969643,1.,-3.49133956289133));
#67149=CARTESIAN_POINT('Ctrl Pts',(-1.95347412486309,1.,-3.48382414832634));
#67150=CARTESIAN_POINT('Ctrl Pts',(-1.95219722189876,1.,-3.47632820495921));
#67151=CARTESIAN_POINT('Ctrl Pts',(-1.95088147859877,1.,-3.46885258974191));
#67152=CARTESIAN_POINT('Ctrl Pts',(-1.94952575850197,1.,-3.46139661060962));
#67153=CARTESIAN_POINT('Ctrl Pts',(-1.94812754766524,1.,-3.45395731584051));
#67154=CARTESIAN_POINT('Ctrl Pts',(-1.94668377715329,1.,-3.44653088665681));
#67155=CARTESIAN_POINT('Ctrl Pts',(-1.94519168842879,1.,-3.43911410197687));
#67156=CARTESIAN_POINT('Ctrl Pts',(-1.94364973660284,1.,-3.43170586602434));
#67157=CARTESIAN_POINT('Ctrl Pts',(-1.94205835913696,1.,-3.42430850941503));
#67158=CARTESIAN_POINT('Ctrl Pts',(-1.94042111965246,1.,-3.41692971994096));
#67159=CARTESIAN_POINT('Ctrl Pts',(-1.93874306008143,1.,-3.40957978266642));
#67160=CARTESIAN_POINT('Ctrl Pts',(-1.93702857723098,1.,-3.40226802104109));
#67161=CARTESIAN_POINT('Ctrl Pts',(-1.93527929945985,1.,-3.39499923640795));
#67162=CARTESIAN_POINT('Ctrl Pts',(-1.93349233176788,1.,-3.38777076883256));
#67163=CARTESIAN_POINT('Ctrl Pts',(-1.93165739093276,1.,-3.3805676852555));
#67164=CARTESIAN_POINT('Ctrl Pts',(-1.92975993109877,1.,-3.37336807068043));
#67165=CARTESIAN_POINT('Ctrl Pts',(-1.92778626543786,1.,-3.36615168657567));
#67166=CARTESIAN_POINT('Ctrl Pts',(-1.92572846125756,1.,-3.35890824422965));
#67167=CARTESIAN_POINT('Ctrl Pts',(-1.92358838440528,1.,-3.35164424847223));
#67168=CARTESIAN_POINT('Ctrl Pts',(-1.92138450828404,1.,-3.34439448941961));
#67169=CARTESIAN_POINT('Ctrl Pts',(-1.9191460961021,1.,-3.33721230710012));
#67170=CARTESIAN_POINT('Ctrl Pts',(-1.91690081930331,1.,-3.33014884257873));
#67171=CARTESIAN_POINT('Ctrl Pts',(-1.91466343916628,1.,-3.32323403454535));
#67172=CARTESIAN_POINT('Ctrl Pts',(-1.91242616234442,1.,-3.31646052426364));
#67173=CARTESIAN_POINT('Ctrl Pts',(-1.91014297830446,1.,-3.30975721158596));
#67174=CARTESIAN_POINT('Ctrl Pts',(-1.90773912171341,1.,-3.30300595568195));
#67175=CARTESIAN_POINT('Ctrl Pts',(-1.90513891864087,1.,-3.29608978722113));
#67176=CARTESIAN_POINT('Ctrl Pts',(-1.90228971247527,1.,-3.2889344860029));
#67177=CARTESIAN_POINT('Ctrl Pts',(-1.89918429230462,1.,-3.28154737912352));
#67178=CARTESIAN_POINT('Ctrl Pts',(-1.89589172903793,1.,-3.27407108933139));
#67179=CARTESIAN_POINT('Ctrl Pts',(-1.89255393500965,1.,-3.26677653888676));
#67180=CARTESIAN_POINT('Ctrl Pts',(-1.88934996203698,1.,-3.25999885193947));
#67181=CARTESIAN_POINT('Ctrl Pts',(-1.88646802523466,1.,-3.25408686339463));
#67182=CARTESIAN_POINT('Ctrl Pts',(-1.88407708646357,1.,-3.24935200511918));
#67183=CARTESIAN_POINT('Ctrl Pts',(-1.88242596600454,1.,-3.2462565441079));
#67184=CARTESIAN_POINT('Ctrl Pts',(-1.88156537699203,1.,-3.24480754676064));
#67185=CARTESIAN_POINT('Ctrl Pts',(-1.88117508446775,1.,-3.24428080353022));
#67186=CARTESIAN_POINT('Ctrl Pts',(-1.8810229239812,1.,-3.24415531671284));
#67187=CARTESIAN_POINT('Ctrl Pts',(-1.88097764062697,1.,-3.24413672884812));
#67188=CARTESIAN_POINT('',(-1.97421938526992,0.,-3.70708211654725));
#67189=CARTESIAN_POINT('Ctrl Pts',(-1.519044091397,-1.,-3.42855728381368));
#67190=CARTESIAN_POINT('Ctrl Pts',(-1.519044091397,1.,-3.42855728381368));
#67191=CARTESIAN_POINT('Ctrl Pts',(-1.51896318668366,-1.,-3.42852521763778));
#67192=CARTESIAN_POINT('Ctrl Pts',(-1.51896318668366,1.,-3.42852521763778));
#67193=CARTESIAN_POINT('Ctrl Pts',(-1.51888450659652,-1.,-3.42860527149177));
#67194=CARTESIAN_POINT('Ctrl Pts',(-1.51888450659652,1.,-3.42860527149177));
#67195=CARTESIAN_POINT('Ctrl Pts',(-1.51901585839109,-1.,-3.42915787669893));
#67196=CARTESIAN_POINT('Ctrl Pts',(-1.51901585839109,1.,-3.42915787669893));
#67197=CARTESIAN_POINT('Ctrl Pts',(-1.51969006980999,-1.,-3.43076036253837));
#67198=CARTESIAN_POINT('Ctrl Pts',(-1.51969006980999,1.,-3.43076036253837));
#67199=CARTESIAN_POINT('Ctrl Pts',(-1.52134826724293,-1.,-3.43417156977893));
#67200=CARTESIAN_POINT('Ctrl Pts',(-1.52134826724293,1.,-3.43417156977893));
#67201=CARTESIAN_POINT('Ctrl Pts',(-1.5237734895035,-1.,-3.4388889597401));
#67202=CARTESIAN_POINT('Ctrl Pts',(-1.5237734895035,1.,-3.4388889597401));
#67203=CARTESIAN_POINT('Ctrl Pts',(-1.52686242875556,-1.,-3.44469547526647));
#67204=CARTESIAN_POINT('Ctrl Pts',(-1.52686242875556,1.,-3.44469547526647));
#67205=CARTESIAN_POINT('Ctrl Pts',(-1.53046244461635,-1.,-3.45127136828305));
#67206=CARTESIAN_POINT('Ctrl Pts',(-1.53046244461635,1.,-3.45127136828305));
#67207=CARTESIAN_POINT('Ctrl Pts',(-1.53440195378792,-1.,-3.45825932955032));
#67208=CARTESIAN_POINT('Ctrl Pts',(-1.53440195378792,1.,-3.45825932955032));
#67209=CARTESIAN_POINT('Ctrl Pts',(-1.53851507915502,-1.,-3.46531752207153));
#67210=CARTESIAN_POINT('Ctrl Pts',(-1.53851507915502,1.,-3.46531752207153));
#67211=CARTESIAN_POINT('Ctrl Pts',(-1.54266605398187,-1.,-3.47217189224653));
#67212=CARTESIAN_POINT('Ctrl Pts',(-1.54266605398187,1.,-3.47217189224653));
#67213=CARTESIAN_POINT('Ctrl Pts',(-1.54678009290276,-1.,-3.47868272898751));
#67214=CARTESIAN_POINT('Ctrl Pts',(-1.54678009290276,1.,-3.47868272898751));
#67215=CARTESIAN_POINT('Ctrl Pts',(-1.55084702970452,-1.,-3.48485155928567));
#67216=CARTESIAN_POINT('Ctrl Pts',(-1.55084702970452,1.,-3.48485155928567));
#67217=CARTESIAN_POINT('Ctrl Pts',(-1.55489595901116,-1.,-3.4907646087742));
#67218=CARTESIAN_POINT('Ctrl Pts',(-1.55489595901116,1.,-3.4907646087742));
#67219=CARTESIAN_POINT('Ctrl Pts',(-1.55897703097874,-1.,-3.49655185179655));
#67220=CARTESIAN_POINT('Ctrl Pts',(-1.55897703097874,1.,-3.49655185179655));
#67221=CARTESIAN_POINT('Ctrl Pts',(-1.56314187758675,-1.,-3.50234321621578));
#67222=CARTESIAN_POINT('Ctrl Pts',(-1.56314187758675,1.,-3.50234321621578));
#67223=CARTESIAN_POINT('Ctrl Pts',(-1.56742097575012,-1.,-3.50821771695363));
#67224=CARTESIAN_POINT('Ctrl Pts',(-1.56742097575012,1.,-3.50821771695363));
#67225=CARTESIAN_POINT('Ctrl Pts',(-1.57181569799743,-1.,-3.51418598431665));
#67226=CARTESIAN_POINT('Ctrl Pts',(-1.57181569799743,1.,-3.51418598431665));
#67227=CARTESIAN_POINT('Ctrl Pts',(-1.57631049988158,-1.,-3.52021847865912));
#67228=CARTESIAN_POINT('Ctrl Pts',(-1.57631049988158,1.,-3.52021847865912));
#67229=CARTESIAN_POINT('Ctrl Pts',(-1.58088027227848,-1.,-3.52626275334881));
#67230=CARTESIAN_POINT('Ctrl Pts',(-1.58088027227848,1.,-3.52626275334881));
#67231=CARTESIAN_POINT('Ctrl Pts',(-1.58549906268088,-1.,-3.5322637814708));
#67232=CARTESIAN_POINT('Ctrl Pts',(-1.58549906268088,1.,-3.5322637814708));
#67233=CARTESIAN_POINT('Ctrl Pts',(-1.59014958368739,-1.,-3.53818616861077));
#67234=CARTESIAN_POINT('Ctrl Pts',(-1.59014958368739,1.,-3.53818616861077));
#67235=CARTESIAN_POINT('Ctrl Pts',(-1.59482766949766,-1.,-3.54402458182337));
#67236=CARTESIAN_POINT('Ctrl Pts',(-1.59482766949766,1.,-3.54402458182337));
#67237=CARTESIAN_POINT('Ctrl Pts',(-1.59953698113457,-1.,-3.54979148634454));
#67238=CARTESIAN_POINT('Ctrl Pts',(-1.59953698113457,1.,-3.54979148634454));
#67239=CARTESIAN_POINT('Ctrl Pts',(-1.60428584699853,-1.,-3.55550985096129));
#67240=CARTESIAN_POINT('Ctrl Pts',(-1.60428584699853,1.,-3.55550985096129));
#67241=CARTESIAN_POINT('Ctrl Pts',(-1.60908344685457,-1.,-3.5612043248298));
#67242=CARTESIAN_POINT('Ctrl Pts',(-1.60908344685457,1.,-3.5612043248298));
#67243=CARTESIAN_POINT('Ctrl Pts',(-1.61393581747514,-1.,-3.56689200468387));
#67244=CARTESIAN_POINT('Ctrl Pts',(-1.61393581747514,1.,-3.56689200468387));
#67245=CARTESIAN_POINT('Ctrl Pts',(-1.61884340915404,-1.,-3.57257679609806));
#67246=CARTESIAN_POINT('Ctrl Pts',(-1.61884340915404,1.,-3.57257679609806));
#67247=CARTESIAN_POINT('Ctrl Pts',(-1.62380329464844,-1.,-3.5782545595439));
#67248=CARTESIAN_POINT('Ctrl Pts',(-1.62380329464844,1.,-3.5782545595439));
#67249=CARTESIAN_POINT('Ctrl Pts',(-1.62881051550745,-1.,-3.58391625774343));
#67250=CARTESIAN_POINT('Ctrl Pts',(-1.62881051550745,1.,-3.58391625774343));
#67251=CARTESIAN_POINT('Ctrl Pts',(-1.6338597145126,-1.,-3.58955176627879));
#67252=CARTESIAN_POINT('Ctrl Pts',(-1.6338597145126,1.,-3.58955176627879));
#67253=CARTESIAN_POINT('Ctrl Pts',(-1.63894676675352,-1.,-3.59515368334893));
#67254=CARTESIAN_POINT('Ctrl Pts',(-1.63894676675352,1.,-3.59515368334893));
#67255=CARTESIAN_POINT('Ctrl Pts',(-1.64407004385582,-1.,-3.60072028513845));
#67256=CARTESIAN_POINT('Ctrl Pts',(-1.64407004385582,1.,-3.60072028513845));
#67257=CARTESIAN_POINT('Ctrl Pts',(-1.64922952425832,-1.,-3.60625346556992));
#67258=CARTESIAN_POINT('Ctrl Pts',(-1.64922952425832,1.,-3.60625346556992));
#67259=CARTESIAN_POINT('Ctrl Pts',(-1.65442619244325,-1.,-3.61175734965127));
#67260=CARTESIAN_POINT('Ctrl Pts',(-1.65442619244325,1.,-3.61175734965127));
#67261=CARTESIAN_POINT('Ctrl Pts',(-1.65966133399186,-1.,-3.61723666482456));
#67262=CARTESIAN_POINT('Ctrl Pts',(-1.65966133399186,1.,-3.61723666482456));
#67263=CARTESIAN_POINT('Ctrl Pts',(-1.66493585923855,-1.,-3.62269517989109));
#67264=CARTESIAN_POINT('Ctrl Pts',(-1.66493585923855,1.,-3.62269517989109));
#67265=CARTESIAN_POINT('Ctrl Pts',(-1.67024966008045,-1.,-3.62813422105271));
#67266=CARTESIAN_POINT('Ctrl Pts',(-1.67024966008045,1.,-3.62813422105271));
#67267=CARTESIAN_POINT('Ctrl Pts',(-1.67560193613156,-1.,-3.63355343201232));
#67268=CARTESIAN_POINT('Ctrl Pts',(-1.67560193613156,1.,-3.63355343201232));
#67269=CARTESIAN_POINT('Ctrl Pts',(-1.68099146651586,-1.,-3.63895140887462));
#67270=CARTESIAN_POINT('Ctrl Pts',(-1.68099146651586,1.,-3.63895140887462));
#67271=CARTESIAN_POINT('Ctrl Pts',(-1.68641690471457,-1.,-3.64432638915203));
#67272=CARTESIAN_POINT('Ctrl Pts',(-1.68641690471457,1.,-3.64432638915203));
#67273=CARTESIAN_POINT('Ctrl Pts',(-1.69187705481689,-1.,-3.64967689827371));
#67274=CARTESIAN_POINT('Ctrl Pts',(-1.69187705481689,1.,-3.64967689827371));
#67275=CARTESIAN_POINT('Ctrl Pts',(-1.69737117722534,-1.,-3.65500246526749));
#67276=CARTESIAN_POINT('Ctrl Pts',(-1.69737117722534,1.,-3.65500246526749));
#67277=CARTESIAN_POINT('Ctrl Pts',(-1.70289888566873,-1.,-3.66030338774847));
#67278=CARTESIAN_POINT('Ctrl Pts',(-1.70289888566873,1.,-3.66030338774847));
#67279=CARTESIAN_POINT('Ctrl Pts',(-1.70846001610956,-1.,-3.66558043198876));
#67280=CARTESIAN_POINT('Ctrl Pts',(-1.70846001610956,1.,-3.66558043198876));
#67281=CARTESIAN_POINT('Ctrl Pts',(-1.71405450210384,-1.,-3.67083454901611));
#67282=CARTESIAN_POINT('Ctrl Pts',(-1.71405450210384,1.,-3.67083454901611));
#67283=CARTESIAN_POINT('Ctrl Pts',(-1.71968225581808,-1.,-3.67606660374709));
#67284=CARTESIAN_POINT('Ctrl Pts',(-1.71968225581808,1.,-3.67606660374709));
#67285=CARTESIAN_POINT('Ctrl Pts',(-1.72534302437056,-1.,-3.68127704936579));
#67286=CARTESIAN_POINT('Ctrl Pts',(-1.72534302437056,1.,-3.68127704936579));
#67287=CARTESIAN_POINT('Ctrl Pts',(-1.73103640956717,-1.,-3.68646597019332));
#67288=CARTESIAN_POINT('Ctrl Pts',(-1.73103640956717,1.,-3.68646597019332));
#67289=CARTESIAN_POINT('Ctrl Pts',(-1.73676193254557,-1.,-3.69163322648036));
#67290=CARTESIAN_POINT('Ctrl Pts',(-1.73676193254557,1.,-3.69163322648036));
#67291=CARTESIAN_POINT('Ctrl Pts',(-1.74251908492617,-1.,-3.69677856910517));
#67292=CARTESIAN_POINT('Ctrl Pts',(-1.74251908492617,1.,-3.69677856910517));
#67293=CARTESIAN_POINT('Ctrl Pts',(-1.74830738046057,-1.,-3.7019017567335));
#67294=CARTESIAN_POINT('Ctrl Pts',(-1.74830738046057,1.,-3.7019017567335));
#67295=CARTESIAN_POINT('Ctrl Pts',(-1.75412641804042,-1.,-3.70700269736659));
#67296=CARTESIAN_POINT('Ctrl Pts',(-1.75412641804042,1.,-3.70700269736659));
#67297=CARTESIAN_POINT('Ctrl Pts',(-1.75997588498865,-1.,-3.71208146346136));
#67298=CARTESIAN_POINT('Ctrl Pts',(-1.75997588498865,1.,-3.71208146346136));
#67299=CARTESIAN_POINT('Ctrl Pts',(-1.76585552124394,-1.,-3.71713822377359));
#67300=CARTESIAN_POINT('Ctrl Pts',(-1.76585552124394,1.,-3.71713822377359));
#67301=CARTESIAN_POINT('Ctrl Pts',(-1.77176509401761,-1.,-3.72217319911254));
#67302=CARTESIAN_POINT('Ctrl Pts',(-1.77176509401761,1.,-3.72217319911254));
#67303=CARTESIAN_POINT('Ctrl Pts',(-1.77770437039658,-1.,-3.72718661205609));
#67304=CARTESIAN_POINT('Ctrl Pts',(-1.77770437039658,1.,-3.72718661205609));
#67305=CARTESIAN_POINT('Ctrl Pts',(-1.78367308442901,-1.,-3.7321786309547));
#67306=CARTESIAN_POINT('Ctrl Pts',(-1.78367308442901,1.,-3.7321786309547));
#67307=CARTESIAN_POINT('Ctrl Pts',(-1.78967092823491,-1.,-3.73714934730681));
#67308=CARTESIAN_POINT('Ctrl Pts',(-1.78967092823491,1.,-3.73714934730681));
#67309=CARTESIAN_POINT('Ctrl Pts',(-1.79569757859422,-1.,-3.74209880352445));
#67310=CARTESIAN_POINT('Ctrl Pts',(-1.79569757859422,1.,-3.74209880352445));
#67311=CARTESIAN_POINT('Ctrl Pts',(-1.8017527148577,-1.,-3.74702700875467));
#67312=CARTESIAN_POINT('Ctrl Pts',(-1.8017527148577,1.,-3.74702700875467));
#67313=CARTESIAN_POINT('Ctrl Pts',(-1.80783603939617,-1.,-3.75193395887977));
#67314=CARTESIAN_POINT('Ctrl Pts',(-1.80783603939617,1.,-3.75193395887977));
#67315=CARTESIAN_POINT('Ctrl Pts',(-1.8139472983358,-1.,-3.75681965683071));
#67316=CARTESIAN_POINT('Ctrl Pts',(-1.8139472983358,1.,-3.75681965683071));
#67317=CARTESIAN_POINT('Ctrl Pts',(-1.82008629694091,-1.,-3.76168412707948));
#67318=CARTESIAN_POINT('Ctrl Pts',(-1.82008629694091,1.,-3.76168412707948));
#67319=CARTESIAN_POINT('Ctrl Pts',(-1.82625289220915,-1.,-3.76652740353775));
#67320=CARTESIAN_POINT('Ctrl Pts',(-1.82625289220915,1.,-3.76652740353775));
#67321=CARTESIAN_POINT('Ctrl Pts',(-1.83120816955645,-1.,-3.77038509817999));
#67322=CARTESIAN_POINT('Ctrl Pts',(-1.83120816955645,1.,-3.77038509817999));
#67323=CARTESIAN_POINT('Ctrl Pts',(-1.83493697934534,-1.,-3.77326886064398));
#67324=CARTESIAN_POINT('Ctrl Pts',(-1.83493697934534,1.,-3.77326886064398));
#67325=CARTESIAN_POINT('Ctrl Pts',(-1.83742834010626,-1.,-3.77518714457833));
#67326=CARTESIAN_POINT('Ctrl Pts',(-1.83742834010626,1.,-3.77518714457833));
#67327=CARTESIAN_POINT('Ctrl Pts',(-1.83867539237861,-1.,-3.77614523045147));
#67328=CARTESIAN_POINT('Ctrl Pts',(-1.83867539237861,1.,-3.77614523045147));
#67329=CARTESIAN_POINT('',(-1.5189508286633,1.,-3.42859860294306));
#67330=CARTESIAN_POINT('Ctrl Pts',(-1.5189508286633,-1.,-3.42859860294306));
#67331=CARTESIAN_POINT('Ctrl Pts',(-1.5189508286633,-0.666666666666667,
-3.42859860294306));
#67332=CARTESIAN_POINT('Ctrl Pts',(-1.5189508286633,-0.333333333333333,
-3.42859860294306));
#67333=CARTESIAN_POINT('Ctrl Pts',(-1.5189508286633,0.333333333333333,-3.42859860294306));
#67334=CARTESIAN_POINT('Ctrl Pts',(-1.5189508286633,0.666666666666667,-3.42859860294305));
#67335=CARTESIAN_POINT('Ctrl Pts',(-1.5189508286633,1.,-3.42859860294305));
#67336=CARTESIAN_POINT('',(-1.83867539237861,1.,-3.77614523045147));
#67337=CARTESIAN_POINT('',(-1.83867539237861,0.,-3.77614523045147));
#67338=CARTESIAN_POINT('Ctrl Pts',(-1.5189508286633,1.,-3.42859860294306));
#67339=CARTESIAN_POINT('Ctrl Pts',(-1.51893924967331,1.,-3.42864616361875));
#67340=CARTESIAN_POINT('Ctrl Pts',(-1.5189513329503,1.,-3.42884302333841));
#67341=CARTESIAN_POINT('Ctrl Pts',(-1.51914806898491,1.,-3.42946838852588));
#67342=CARTESIAN_POINT('Ctrl Pts',(-1.5198144909338,1.,-3.43101631893414));
#67343=CARTESIAN_POINT('Ctrl Pts',(-1.52134826724293,1.,-3.43417156977893));
#67344=CARTESIAN_POINT('Ctrl Pts',(-1.5237734895035,1.,-3.4388889597401));
#67345=CARTESIAN_POINT('Ctrl Pts',(-1.52686242875556,1.,-3.44469547526647));
#67346=CARTESIAN_POINT('Ctrl Pts',(-1.53046244461635,1.,-3.45127136828305));
#67347=CARTESIAN_POINT('Ctrl Pts',(-1.53440195378792,1.,-3.45825932955032));
#67348=CARTESIAN_POINT('Ctrl Pts',(-1.53851507915502,1.,-3.46531752207153));
#67349=CARTESIAN_POINT('Ctrl Pts',(-1.54266605398187,1.,-3.47217189224653));
#67350=CARTESIAN_POINT('Ctrl Pts',(-1.54678009290276,1.,-3.47868272898751));
#67351=CARTESIAN_POINT('Ctrl Pts',(-1.55084702970452,1.,-3.48485155928567));
#67352=CARTESIAN_POINT('Ctrl Pts',(-1.55489595901116,1.,-3.4907646087742));
#67353=CARTESIAN_POINT('Ctrl Pts',(-1.55897703097874,1.,-3.49655185179655));
#67354=CARTESIAN_POINT('Ctrl Pts',(-1.56314187758675,1.,-3.50234321621578));
#67355=CARTESIAN_POINT('Ctrl Pts',(-1.56742097575012,1.,-3.50821771695363));
#67356=CARTESIAN_POINT('Ctrl Pts',(-1.57181569799743,1.,-3.51418598431665));
#67357=CARTESIAN_POINT('Ctrl Pts',(-1.57631049988158,1.,-3.52021847865912));
#67358=CARTESIAN_POINT('Ctrl Pts',(-1.58088027227848,1.,-3.52626275334881));
#67359=CARTESIAN_POINT('Ctrl Pts',(-1.58549906268088,1.,-3.5322637814708));
#67360=CARTESIAN_POINT('Ctrl Pts',(-1.59014958368739,1.,-3.53818616861077));
#67361=CARTESIAN_POINT('Ctrl Pts',(-1.59482766949766,1.,-3.54402458182337));
#67362=CARTESIAN_POINT('Ctrl Pts',(-1.59953698113457,1.,-3.54979148634454));
#67363=CARTESIAN_POINT('Ctrl Pts',(-1.60428584699853,1.,-3.55550985096129));
#67364=CARTESIAN_POINT('Ctrl Pts',(-1.60908344685457,1.,-3.5612043248298));
#67365=CARTESIAN_POINT('Ctrl Pts',(-1.61393581747514,1.,-3.56689200468387));
#67366=CARTESIAN_POINT('Ctrl Pts',(-1.61884340915404,1.,-3.57257679609806));
#67367=CARTESIAN_POINT('Ctrl Pts',(-1.62380329464844,1.,-3.5782545595439));
#67368=CARTESIAN_POINT('Ctrl Pts',(-1.62881051550745,1.,-3.58391625774343));
#67369=CARTESIAN_POINT('Ctrl Pts',(-1.6338597145126,1.,-3.58955176627879));
#67370=CARTESIAN_POINT('Ctrl Pts',(-1.63894676675352,1.,-3.59515368334893));
#67371=CARTESIAN_POINT('Ctrl Pts',(-1.64407004385582,1.,-3.60072028513845));
#67372=CARTESIAN_POINT('Ctrl Pts',(-1.64922952425832,1.,-3.60625346556992));
#67373=CARTESIAN_POINT('Ctrl Pts',(-1.65442619244325,1.,-3.61175734965127));
#67374=CARTESIAN_POINT('Ctrl Pts',(-1.65966133399186,1.,-3.61723666482456));
#67375=CARTESIAN_POINT('Ctrl Pts',(-1.66493585923855,1.,-3.62269517989109));
#67376=CARTESIAN_POINT('Ctrl Pts',(-1.67024966008045,1.,-3.62813422105271));
#67377=CARTESIAN_POINT('Ctrl Pts',(-1.67560193613156,1.,-3.63355343201232));
#67378=CARTESIAN_POINT('Ctrl Pts',(-1.68099146651586,1.,-3.63895140887462));
#67379=CARTESIAN_POINT('Ctrl Pts',(-1.68641690471457,1.,-3.64432638915203));
#67380=CARTESIAN_POINT('Ctrl Pts',(-1.69187705481689,1.,-3.64967689827371));
#67381=CARTESIAN_POINT('Ctrl Pts',(-1.69737117722534,1.,-3.65500246526749));
#67382=CARTESIAN_POINT('Ctrl Pts',(-1.70289888566873,1.,-3.66030338774847));
#67383=CARTESIAN_POINT('Ctrl Pts',(-1.70846001610956,1.,-3.66558043198876));
#67384=CARTESIAN_POINT('Ctrl Pts',(-1.71405450210384,1.,-3.67083454901611));
#67385=CARTESIAN_POINT('Ctrl Pts',(-1.71968225581808,1.,-3.67606660374709));
#67386=CARTESIAN_POINT('Ctrl Pts',(-1.72534302437056,1.,-3.68127704936579));
#67387=CARTESIAN_POINT('Ctrl Pts',(-1.73103640956717,1.,-3.68646597019332));
#67388=CARTESIAN_POINT('Ctrl Pts',(-1.73676193254557,1.,-3.69163322648036));
#67389=CARTESIAN_POINT('Ctrl Pts',(-1.74251908492617,1.,-3.69677856910517));
#67390=CARTESIAN_POINT('Ctrl Pts',(-1.74830738046057,1.,-3.7019017567335));
#67391=CARTESIAN_POINT('Ctrl Pts',(-1.75412641804042,1.,-3.70700269736659));
#67392=CARTESIAN_POINT('Ctrl Pts',(-1.75997588498865,1.,-3.71208146346136));
#67393=CARTESIAN_POINT('Ctrl Pts',(-1.76585552124394,1.,-3.71713822377359));
#67394=CARTESIAN_POINT('Ctrl Pts',(-1.77176509401761,1.,-3.72217319911254));
#67395=CARTESIAN_POINT('Ctrl Pts',(-1.77770437039658,1.,-3.72718661205609));
#67396=CARTESIAN_POINT('Ctrl Pts',(-1.78367308442901,1.,-3.7321786309547));
#67397=CARTESIAN_POINT('Ctrl Pts',(-1.78967092823491,1.,-3.73714934730681));
#67398=CARTESIAN_POINT('Ctrl Pts',(-1.79569757859422,1.,-3.74209880352445));
#67399=CARTESIAN_POINT('Ctrl Pts',(-1.8017527148577,1.,-3.74702700875467));
#67400=CARTESIAN_POINT('Ctrl Pts',(-1.80783603939617,1.,-3.75193395887977));
#67401=CARTESIAN_POINT('Ctrl Pts',(-1.8139472983358,1.,-3.75681965683071));
#67402=CARTESIAN_POINT('Ctrl Pts',(-1.82008629694091,1.,-3.76168412707948));
#67403=CARTESIAN_POINT('Ctrl Pts',(-1.82625289220915,1.,-3.76652740353775));
#67404=CARTESIAN_POINT('Ctrl Pts',(-1.83120816955645,1.,-3.77038509817999));
#67405=CARTESIAN_POINT('Ctrl Pts',(-1.83493697934534,1.,-3.77326886064398));
#67406=CARTESIAN_POINT('Ctrl Pts',(-1.83742834010626,1.,-3.77518714457833));
#67407=CARTESIAN_POINT('Ctrl Pts',(-1.83867539237861,1.,-3.77614523045147));
#67408=CARTESIAN_POINT('Origin',(-1.83867539237861,0.,-3.77614523045147));
#67409=CARTESIAN_POINT('',(-1.97421938526992,1.,-3.70708211654725));
#67410=CARTESIAN_POINT('Origin',(0.,0.,0.));
#67411=CARTESIAN_POINT('',(-1.35032489087269,1.,-3.49844575334386));
#67412=CARTESIAN_POINT('Origin',(0.,1.,0.));
#67413=CARTESIAN_POINT('Ctrl Pts',(-1.35032489087269,1.,-3.49844575334386));
#67414=CARTESIAN_POINT('Ctrl Pts',(-1.35032489087269,0.666666666666667,
-3.49844575334386));
#67415=CARTESIAN_POINT('Ctrl Pts',(-1.35032489087269,0.333333333333333,
-3.49844575334386));
#67416=CARTESIAN_POINT('Ctrl Pts',(-1.35032489087269,-0.333333333333333,
-3.49844575334386));
#67417=CARTESIAN_POINT('Ctrl Pts',(-1.35032489087269,-0.666666666666667,
-3.49844575334386));
#67418=CARTESIAN_POINT('Ctrl Pts',(-1.35032489087269,-1.,-3.49844575334386));
#67419=CARTESIAN_POINT('Ctrl Pts',(-1.36999806084572,-1.,-3.97027773754922));
#67420=CARTESIAN_POINT('Ctrl Pts',(-1.36999806084572,1.,-3.97027773754922));
#67421=CARTESIAN_POINT('Ctrl Pts',(-1.37020239094758,-1.,-3.9687184694173));
#67422=CARTESIAN_POINT('Ctrl Pts',(-1.37020239094758,1.,-3.9687184694173));
#67423=CARTESIAN_POINT('Ctrl Pts',(-1.37060761746027,-1.,-3.96560037975788));
#67424=CARTESIAN_POINT('Ctrl Pts',(-1.37060761746027,1.,-3.96560037975788));
#67425=CARTESIAN_POINT('Ctrl Pts',(-1.37120515615663,-1.,-3.96092458508407));
#67426=CARTESIAN_POINT('Ctrl Pts',(-1.37120515615663,1.,-3.96092458508407));
#67427=CARTESIAN_POINT('Ctrl Pts',(-1.37198126433139,-1.,-3.95469287283105));
#67428=CARTESIAN_POINT('Ctrl Pts',(-1.37198126433139,1.,-3.95469287283105));
#67429=CARTESIAN_POINT('Ctrl Pts',(-1.37291699203423,-1.,-3.94690771786926));
#67430=CARTESIAN_POINT('Ctrl Pts',(-1.37291699203423,1.,-3.94690771786926));
#67431=CARTESIAN_POINT('Ctrl Pts',(-1.37381821967499,-1.,-3.93912709041791));
#67432=CARTESIAN_POINT('Ctrl Pts',(-1.37381821967499,1.,-3.93912709041791));
#67433=CARTESIAN_POINT('Ctrl Pts',(-1.37468482215784,-1.,-3.93135106761941));
#67434=CARTESIAN_POINT('Ctrl Pts',(-1.37468482215784,1.,-3.93135106761941));
#67435=CARTESIAN_POINT('Ctrl Pts',(-1.37551664448057,-1.,-3.92357976987132));
#67436=CARTESIAN_POINT('Ctrl Pts',(-1.37551664448057,1.,-3.92357976987132));
#67437=CARTESIAN_POINT('Ctrl Pts',(-1.37631350505516,-1.,-3.91581337461825));
#67438=CARTESIAN_POINT('Ctrl Pts',(-1.37631350505516,1.,-3.91581337461825));
#67439=CARTESIAN_POINT('Ctrl Pts',(-1.3770751963376,-1.,-3.90805209522729));
#67440=CARTESIAN_POINT('Ctrl Pts',(-1.3770751963376,1.,-3.90805209522729));
#67441=CARTESIAN_POINT('Ctrl Pts',(-1.3778014851263,-1.,-3.90029615196255));
#67442=CARTESIAN_POINT('Ctrl Pts',(-1.3778014851263,1.,-3.90029615196255));
#67443=CARTESIAN_POINT('Ctrl Pts',(-1.37849211287981,-1.,-3.89254574338385));
#67444=CARTESIAN_POINT('Ctrl Pts',(-1.37849211287981,1.,-3.89254574338385));
#67445=CARTESIAN_POINT('Ctrl Pts',(-1.37914679719446,-1.,-3.88480102249461));
#67446=CARTESIAN_POINT('Ctrl Pts',(-1.37914679719446,1.,-3.88480102249461));
#67447=CARTESIAN_POINT('Ctrl Pts',(-1.37976523097187,-1.,-3.87706205830865));
#67448=CARTESIAN_POINT('Ctrl Pts',(-1.37976523097187,1.,-3.87706205830865));
#67449=CARTESIAN_POINT('Ctrl Pts',(-1.38034709213129,-1.,-3.86932885813403));
#67450=CARTESIAN_POINT('Ctrl Pts',(-1.38034709213129,1.,-3.86932885813403));
#67451=CARTESIAN_POINT('Ctrl Pts',(-1.38089205993067,-1.,-3.86160143044187));
#67452=CARTESIAN_POINT('Ctrl Pts',(-1.38089205993067,1.,-3.86160143044187));
#67453=CARTESIAN_POINT('Ctrl Pts',(-1.38139983115075,-1.,-3.85387983979557));
#67454=CARTESIAN_POINT('Ctrl Pts',(-1.38139983115075,1.,-3.85387983979557));
#67455=CARTESIAN_POINT('Ctrl Pts',(-1.38187013346089,-1.,-3.84616425605705));
#67456=CARTESIAN_POINT('Ctrl Pts',(-1.38187013346089,1.,-3.84616425605705));
#67457=CARTESIAN_POINT('Ctrl Pts',(-1.38230274828774,-1.,-3.83845502790609));
#67458=CARTESIAN_POINT('Ctrl Pts',(-1.38230274828774,1.,-3.83845502790609));
#67459=CARTESIAN_POINT('Ctrl Pts',(-1.38269750245086,-1.,-3.83075266982138));
#67460=CARTESIAN_POINT('Ctrl Pts',(-1.38269750245086,1.,-3.83075266982138));
#67461=CARTESIAN_POINT('Ctrl Pts',(-1.38305421262724,-1.,-3.82305771743715));
#67462=CARTESIAN_POINT('Ctrl Pts',(-1.38305421262724,1.,-3.82305771743715));
#67463=CARTESIAN_POINT('Ctrl Pts',(-1.38337263902766,-1.,-3.81537060817765));
#67464=CARTESIAN_POINT('Ctrl Pts',(-1.38337263902766,1.,-3.81537060817765));
#67465=CARTESIAN_POINT('Ctrl Pts',(-1.38365244046226,-1.,-3.80769156398429));
#67466=CARTESIAN_POINT('Ctrl Pts',(-1.38365244046226,1.,-3.80769156398429));
#67467=CARTESIAN_POINT('Ctrl Pts',(-1.38389311766701,-1.,-3.80002044322169));
#67468=CARTESIAN_POINT('Ctrl Pts',(-1.38389311766701,1.,-3.80002044322169));
#67469=CARTESIAN_POINT('Ctrl Pts',(-1.38409399694589,-1.,-3.79235669640907));
#67470=CARTESIAN_POINT('Ctrl Pts',(-1.38409399694589,1.,-3.79235669640907));
#67471=CARTESIAN_POINT('Ctrl Pts',(-1.38425435883773,-1.,-3.78469969805134));
#67472=CARTESIAN_POINT('Ctrl Pts',(-1.38425435883773,1.,-3.78469969805134));
#67473=CARTESIAN_POINT('Ctrl Pts',(-1.38437354551435,-1.,-3.77704902230441));
#67474=CARTESIAN_POINT('Ctrl Pts',(-1.38437354551435,1.,-3.77704902230441));
#67475=CARTESIAN_POINT('Ctrl Pts',(-1.38445107339517,-1.,-3.76940473185775));
#67476=CARTESIAN_POINT('Ctrl Pts',(-1.38445107339517,1.,-3.76940473185775));
#67477=CARTESIAN_POINT('Ctrl Pts',(-1.38448675253343,-1.,-3.76176768271347));
#67478=CARTESIAN_POINT('Ctrl Pts',(-1.38448675253343,1.,-3.76176768271347));
#67479=CARTESIAN_POINT('Ctrl Pts',(-1.38448077997155,-1.,-3.75413976318727));
#67480=CARTESIAN_POINT('Ctrl Pts',(-1.38448077997155,1.,-3.75413976318727));
#67481=CARTESIAN_POINT('Ctrl Pts',(-1.38443344984389,-1.,-3.7465231716786));
#67482=CARTESIAN_POINT('Ctrl Pts',(-1.38443344984389,1.,-3.7465231716786));
#67483=CARTESIAN_POINT('Ctrl Pts',(-1.38434489156456,-1.,-3.73891976418099));
#67484=CARTESIAN_POINT('Ctrl Pts',(-1.38434489156456,1.,-3.73891976418099));
#67485=CARTESIAN_POINT('Ctrl Pts',(-1.38421479111531,-1.,-3.73133035859283));
#67486=CARTESIAN_POINT('Ctrl Pts',(-1.38421479111531,1.,-3.73133035859283));
#67487=CARTESIAN_POINT('Ctrl Pts',(-1.3840421342895,-1.,-3.72375409358805));
#67488=CARTESIAN_POINT('Ctrl Pts',(-1.3840421342895,1.,-3.72375409358805));
#67489=CARTESIAN_POINT('Ctrl Pts',(-1.38382489984585,-1.,-3.7161876605181));
#67490=CARTESIAN_POINT('Ctrl Pts',(-1.38382489984585,1.,-3.7161876605181));
#67491=CARTESIAN_POINT('Ctrl Pts',(-1.38356065402122,-1.,-3.70862680753343));
#67492=CARTESIAN_POINT('Ctrl Pts',(-1.38356065402122,1.,-3.70862680753343));
#67493=CARTESIAN_POINT('Ctrl Pts',(-1.38324717612862,-1.,-3.70106792167894));
#67494=CARTESIAN_POINT('Ctrl Pts',(-1.38324717612862,1.,-3.70106792167894));
#67495=CARTESIAN_POINT('Ctrl Pts',(-1.38288311171649,-1.,-3.69350967899523));
#67496=CARTESIAN_POINT('Ctrl Pts',(-1.38288311171649,1.,-3.69350967899523));
#67497=CARTESIAN_POINT('Ctrl Pts',(-1.38246852827185,-1.,-3.68595444983844));
#67498=CARTESIAN_POINT('Ctrl Pts',(-1.38246852827185,1.,-3.68595444983844));
#67499=CARTESIAN_POINT('Ctrl Pts',(-1.38200574290626,-1.,-3.6784103848243));
#67500=CARTESIAN_POINT('Ctrl Pts',(-1.38200574290626,1.,-3.6784103848243));
#67501=CARTESIAN_POINT('Ctrl Pts',(-1.38149812653876,-1.,-3.67088843112282));
#67502=CARTESIAN_POINT('Ctrl Pts',(-1.38149812653876,1.,-3.67088843112282));
#67503=CARTESIAN_POINT('Ctrl Pts',(-1.38094856333558,-1.,-3.66339848520874));
#67504=CARTESIAN_POINT('Ctrl Pts',(-1.38094856333558,1.,-3.66339848520874));
#67505=CARTESIAN_POINT('Ctrl Pts',(-1.38035791051215,-1.,-3.65594554404396));
#67506=CARTESIAN_POINT('Ctrl Pts',(-1.38035791051215,1.,-3.65594554404396));
#67507=CARTESIAN_POINT('Ctrl Pts',(-1.37972372481598,-1.,-3.64852652756444));
#67508=CARTESIAN_POINT('Ctrl Pts',(-1.37972372481598,1.,-3.64852652756444));
#67509=CARTESIAN_POINT('Ctrl Pts',(-1.37903818567347,-1.,-3.64112507791112));
#67510=CARTESIAN_POINT('Ctrl Pts',(-1.37903818567347,1.,-3.64112507791112));
#67511=CARTESIAN_POINT('Ctrl Pts',(-1.37829035457324,-1.,-3.63371727442448));
#67512=CARTESIAN_POINT('Ctrl Pts',(-1.37829035457324,1.,-3.63371727442448));
#67513=CARTESIAN_POINT('Ctrl Pts',(-1.37746987919868,-1.,-3.62628098665112));
#67514=CARTESIAN_POINT('Ctrl Pts',(-1.37746987919868,1.,-3.62628098665112));
#67515=CARTESIAN_POINT('Ctrl Pts',(-1.37657053403102,-1.,-3.61880481160408));
#67516=CARTESIAN_POINT('Ctrl Pts',(-1.37657053403102,1.,-3.61880481160408));
#67517=CARTESIAN_POINT('Ctrl Pts',(-1.37559314436641,-1.,-3.61129546591082));
#67518=CARTESIAN_POINT('Ctrl Pts',(-1.37559314436641,1.,-3.61129546591082));
#67519=CARTESIAN_POINT('Ctrl Pts',(-1.37455051379642,-1.,-3.60379020124038));
#67520=CARTESIAN_POINT('Ctrl Pts',(-1.37455051379642,1.,-3.60379020124038));
#67521=CARTESIAN_POINT('Ctrl Pts',(-1.37346320103184,-1.,-3.59634627869117));
#67522=CARTESIAN_POINT('Ctrl Pts',(-1.37346320103184,1.,-3.59634627869117));
#67523=CARTESIAN_POINT('Ctrl Pts',(-1.37235053661,-1.,-3.5890185384643));
#67524=CARTESIAN_POINT('Ctrl Pts',(-1.37235053661,1.,-3.5890185384643));
#67525=CARTESIAN_POINT('Ctrl Pts',(-1.37122241663073,-1.,-3.58183885982745));
#67526=CARTESIAN_POINT('Ctrl Pts',(-1.37122241663073,1.,-3.58183885982745));
#67527=CARTESIAN_POINT('Ctrl Pts',(-1.37007229485646,-1.,-3.57479875549453));
#67528=CARTESIAN_POINT('Ctrl Pts',(-1.37007229485646,1.,-3.57479875549453));
#67529=CARTESIAN_POINT('Ctrl Pts',(-1.36886584973349,-1.,-3.56782080304554));
#67530=CARTESIAN_POINT('Ctrl Pts',(-1.36886584973349,1.,-3.56782080304554));
#67531=CARTESIAN_POINT('Ctrl Pts',(-1.36754771771174,-1.,-3.56077662028492));
#67532=CARTESIAN_POINT('Ctrl Pts',(-1.36754771771174,1.,-3.56077662028492));
#67533=CARTESIAN_POINT('Ctrl Pts',(-1.36606145456711,-1.,-3.55353883995793));
#67534=CARTESIAN_POINT('Ctrl Pts',(-1.36606145456711,1.,-3.55353883995793));
#67535=CARTESIAN_POINT('Ctrl Pts',(-1.36436666257567,-1.,-3.54602591832893));
#67536=CARTESIAN_POINT('Ctrl Pts',(-1.36436666257567,1.,-3.54602591832893));
#67537=CARTESIAN_POINT('Ctrl Pts',(-1.36245507339334,-1.,-3.53824396425032));
#67538=CARTESIAN_POINT('Ctrl Pts',(-1.36245507339334,1.,-3.53824396425032));
#67539=CARTESIAN_POINT('Ctrl Pts',(-1.36037259643827,-1.,-3.53034464961849));
#67540=CARTESIAN_POINT('Ctrl Pts',(-1.36037259643827,1.,-3.53034464961849));
#67541=CARTESIAN_POINT('Ctrl Pts',(-1.35821701528975,-1.,-3.52261776117121));
#67542=CARTESIAN_POINT('Ctrl Pts',(-1.35821701528975,1.,-3.52261776117121));
#67543=CARTESIAN_POINT('Ctrl Pts',(-1.35611275237288,-1.,-3.51542230699919));
#67544=CARTESIAN_POINT('Ctrl Pts',(-1.35611275237288,1.,-3.51542230699919));
#67545=CARTESIAN_POINT('Ctrl Pts',(-1.35419113576022,-1.,-3.50913227060177));
#67546=CARTESIAN_POINT('Ctrl Pts',(-1.35419113576022,1.,-3.50913227060177));
#67547=CARTESIAN_POINT('Ctrl Pts',(-1.3525703284343,-1.,-3.50408168106113));
#67548=CARTESIAN_POINT('Ctrl Pts',(-1.3525703284343,1.,-3.50408168106113));
#67549=CARTESIAN_POINT('Ctrl Pts',(-1.35133076331065,-1.,-3.50049707063673));
#67550=CARTESIAN_POINT('Ctrl Pts',(-1.35133076331065,1.,-3.50049707063673));
#67551=CARTESIAN_POINT('Ctrl Pts',(-1.35067437417289,-1.,-3.49888720256612));
#67552=CARTESIAN_POINT('Ctrl Pts',(-1.35067437417289,1.,-3.49888720256612));
#67553=CARTESIAN_POINT('Ctrl Pts',(-1.35037650302887,-1.,-3.49840357193384));
#67554=CARTESIAN_POINT('Ctrl Pts',(-1.35037650302887,1.,-3.49840357193384));
#67555=CARTESIAN_POINT('Ctrl Pts',(-1.35026426118351,-1.,-3.49840260053616));
#67556=CARTESIAN_POINT('Ctrl Pts',(-1.35026426118351,1.,-3.49840260053616));
#67557=CARTESIAN_POINT('Ctrl Pts',(-1.35022972712301,-1.,-3.49848248301936));
#67558=CARTESIAN_POINT('Ctrl Pts',(-1.35022972712301,1.,-3.49848248301936));
#67559=CARTESIAN_POINT('',(-1.36999806084572,1.,-3.97027773754922));
#67560=CARTESIAN_POINT('Ctrl Pts',(-1.36999806084572,1.,-3.97027773754922));
#67561=CARTESIAN_POINT('Ctrl Pts',(-1.37020239094758,1.,-3.9687184694173));
#67562=CARTESIAN_POINT('Ctrl Pts',(-1.37060761746027,1.,-3.96560037975788));
#67563=CARTESIAN_POINT('Ctrl Pts',(-1.37120515615663,1.,-3.96092458508407));
#67564=CARTESIAN_POINT('Ctrl Pts',(-1.37198126433139,1.,-3.95469287283105));
#67565=CARTESIAN_POINT('Ctrl Pts',(-1.37291699203423,1.,-3.94690771786926));
#67566=CARTESIAN_POINT('Ctrl Pts',(-1.37381821967499,1.,-3.93912709041791));
#67567=CARTESIAN_POINT('Ctrl Pts',(-1.37468482215784,1.,-3.93135106761941));
#67568=CARTESIAN_POINT('Ctrl Pts',(-1.37551664448057,1.,-3.92357976987132));
#67569=CARTESIAN_POINT('Ctrl Pts',(-1.37631350505516,1.,-3.91581337461825));
#67570=CARTESIAN_POINT('Ctrl Pts',(-1.3770751963376,1.,-3.90805209522729));
#67571=CARTESIAN_POINT('Ctrl Pts',(-1.3778014851263,1.,-3.90029615196255));
#67572=CARTESIAN_POINT('Ctrl Pts',(-1.37849211287981,1.,-3.89254574338385));
#67573=CARTESIAN_POINT('Ctrl Pts',(-1.37914679719446,1.,-3.88480102249461));
#67574=CARTESIAN_POINT('Ctrl Pts',(-1.37976523097187,1.,-3.87706205830865));
#67575=CARTESIAN_POINT('Ctrl Pts',(-1.38034709213129,1.,-3.86932885813403));
#67576=CARTESIAN_POINT('Ctrl Pts',(-1.38089205993067,1.,-3.86160143044187));
#67577=CARTESIAN_POINT('Ctrl Pts',(-1.38139983115075,1.,-3.85387983979557));
#67578=CARTESIAN_POINT('Ctrl Pts',(-1.38187013346089,1.,-3.84616425605705));
#67579=CARTESIAN_POINT('Ctrl Pts',(-1.38230274828774,1.,-3.83845502790609));
#67580=CARTESIAN_POINT('Ctrl Pts',(-1.38269750245086,1.,-3.83075266982138));
#67581=CARTESIAN_POINT('Ctrl Pts',(-1.38305421262724,1.,-3.82305771743715));
#67582=CARTESIAN_POINT('Ctrl Pts',(-1.38337263902766,1.,-3.81537060817765));
#67583=CARTESIAN_POINT('Ctrl Pts',(-1.38365244046226,1.,-3.80769156398429));
#67584=CARTESIAN_POINT('Ctrl Pts',(-1.38389311766701,1.,-3.80002044322169));
#67585=CARTESIAN_POINT('Ctrl Pts',(-1.38409399694589,1.,-3.79235669640907));
#67586=CARTESIAN_POINT('Ctrl Pts',(-1.38425435883773,1.,-3.78469969805134));
#67587=CARTESIAN_POINT('Ctrl Pts',(-1.38437354551435,1.,-3.77704902230441));
#67588=CARTESIAN_POINT('Ctrl Pts',(-1.38445107339517,1.,-3.76940473185775));
#67589=CARTESIAN_POINT('Ctrl Pts',(-1.38448675253343,1.,-3.76176768271347));
#67590=CARTESIAN_POINT('Ctrl Pts',(-1.38448077997155,1.,-3.75413976318727));
#67591=CARTESIAN_POINT('Ctrl Pts',(-1.38443344984389,1.,-3.7465231716786));
#67592=CARTESIAN_POINT('Ctrl Pts',(-1.38434489156456,1.,-3.73891976418099));
#67593=CARTESIAN_POINT('Ctrl Pts',(-1.38421479111531,1.,-3.73133035859283));
#67594=CARTESIAN_POINT('Ctrl Pts',(-1.3840421342895,1.,-3.72375409358805));
#67595=CARTESIAN_POINT('Ctrl Pts',(-1.38382489984585,1.,-3.7161876605181));
#67596=CARTESIAN_POINT('Ctrl Pts',(-1.38356065402122,1.,-3.70862680753343));
#67597=CARTESIAN_POINT('Ctrl Pts',(-1.38324717612862,1.,-3.70106792167894));
#67598=CARTESIAN_POINT('Ctrl Pts',(-1.38288311171649,1.,-3.69350967899523));
#67599=CARTESIAN_POINT('Ctrl Pts',(-1.38246852827185,1.,-3.68595444983844));
#67600=CARTESIAN_POINT('Ctrl Pts',(-1.38200574290626,1.,-3.6784103848243));
#67601=CARTESIAN_POINT('Ctrl Pts',(-1.38149812653876,1.,-3.67088843112282));
#67602=CARTESIAN_POINT('Ctrl Pts',(-1.38094856333558,1.,-3.66339848520874));
#67603=CARTESIAN_POINT('Ctrl Pts',(-1.38035791051215,1.,-3.65594554404396));
#67604=CARTESIAN_POINT('Ctrl Pts',(-1.37972372481598,1.,-3.64852652756444));
#67605=CARTESIAN_POINT('Ctrl Pts',(-1.37903818567347,1.,-3.64112507791112));
#67606=CARTESIAN_POINT('Ctrl Pts',(-1.37829035457324,1.,-3.63371727442448));
#67607=CARTESIAN_POINT('Ctrl Pts',(-1.37746987919868,1.,-3.62628098665112));
#67608=CARTESIAN_POINT('Ctrl Pts',(-1.37657053403102,1.,-3.61880481160408));
#67609=CARTESIAN_POINT('Ctrl Pts',(-1.37559314436641,1.,-3.61129546591082));
#67610=CARTESIAN_POINT('Ctrl Pts',(-1.37455051379642,1.,-3.60379020124038));
#67611=CARTESIAN_POINT('Ctrl Pts',(-1.37346320103184,1.,-3.59634627869117));
#67612=CARTESIAN_POINT('Ctrl Pts',(-1.37235053661,1.,-3.5890185384643));
#67613=CARTESIAN_POINT('Ctrl Pts',(-1.37122241663073,1.,-3.58183885982745));
#67614=CARTESIAN_POINT('Ctrl Pts',(-1.37007229485646,1.,-3.57479875549453));
#67615=CARTESIAN_POINT('Ctrl Pts',(-1.36886584973349,1.,-3.56782080304554));
#67616=CARTESIAN_POINT('Ctrl Pts',(-1.36754771771174,1.,-3.56077662028492));
#67617=CARTESIAN_POINT('Ctrl Pts',(-1.36606145456711,1.,-3.55353883995793));
#67618=CARTESIAN_POINT('Ctrl Pts',(-1.36436666257567,1.,-3.54602591832893));
#67619=CARTESIAN_POINT('Ctrl Pts',(-1.36245507339334,1.,-3.53824396425032));
#67620=CARTESIAN_POINT('Ctrl Pts',(-1.36037259643827,1.,-3.53034464961849));
#67621=CARTESIAN_POINT('Ctrl Pts',(-1.35821701528975,1.,-3.52261776117121));
#67622=CARTESIAN_POINT('Ctrl Pts',(-1.35611275237288,1.,-3.51542230699919));
#67623=CARTESIAN_POINT('Ctrl Pts',(-1.35419113576022,1.,-3.50913227060177));
#67624=CARTESIAN_POINT('Ctrl Pts',(-1.3525703284343,1.,-3.50408168106113));
#67625=CARTESIAN_POINT('Ctrl Pts',(-1.35142377279535,1.,-3.5007660381658));
#67626=CARTESIAN_POINT('Ctrl Pts',(-1.35080045218652,1.,-3.49920025459856));
#67627=CARTESIAN_POINT('Ctrl Pts',(-1.35049736560633,1.,-3.49861894124915));
#67628=CARTESIAN_POINT('Ctrl Pts',(-1.35036670893102,1.,-3.49847119623841));
#67629=CARTESIAN_POINT('Ctrl Pts',(-1.35032489087269,1.,-3.49844575334386));
#67630=CARTESIAN_POINT('',(-1.36999806084572,0.,-3.97027773754922));
#67631=CARTESIAN_POINT('Ctrl Pts',(-0.96399761336957,-1.,-3.62397690409552));
#67632=CARTESIAN_POINT('Ctrl Pts',(-0.96399761336957,1.,-3.62397690409552));
#67633=CARTESIAN_POINT('Ctrl Pts',(-0.963922720982576,-1.,-3.62393257642191));
#67634=CARTESIAN_POINT('Ctrl Pts',(-0.963922720982576,1.,-3.62393257642191));
#67635=CARTESIAN_POINT('Ctrl Pts',(-0.963832486396055,-1.,-3.62399933640277));
#67636=CARTESIAN_POINT('Ctrl Pts',(-0.963832486396055,1.,-3.62399933640277));
#67637=CARTESIAN_POINT('Ctrl Pts',(-0.963875774532103,-1.,-3.62456568607055));
#67638=CARTESIAN_POINT('Ctrl Pts',(-0.963875774532103,1.,-3.62456568607055));
#67639=CARTESIAN_POINT('Ctrl Pts',(-0.964291001274618,-1.,-3.62625391255277));
#67640=CARTESIAN_POINT('Ctrl Pts',(-0.964291001274618,1.,-3.62625391255277));
#67641=CARTESIAN_POINT('Ctrl Pts',(-0.965395153165716,-1.,-3.62988252139998));
#67642=CARTESIAN_POINT('Ctrl Pts',(-0.965395153165716,1.,-3.62988252139998));
#67643=CARTESIAN_POINT('Ctrl Pts',(-0.967052554540877,-1.,-3.6349212208096));
#67644=CARTESIAN_POINT('Ctrl Pts',(-0.967052554540877,1.,-3.6349212208096));
#67645=CARTESIAN_POINT('Ctrl Pts',(-0.969195124674829,-1.,-3.64113946505393));
#67646=CARTESIAN_POINT('Ctrl Pts',(-0.969195124674829,1.,-3.64113946505393));
#67647=CARTESIAN_POINT('Ctrl Pts',(-0.971722122060277,-1.,-3.64819756447072));
#67648=CARTESIAN_POINT('Ctrl Pts',(-0.971722122060277,1.,-3.64819756447072));
#67649=CARTESIAN_POINT('Ctrl Pts',(-0.974519971354139,-1.,-3.6557157673487));
#67650=CARTESIAN_POINT('Ctrl Pts',(-0.974519971354139,1.,-3.6557157673487));
#67651=CARTESIAN_POINT('Ctrl Pts',(-0.977478312751416,-1.,-3.66333049637403));
#67652=CARTESIAN_POINT('Ctrl Pts',(-0.977478312751416,1.,-3.66333049637403));
#67653=CARTESIAN_POINT('Ctrl Pts',(-0.980505922458494,-1.,-3.67074983340444));
#67654=CARTESIAN_POINT('Ctrl Pts',(-0.980505922458494,1.,-3.67074983340444));
#67655=CARTESIAN_POINT('Ctrl Pts',(-0.983550791470864,-1.,-3.67782408841876));
#67656=CARTESIAN_POINT('Ctrl Pts',(-0.983550791470864,1.,-3.67782408841876));
#67657=CARTESIAN_POINT('Ctrl Pts',(-0.986602639864286,-1.,-3.6845531792623));
#67658=CARTESIAN_POINT('Ctrl Pts',(-0.986602639864286,1.,-3.6845531792623));
#67659=CARTESIAN_POINT('Ctrl Pts',(-0.989676715398858,-1.,-3.69102682138955));
#67660=CARTESIAN_POINT('Ctrl Pts',(-0.989676715398858,1.,-3.69102682138955));
#67661=CARTESIAN_POINT('Ctrl Pts',(-0.992802218332104,-1.,-3.69738123415696));
#67662=CARTESIAN_POINT('Ctrl Pts',(-0.992802218332104,1.,-3.69738123415696));
#67663=CARTESIAN_POINT('Ctrl Pts',(-0.996009819772432,-1.,-3.70375282282107));
#67664=CARTESIAN_POINT('Ctrl Pts',(-0.996009819772432,1.,-3.70375282282107));
#67665=CARTESIAN_POINT('Ctrl Pts',(-0.999317260756344,-1.,-3.7102243971387));
#67666=CARTESIAN_POINT('Ctrl Pts',(-0.999317260756344,1.,-3.7102243971387));
#67667=CARTESIAN_POINT('Ctrl Pts',(-1.00272423396802,-1.,-3.71680667125047));
#67668=CARTESIAN_POINT('Ctrl Pts',(-1.00272423396802,1.,-3.71680667125047));
#67669=CARTESIAN_POINT('Ctrl Pts',(-1.00622000735696,-1.,-3.72346803750544));
#67670=CARTESIAN_POINT('Ctrl Pts',(-1.00622000735696,1.,-3.72346803750544));
#67671=CARTESIAN_POINT('Ctrl Pts',(-1.00978798539491,-1.,-3.73015276704407));
#67672=CARTESIAN_POINT('Ctrl Pts',(-1.00978798539491,1.,-3.73015276704407));
#67673=CARTESIAN_POINT('Ctrl Pts',(-1.01341114319906,-1.,-3.73680245055747));
#67674=CARTESIAN_POINT('Ctrl Pts',(-1.01341114319906,1.,-3.73680245055747));
#67675=CARTESIAN_POINT('Ctrl Pts',(-1.01707794311088,-1.,-3.74337942504993));
#67676=CARTESIAN_POINT('Ctrl Pts',(-1.01707794311088,1.,-3.74337942504993));
#67677=CARTESIAN_POINT('Ctrl Pts',(-1.02078510487439,-1.,-3.74987777155873));
#67678=CARTESIAN_POINT('Ctrl Pts',(-1.02078510487439,1.,-3.74987777155873));
#67679=CARTESIAN_POINT('Ctrl Pts',(-1.02453429444668,-1.,-3.75631037456224));
#67680=CARTESIAN_POINT('Ctrl Pts',(-1.02453429444668,1.,-3.75631037456224));
#67681=CARTESIAN_POINT('Ctrl Pts',(-1.02833014458184,-1.,-3.76270122291245));
#67682=CARTESIAN_POINT('Ctrl Pts',(-1.02833014458184,1.,-3.76270122291245));
#67683=CARTESIAN_POINT('Ctrl Pts',(-1.03217786604919,-1.,-3.76907609832516));
#67684=CARTESIAN_POINT('Ctrl Pts',(-1.03217786604919,1.,-3.76907609832516));
#67685=CARTESIAN_POINT('Ctrl Pts',(-1.03608074678008,-1.,-3.77545283140427));
#67686=CARTESIAN_POINT('Ctrl Pts',(-1.03608074678008,1.,-3.77545283140427));
#67687=CARTESIAN_POINT('Ctrl Pts',(-1.04003862055798,-1.,-3.7818353500817));
#67688=CARTESIAN_POINT('Ctrl Pts',(-1.04003862055798,1.,-3.7818353500817));
#67689=CARTESIAN_POINT('Ctrl Pts',(-1.04404924374422,-1.,-3.78821910787179));
#67690=CARTESIAN_POINT('Ctrl Pts',(-1.04404924374422,1.,-3.78821910787179));
#67691=CARTESIAN_POINT('Ctrl Pts',(-1.04810913267639,-1.,-3.79459440308786));
#67692=CARTESIAN_POINT('Ctrl Pts',(-1.04810913267639,1.,-3.79459440308786));
#67693=CARTESIAN_POINT('Ctrl Pts',(-1.05221457990016,-1.,-3.80095039790681));
#67694=CARTESIAN_POINT('Ctrl Pts',(-1.05221457990016,1.,-3.80095039790681));
#67695=CARTESIAN_POINT('Ctrl Pts',(-1.05636266918644,-1.,-3.80727913637791));
#67696=CARTESIAN_POINT('Ctrl Pts',(-1.05636266918644,1.,-3.80727913637791));
#67697=CARTESIAN_POINT('Ctrl Pts',(-1.06055206187299,-1.,-3.8135786611749));
#67698=CARTESIAN_POINT('Ctrl Pts',(-1.06055206187299,1.,-3.8135786611749));
#67699=CARTESIAN_POINT('Ctrl Pts',(-1.0647824403893,-1.,-3.81985083953012));
#67700=CARTESIAN_POINT('Ctrl Pts',(-1.0647824403893,1.,-3.81985083953012));
#67701=CARTESIAN_POINT('Ctrl Pts',(-1.06905413180359,-1.,-3.82609989967276));
#67702=CARTESIAN_POINT('Ctrl Pts',(-1.06905413180359,1.,-3.82609989967276));
#67703=CARTESIAN_POINT('Ctrl Pts',(-1.07336766633459,-1.,-3.83233071195144));
#67704=CARTESIAN_POINT('Ctrl Pts',(-1.07336766633459,1.,-3.83233071195144));
#67705=CARTESIAN_POINT('Ctrl Pts',(-1.07772335353858,-1.,-3.83854714117491));
#67706=CARTESIAN_POINT('Ctrl Pts',(-1.07772335353858,1.,-3.83854714117491));
#67707=CARTESIAN_POINT('Ctrl Pts',(-1.08212087917991,-1.,-3.8447504803063));
#67708=CARTESIAN_POINT('Ctrl Pts',(-1.08212087917991,1.,-3.8447504803063));
#67709=CARTESIAN_POINT('Ctrl Pts',(-1.08655950846384,-1.,-3.85094025222713));
#67710=CARTESIAN_POINT('Ctrl Pts',(-1.08655950846384,1.,-3.85094025222713));
#67711=CARTESIAN_POINT('Ctrl Pts',(-1.09103825516294,-1.,-3.85711487933931));
#67712=CARTESIAN_POINT('Ctrl Pts',(-1.09103825516294,1.,-3.85711487933931));
#67713=CARTESIAN_POINT('Ctrl Pts',(-1.09555606505013,-1.,-3.86327241021247));
#67714=CARTESIAN_POINT('Ctrl Pts',(-1.09555606505013,1.,-3.86327241021247));
#67715=CARTESIAN_POINT('Ctrl Pts',(-1.10011198761195,-1.,-3.86941120134849));
#67716=CARTESIAN_POINT('Ctrl Pts',(-1.10011198761195,1.,-3.86941120134849));
#67717=CARTESIAN_POINT('Ctrl Pts',(-1.10470536603287,-1.,-3.87553067187514));
#67718=CARTESIAN_POINT('Ctrl Pts',(-1.10470536603287,1.,-3.87553067187514));
#67719=CARTESIAN_POINT('Ctrl Pts',(-1.10933577224008,-1.,-3.88163105531724));
#67720=CARTESIAN_POINT('Ctrl Pts',(-1.10933577224008,1.,-3.88163105531724));
#67721=CARTESIAN_POINT('Ctrl Pts',(-1.11400292434429,-1.,-3.88771308285171));
#67722=CARTESIAN_POINT('Ctrl Pts',(-1.11400292434429,1.,-3.88771308285171));
#67723=CARTESIAN_POINT('Ctrl Pts',(-1.11870660794603,-1.,-3.89377768340344));
#67724=CARTESIAN_POINT('Ctrl Pts',(-1.11870660794603,1.,-3.89377768340344));
#67725=CARTESIAN_POINT('Ctrl Pts',(-1.12344660099043,-1.,-3.89982569750025));
#67726=CARTESIAN_POINT('Ctrl Pts',(-1.12344660099043,1.,-3.89982569750025));
#67727=CARTESIAN_POINT('Ctrl Pts',(-1.12822258281553,-1.,-3.90585753318737));
#67728=CARTESIAN_POINT('Ctrl Pts',(-1.12822258281553,1.,-3.90585753318737));
#67729=CARTESIAN_POINT('Ctrl Pts',(-1.13303414693896,-1.,-3.91187321145649));
#67730=CARTESIAN_POINT('Ctrl Pts',(-1.13303414693896,1.,-3.91187321145649));
#67731=CARTESIAN_POINT('Ctrl Pts',(-1.13788084225554,-1.,-3.91787251936827));
#67732=CARTESIAN_POINT('Ctrl Pts',(-1.13788084225554,1.,-3.91787251936827));
#67733=CARTESIAN_POINT('Ctrl Pts',(-1.14276220561593,-1.,-3.92385513133997));
#67734=CARTESIAN_POINT('Ctrl Pts',(-1.14276220561593,1.,-3.92385513133997));
#67735=CARTESIAN_POINT('Ctrl Pts',(-1.14767779451123,-1.,-3.92982073294257));
#67736=CARTESIAN_POINT('Ctrl Pts',(-1.14767779451123,1.,-3.92982073294257));
#67737=CARTESIAN_POINT('Ctrl Pts',(-1.1526272271632,-1.,-3.9357691705628));
#67738=CARTESIAN_POINT('Ctrl Pts',(-1.1526272271632,1.,-3.9357691705628));
#67739=CARTESIAN_POINT('Ctrl Pts',(-1.15761018340956,-1.,-3.94170046685203));
#67740=CARTESIAN_POINT('Ctrl Pts',(-1.15761018340956,1.,-3.94170046685203));
#67741=CARTESIAN_POINT('Ctrl Pts',(-1.16262637999157,-1.,-3.94761474780583));
#67742=CARTESIAN_POINT('Ctrl Pts',(-1.16262637999157,1.,-3.94761474780583));
#67743=CARTESIAN_POINT('Ctrl Pts',(-1.16767555244438,-1.,-3.95351219509876));
#67744=CARTESIAN_POINT('Ctrl Pts',(-1.16767555244438,1.,-3.95351219509876));
#67745=CARTESIAN_POINT('Ctrl Pts',(-1.17275743590361,-1.,-3.95939299213276));
#67746=CARTESIAN_POINT('Ctrl Pts',(-1.17275743590361,1.,-3.95939299213276));
#67747=CARTESIAN_POINT('Ctrl Pts',(-1.17787174135592,-1.,-3.96525726358159));
#67748=CARTESIAN_POINT('Ctrl Pts',(-1.17787174135592,1.,-3.96525726358159));
#67749=CARTESIAN_POINT('Ctrl Pts',(-1.18301815039831,-1.,-3.97110505165415));
#67750=CARTESIAN_POINT('Ctrl Pts',(-1.18301815039831,1.,-3.97110505165415));
#67751=CARTESIAN_POINT('Ctrl Pts',(-1.18819633715539,-1.,-3.97693634767754));
#67752=CARTESIAN_POINT('Ctrl Pts',(-1.18819633715539,1.,-3.97693634767754));
#67753=CARTESIAN_POINT('Ctrl Pts',(-1.19340598349475,-1.,-3.98275111052561));
#67754=CARTESIAN_POINT('Ctrl Pts',(-1.19340598349475,1.,-3.98275111052561));
#67755=CARTESIAN_POINT('Ctrl Pts',(-1.19864679609566,-1.,-3.98854928957189));
#67756=CARTESIAN_POINT('Ctrl Pts',(-1.19864679609566,1.,-3.98854928957189));
#67757=CARTESIAN_POINT('Ctrl Pts',(-1.20391852375139,-1.,-3.99433084799666));
#67758=CARTESIAN_POINT('Ctrl Pts',(-1.20391852375139,1.,-3.99433084799666));
#67759=CARTESIAN_POINT('Ctrl Pts',(-1.20922097029551,-1.,-4.00009577950721));
#67760=CARTESIAN_POINT('Ctrl Pts',(-1.20922097029551,1.,-4.00009577950721));
#67761=CARTESIAN_POINT('Ctrl Pts',(-1.21455398918133,-1.,-4.00584409522722));
#67762=CARTESIAN_POINT('Ctrl Pts',(-1.21455398918133,1.,-4.00584409522722));
#67763=CARTESIAN_POINT('Ctrl Pts',(-1.21884478244403,-1.,-4.01042947140789));
#67764=CARTESIAN_POINT('Ctrl Pts',(-1.21884478244403,1.,-4.01042947140789));
#67765=CARTESIAN_POINT('Ctrl Pts',(-1.22207656455845,-1.,-4.01386104433519));
#67766=CARTESIAN_POINT('Ctrl Pts',(-1.22207656455845,1.,-4.01386104433519));
#67767=CARTESIAN_POINT('Ctrl Pts',(-1.22423716681317,-1.,-4.01614544569895));
#67768=CARTESIAN_POINT('Ctrl Pts',(-1.22423716681317,1.,-4.01614544569895));
#67769=CARTESIAN_POINT('Ctrl Pts',(-1.22531898815164,-1.,-4.01728681790024));
#67770=CARTESIAN_POINT('Ctrl Pts',(-1.22531898815164,1.,-4.01728681790024));
#67771=CARTESIAN_POINT('',(-0.963899035118984,1.,-3.62400312501199));
#67772=CARTESIAN_POINT('Ctrl Pts',(-0.963899035118985,-1.,-3.62400312501199));
#67773=CARTESIAN_POINT('Ctrl Pts',(-0.963899035118985,-0.666666666666667,
-3.62400312501199));
#67774=CARTESIAN_POINT('Ctrl Pts',(-0.963899035118985,-0.333333333333333,
-3.62400312501199));
#67775=CARTESIAN_POINT('Ctrl Pts',(-0.963899035118985,0.333333333333333,
-3.62400312501199));
#67776=CARTESIAN_POINT('Ctrl Pts',(-0.963899035118986,0.666666666666667,
-3.62400312501199));
#67777=CARTESIAN_POINT('Ctrl Pts',(-0.963899035118986,1.,-3.62400312501199));
#67778=CARTESIAN_POINT('',(-1.22531898815164,1.,-4.01728681790024));
#67779=CARTESIAN_POINT('',(-1.22531898815164,0.,-4.01728681790024));
#67780=CARTESIAN_POINT('Ctrl Pts',(-0.963899035118985,1.,-3.62400312501199));
#67781=CARTESIAN_POINT('Ctrl Pts',(-0.963880158556713,1.,-3.62404828878375));
#67782=CARTESIAN_POINT('Ctrl Pts',(-0.963861297423579,1.,-3.62424461507455));
#67783=CARTESIAN_POINT('Ctrl Pts',(-0.963957782642589,1.,-3.62489305727516));
#67784=CARTESIAN_POINT('Ctrl Pts',(-0.964373850166081,1.,-3.62652618145252));
#67785=CARTESIAN_POINT('Ctrl Pts',(-0.965395153165716,1.,-3.62988252139998));
#67786=CARTESIAN_POINT('Ctrl Pts',(-0.967052554540877,1.,-3.6349212208096));
#67787=CARTESIAN_POINT('Ctrl Pts',(-0.969195124674829,1.,-3.64113946505393));
#67788=CARTESIAN_POINT('Ctrl Pts',(-0.971722122060277,1.,-3.64819756447072));
#67789=CARTESIAN_POINT('Ctrl Pts',(-0.974519971354139,1.,-3.6557157673487));
#67790=CARTESIAN_POINT('Ctrl Pts',(-0.977478312751416,1.,-3.66333049637403));
#67791=CARTESIAN_POINT('Ctrl Pts',(-0.980505922458494,1.,-3.67074983340444));
#67792=CARTESIAN_POINT('Ctrl Pts',(-0.983550791470864,1.,-3.67782408841876));
#67793=CARTESIAN_POINT('Ctrl Pts',(-0.986602639864286,1.,-3.6845531792623));
#67794=CARTESIAN_POINT('Ctrl Pts',(-0.989676715398858,1.,-3.69102682138955));
#67795=CARTESIAN_POINT('Ctrl Pts',(-0.992802218332104,1.,-3.69738123415696));
#67796=CARTESIAN_POINT('Ctrl Pts',(-0.996009819772432,1.,-3.70375282282107));
#67797=CARTESIAN_POINT('Ctrl Pts',(-0.999317260756344,1.,-3.7102243971387));
#67798=CARTESIAN_POINT('Ctrl Pts',(-1.00272423396802,1.,-3.71680667125047));
#67799=CARTESIAN_POINT('Ctrl Pts',(-1.00622000735696,1.,-3.72346803750544));
#67800=CARTESIAN_POINT('Ctrl Pts',(-1.00978798539491,1.,-3.73015276704407));
#67801=CARTESIAN_POINT('Ctrl Pts',(-1.01341114319906,1.,-3.73680245055747));
#67802=CARTESIAN_POINT('Ctrl Pts',(-1.01707794311088,1.,-3.74337942504993));
#67803=CARTESIAN_POINT('Ctrl Pts',(-1.02078510487439,1.,-3.74987777155873));
#67804=CARTESIAN_POINT('Ctrl Pts',(-1.02453429444668,1.,-3.75631037456224));
#67805=CARTESIAN_POINT('Ctrl Pts',(-1.02833014458184,1.,-3.76270122291245));
#67806=CARTESIAN_POINT('Ctrl Pts',(-1.03217786604919,1.,-3.76907609832516));
#67807=CARTESIAN_POINT('Ctrl Pts',(-1.03608074678008,1.,-3.77545283140427));
#67808=CARTESIAN_POINT('Ctrl Pts',(-1.04003862055798,1.,-3.7818353500817));
#67809=CARTESIAN_POINT('Ctrl Pts',(-1.04404924374422,1.,-3.78821910787179));
#67810=CARTESIAN_POINT('Ctrl Pts',(-1.04810913267639,1.,-3.79459440308786));
#67811=CARTESIAN_POINT('Ctrl Pts',(-1.05221457990016,1.,-3.80095039790681));
#67812=CARTESIAN_POINT('Ctrl Pts',(-1.05636266918644,1.,-3.80727913637791));
#67813=CARTESIAN_POINT('Ctrl Pts',(-1.06055206187299,1.,-3.8135786611749));
#67814=CARTESIAN_POINT('Ctrl Pts',(-1.0647824403893,1.,-3.81985083953012));
#67815=CARTESIAN_POINT('Ctrl Pts',(-1.06905413180359,1.,-3.82609989967276));
#67816=CARTESIAN_POINT('Ctrl Pts',(-1.07336766633459,1.,-3.83233071195144));
#67817=CARTESIAN_POINT('Ctrl Pts',(-1.07772335353858,1.,-3.83854714117491));
#67818=CARTESIAN_POINT('Ctrl Pts',(-1.08212087917991,1.,-3.8447504803063));
#67819=CARTESIAN_POINT('Ctrl Pts',(-1.08655950846384,1.,-3.85094025222713));
#67820=CARTESIAN_POINT('Ctrl Pts',(-1.09103825516294,1.,-3.85711487933931));
#67821=CARTESIAN_POINT('Ctrl Pts',(-1.09555606505013,1.,-3.86327241021247));
#67822=CARTESIAN_POINT('Ctrl Pts',(-1.10011198761195,1.,-3.86941120134849));
#67823=CARTESIAN_POINT('Ctrl Pts',(-1.10470536603287,1.,-3.87553067187514));
#67824=CARTESIAN_POINT('Ctrl Pts',(-1.10933577224008,1.,-3.88163105531724));
#67825=CARTESIAN_POINT('Ctrl Pts',(-1.11400292434429,1.,-3.88771308285171));
#67826=CARTESIAN_POINT('Ctrl Pts',(-1.11870660794603,1.,-3.89377768340344));
#67827=CARTESIAN_POINT('Ctrl Pts',(-1.12344660099043,1.,-3.89982569750025));
#67828=CARTESIAN_POINT('Ctrl Pts',(-1.12822258281553,1.,-3.90585753318737));
#67829=CARTESIAN_POINT('Ctrl Pts',(-1.13303414693896,1.,-3.91187321145649));
#67830=CARTESIAN_POINT('Ctrl Pts',(-1.13788084225554,1.,-3.91787251936827));
#67831=CARTESIAN_POINT('Ctrl Pts',(-1.14276220561593,1.,-3.92385513133997));
#67832=CARTESIAN_POINT('Ctrl Pts',(-1.14767779451123,1.,-3.92982073294257));
#67833=CARTESIAN_POINT('Ctrl Pts',(-1.1526272271632,1.,-3.9357691705628));
#67834=CARTESIAN_POINT('Ctrl Pts',(-1.15761018340956,1.,-3.94170046685203));
#67835=CARTESIAN_POINT('Ctrl Pts',(-1.16262637999157,1.,-3.94761474780583));
#67836=CARTESIAN_POINT('Ctrl Pts',(-1.16767555244438,1.,-3.95351219509876));
#67837=CARTESIAN_POINT('Ctrl Pts',(-1.17275743590361,1.,-3.95939299213276));
#67838=CARTESIAN_POINT('Ctrl Pts',(-1.17787174135592,1.,-3.96525726358159));
#67839=CARTESIAN_POINT('Ctrl Pts',(-1.18301815039831,1.,-3.97110505165415));
#67840=CARTESIAN_POINT('Ctrl Pts',(-1.18819633715539,1.,-3.97693634767754));
#67841=CARTESIAN_POINT('Ctrl Pts',(-1.19340598349475,1.,-3.98275111052561));
#67842=CARTESIAN_POINT('Ctrl Pts',(-1.19864679609566,1.,-3.98854928957189));
#67843=CARTESIAN_POINT('Ctrl Pts',(-1.20391852375139,1.,-3.99433084799666));
#67844=CARTESIAN_POINT('Ctrl Pts',(-1.20922097029551,1.,-4.00009577950721));
#67845=CARTESIAN_POINT('Ctrl Pts',(-1.21455398918133,1.,-4.00584409522722));
#67846=CARTESIAN_POINT('Ctrl Pts',(-1.21884478244403,1.,-4.01042947140789));
#67847=CARTESIAN_POINT('Ctrl Pts',(-1.22207656455845,1.,-4.01386104433519));
#67848=CARTESIAN_POINT('Ctrl Pts',(-1.22423716681317,1.,-4.01614544569895));
#67849=CARTESIAN_POINT('Ctrl Pts',(-1.22531898815164,1.,-4.01728681790024));
#67850=CARTESIAN_POINT('Origin',(-1.22531898815164,0.,-4.01728681790024));
#67851=CARTESIAN_POINT('',(-1.36999806084572,1.,-3.97027773754922));
#67852=CARTESIAN_POINT('Origin',(0.,0.,0.));
#67853=CARTESIAN_POINT('',(-0.786422660833743,1.,-3.66661143271648));
#67854=CARTESIAN_POINT('Origin',(0.,1.,0.));
#67855=CARTESIAN_POINT('Ctrl Pts',(-0.786422660833742,1.,-3.66661143271648));
#67856=CARTESIAN_POINT('Ctrl Pts',(-0.786422660833742,0.666666666666667,
-3.66661143271648));
#67857=CARTESIAN_POINT('Ctrl Pts',(-0.786422660833742,0.333333333333333,
-3.66661143271648));
#67858=CARTESIAN_POINT('Ctrl Pts',(-0.786422660833742,-0.333333333333333,
-3.66661143271648));
#67859=CARTESIAN_POINT('Ctrl Pts',(-0.786422660833742,-0.666666666666667,
-3.66661143271648));
#67860=CARTESIAN_POINT('Ctrl Pts',(-0.786422660833742,-1.,-3.66661143271648));
#67861=CARTESIAN_POINT('Ctrl Pts',(-0.732042837400619,-1.,-4.13571194405636));
#67862=CARTESIAN_POINT('Ctrl Pts',(-0.732042837400619,1.,-4.13571194405636));
#67863=CARTESIAN_POINT('Ctrl Pts',(-0.732488575135926,-1.,-4.13420383737278));
#67864=CARTESIAN_POINT('Ctrl Pts',(-0.732488575135926,1.,-4.13420383737278));
#67865=CARTESIAN_POINT('Ctrl Pts',(-0.733376589325634,-1.,-4.13118752796397));
#67866=CARTESIAN_POINT('Ctrl Pts',(-0.733376589325634,1.,-4.13118752796397));
#67867=CARTESIAN_POINT('Ctrl Pts',(-0.734698226767512,-1.,-4.12666277572794));
#67868=CARTESIAN_POINT('Ctrl Pts',(-0.734698226767512,1.,-4.12666277572794));
#67869=CARTESIAN_POINT('Ctrl Pts',(-0.736439634335347,-1.,-4.12062919626082));
#67870=CARTESIAN_POINT('Ctrl Pts',(-0.736439634335347,1.,-4.12062919626082));
#67871=CARTESIAN_POINT('Ctrl Pts',(-0.738581708229119,-1.,-4.11308626953795));
#67872=CARTESIAN_POINT('Ctrl Pts',(-0.738581708229119,1.,-4.11308626953795));
#67873=CARTESIAN_POINT('Ctrl Pts',(-0.740688998555152,-1.,-4.1055424175856));
#67874=CARTESIAN_POINT('Ctrl Pts',(-0.740688998555152,1.,-4.1055424175856));
#67875=CARTESIAN_POINT('Ctrl Pts',(-0.742761369690018,-1.,-4.09799769702712));
#67876=CARTESIAN_POINT('Ctrl Pts',(-0.742761369690018,1.,-4.09799769702712));
#67877=CARTESIAN_POINT('Ctrl Pts',(-0.744798649705514,-1.,-4.09045220253011));
#67878=CARTESIAN_POINT('Ctrl Pts',(-0.744798649705514,1.,-4.09045220253011));
#67879=CARTESIAN_POINT('Ctrl Pts',(-0.746800631490822,-1.,-4.08290608094789));
#67880=CARTESIAN_POINT('Ctrl Pts',(-0.746800631490822,1.,-4.08290608094789));
#67881=CARTESIAN_POINT('Ctrl Pts',(-0.748767076679177,-1.,-4.07535951055363));
#67882=CARTESIAN_POINT('Ctrl Pts',(-0.748767076679177,1.,-4.07535951055363));
#67883=CARTESIAN_POINT('Ctrl Pts',(-0.750697720483176,-1.,-4.06781267241886));
#67884=CARTESIAN_POINT('Ctrl Pts',(-0.750697720483176,1.,-4.06781267241886));
#67885=CARTESIAN_POINT('Ctrl Pts',(-0.752592276482869,-1.,-4.06026572221399));
#67886=CARTESIAN_POINT('Ctrl Pts',(-0.752592276482869,1.,-4.06026572221399));
#67887=CARTESIAN_POINT('Ctrl Pts',(-0.754450441816412,-1.,-4.05271876688106));
#67888=CARTESIAN_POINT('Ctrl Pts',(-0.754450441816412,1.,-4.05271876688106));
#67889=CARTESIAN_POINT('Ctrl Pts',(-0.756271902370187,-1.,-4.04517182654344));
#67890=CARTESIAN_POINT('Ctrl Pts',(-0.756271902370187,1.,-4.04517182654344));
#67891=CARTESIAN_POINT('Ctrl Pts',(-0.758056338885554,-1.,-4.03762485803468));
#67892=CARTESIAN_POINT('Ctrl Pts',(-0.758056338885554,1.,-4.03762485803468));
#67893=CARTESIAN_POINT('Ctrl Pts',(-0.759803433244166,-1.,-4.0300778195465));
#67894=CARTESIAN_POINT('Ctrl Pts',(-0.759803433244166,1.,-4.0300778195465));
#67895=CARTESIAN_POINT('Ctrl Pts',(-0.761512875859942,-1.,-4.02253072741347));
#67896=CARTESIAN_POINT('Ctrl Pts',(-0.761512875859942,1.,-4.02253072741347));
#67897=CARTESIAN_POINT('Ctrl Pts',(-0.763184371182827,-1.,-4.01498370680434));
#67898=CARTESIAN_POINT('Ctrl Pts',(-0.763184371182827,1.,-4.01498370680434));
#67899=CARTESIAN_POINT('Ctrl Pts',(-0.764817648784946,-1.,-4.00743706791366));
#67900=CARTESIAN_POINT('Ctrl Pts',(-0.764817648784946,1.,-4.00743706791366));
#67901=CARTESIAN_POINT('Ctrl Pts',(-0.766412457135786,-1.,-3.99989129179464));
#67902=CARTESIAN_POINT('Ctrl Pts',(-0.766412457135786,1.,-3.99989129179464));
#67903=CARTESIAN_POINT('Ctrl Pts',(-0.767968531377708,-1.,-3.99234687880892));
#67904=CARTESIAN_POINT('Ctrl Pts',(-0.767968531377708,1.,-3.99234687880892));
#67905=CARTESIAN_POINT('Ctrl Pts',(-0.769485566245459,-1.,-3.98480422348403));
#67906=CARTESIAN_POINT('Ctrl Pts',(-0.769485566245459,1.,-3.98480422348403));
#67907=CARTESIAN_POINT('Ctrl Pts',(-0.770963190030504,-1.,-3.97726349165507));
#67908=CARTESIAN_POINT('Ctrl Pts',(-0.770963190030504,1.,-3.97726349165507));
#67909=CARTESIAN_POINT('Ctrl Pts',(-0.772400931772239,-1.,-3.96972446532832));
#67910=CARTESIAN_POINT('Ctrl Pts',(-0.772400931772239,1.,-3.96972446532832));
#67911=CARTESIAN_POINT('Ctrl Pts',(-0.773798212026683,-1.,-3.96218649639876));
#67912=CARTESIAN_POINT('Ctrl Pts',(-0.773798212026683,1.,-3.96218649639876));
#67913=CARTESIAN_POINT('Ctrl Pts',(-0.775154418039441,-1.,-3.95464885452364));
#67914=CARTESIAN_POINT('Ctrl Pts',(-0.775154418039441,1.,-3.95464885452364));
#67915=CARTESIAN_POINT('Ctrl Pts',(-0.77646896669796,-1.,-3.94711101619471));
#67916=CARTESIAN_POINT('Ctrl Pts',(-0.77646896669796,1.,-3.94711101619471));
#67917=CARTESIAN_POINT('Ctrl Pts',(-0.77774137056855,-1.,-3.93957296768098));
#67918=CARTESIAN_POINT('Ctrl Pts',(-0.77774137056855,1.,-3.93957296768098));
#67919=CARTESIAN_POINT('Ctrl Pts',(-0.778971308134786,-1.,-3.93203552473153));
#67920=CARTESIAN_POINT('Ctrl Pts',(-0.778971308134786,1.,-3.93203552473153));
#67921=CARTESIAN_POINT('Ctrl Pts',(-0.780158678615507,-1.,-3.92450058323799));
#67922=CARTESIAN_POINT('Ctrl Pts',(-0.780158678615507,1.,-3.92450058323799));
#67923=CARTESIAN_POINT('Ctrl Pts',(-0.781303428618344,-1.,-3.9169703605466));
#67924=CARTESIAN_POINT('Ctrl Pts',(-0.781303428618344,1.,-3.9169703605466));
#67925=CARTESIAN_POINT('Ctrl Pts',(-0.782405395622759,-1.,-3.90944671004536));
#67926=CARTESIAN_POINT('Ctrl Pts',(-0.782405395622759,1.,-3.90944671004536));
#67927=CARTESIAN_POINT('Ctrl Pts',(-0.783464141529082,-1.,-3.90193039043971));
#67928=CARTESIAN_POINT('Ctrl Pts',(-0.783464141529082,1.,-3.90193039043971));
#67929=CARTESIAN_POINT('Ctrl Pts',(-0.784478799358336,-1.,-3.89442039235105));
#67930=CARTESIAN_POINT('Ctrl Pts',(-0.784478799358336,1.,-3.89442039235105));
#67931=CARTESIAN_POINT('Ctrl Pts',(-0.785447890340723,-1.,-3.88691313167399));
#67932=CARTESIAN_POINT('Ctrl Pts',(-0.785447890340723,1.,-3.88691313167399));
#67933=CARTESIAN_POINT('Ctrl Pts',(-0.786369675812592,-1.,-3.87940402818186));
#67934=CARTESIAN_POINT('Ctrl Pts',(-0.786369675812592,1.,-3.87940402818186));
#67935=CARTESIAN_POINT('Ctrl Pts',(-0.78724252761798,-1.,-3.87188916600905));
#67936=CARTESIAN_POINT('Ctrl Pts',(-0.78724252761798,1.,-3.87188916600905));
#67937=CARTESIAN_POINT('Ctrl Pts',(-0.788065315093771,-1.,-3.86436702561342));
#67938=CARTESIAN_POINT('Ctrl Pts',(-0.788065315093771,1.,-3.86436702561342));
#67939=CARTESIAN_POINT('Ctrl Pts',(-0.788837734090688,-1.,-3.85683995872536));
#67940=CARTESIAN_POINT('Ctrl Pts',(-0.788837734090688,1.,-3.85683995872536));
#67941=CARTESIAN_POINT('Ctrl Pts',(-0.789560798155619,-1.,-3.8493163780891));
#67942=CARTESIAN_POINT('Ctrl Pts',(-0.789560798155619,1.,-3.8493163780891));
#67943=CARTESIAN_POINT('Ctrl Pts',(-0.790236124191289,-1.,-3.84180762342476));
#67944=CARTESIAN_POINT('Ctrl Pts',(-0.790236124191289,1.,-3.84180762342476));
#67945=CARTESIAN_POINT('Ctrl Pts',(-0.79086501270534,-1.,-3.83432392054804));
#67946=CARTESIAN_POINT('Ctrl Pts',(-0.79086501270534,1.,-3.83432392054804));
#67947=CARTESIAN_POINT('Ctrl Pts',(-0.791447528662381,-1.,-3.82687033899799));
#67948=CARTESIAN_POINT('Ctrl Pts',(-0.791447528662381,1.,-3.82687033899799));
#67949=CARTESIAN_POINT('Ctrl Pts',(-0.791981740718606,-1.,-3.81944345442237));
#67950=CARTESIAN_POINT('Ctrl Pts',(-0.791981740718606,1.,-3.81944345442237));
#67951=CARTESIAN_POINT('Ctrl Pts',(-0.792462483517568,-1.,-3.81202588694726));
#67952=CARTESIAN_POINT('Ctrl Pts',(-0.792462483517568,1.,-3.81202588694726));
#67953=CARTESIAN_POINT('Ctrl Pts',(-0.792882695234693,-1.,-3.80459229925598));
#67954=CARTESIAN_POINT('Ctrl Pts',(-0.792882695234693,1.,-3.80459229925598));
#67955=CARTESIAN_POINT('Ctrl Pts',(-0.7932356129732,-1.,-3.79711921389862));
#67956=CARTESIAN_POINT('Ctrl Pts',(-0.7932356129732,1.,-3.79711921389862));
#67957=CARTESIAN_POINT('Ctrl Pts',(-0.793516871680966,-1.,-3.78959439439222));
#67958=CARTESIAN_POINT('Ctrl Pts',(-0.793516871680966,1.,-3.78959439439222));
#67959=CARTESIAN_POINT('Ctrl Pts',(-0.793726235781339,-1.,-3.78202460377617));
#67960=CARTESIAN_POINT('Ctrl Pts',(-0.793726235781339,1.,-3.78202460377617));
#67961=CARTESIAN_POINT('Ctrl Pts',(-0.793870523787515,-1.,-3.77444863801264));
#67962=CARTESIAN_POINT('Ctrl Pts',(-0.793870523787515,1.,-3.77444863801264));
#67963=CARTESIAN_POINT('Ctrl Pts',(-0.793961083689141,-1.,-3.76692626931184));
#67964=CARTESIAN_POINT('Ctrl Pts',(-0.793961083689141,1.,-3.76692626931184));
#67965=CARTESIAN_POINT('Ctrl Pts',(-0.794008429135047,-1.,-3.75951468666325));
#67966=CARTESIAN_POINT('Ctrl Pts',(-0.794008429135047,1.,-3.75951468666325));
#67967=CARTESIAN_POINT('Ctrl Pts',(-0.794017347371441,-1.,-3.75224692493895));
#67968=CARTESIAN_POINT('Ctrl Pts',(-0.794017347371441,1.,-3.75224692493895));
#67969=CARTESIAN_POINT('Ctrl Pts',(-0.79398270045988,-1.,-3.74511357728827));
#67970=CARTESIAN_POINT('Ctrl Pts',(-0.79398270045988,1.,-3.74511357728827));
#67971=CARTESIAN_POINT('Ctrl Pts',(-0.79388270093679,-1.,-3.73803280541576));
#67972=CARTESIAN_POINT('Ctrl Pts',(-0.79388270093679,1.,-3.73803280541576));
#67973=CARTESIAN_POINT('Ctrl Pts',(-0.793682750269347,-1.,-3.7308691469564));
#67974=CARTESIAN_POINT('Ctrl Pts',(-0.793682750269347,1.,-3.7308691469564));
#67975=CARTESIAN_POINT('Ctrl Pts',(-0.79334702378387,-1.,-3.7234879729357));
#67976=CARTESIAN_POINT('Ctrl Pts',(-0.79334702378387,1.,-3.7234879729357));
#67977=CARTESIAN_POINT('Ctrl Pts',(-0.792848377370115,-1.,-3.7158024239604));
#67978=CARTESIAN_POINT('Ctrl Pts',(-0.792848377370115,1.,-3.7158024239604));
#67979=CARTESIAN_POINT('Ctrl Pts',(-0.792177688845968,-1.,-3.70781724021879));
#67980=CARTESIAN_POINT('Ctrl Pts',(-0.792177688845968,1.,-3.70781724021879));
#67981=CARTESIAN_POINT('Ctrl Pts',(-0.791356575696509,-1.,-3.69968940808982));
#67982=CARTESIAN_POINT('Ctrl Pts',(-0.791356575696509,1.,-3.69968940808982));
#67983=CARTESIAN_POINT('Ctrl Pts',(-0.79043628498958,-1.,-3.69172044327754));
#67984=CARTESIAN_POINT('Ctrl Pts',(-0.79043628498958,1.,-3.69172044327754));
#67985=CARTESIAN_POINT('Ctrl Pts',(-0.789483546065158,-1.,-3.68428439784285));
#67986=CARTESIAN_POINT('Ctrl Pts',(-0.789483546065158,1.,-3.68428439784285));
#67987=CARTESIAN_POINT('Ctrl Pts',(-0.788569566220662,-1.,-3.67777119516438));
#67988=CARTESIAN_POINT('Ctrl Pts',(-0.788569566220662,1.,-3.67777119516438));
#67989=CARTESIAN_POINT('Ctrl Pts',(-0.787758799995426,-1.,-3.672529236635));
#67990=CARTESIAN_POINT('Ctrl Pts',(-0.787758799995426,1.,-3.672529236635));
#67991=CARTESIAN_POINT('Ctrl Pts',(-0.787095252589508,-1.,-3.66879484800625));
#67992=CARTESIAN_POINT('Ctrl Pts',(-0.787095252589508,1.,-3.66879484800625));
#67993=CARTESIAN_POINT('Ctrl Pts',(-0.786698783541658,-1.,-3.66710211819938));
#67994=CARTESIAN_POINT('Ctrl Pts',(-0.786698783541658,1.,-3.66710211819938));
#67995=CARTESIAN_POINT('Ctrl Pts',(-0.786480236184947,-1.,-3.66657784454965));
#67996=CARTESIAN_POINT('Ctrl Pts',(-0.786480236184947,1.,-3.66657784454965));
#67997=CARTESIAN_POINT('Ctrl Pts',(-0.786369528183039,-1.,-3.66655932661846));
#67998=CARTESIAN_POINT('Ctrl Pts',(-0.786369528183039,1.,-3.66655932661846));
#67999=CARTESIAN_POINT('Ctrl Pts',(-0.786322922920599,-1.,-3.66663282329846));
#68000=CARTESIAN_POINT('Ctrl Pts',(-0.786322922920599,1.,-3.66663282329846));
#68001=CARTESIAN_POINT('',(-0.732042837400619,1.,-4.13571194405636));
#68002=CARTESIAN_POINT('Ctrl Pts',(-0.732042837400619,1.,-4.13571194405636));
#68003=CARTESIAN_POINT('Ctrl Pts',(-0.732488575135926,1.,-4.13420383737278));
#68004=CARTESIAN_POINT('Ctrl Pts',(-0.733376589325634,1.,-4.13118752796397));
#68005=CARTESIAN_POINT('Ctrl Pts',(-0.734698226767512,1.,-4.12666277572794));
#68006=CARTESIAN_POINT('Ctrl Pts',(-0.736439634335347,1.,-4.12062919626082));
#68007=CARTESIAN_POINT('Ctrl Pts',(-0.738581708229119,1.,-4.11308626953795));
#68008=CARTESIAN_POINT('Ctrl Pts',(-0.740688998555152,1.,-4.1055424175856));
#68009=CARTESIAN_POINT('Ctrl Pts',(-0.742761369690018,1.,-4.09799769702712));
#68010=CARTESIAN_POINT('Ctrl Pts',(-0.744798649705514,1.,-4.09045220253011));
#68011=CARTESIAN_POINT('Ctrl Pts',(-0.746800631490822,1.,-4.08290608094789));
#68012=CARTESIAN_POINT('Ctrl Pts',(-0.748767076679177,1.,-4.07535951055363));
#68013=CARTESIAN_POINT('Ctrl Pts',(-0.750697720483176,1.,-4.06781267241886));
#68014=CARTESIAN_POINT('Ctrl Pts',(-0.752592276482869,1.,-4.06026572221399));
#68015=CARTESIAN_POINT('Ctrl Pts',(-0.754450441816412,1.,-4.05271876688106));
#68016=CARTESIAN_POINT('Ctrl Pts',(-0.756271902370187,1.,-4.04517182654344));
#68017=CARTESIAN_POINT('Ctrl Pts',(-0.758056338885554,1.,-4.03762485803468));
#68018=CARTESIAN_POINT('Ctrl Pts',(-0.759803433244166,1.,-4.0300778195465));
#68019=CARTESIAN_POINT('Ctrl Pts',(-0.761512875859942,1.,-4.02253072741347));
#68020=CARTESIAN_POINT('Ctrl Pts',(-0.763184371182827,1.,-4.01498370680434));
#68021=CARTESIAN_POINT('Ctrl Pts',(-0.764817648784946,1.,-4.00743706791366));
#68022=CARTESIAN_POINT('Ctrl Pts',(-0.766412457135786,1.,-3.99989129179464));
#68023=CARTESIAN_POINT('Ctrl Pts',(-0.767968531377708,1.,-3.99234687880892));
#68024=CARTESIAN_POINT('Ctrl Pts',(-0.769485566245459,1.,-3.98480422348403));
#68025=CARTESIAN_POINT('Ctrl Pts',(-0.770963190030504,1.,-3.97726349165507));
#68026=CARTESIAN_POINT('Ctrl Pts',(-0.772400931772239,1.,-3.96972446532832));
#68027=CARTESIAN_POINT('Ctrl Pts',(-0.773798212026683,1.,-3.96218649639876));
#68028=CARTESIAN_POINT('Ctrl Pts',(-0.775154418039441,1.,-3.95464885452364));
#68029=CARTESIAN_POINT('Ctrl Pts',(-0.77646896669796,1.,-3.94711101619471));
#68030=CARTESIAN_POINT('Ctrl Pts',(-0.77774137056855,1.,-3.93957296768098));
#68031=CARTESIAN_POINT('Ctrl Pts',(-0.778971308134786,1.,-3.93203552473153));
#68032=CARTESIAN_POINT('Ctrl Pts',(-0.780158678615507,1.,-3.92450058323799));
#68033=CARTESIAN_POINT('Ctrl Pts',(-0.781303428618344,1.,-3.9169703605466));
#68034=CARTESIAN_POINT('Ctrl Pts',(-0.782405395622759,1.,-3.90944671004536));
#68035=CARTESIAN_POINT('Ctrl Pts',(-0.783464141529082,1.,-3.90193039043971));
#68036=CARTESIAN_POINT('Ctrl Pts',(-0.784478799358336,1.,-3.89442039235105));
#68037=CARTESIAN_POINT('Ctrl Pts',(-0.785447890340723,1.,-3.88691313167399));
#68038=CARTESIAN_POINT('Ctrl Pts',(-0.786369675812592,1.,-3.87940402818186));
#68039=CARTESIAN_POINT('Ctrl Pts',(-0.78724252761798,1.,-3.87188916600905));
#68040=CARTESIAN_POINT('Ctrl Pts',(-0.788065315093771,1.,-3.86436702561342));
#68041=CARTESIAN_POINT('Ctrl Pts',(-0.788837734090688,1.,-3.85683995872536));
#68042=CARTESIAN_POINT('Ctrl Pts',(-0.789560798155619,1.,-3.8493163780891));
#68043=CARTESIAN_POINT('Ctrl Pts',(-0.790236124191289,1.,-3.84180762342476));
#68044=CARTESIAN_POINT('Ctrl Pts',(-0.79086501270534,1.,-3.83432392054804));
#68045=CARTESIAN_POINT('Ctrl Pts',(-0.791447528662381,1.,-3.82687033899799));
#68046=CARTESIAN_POINT('Ctrl Pts',(-0.791981740718606,1.,-3.81944345442237));
#68047=CARTESIAN_POINT('Ctrl Pts',(-0.792462483517568,1.,-3.81202588694726));
#68048=CARTESIAN_POINT('Ctrl Pts',(-0.792882695234693,1.,-3.80459229925598));
#68049=CARTESIAN_POINT('Ctrl Pts',(-0.7932356129732,1.,-3.79711921389862));
#68050=CARTESIAN_POINT('Ctrl Pts',(-0.793516871680966,1.,-3.78959439439222));
#68051=CARTESIAN_POINT('Ctrl Pts',(-0.793726235781339,1.,-3.78202460377617));
#68052=CARTESIAN_POINT('Ctrl Pts',(-0.793870523787515,1.,-3.77444863801264));
#68053=CARTESIAN_POINT('Ctrl Pts',(-0.793961083689141,1.,-3.76692626931184));
#68054=CARTESIAN_POINT('Ctrl Pts',(-0.794008429135047,1.,-3.75951468666325));
#68055=CARTESIAN_POINT('Ctrl Pts',(-0.794017347371441,1.,-3.75224692493895));
#68056=CARTESIAN_POINT('Ctrl Pts',(-0.79398270045988,1.,-3.74511357728827));
#68057=CARTESIAN_POINT('Ctrl Pts',(-0.79388270093679,1.,-3.73803280541576));
#68058=CARTESIAN_POINT('Ctrl Pts',(-0.793682750269347,1.,-3.7308691469564));
#68059=CARTESIAN_POINT('Ctrl Pts',(-0.79334702378387,1.,-3.7234879729357));
#68060=CARTESIAN_POINT('Ctrl Pts',(-0.792848377370115,1.,-3.7158024239604));
#68061=CARTESIAN_POINT('Ctrl Pts',(-0.792177688845968,1.,-3.70781724021879));
#68062=CARTESIAN_POINT('Ctrl Pts',(-0.791356575696509,1.,-3.69968940808982));
#68063=CARTESIAN_POINT('Ctrl Pts',(-0.79043628498958,1.,-3.69172044327754));
#68064=CARTESIAN_POINT('Ctrl Pts',(-0.789483546065158,1.,-3.68428439784285));
#68065=CARTESIAN_POINT('Ctrl Pts',(-0.788569566220662,1.,-3.67777119516438));
#68066=CARTESIAN_POINT('Ctrl Pts',(-0.787758799995426,1.,-3.672529236635));
#68067=CARTESIAN_POINT('Ctrl Pts',(-0.787145041181589,1.,-3.66907505398769));
#68068=CARTESIAN_POINT('Ctrl Pts',(-0.7867743371985,1.,-3.66743103898844));
#68069=CARTESIAN_POINT('Ctrl Pts',(-0.78656591955989,1.,-3.66680946938396));
#68070=CARTESIAN_POINT('Ctrl Pts',(-0.786459983896781,1.,-3.66664310415236));
#68071=CARTESIAN_POINT('Ctrl Pts',(-0.786422660833743,1.,-3.66661143271648));
#68072=CARTESIAN_POINT('',(-0.732042837400619,0.,-4.13571194405636));
#68073=CARTESIAN_POINT('Ctrl Pts',(-0.385214314776329,-1.,-3.73016218570874));
#68074=CARTESIAN_POINT('Ctrl Pts',(-0.385214314776329,1.,-3.73016218570874));
#68075=CARTESIAN_POINT('Ctrl Pts',(-0.385147278814804,-1.,-3.73010668803185));
#68076=CARTESIAN_POINT('Ctrl Pts',(-0.385147278814804,1.,-3.73010668803185));
#68077=CARTESIAN_POINT('Ctrl Pts',(-0.385047711603887,-1.,-3.73015851028729));
#68078=CARTESIAN_POINT('Ctrl Pts',(-0.385047711603887,1.,-3.73015851028729));
#68079=CARTESIAN_POINT('Ctrl Pts',(-0.385001870183841,-1.,-3.73072465900727));
#68080=CARTESIAN_POINT('Ctrl Pts',(-0.385001870183841,1.,-3.73072465900727));
#68081=CARTESIAN_POINT('Ctrl Pts',(-0.385147887989515,-1.,-3.73245705639337));
#68082=CARTESIAN_POINT('Ctrl Pts',(-0.385147887989515,1.,-3.73245705639337));
#68083=CARTESIAN_POINT('Ctrl Pts',(-0.385670806454744,-1.,-3.73621371845475));
#68084=CARTESIAN_POINT('Ctrl Pts',(-0.385670806454744,1.,-3.73621371845475));
#68085=CARTESIAN_POINT('Ctrl Pts',(-0.386519576222035,-1.,-3.74144965781088));
#68086=CARTESIAN_POINT('Ctrl Pts',(-0.386519576222035,1.,-3.74144965781088));
#68087=CARTESIAN_POINT('Ctrl Pts',(-0.387663020050396,-1.,-3.74792651696269));
#68088=CARTESIAN_POINT('Ctrl Pts',(-0.387663020050396,1.,-3.74792651696269));
#68089=CARTESIAN_POINT('Ctrl Pts',(-0.389054775898251,-1.,-3.75529302894757));
#68090=CARTESIAN_POINT('Ctrl Pts',(-0.389054775898251,1.,-3.75529302894757));
#68091=CARTESIAN_POINT('Ctrl Pts',(-0.390642072979259,-1.,-3.76315635032993));
#68092=CARTESIAN_POINT('Ctrl Pts',(-0.390642072979259,1.,-3.76315635032993));
#68093=CARTESIAN_POINT('Ctrl Pts',(-0.392372786223347,-1.,-3.77114011595892));
#68094=CARTESIAN_POINT('Ctrl Pts',(-0.392372786223347,1.,-3.77114011595892));
#68095=CARTESIAN_POINT('Ctrl Pts',(-0.394202481011595,-1.,-3.77894173114368));
#68096=CARTESIAN_POINT('Ctrl Pts',(-0.394202481011595,1.,-3.77894173114368));
#68097=CARTESIAN_POINT('Ctrl Pts',(-0.396103205335029,-1.,-3.78640521279479));
#68098=CARTESIAN_POINT('Ctrl Pts',(-0.396103205335029,1.,-3.78640521279479));
#68099=CARTESIAN_POINT('Ctrl Pts',(-0.398064818684158,-1.,-3.79352887163457));
#68100=CARTESIAN_POINT('Ctrl Pts',(-0.398064818684158,1.,-3.79352887163457));
#68101=CARTESIAN_POINT('Ctrl Pts',(-0.400088346504727,-1.,-3.80040370384659));
#68102=CARTESIAN_POINT('Ctrl Pts',(-0.400088346504727,1.,-3.80040370384659));
#68103=CARTESIAN_POINT('Ctrl Pts',(-0.402181320148475,-1.,-3.80716881962763));
#68104=CARTESIAN_POINT('Ctrl Pts',(-0.402181320148475,1.,-3.80716881962763));
#68105=CARTESIAN_POINT('Ctrl Pts',(-0.404352694628236,-1.,-3.81396374287762));
#68106=CARTESIAN_POINT('Ctrl Pts',(-0.404352694628236,1.,-3.81396374287762));
#68107=CARTESIAN_POINT('Ctrl Pts',(-0.406607038258906,-1.,-3.82087303913741));
#68108=CARTESIAN_POINT('Ctrl Pts',(-0.406607038258906,1.,-3.82087303913741));
#68109=CARTESIAN_POINT('Ctrl Pts',(-0.408942371447377,-1.,-3.82790724256397));
#68110=CARTESIAN_POINT('Ctrl Pts',(-0.408942371447377,1.,-3.82790724256397));
#68111=CARTESIAN_POINT('Ctrl Pts',(-0.41135303879846,-1.,-3.83503345578645));
#68112=CARTESIAN_POINT('Ctrl Pts',(-0.41135303879846,1.,-3.83503345578645));
#68113=CARTESIAN_POINT('Ctrl Pts',(-0.413831367016727,-1.,-3.84219403994742));
#68114=CARTESIAN_POINT('Ctrl Pts',(-0.413831367016727,1.,-3.84219403994742));
#68115=CARTESIAN_POINT('Ctrl Pts',(-0.41636967805292,-1.,-3.8493286415751));
#68116=CARTESIAN_POINT('Ctrl Pts',(-0.41636967805292,1.,-3.8493286415751));
#68117=CARTESIAN_POINT('Ctrl Pts',(-0.41896246808681,-1.,-3.85639825648031));
#68118=CARTESIAN_POINT('Ctrl Pts',(-0.41896246808681,1.,-3.85639825648031));
#68119=CARTESIAN_POINT('Ctrl Pts',(-0.421607423177576,-1.,-3.86339652542749));
#68120=CARTESIAN_POINT('Ctrl Pts',(-0.421607423177576,1.,-3.86339652542749));
#68121=CARTESIAN_POINT('Ctrl Pts',(-0.424304173195142,-1.,-3.87033643487882));
#68122=CARTESIAN_POINT('Ctrl Pts',(-0.424304173195142,1.,-3.87033643487882));
#68123=CARTESIAN_POINT('Ctrl Pts',(-0.427053541173469,-1.,-3.87724240306609));
#68124=CARTESIAN_POINT('Ctrl Pts',(-0.427053541173469,1.,-3.87724240306609));
#68125=CARTESIAN_POINT('Ctrl Pts',(-0.429856640579734,-1.,-3.88414070943334));
#68126=CARTESIAN_POINT('Ctrl Pts',(-0.429856640579734,1.,-3.88414070943334));
#68127=CARTESIAN_POINT('Ctrl Pts',(-0.432713929544439,-1.,-3.89104947940592));
#68128=CARTESIAN_POINT('Ctrl Pts',(-0.432713929544439,1.,-3.89104947940592));
#68129=CARTESIAN_POINT('Ctrl Pts',(-0.435624629433506,-1.,-3.8979725665544));
#68130=CARTESIAN_POINT('Ctrl Pts',(-0.435624629433506,1.,-3.8979725665544));
#68131=CARTESIAN_POINT('Ctrl Pts',(-0.438587235458233,-1.,-3.90490512938546));
#68132=CARTESIAN_POINT('Ctrl Pts',(-0.438587235458233,1.,-3.90490512938546));
#68133=CARTESIAN_POINT('Ctrl Pts',(-0.441599824524047,-1.,-3.91183704069146));
#68134=CARTESIAN_POINT('Ctrl Pts',(-0.441599824524047,1.,-3.91183704069146));
#68135=CARTESIAN_POINT('Ctrl Pts',(-0.444660430230593,-1.,-3.91875701610721));
#68136=CARTESIAN_POINT('Ctrl Pts',(-0.444660430230593,1.,-3.91875701610721));
#68137=CARTESIAN_POINT('Ctrl Pts',(-0.447767416837297,-1.,-3.92565674143424));
#68138=CARTESIAN_POINT('Ctrl Pts',(-0.447767416837297,1.,-3.92565674143424));
#68139=CARTESIAN_POINT('Ctrl Pts',(-0.450919768356347,-1.,-3.93253407403128));
#68140=CARTESIAN_POINT('Ctrl Pts',(-0.450919768356347,1.,-3.93253407403128));
#68141=CARTESIAN_POINT('Ctrl Pts',(-0.454116879027576,-1.,-3.93939080846298));
#68142=CARTESIAN_POINT('Ctrl Pts',(-0.454116879027576,1.,-3.93939080846298));
#68143=CARTESIAN_POINT('Ctrl Pts',(-0.457358410451674,-1.,-3.94623117206675));
#68144=CARTESIAN_POINT('Ctrl Pts',(-0.457358410451674,1.,-3.94623117206675));
#68145=CARTESIAN_POINT('Ctrl Pts',(-0.460644124429119,-1.,-3.95306005817363));
#68146=CARTESIAN_POINT('Ctrl Pts',(-0.460644124429119,1.,-3.95306005817363));
#68147=CARTESIAN_POINT('Ctrl Pts',(-0.463973722115744,-1.,-3.95988133243543));
#68148=CARTESIAN_POINT('Ctrl Pts',(-0.463973722115744,1.,-3.95988133243543));
#68149=CARTESIAN_POINT('Ctrl Pts',(-0.467346690880672,-1.,-3.96669622273946));
#68150=CARTESIAN_POINT('Ctrl Pts',(-0.467346690880672,1.,-3.96669622273946));
#68151=CARTESIAN_POINT('Ctrl Pts',(-0.470762379613477,-1.,-3.97350414289415));
#68152=CARTESIAN_POINT('Ctrl Pts',(-0.470762379613477,1.,-3.97350414289415));
#68153=CARTESIAN_POINT('Ctrl Pts',(-0.474220061019542,-1.,-3.9803033804443));
#68154=CARTESIAN_POINT('Ctrl Pts',(-0.474220061019542,1.,-3.9803033804443));
#68155=CARTESIAN_POINT('Ctrl Pts',(-0.477718999122033,-1.,-3.98709184306743));
#68156=CARTESIAN_POINT('Ctrl Pts',(-0.477718999122033,1.,-3.98709184306743));
#68157=CARTESIAN_POINT('Ctrl Pts',(-0.481258512209638,-1.,-3.99386775880655));
#68158=CARTESIAN_POINT('Ctrl Pts',(-0.481258512209638,1.,-3.99386775880655));
#68159=CARTESIAN_POINT('Ctrl Pts',(-0.484838042421754,-1.,-4.00063045119234));
#68160=CARTESIAN_POINT('Ctrl Pts',(-0.484838042421754,1.,-4.00063045119234));
#68161=CARTESIAN_POINT('Ctrl Pts',(-0.488457130424531,-1.,-4.0073800839092));
#68162=CARTESIAN_POINT('Ctrl Pts',(-0.488457130424531,1.,-4.0073800839092));
#68163=CARTESIAN_POINT('Ctrl Pts',(-0.492115383417931,-1.,-4.01411733503486));
#68164=CARTESIAN_POINT('Ctrl Pts',(-0.492115383417931,1.,-4.01411733503486));
#68165=CARTESIAN_POINT('Ctrl Pts',(-0.495812444326223,-1.,-4.02084308851813));
#68166=CARTESIAN_POINT('Ctrl Pts',(-0.495812444326223,1.,-4.02084308851813));
#68167=CARTESIAN_POINT('Ctrl Pts',(-0.49954796234089,-1.,-4.0275581398015));
#68168=CARTESIAN_POINT('Ctrl Pts',(-0.49954796234089,1.,-4.0275581398015));
#68169=CARTESIAN_POINT('Ctrl Pts',(-0.503321556915514,-1.,-4.0342628417439));
#68170=CARTESIAN_POINT('Ctrl Pts',(-0.503321556915514,1.,-4.0342628417439));
#68171=CARTESIAN_POINT('Ctrl Pts',(-0.507132823288362,-1.,-4.04095715149074));
#68172=CARTESIAN_POINT('Ctrl Pts',(-0.507132823288362,1.,-4.04095715149074));
#68173=CARTESIAN_POINT('Ctrl Pts',(-0.510981349219174,-1.,-4.04764078815591));
#68174=CARTESIAN_POINT('Ctrl Pts',(-0.510981349219174,1.,-4.04764078815591));
#68175=CARTESIAN_POINT('Ctrl Pts',(-0.514866728193104,-1.,-4.05431335771261));
#68176=CARTESIAN_POINT('Ctrl Pts',(-0.514866728193104,1.,-4.05431335771261));
#68177=CARTESIAN_POINT('Ctrl Pts',(-0.51878857233681,-1.,-4.06097448037934));
#68178=CARTESIAN_POINT('Ctrl Pts',(-0.51878857233681,1.,-4.06097448037934));
#68179=CARTESIAN_POINT('Ctrl Pts',(-0.522746528602768,-1.,-4.06762394471075));
#68180=CARTESIAN_POINT('Ctrl Pts',(-0.522746528602768,1.,-4.06762394471075));
#68181=CARTESIAN_POINT('Ctrl Pts',(-0.526740277227,-1.,-4.07426172299496));
#68182=CARTESIAN_POINT('Ctrl Pts',(-0.526740277227,1.,-4.07426172299496));
#68183=CARTESIAN_POINT('Ctrl Pts',(-0.530769518728075,-1.,-4.08088789536488));
#68184=CARTESIAN_POINT('Ctrl Pts',(-0.530769518728075,1.,-4.08088789536488));
#68185=CARTESIAN_POINT('Ctrl Pts',(-0.534833963476999,-1.,-4.08750259988693));
#68186=CARTESIAN_POINT('Ctrl Pts',(-0.534833963476999,1.,-4.08750259988693));
#68187=CARTESIAN_POINT('Ctrl Pts',(-0.538933321179921,-1.,-4.09410597627116));
#68188=CARTESIAN_POINT('Ctrl Pts',(-0.538933321179921,1.,-4.09410597627116));
#68189=CARTESIAN_POINT('Ctrl Pts',(-0.543067286878457,-1.,-4.10069810244473));
#68190=CARTESIAN_POINT('Ctrl Pts',(-0.543067286878457,1.,-4.10069810244473));
#68191=CARTESIAN_POINT('Ctrl Pts',(-0.54723553948676,-1.,-4.1072789702877));
#68192=CARTESIAN_POINT('Ctrl Pts',(-0.54723553948676,1.,-4.1072789702877));
#68193=CARTESIAN_POINT('Ctrl Pts',(-0.551437758498247,-1.,-4.11384852025578));
#68194=CARTESIAN_POINT('Ctrl Pts',(-0.551437758498247,1.,-4.11384852025578));
#68195=CARTESIAN_POINT('Ctrl Pts',(-0.555673636130778,-1.,-4.1204066619623));
#68196=CARTESIAN_POINT('Ctrl Pts',(-0.555673636130778,1.,-4.1204066619623));
#68197=CARTESIAN_POINT('Ctrl Pts',(-0.559942890594628,-1.,-4.12695329951859));
#68198=CARTESIAN_POINT('Ctrl Pts',(-0.559942890594628,1.,-4.12695329951859));
#68199=CARTESIAN_POINT('Ctrl Pts',(-0.564245279535705,-1.,-4.13348835726086));
#68200=CARTESIAN_POINT('Ctrl Pts',(-0.564245279535705,1.,-4.13348835726086));
#68201=CARTESIAN_POINT('Ctrl Pts',(-0.568580610187116,-1.,-4.14001179828669));
#68202=CARTESIAN_POINT('Ctrl Pts',(-0.568580610187116,1.,-4.14001179828669));
#68203=CARTESIAN_POINT('Ctrl Pts',(-0.572948736066277,-1.,-4.14652361065787));
#68204=CARTESIAN_POINT('Ctrl Pts',(-0.572948736066277,1.,-4.14652361065787));
#68205=CARTESIAN_POINT('Ctrl Pts',(-0.576469391673917,-1.,-4.1517237611974));
#68206=CARTESIAN_POINT('Ctrl Pts',(-0.576469391673917,1.,-4.1517237611974));
#68207=CARTESIAN_POINT('Ctrl Pts',(-0.579124568912543,-1.,-4.15561864787379));
#68208=CARTESIAN_POINT('Ctrl Pts',(-0.579124568912543,1.,-4.15561864787379));
#68209=CARTESIAN_POINT('Ctrl Pts',(-0.580901211462913,-1.,-4.15821291712391));
#68210=CARTESIAN_POINT('Ctrl Pts',(-0.580901211462913,1.,-4.15821291712391));
#68211=CARTESIAN_POINT('Ctrl Pts',(-0.581791163835814,-1.,-4.15950947128175));
#68212=CARTESIAN_POINT('Ctrl Pts',(-0.581791163835814,1.,-4.15950947128175));
#68213=CARTESIAN_POINT('',(-0.385112848332548,1.,-3.73017266276632));
#68214=CARTESIAN_POINT('Ctrl Pts',(-0.385112848332549,-1.,-3.73017266276632));
#68215=CARTESIAN_POINT('Ctrl Pts',(-0.385112848332549,-0.666666666666667,
-3.73017266276632));
#68216=CARTESIAN_POINT('Ctrl Pts',(-0.385112848332549,-0.333333333333333,
-3.73017266276632));
#68217=CARTESIAN_POINT('Ctrl Pts',(-0.385112848332549,0.333333333333333,
-3.73017266276632));
#68218=CARTESIAN_POINT('Ctrl Pts',(-0.385112848332549,0.666666666666667,
-3.73017266276632));
#68219=CARTESIAN_POINT('Ctrl Pts',(-0.385112848332549,1.,-3.73017266276632));
#68220=CARTESIAN_POINT('',(-0.581791163835814,1.,-4.15950947128175));
#68221=CARTESIAN_POINT('',(-0.581791163835814,0.,-4.15950947128175));
#68222=CARTESIAN_POINT('Ctrl Pts',(-0.385112848332549,1.,-3.73017266276632));
#68223=CARTESIAN_POINT('Ctrl Pts',(-0.385087139001609,1.,-3.73021431755218));
#68224=CARTESIAN_POINT('Ctrl Pts',(-0.385037797882046,1.,-3.73040527620929));
#68225=CARTESIAN_POINT('Ctrl Pts',(-0.385031656499142,1.,-3.731060828624));
#68226=CARTESIAN_POINT('Ctrl Pts',(-0.385187124633965,1.,-3.73273893363318));
#68227=CARTESIAN_POINT('Ctrl Pts',(-0.385670806454744,1.,-3.73621371845475));
#68228=CARTESIAN_POINT('Ctrl Pts',(-0.386519576222035,1.,-3.74144965781088));
#68229=CARTESIAN_POINT('Ctrl Pts',(-0.387663020050396,1.,-3.74792651696269));
#68230=CARTESIAN_POINT('Ctrl Pts',(-0.389054775898251,1.,-3.75529302894757));
#68231=CARTESIAN_POINT('Ctrl Pts',(-0.390642072979259,1.,-3.76315635032993));
#68232=CARTESIAN_POINT('Ctrl Pts',(-0.392372786223347,1.,-3.77114011595892));
#68233=CARTESIAN_POINT('Ctrl Pts',(-0.394202481011595,1.,-3.77894173114368));
#68234=CARTESIAN_POINT('Ctrl Pts',(-0.396103205335029,1.,-3.78640521279479));
#68235=CARTESIAN_POINT('Ctrl Pts',(-0.398064818684158,1.,-3.79352887163457));
#68236=CARTESIAN_POINT('Ctrl Pts',(-0.400088346504727,1.,-3.80040370384659));
#68237=CARTESIAN_POINT('Ctrl Pts',(-0.402181320148475,1.,-3.80716881962763));
#68238=CARTESIAN_POINT('Ctrl Pts',(-0.404352694628236,1.,-3.81396374287762));
#68239=CARTESIAN_POINT('Ctrl Pts',(-0.406607038258906,1.,-3.82087303913741));
#68240=CARTESIAN_POINT('Ctrl Pts',(-0.408942371447377,1.,-3.82790724256397));
#68241=CARTESIAN_POINT('Ctrl Pts',(-0.41135303879846,1.,-3.83503345578645));
#68242=CARTESIAN_POINT('Ctrl Pts',(-0.413831367016727,1.,-3.84219403994742));
#68243=CARTESIAN_POINT('Ctrl Pts',(-0.41636967805292,1.,-3.8493286415751));
#68244=CARTESIAN_POINT('Ctrl Pts',(-0.41896246808681,1.,-3.85639825648031));
#68245=CARTESIAN_POINT('Ctrl Pts',(-0.421607423177576,1.,-3.86339652542749));
#68246=CARTESIAN_POINT('Ctrl Pts',(-0.424304173195142,1.,-3.87033643487882));
#68247=CARTESIAN_POINT('Ctrl Pts',(-0.427053541173469,1.,-3.87724240306609));
#68248=CARTESIAN_POINT('Ctrl Pts',(-0.429856640579734,1.,-3.88414070943334));
#68249=CARTESIAN_POINT('Ctrl Pts',(-0.432713929544439,1.,-3.89104947940592));
#68250=CARTESIAN_POINT('Ctrl Pts',(-0.435624629433506,1.,-3.8979725665544));
#68251=CARTESIAN_POINT('Ctrl Pts',(-0.438587235458233,1.,-3.90490512938546));
#68252=CARTESIAN_POINT('Ctrl Pts',(-0.441599824524047,1.,-3.91183704069146));
#68253=CARTESIAN_POINT('Ctrl Pts',(-0.444660430230593,1.,-3.91875701610721));
#68254=CARTESIAN_POINT('Ctrl Pts',(-0.447767416837297,1.,-3.92565674143424));
#68255=CARTESIAN_POINT('Ctrl Pts',(-0.450919768356347,1.,-3.93253407403128));
#68256=CARTESIAN_POINT('Ctrl Pts',(-0.454116879027576,1.,-3.93939080846298));
#68257=CARTESIAN_POINT('Ctrl Pts',(-0.457358410451674,1.,-3.94623117206675));
#68258=CARTESIAN_POINT('Ctrl Pts',(-0.460644124429119,1.,-3.95306005817363));
#68259=CARTESIAN_POINT('Ctrl Pts',(-0.463973722115744,1.,-3.95988133243543));
#68260=CARTESIAN_POINT('Ctrl Pts',(-0.467346690880672,1.,-3.96669622273946));
#68261=CARTESIAN_POINT('Ctrl Pts',(-0.470762379613477,1.,-3.97350414289415));
#68262=CARTESIAN_POINT('Ctrl Pts',(-0.474220061019542,1.,-3.9803033804443));
#68263=CARTESIAN_POINT('Ctrl Pts',(-0.477718999122033,1.,-3.98709184306743));
#68264=CARTESIAN_POINT('Ctrl Pts',(-0.481258512209638,1.,-3.99386775880655));
#68265=CARTESIAN_POINT('Ctrl Pts',(-0.484838042421754,1.,-4.00063045119234));
#68266=CARTESIAN_POINT('Ctrl Pts',(-0.488457130424531,1.,-4.0073800839092));
#68267=CARTESIAN_POINT('Ctrl Pts',(-0.492115383417931,1.,-4.01411733503486));
#68268=CARTESIAN_POINT('Ctrl Pts',(-0.495812444326223,1.,-4.02084308851813));
#68269=CARTESIAN_POINT('Ctrl Pts',(-0.49954796234089,1.,-4.0275581398015));
#68270=CARTESIAN_POINT('Ctrl Pts',(-0.503321556915514,1.,-4.0342628417439));
#68271=CARTESIAN_POINT('Ctrl Pts',(-0.507132823288362,1.,-4.04095715149074));
#68272=CARTESIAN_POINT('Ctrl Pts',(-0.510981349219174,1.,-4.04764078815591));
#68273=CARTESIAN_POINT('Ctrl Pts',(-0.514866728193104,1.,-4.05431335771261));
#68274=CARTESIAN_POINT('Ctrl Pts',(-0.51878857233681,1.,-4.06097448037934));
#68275=CARTESIAN_POINT('Ctrl Pts',(-0.522746528602768,1.,-4.06762394471075));
#68276=CARTESIAN_POINT('Ctrl Pts',(-0.526740277227,1.,-4.07426172299496));
#68277=CARTESIAN_POINT('Ctrl Pts',(-0.530769518728075,1.,-4.08088789536488));
#68278=CARTESIAN_POINT('Ctrl Pts',(-0.534833963476999,1.,-4.08750259988693));
#68279=CARTESIAN_POINT('Ctrl Pts',(-0.538933321179921,1.,-4.09410597627116));
#68280=CARTESIAN_POINT('Ctrl Pts',(-0.543067286878457,1.,-4.10069810244473));
#68281=CARTESIAN_POINT('Ctrl Pts',(-0.54723553948676,1.,-4.1072789702877));
#68282=CARTESIAN_POINT('Ctrl Pts',(-0.551437758498247,1.,-4.11384852025578));
#68283=CARTESIAN_POINT('Ctrl Pts',(-0.555673636130778,1.,-4.1204066619623));
#68284=CARTESIAN_POINT('Ctrl Pts',(-0.559942890594628,1.,-4.12695329951859));
#68285=CARTESIAN_POINT('Ctrl Pts',(-0.564245279535705,1.,-4.13348835726086));
#68286=CARTESIAN_POINT('Ctrl Pts',(-0.568580610187116,1.,-4.14001179828669));
#68287=CARTESIAN_POINT('Ctrl Pts',(-0.572948736066277,1.,-4.14652361065787));
#68288=CARTESIAN_POINT('Ctrl Pts',(-0.576469391673917,1.,-4.1517237611974));
#68289=CARTESIAN_POINT('Ctrl Pts',(-0.579124568912543,1.,-4.15561864787379));
#68290=CARTESIAN_POINT('Ctrl Pts',(-0.580901211462913,1.,-4.15821291712391));
#68291=CARTESIAN_POINT('Ctrl Pts',(-0.581791163835814,1.,-4.15950947128175));
#68292=CARTESIAN_POINT('Origin',(-0.581791163835814,0.,-4.15950947128175));
#68293=CARTESIAN_POINT('',(-0.732042837400619,1.,-4.13571194405636));
#68294=CARTESIAN_POINT('Origin',(0.,0.,0.));
#68295=CARTESIAN_POINT('',(-0.203156094897896,1.,-3.74449296982994));
#68296=CARTESIAN_POINT('Origin',(0.,1.,0.));
#68297=CARTESIAN_POINT('Ctrl Pts',(-0.203156094897896,1.,-3.74449296982994));
#68298=CARTESIAN_POINT('Ctrl Pts',(-0.203156094897896,0.666666666666667,
-3.74449296982994));
#68299=CARTESIAN_POINT('Ctrl Pts',(-0.203156094897896,0.333333333333333,
-3.74449296982994));
#68300=CARTESIAN_POINT('Ctrl Pts',(-0.203156094897896,-0.333333333333333,
-3.74449296982994));
#68301=CARTESIAN_POINT('Ctrl Pts',(-0.203156094897896,-0.666666666666667,
-3.74449296982994));
#68302=CARTESIAN_POINT('Ctrl Pts',(-0.203156094897896,-1.,-3.74449296982994));
#68303=CARTESIAN_POINT('Ctrl Pts',(-0.0760622897878238,-1.,-4.19931119685982));
#68304=CARTESIAN_POINT('Ctrl Pts',(-0.0760622897878238,1.,-4.19931119685982));
#68305=CARTESIAN_POINT('Ctrl Pts',(-0.0767384596142197,-1.,-4.19789138621624));
#68306=CARTESIAN_POINT('Ctrl Pts',(-0.0767384596142197,1.,-4.19789138621624));
#68307=CARTESIAN_POINT('Ctrl Pts',(-0.0780873956244405,-1.,-4.19505112860624));
#68308=CARTESIAN_POINT('Ctrl Pts',(-0.0780873956244405,1.,-4.19505112860624));
#68309=CARTESIAN_POINT('Ctrl Pts',(-0.0801005887117605,-1.,-4.19078883322483));
#68310=CARTESIAN_POINT('Ctrl Pts',(-0.0801005887117605,1.,-4.19078883322483));
#68311=CARTESIAN_POINT('Ctrl Pts',(-0.0827644164389512,-1.,-4.1851019532944));
#68312=CARTESIAN_POINT('Ctrl Pts',(-0.0827644164389512,1.,-4.1851019532944));
#68313=CARTESIAN_POINT('Ctrl Pts',(-0.0860600915552517,-1.,-4.17798698669991));
#68314=CARTESIAN_POINT('Ctrl Pts',(-0.0860600915552517,1.,-4.17798698669991));
#68315=CARTESIAN_POINT('Ctrl Pts',(-0.089321556085033,-1.,-4.17086566491823));
#68316=CARTESIAN_POINT('Ctrl Pts',(-0.089321556085033,1.,-4.17086566491823));
#68317=CARTESIAN_POINT('Ctrl Pts',(-0.0925486672167692,-1.,-4.16373802265942));
#68318=CARTESIAN_POINT('Ctrl Pts',(-0.0925486672167692,1.,-4.16373802265942));
#68319=CARTESIAN_POINT('Ctrl Pts',(-0.095741240329707,-1.,-4.15660412653006));
#68320=CARTESIAN_POINT('Ctrl Pts',(-0.095741240329707,1.,-4.15660412653006));
#68321=CARTESIAN_POINT('Ctrl Pts',(-0.0988990478899814,-1.,-4.1494640891762));
#68322=CARTESIAN_POINT('Ctrl Pts',(-0.0988990478899814,1.,-4.1494640891762));
#68323=CARTESIAN_POINT('Ctrl Pts',(-0.102021826577454,-1.,-4.14231804938737));
#68324=CARTESIAN_POINT('Ctrl Pts',(-0.102021826577454,1.,-4.14231804938737));
#68325=CARTESIAN_POINT('Ctrl Pts',(-0.105109286538864,-1.,-4.13516614458396));
#68326=CARTESIAN_POINT('Ctrl Pts',(-0.105109286538864,1.,-4.13516614458396));
#68327=CARTESIAN_POINT('Ctrl Pts',(-0.10816112052835,-1.,-4.12800848371386));
#68328=CARTESIAN_POINT('Ctrl Pts',(-0.10816112052835,1.,-4.12800848371386));
#68329=CARTESIAN_POINT('Ctrl Pts',(-0.111177012683377,-1.,-4.12084512502444));
#68330=CARTESIAN_POINT('Ctrl Pts',(-0.111177012683377,1.,-4.12084512502444));
#68331=CARTESIAN_POINT('Ctrl Pts',(-0.114156649609602,-1.,-4.11367603925313));
#68332=CARTESIAN_POINT('Ctrl Pts',(-0.114156649609602,1.,-4.11367603925313));
#68333=CARTESIAN_POINT('Ctrl Pts',(-0.117099722731705,-1.,-4.10650113382187));
#68334=CARTESIAN_POINT('Ctrl Pts',(-0.117099722731705,1.,-4.10650113382187));
#68335=CARTESIAN_POINT('Ctrl Pts',(-0.120005924388162,-1.,-4.09932031767243));
#68336=CARTESIAN_POINT('Ctrl Pts',(-0.120005924388162,1.,-4.09932031767243));
#68337=CARTESIAN_POINT('Ctrl Pts',(-0.122874946249119,-1.,-4.09213355850836));
#68338=CARTESIAN_POINT('Ctrl Pts',(-0.122874946249119,1.,-4.09213355850836));
#68339=CARTESIAN_POINT('Ctrl Pts',(-0.125706476822529,-1.,-4.08494093372315));
#68340=CARTESIAN_POINT('Ctrl Pts',(-0.125706476822529,1.,-4.08494093372315));
#68341=CARTESIAN_POINT('Ctrl Pts',(-0.128500200484814,-1.,-4.07774270738809));
#68342=CARTESIAN_POINT('Ctrl Pts',(-0.128500200484814,1.,-4.07774270738809));
#68343=CARTESIAN_POINT('Ctrl Pts',(-0.131255793548914,-1.,-4.07053931528579));
#68344=CARTESIAN_POINT('Ctrl Pts',(-0.131255793548914,1.,-4.07053931528579));
#68345=CARTESIAN_POINT('Ctrl Pts',(-0.133972916144225,-1.,-4.06333121018476));
#68346=CARTESIAN_POINT('Ctrl Pts',(-0.133972916144225,1.,-4.06333121018476));
#68347=CARTESIAN_POINT('Ctrl Pts',(-0.136651205046111,-1.,-4.05611873400122));
#68348=CARTESIAN_POINT('Ctrl Pts',(-0.136651205046111,1.,-4.05611873400122));
#68349=CARTESIAN_POINT('Ctrl Pts',(-0.13929026718006,-1.,-4.04890199238056));
#68350=CARTESIAN_POINT('Ctrl Pts',(-0.13929026718006,1.,-4.04890199238056));
#68351=CARTESIAN_POINT('Ctrl Pts',(-0.141889671485508,-1.,-4.04168069633842));
#68352=CARTESIAN_POINT('Ctrl Pts',(-0.141889671485508,1.,-4.04168069633842));
#68353=CARTESIAN_POINT('Ctrl Pts',(-0.144448947038352,-1.,-4.03445411510403));
#68354=CARTESIAN_POINT('Ctrl Pts',(-0.144448947038352,1.,-4.03445411510403));
#68355=CARTESIAN_POINT('Ctrl Pts',(-0.146967602878999,-1.,-4.02722143147048));
#68356=CARTESIAN_POINT('Ctrl Pts',(-0.146967602878999,1.,-4.02722143147048));
#68357=CARTESIAN_POINT('Ctrl Pts',(-0.149445144968708,-1.,-4.01998203715588));
#68358=CARTESIAN_POINT('Ctrl Pts',(-0.149445144968708,1.,-4.01998203715588));
#68359=CARTESIAN_POINT('Ctrl Pts',(-0.151881094022909,-1.,-4.01273584234684));
#68360=CARTESIAN_POINT('Ctrl Pts',(-0.151881094022909,1.,-4.01273584234684));
#68361=CARTESIAN_POINT('Ctrl Pts',(-0.15427500487231,-1.,-4.00548360245297));
#68362=CARTESIAN_POINT('Ctrl Pts',(-0.15427500487231,1.,-4.00548360245297));
#68363=CARTESIAN_POINT('Ctrl Pts',(-0.156626481393736,-1.,-3.99822717425869));
#68364=CARTESIAN_POINT('Ctrl Pts',(-0.156626481393736,1.,-3.99822717425869));
#68365=CARTESIAN_POINT('Ctrl Pts',(-0.158935123982796,-1.,-3.99096873945862));
#68366=CARTESIAN_POINT('Ctrl Pts',(-0.158935123982796,1.,-3.99096873945862));
#68367=CARTESIAN_POINT('Ctrl Pts',(-0.161200482186088,-1.,-3.98371010319866));
#68368=CARTESIAN_POINT('Ctrl Pts',(-0.161200482186088,1.,-3.98371010319866));
#68369=CARTESIAN_POINT('Ctrl Pts',(-0.163422004609999,-1.,-3.97645194630944));
#68370=CARTESIAN_POINT('Ctrl Pts',(-0.163422004609999,1.,-3.97645194630944));
#68371=CARTESIAN_POINT('Ctrl Pts',(-0.165598992851098,-1.,-3.9691931362141));
#68372=CARTESIAN_POINT('Ctrl Pts',(-0.165598992851098,1.,-3.9691931362141));
#68373=CARTESIAN_POINT('Ctrl Pts',(-0.167730547023312,-1.,-3.96192990160296));
#68374=CARTESIAN_POINT('Ctrl Pts',(-0.167730547023312,1.,-3.96192990160296));
#68375=CARTESIAN_POINT('Ctrl Pts',(-0.16981566637413,-1.,-3.95465744665263));
#68376=CARTESIAN_POINT('Ctrl Pts',(-0.16981566637413,1.,-3.95465744665263));
#68377=CARTESIAN_POINT('Ctrl Pts',(-0.171853355369233,-1.,-3.94737164900861));
#68378=CARTESIAN_POINT('Ctrl Pts',(-0.171853355369233,1.,-3.94737164900861));
#68379=CARTESIAN_POINT('Ctrl Pts',(-0.173842734974607,-1.,-3.94007083096214));
#68380=CARTESIAN_POINT('Ctrl Pts',(-0.173842734974607,1.,-3.94007083096214));
#68381=CARTESIAN_POINT('Ctrl Pts',(-0.175783136893873,-1.,-3.93275726771049));
#68382=CARTESIAN_POINT('Ctrl Pts',(-0.175783136893873,1.,-3.93275726771049));
#68383=CARTESIAN_POINT('Ctrl Pts',(-0.177674246152328,-1.,-3.92543942697672));
#68384=CARTESIAN_POINT('Ctrl Pts',(-0.177674246152328,1.,-3.92543942697672));
#68385=CARTESIAN_POINT('Ctrl Pts',(-0.179515885822895,-1.,-3.91812876180948));
#68386=CARTESIAN_POINT('Ctrl Pts',(-0.179515885822895,1.,-3.91812876180948));
#68387=CARTESIAN_POINT('Ctrl Pts',(-0.181307740731796,-1.,-3.91083557557193));
#68388=CARTESIAN_POINT('Ctrl Pts',(-0.181307740731796,1.,-3.91083557557193));
#68389=CARTESIAN_POINT('Ctrl Pts',(-0.183049081993193,-1.,-3.90356488555138));
#68390=CARTESIAN_POINT('Ctrl Pts',(-0.183049081993193,1.,-3.90356488555138));
#68391=CARTESIAN_POINT('Ctrl Pts',(-0.184738537728035,-1.,-3.89631300742633));
#68392=CARTESIAN_POINT('Ctrl Pts',(-0.184738537728035,1.,-3.89631300742633));
#68393=CARTESIAN_POINT('Ctrl Pts',(-0.186373724985263,-1.,-3.88906196725817));
#68394=CARTESIAN_POINT('Ctrl Pts',(-0.186373724985263,1.,-3.88906196725817));
#68395=CARTESIAN_POINT('Ctrl Pts',(-0.187951632512663,-1.,-3.88178563496187));
#68396=CARTESIAN_POINT('Ctrl Pts',(-0.187951632512663,1.,-3.88178563496187));
#68397=CARTESIAN_POINT('Ctrl Pts',(-0.189469253358254,-1.,-3.87445976418377));
#68398=CARTESIAN_POINT('Ctrl Pts',(-0.189469253358254,1.,-3.87445976418377));
#68399=CARTESIAN_POINT('Ctrl Pts',(-0.190924190418613,-1.,-3.8670715862477));
#68400=CARTESIAN_POINT('Ctrl Pts',(-0.190924190418613,1.,-3.8670715862477));
#68401=CARTESIAN_POINT('Ctrl Pts',(-0.19231515304498,-1.,-3.85962774407652));
#68402=CARTESIAN_POINT('Ctrl Pts',(-0.19231515304498,1.,-3.85962774407652));
#68403=CARTESIAN_POINT('Ctrl Pts',(-0.193642806777748,-1.,-3.85216762264019));
#68404=CARTESIAN_POINT('Ctrl Pts',(-0.193642806777748,1.,-3.85216762264019));
#68405=CARTESIAN_POINT('Ctrl Pts',(-0.194909009460255,-1.,-3.84475203347052));
#68406=CARTESIAN_POINT('Ctrl Pts',(-0.194909009460255,1.,-3.84475203347052));
#68407=CARTESIAN_POINT('Ctrl Pts',(-0.19611519897189,-1.,-3.83743910616265));
#68408=CARTESIAN_POINT('Ctrl Pts',(-0.19611519897189,1.,-3.83743910616265));
#68409=CARTESIAN_POINT('Ctrl Pts',(-0.197260935827375,-1.,-3.83026221776488));
#68410=CARTESIAN_POINT('Ctrl Pts',(-0.197260935827375,1.,-3.83026221776488));
#68411=CARTESIAN_POINT('Ctrl Pts',(-0.19834261690047,-1.,-3.82321127348981));
#68412=CARTESIAN_POINT('Ctrl Pts',(-0.19834261690047,1.,-3.82321127348981));
#68413=CARTESIAN_POINT('Ctrl Pts',(-0.199351525297396,-1.,-3.81620203429702));
#68414=CARTESIAN_POINT('Ctrl Pts',(-0.199351525297396,1.,-3.81620203429702));
#68415=CARTESIAN_POINT('Ctrl Pts',(-0.20027467943329,-1.,-3.80909529318501));
#68416=CARTESIAN_POINT('Ctrl Pts',(-0.20027467943329,1.,-3.80909529318501));
#68417=CARTESIAN_POINT('Ctrl Pts',(-0.201097756307252,-1.,-3.80175247447171));
#68418=CARTESIAN_POINT('Ctrl Pts',(-0.201097756307252,1.,-3.80175247447171));
#68419=CARTESIAN_POINT('Ctrl Pts',(-0.201807533800799,-1.,-3.79408354187274));
#68420=CARTESIAN_POINT('Ctrl Pts',(-0.201807533800799,1.,-3.79408354187274));
#68421=CARTESIAN_POINT('Ctrl Pts',(-0.202394260512193,-1.,-3.78609175019317));
#68422=CARTESIAN_POINT('Ctrl Pts',(-0.202394260512193,1.,-3.78609175019317));
#68423=CARTESIAN_POINT('Ctrl Pts',(-0.202854729699197,-1.,-3.77793553476879));
#68424=CARTESIAN_POINT('Ctrl Pts',(-0.202854729699197,1.,-3.77793553476879));
#68425=CARTESIAN_POINT('Ctrl Pts',(-0.203192390045337,-1.,-3.76992071595267));
#68426=CARTESIAN_POINT('Ctrl Pts',(-0.203192390045337,1.,-3.76992071595267));
#68427=CARTESIAN_POINT('Ctrl Pts',(-0.203414634707646,-1.,-3.76242717937273));
#68428=CARTESIAN_POINT('Ctrl Pts',(-0.203414634707646,1.,-3.76242717937273));
#68429=CARTESIAN_POINT('Ctrl Pts',(-0.203530796848404,-1.,-3.75585118707924));
#68430=CARTESIAN_POINT('Ctrl Pts',(-0.203530796848404,1.,-3.75585118707924));
#68431=CARTESIAN_POINT('Ctrl Pts',(-0.203550035479097,-1.,-3.75054693397716));
#68432=CARTESIAN_POINT('Ctrl Pts',(-0.203550035479097,1.,-3.75054693397716));
#68433=CARTESIAN_POINT('Ctrl Pts',(-0.20347884453023,-1.,-3.74675472018582));
#68434=CARTESIAN_POINT('Ctrl Pts',(-0.20347884453023,1.,-3.74675472018582));
#68435=CARTESIAN_POINT('Ctrl Pts',(-0.203352057956055,-1.,-3.7450208092684));
#68436=CARTESIAN_POINT('Ctrl Pts',(-0.203352057956055,1.,-3.7450208092684));
#68437=CARTESIAN_POINT('Ctrl Pts',(-0.203218215747895,-1.,-3.74446880195845));
#68438=CARTESIAN_POINT('Ctrl Pts',(-0.203218215747895,1.,-3.74446880195845));
#68439=CARTESIAN_POINT('Ctrl Pts',(-0.20311176758786,-1.,-3.74443319346666));
#68440=CARTESIAN_POINT('Ctrl Pts',(-0.20311176758786,1.,-3.74443319346666));
#68441=CARTESIAN_POINT('Ctrl Pts',(-0.203054238699719,-1.,-3.74449849461127));
#68442=CARTESIAN_POINT('Ctrl Pts',(-0.203054238699719,1.,-3.74449849461127));
#68443=CARTESIAN_POINT('',(-0.0760622897878238,1.,-4.19931119685982));
#68444=CARTESIAN_POINT('Ctrl Pts',(-0.0760622897878238,1.,-4.19931119685982));
#68445=CARTESIAN_POINT('Ctrl Pts',(-0.0767384596142197,1.,-4.19789138621624));
#68446=CARTESIAN_POINT('Ctrl Pts',(-0.0780873956244405,1.,-4.19505112860624));
#68447=CARTESIAN_POINT('Ctrl Pts',(-0.0801005887117605,1.,-4.19078883322483));
#68448=CARTESIAN_POINT('Ctrl Pts',(-0.0827644164389512,1.,-4.1851019532944));
#68449=CARTESIAN_POINT('Ctrl Pts',(-0.0860600915552517,1.,-4.17798698669991));
#68450=CARTESIAN_POINT('Ctrl Pts',(-0.089321556085033,1.,-4.17086566491823));
#68451=CARTESIAN_POINT('Ctrl Pts',(-0.0925486672167692,1.,-4.16373802265942));
#68452=CARTESIAN_POINT('Ctrl Pts',(-0.095741240329707,1.,-4.15660412653006));
#68453=CARTESIAN_POINT('Ctrl Pts',(-0.0988990478899814,1.,-4.1494640891762));
#68454=CARTESIAN_POINT('Ctrl Pts',(-0.102021826577454,1.,-4.14231804938737));
#68455=CARTESIAN_POINT('Ctrl Pts',(-0.105109286538864,1.,-4.13516614458396));
#68456=CARTESIAN_POINT('Ctrl Pts',(-0.10816112052835,1.,-4.12800848371386));
#68457=CARTESIAN_POINT('Ctrl Pts',(-0.111177012683377,1.,-4.12084512502444));
#68458=CARTESIAN_POINT('Ctrl Pts',(-0.114156649609602,1.,-4.11367603925313));
#68459=CARTESIAN_POINT('Ctrl Pts',(-0.117099722731705,1.,-4.10650113382187));
#68460=CARTESIAN_POINT('Ctrl Pts',(-0.120005924388162,1.,-4.09932031767243));
#68461=CARTESIAN_POINT('Ctrl Pts',(-0.122874946249119,1.,-4.09213355850836));
#68462=CARTESIAN_POINT('Ctrl Pts',(-0.125706476822529,1.,-4.08494093372315));
#68463=CARTESIAN_POINT('Ctrl Pts',(-0.128500200484814,1.,-4.07774270738809));
#68464=CARTESIAN_POINT('Ctrl Pts',(-0.131255793548914,1.,-4.07053931528579));
#68465=CARTESIAN_POINT('Ctrl Pts',(-0.133972916144225,1.,-4.06333121018476));
#68466=CARTESIAN_POINT('Ctrl Pts',(-0.136651205046111,1.,-4.05611873400122));
#68467=CARTESIAN_POINT('Ctrl Pts',(-0.13929026718006,1.,-4.04890199238056));
#68468=CARTESIAN_POINT('Ctrl Pts',(-0.141889671485508,1.,-4.04168069633842));
#68469=CARTESIAN_POINT('Ctrl Pts',(-0.144448947038352,1.,-4.03445411510403));
#68470=CARTESIAN_POINT('Ctrl Pts',(-0.146967602878999,1.,-4.02722143147048));
#68471=CARTESIAN_POINT('Ctrl Pts',(-0.149445144968708,1.,-4.01998203715588));
#68472=CARTESIAN_POINT('Ctrl Pts',(-0.151881094022909,1.,-4.01273584234684));
#68473=CARTESIAN_POINT('Ctrl Pts',(-0.15427500487231,1.,-4.00548360245297));
#68474=CARTESIAN_POINT('Ctrl Pts',(-0.156626481393736,1.,-3.99822717425869));
#68475=CARTESIAN_POINT('Ctrl Pts',(-0.158935123982796,1.,-3.99096873945862));
#68476=CARTESIAN_POINT('Ctrl Pts',(-0.161200482186088,1.,-3.98371010319866));
#68477=CARTESIAN_POINT('Ctrl Pts',(-0.163422004609999,1.,-3.97645194630944));
#68478=CARTESIAN_POINT('Ctrl Pts',(-0.165598992851098,1.,-3.9691931362141));
#68479=CARTESIAN_POINT('Ctrl Pts',(-0.167730547023312,1.,-3.96192990160296));
#68480=CARTESIAN_POINT('Ctrl Pts',(-0.16981566637413,1.,-3.95465744665263));
#68481=CARTESIAN_POINT('Ctrl Pts',(-0.171853355369233,1.,-3.94737164900861));
#68482=CARTESIAN_POINT('Ctrl Pts',(-0.173842734974607,1.,-3.94007083096214));
#68483=CARTESIAN_POINT('Ctrl Pts',(-0.175783136893873,1.,-3.93275726771049));
#68484=CARTESIAN_POINT('Ctrl Pts',(-0.177674246152328,1.,-3.92543942697672));
#68485=CARTESIAN_POINT('Ctrl Pts',(-0.179515885822895,1.,-3.91812876180948));
#68486=CARTESIAN_POINT('Ctrl Pts',(-0.181307740731796,1.,-3.91083557557193));
#68487=CARTESIAN_POINT('Ctrl Pts',(-0.183049081993193,1.,-3.90356488555138));
#68488=CARTESIAN_POINT('Ctrl Pts',(-0.184738537728035,1.,-3.89631300742633));
#68489=CARTESIAN_POINT('Ctrl Pts',(-0.186373724985263,1.,-3.88906196725817));
#68490=CARTESIAN_POINT('Ctrl Pts',(-0.187951632512663,1.,-3.88178563496187));
#68491=CARTESIAN_POINT('Ctrl Pts',(-0.189469253358254,1.,-3.87445976418377));
#68492=CARTESIAN_POINT('Ctrl Pts',(-0.190924190418613,1.,-3.8670715862477));
#68493=CARTESIAN_POINT('Ctrl Pts',(-0.19231515304498,1.,-3.85962774407652));
#68494=CARTESIAN_POINT('Ctrl Pts',(-0.193642806777748,1.,-3.85216762264019));
#68495=CARTESIAN_POINT('Ctrl Pts',(-0.194909009460255,1.,-3.84475203347052));
#68496=CARTESIAN_POINT('Ctrl Pts',(-0.19611519897189,1.,-3.83743910616265));
#68497=CARTESIAN_POINT('Ctrl Pts',(-0.197260935827375,1.,-3.83026221776488));
#68498=CARTESIAN_POINT('Ctrl Pts',(-0.19834261690047,1.,-3.82321127348981));
#68499=CARTESIAN_POINT('Ctrl Pts',(-0.199351525297396,1.,-3.81620203429702));
#68500=CARTESIAN_POINT('Ctrl Pts',(-0.20027467943329,1.,-3.80909529318501));
#68501=CARTESIAN_POINT('Ctrl Pts',(-0.201097756307252,1.,-3.80175247447171));
#68502=CARTESIAN_POINT('Ctrl Pts',(-0.201807533800799,1.,-3.79408354187274));
#68503=CARTESIAN_POINT('Ctrl Pts',(-0.202394260512193,1.,-3.78609175019317));
#68504=CARTESIAN_POINT('Ctrl Pts',(-0.202854729699197,1.,-3.77793553476879));
#68505=CARTESIAN_POINT('Ctrl Pts',(-0.203192390045337,1.,-3.76992071595267));
#68506=CARTESIAN_POINT('Ctrl Pts',(-0.203414634707646,1.,-3.76242717937273));
#68507=CARTESIAN_POINT('Ctrl Pts',(-0.203530796848404,1.,-3.75585118707924));
#68508=CARTESIAN_POINT('Ctrl Pts',(-0.203550035479097,1.,-3.75054693397716));
#68509=CARTESIAN_POINT('Ctrl Pts',(-0.203484186269315,1.,-3.74703926501843));
#68510=CARTESIAN_POINT('Ctrl Pts',(-0.203375226874331,1.,-3.74535749969262));
#68511=CARTESIAN_POINT('Ctrl Pts',(-0.203266610111264,1.,-3.74471097893961));
#68512=CARTESIAN_POINT('Ctrl Pts',(-0.203188003947965,1.,-3.74453008995129));
#68513=CARTESIAN_POINT('Ctrl Pts',(-0.203156094897896,1.,-3.74449296982994));
#68514=CARTESIAN_POINT('',(-0.0760622897878238,0.,-4.19931119685982));
#68515=CARTESIAN_POINT('Ctrl Pts',(0.20305423869972,-1.,-3.74449849461127));
#68516=CARTESIAN_POINT('Ctrl Pts',(0.20305423869972,1.,-3.74449849461127));
#68517=CARTESIAN_POINT('Ctrl Pts',(0.203111767587923,-1.,-3.7444331934681));
#68518=CARTESIAN_POINT('Ctrl Pts',(0.203111767587923,1.,-3.7444331934681));
#68519=CARTESIAN_POINT('Ctrl Pts',(0.203218215748058,-1.,-3.7444688019622));
#68520=CARTESIAN_POINT('Ctrl Pts',(0.203218215748058,1.,-3.7444688019622));
#68521=CARTESIAN_POINT('Ctrl Pts',(0.203352057956297,-1.,-3.74502080927395));
#68522=CARTESIAN_POINT('Ctrl Pts',(0.203352057956297,1.,-3.74502080927395));
#68523=CARTESIAN_POINT('Ctrl Pts',(0.203478844530447,-1.,-3.7467547201908));
#68524=CARTESIAN_POINT('Ctrl Pts',(0.203478844530447,1.,-3.7467547201908));
#68525=CARTESIAN_POINT('Ctrl Pts',(0.203550035479166,-1.,-3.75054693397875));
#68526=CARTESIAN_POINT('Ctrl Pts',(0.203550035479166,1.,-3.75054693397875));
#68527=CARTESIAN_POINT('Ctrl Pts',(0.203530796848321,-1.,-3.75585118707734));
#68528=CARTESIAN_POINT('Ctrl Pts',(0.203530796848321,1.,-3.75585118707734));
#68529=CARTESIAN_POINT('Ctrl Pts',(0.203414634707478,-1.,-3.76242717936885));
#68530=CARTESIAN_POINT('Ctrl Pts',(0.203414634707478,1.,-3.76242717936885));
#68531=CARTESIAN_POINT('Ctrl Pts',(0.203192390045164,-1.,-3.7699207159487));
#68532=CARTESIAN_POINT('Ctrl Pts',(0.203192390045164,1.,-3.7699207159487));
#68533=CARTESIAN_POINT('Ctrl Pts',(0.202854729699081,-1.,-3.77793553476614));
#68534=CARTESIAN_POINT('Ctrl Pts',(0.202854729699081,1.,-3.77793553476614));
#68535=CARTESIAN_POINT('Ctrl Pts',(0.20239426051216,-1.,-3.78609175019242));
#68536=CARTESIAN_POINT('Ctrl Pts',(0.20239426051216,1.,-3.78609175019242));
#68537=CARTESIAN_POINT('Ctrl Pts',(0.201807533800837,-1.,-3.7940835418736));
#68538=CARTESIAN_POINT('Ctrl Pts',(0.201807533800837,1.,-3.7940835418736));
#68539=CARTESIAN_POINT('Ctrl Pts',(0.201097756307326,-1.,-3.80175247447337));
#68540=CARTESIAN_POINT('Ctrl Pts',(0.201097756307326,1.,-3.80175247447337));
#68541=CARTESIAN_POINT('Ctrl Pts',(0.200274679433364,-1.,-3.80909529318669));
#68542=CARTESIAN_POINT('Ctrl Pts',(0.200274679433364,1.,-3.80909529318669));
#68543=CARTESIAN_POINT('Ctrl Pts',(0.199351525297447,-1.,-3.81620203429815));
#68544=CARTESIAN_POINT('Ctrl Pts',(0.199351525297447,1.,-3.81620203429815));
#68545=CARTESIAN_POINT('Ctrl Pts',(0.198342616900486,-1.,-3.82321127349016));
#68546=CARTESIAN_POINT('Ctrl Pts',(0.198342616900486,1.,-3.82321127349016));
#68547=CARTESIAN_POINT('Ctrl Pts',(0.197260935827361,-1.,-3.83026221776456));
#68548=CARTESIAN_POINT('Ctrl Pts',(0.197260935827361,1.,-3.83026221776456));
#68549=CARTESIAN_POINT('Ctrl Pts',(0.196115198971859,-1.,-3.83743910616195));
#68550=CARTESIAN_POINT('Ctrl Pts',(0.196115198971859,1.,-3.83743910616195));
#68551=CARTESIAN_POINT('Ctrl Pts',(0.19490900946022,-1.,-3.84475203346977));
#68552=CARTESIAN_POINT('Ctrl Pts',(0.19490900946022,1.,-3.84475203346977));
#68553=CARTESIAN_POINT('Ctrl Pts',(0.193642806777723,-1.,-3.85216762263966));
#68554=CARTESIAN_POINT('Ctrl Pts',(0.193642806777723,1.,-3.85216762263966));
#68555=CARTESIAN_POINT('Ctrl Pts',(0.19231515304497,-1.,-3.85962774407633));
#68556=CARTESIAN_POINT('Ctrl Pts',(0.19231515304497,1.,-3.85962774407633));
#68557=CARTESIAN_POINT('Ctrl Pts',(0.19092419041862,-1.,-3.86707158624783));
#68558=CARTESIAN_POINT('Ctrl Pts',(0.19092419041862,1.,-3.86707158624783));
#68559=CARTESIAN_POINT('Ctrl Pts',(0.189469253358272,-1.,-3.87445976418412));
#68560=CARTESIAN_POINT('Ctrl Pts',(0.189469253358272,1.,-3.87445976418412));
#68561=CARTESIAN_POINT('Ctrl Pts',(0.187951632512685,-1.,-3.88178563496228));
#68562=CARTESIAN_POINT('Ctrl Pts',(0.187951632512685,1.,-3.88178563496228));
#68563=CARTESIAN_POINT('Ctrl Pts',(0.18637372498528,-1.,-3.88906196725848));
#68564=CARTESIAN_POINT('Ctrl Pts',(0.18637372498528,1.,-3.88906196725848));
#68565=CARTESIAN_POINT('Ctrl Pts',(0.184738537728043,-1.,-3.89631300742646));
#68566=CARTESIAN_POINT('Ctrl Pts',(0.184738537728043,1.,-3.89631300742646));
#68567=CARTESIAN_POINT('Ctrl Pts',(0.18304908199319,-1.,-3.90356488555132));
#68568=CARTESIAN_POINT('Ctrl Pts',(0.18304908199319,1.,-3.90356488555132));
#68569=CARTESIAN_POINT('Ctrl Pts',(0.181307740731785,-1.,-3.91083557557175));
#68570=CARTESIAN_POINT('Ctrl Pts',(0.181307740731785,1.,-3.91083557557175));
#68571=CARTESIAN_POINT('Ctrl Pts',(0.179515885822881,-1.,-3.91812876180926));
#68572=CARTESIAN_POINT('Ctrl Pts',(0.179515885822881,1.,-3.91812876180926));
#68573=CARTESIAN_POINT('Ctrl Pts',(0.177674246152317,-1.,-3.92543942697655));
#68574=CARTESIAN_POINT('Ctrl Pts',(0.177674246152317,1.,-3.92543942697655));
#68575=CARTESIAN_POINT('Ctrl Pts',(0.175783136893868,-1.,-3.93275726771042));
#68576=CARTESIAN_POINT('Ctrl Pts',(0.175783136893868,1.,-3.93275726771042));
#68577=CARTESIAN_POINT('Ctrl Pts',(0.173842734974609,-1.,-3.94007083096217));
#68578=CARTESIAN_POINT('Ctrl Pts',(0.173842734974609,1.,-3.94007083096217));
#68579=CARTESIAN_POINT('Ctrl Pts',(0.17185335536924,-1.,-3.94737164900868));
#68580=CARTESIAN_POINT('Ctrl Pts',(0.17185335536924,1.,-3.94737164900868));
#68581=CARTESIAN_POINT('Ctrl Pts',(0.169815666374139,-1.,-3.95465744665268));
#68582=CARTESIAN_POINT('Ctrl Pts',(0.169815666374139,1.,-3.95465744665268));
#68583=CARTESIAN_POINT('Ctrl Pts',(0.167730547023319,-1.,-3.96192990160296));
#68584=CARTESIAN_POINT('Ctrl Pts',(0.167730547023319,1.,-3.96192990160296));
#68585=CARTESIAN_POINT('Ctrl Pts',(0.165598992851102,-1.,-3.96919313621407));
#68586=CARTESIAN_POINT('Ctrl Pts',(0.165598992851102,1.,-3.96919313621407));
#68587=CARTESIAN_POINT('Ctrl Pts',(0.163422004609999,-1.,-3.97645194630943));
#68588=CARTESIAN_POINT('Ctrl Pts',(0.163422004609999,1.,-3.97645194630943));
#68589=CARTESIAN_POINT('Ctrl Pts',(0.161200482186084,-1.,-3.98371010319872));
#68590=CARTESIAN_POINT('Ctrl Pts',(0.161200482186084,1.,-3.98371010319872));
#68591=CARTESIAN_POINT('Ctrl Pts',(0.158935123982793,-1.,-3.99096873945878));
#68592=CARTESIAN_POINT('Ctrl Pts',(0.158935123982793,1.,-3.99096873945878));
#68593=CARTESIAN_POINT('Ctrl Pts',(0.156626481393734,-1.,-3.99822717425893));
#68594=CARTESIAN_POINT('Ctrl Pts',(0.156626481393734,1.,-3.99822717425893));
#68595=CARTESIAN_POINT('Ctrl Pts',(0.15427500487231,-1.,-4.00548360245319));
#68596=CARTESIAN_POINT('Ctrl Pts',(0.15427500487231,1.,-4.00548360245319));
#68597=CARTESIAN_POINT('Ctrl Pts',(0.15188109402291,-1.,-4.01273584234689));
#68598=CARTESIAN_POINT('Ctrl Pts',(0.15188109402291,1.,-4.01273584234689));
#68599=CARTESIAN_POINT('Ctrl Pts',(0.149445144968707,-1.,-4.01998203715564));
#68600=CARTESIAN_POINT('Ctrl Pts',(0.149445144968707,1.,-4.01998203715564));
#68601=CARTESIAN_POINT('Ctrl Pts',(0.146967602878994,-1.,-4.02722143146994));
#68602=CARTESIAN_POINT('Ctrl Pts',(0.146967602878994,1.,-4.02722143146994));
#68603=CARTESIAN_POINT('Ctrl Pts',(0.144448947038344,-1.,-4.03445411510333));
#68604=CARTESIAN_POINT('Ctrl Pts',(0.144448947038344,1.,-4.03445411510333));
#68605=CARTESIAN_POINT('Ctrl Pts',(0.1418896714855,-1.,-4.04168069633781));
#68606=CARTESIAN_POINT('Ctrl Pts',(0.1418896714855,1.,-4.04168069633781));
#68607=CARTESIAN_POINT('Ctrl Pts',(0.139290267180057,-1.,-4.04890199238036));
#68608=CARTESIAN_POINT('Ctrl Pts',(0.139290267180057,1.,-4.04890199238036));
#68609=CARTESIAN_POINT('Ctrl Pts',(0.136651205046119,-1.,-4.05611873400172));
#68610=CARTESIAN_POINT('Ctrl Pts',(0.136651205046119,1.,-4.05611873400172));
#68611=CARTESIAN_POINT('Ctrl Pts',(0.133972916144245,-1.,-4.06333121018596));
#68612=CARTESIAN_POINT('Ctrl Pts',(0.133972916144245,1.,-4.06333121018596));
#68613=CARTESIAN_POINT('Ctrl Pts',(0.13125579354894,-1.,-4.0705393152874));
#68614=CARTESIAN_POINT('Ctrl Pts',(0.13125579354894,1.,-4.0705393152874));
#68615=CARTESIAN_POINT('Ctrl Pts',(0.128500200484837,-1.,-4.07774270738954));
#68616=CARTESIAN_POINT('Ctrl Pts',(0.128500200484837,1.,-4.07774270738954));
#68617=CARTESIAN_POINT('Ctrl Pts',(0.12570647682254,-1.,-4.08494093372377));
#68618=CARTESIAN_POINT('Ctrl Pts',(0.12570647682254,1.,-4.08494093372377));
#68619=CARTESIAN_POINT('Ctrl Pts',(0.122874946249107,-1.,-4.09213355850756));
#68620=CARTESIAN_POINT('Ctrl Pts',(0.122874946249107,1.,-4.09213355850756));
#68621=CARTESIAN_POINT('Ctrl Pts',(0.120005924388124,-1.,-4.09932031767002));
#68622=CARTESIAN_POINT('Ctrl Pts',(0.120005924388124,1.,-4.09932031767002));
#68623=CARTESIAN_POINT('Ctrl Pts',(0.117099722731648,-1.,-4.10650113381833));
#68624=CARTESIAN_POINT('Ctrl Pts',(0.117099722731648,1.,-4.10650113381833));
#68625=CARTESIAN_POINT('Ctrl Pts',(0.114156649609545,-1.,-4.11367603924961));
#68626=CARTESIAN_POINT('Ctrl Pts',(0.114156649609545,1.,-4.11367603924961));
#68627=CARTESIAN_POINT('Ctrl Pts',(0.111177012683346,-1.,-4.1208451250225));
#68628=CARTESIAN_POINT('Ctrl Pts',(0.111177012683346,1.,-4.1208451250225));
#68629=CARTESIAN_POINT('Ctrl Pts',(0.108161120528369,-1.,-4.12800848371504));
#68630=CARTESIAN_POINT('Ctrl Pts',(0.108161120528369,1.,-4.12800848371504));
#68631=CARTESIAN_POINT('Ctrl Pts',(0.105109286538945,-1.,-4.13516614458895));
#68632=CARTESIAN_POINT('Ctrl Pts',(0.105109286538945,1.,-4.13516614458895));
#68633=CARTESIAN_POINT('Ctrl Pts',(0.102021826577584,-1.,-4.14231804939538));
#68634=CARTESIAN_POINT('Ctrl Pts',(0.102021826577584,1.,-4.14231804939538));
#68635=CARTESIAN_POINT('Ctrl Pts',(0.0988990478901223,-1.,-4.14946408918485));
#68636=CARTESIAN_POINT('Ctrl Pts',(0.0988990478901223,1.,-4.14946408918485));
#68637=CARTESIAN_POINT('Ctrl Pts',(0.0957412403298004,-1.,-4.15660412653577));
#68638=CARTESIAN_POINT('Ctrl Pts',(0.0957412403298004,1.,-4.15660412653577));
#68639=CARTESIAN_POINT('Ctrl Pts',(0.0925486672167528,-1.,-4.16373802265839));
#68640=CARTESIAN_POINT('Ctrl Pts',(0.0925486672167528,1.,-4.16373802265839));
#68641=CARTESIAN_POINT('Ctrl Pts',(0.0893215560848647,-1.,-4.17086566490794));
#68642=CARTESIAN_POINT('Ctrl Pts',(0.0893215560848647,1.,-4.17086566490794));
#68643=CARTESIAN_POINT('Ctrl Pts',(0.0860600915549394,-1.,-4.17798698668094));
#68644=CARTESIAN_POINT('Ctrl Pts',(0.0860600915549394,1.,-4.17798698668094));
#68645=CARTESIAN_POINT('Ctrl Pts',(0.0827644164385676,-1.,-4.18510195327123));
#68646=CARTESIAN_POINT('Ctrl Pts',(0.0827644164385676,1.,-4.18510195327123));
#68647=CARTESIAN_POINT('Ctrl Pts',(0.0801005887114317,-1.,-4.19078883320504));
#68648=CARTESIAN_POINT('Ctrl Pts',(0.0801005887114317,1.,-4.19078883320504));
#68649=CARTESIAN_POINT('Ctrl Pts',(0.0780873956242395,-1.,-4.19505112859416));
#68650=CARTESIAN_POINT('Ctrl Pts',(0.0780873956242395,1.,-4.19505112859416));
#68651=CARTESIAN_POINT('Ctrl Pts',(0.0767384596141462,-1.,-4.1978913862118));
#68652=CARTESIAN_POINT('Ctrl Pts',(0.0767384596141462,1.,-4.1978913862118));
#68653=CARTESIAN_POINT('Ctrl Pts',(0.0760622897878244,-1.,-4.19931119685982));
#68654=CARTESIAN_POINT('Ctrl Pts',(0.0760622897878244,1.,-4.19931119685982));
#68655=CARTESIAN_POINT('',(0.203156094896102,1.,-3.74449296983004));
#68656=CARTESIAN_POINT('Ctrl Pts',(0.2031560948961,-1.,-3.74449296983004));
#68657=CARTESIAN_POINT('Ctrl Pts',(0.2031560948961,-0.666666666666667,-3.74449296983004));
#68658=CARTESIAN_POINT('Ctrl Pts',(0.2031560948961,-0.333333333333333,-3.74449296983004));
#68659=CARTESIAN_POINT('Ctrl Pts',(0.2031560948961,0.333333333333333,-3.74449296983004));
#68660=CARTESIAN_POINT('Ctrl Pts',(0.203156094896101,0.666666666666667,
-3.74449296983004));
#68661=CARTESIAN_POINT('Ctrl Pts',(0.203156094896101,1.,-3.74449296983004));
#68662=CARTESIAN_POINT('',(0.0760622897878244,1.,-4.19931119685982));
#68663=CARTESIAN_POINT('',(0.0760622897878244,0.,-4.19931119685982));
#68664=CARTESIAN_POINT('Ctrl Pts',(0.203156094896101,1.,-3.74449296983004));
#68665=CARTESIAN_POINT('Ctrl Pts',(0.203188003946657,1.,-3.74453008995093));
#68666=CARTESIAN_POINT('Ctrl Pts',(0.203266610110531,1.,-3.74471097893845));
#68667=CARTESIAN_POINT('Ctrl Pts',(0.203375226874121,1.,-3.74535749969115));
#68668=CARTESIAN_POINT('Ctrl Pts',(0.203484186269415,1.,-3.74703926501752));
#68669=CARTESIAN_POINT('Ctrl Pts',(0.203550035479166,1.,-3.75054693397875));
#68670=CARTESIAN_POINT('Ctrl Pts',(0.203530796848321,1.,-3.75585118707734));
#68671=CARTESIAN_POINT('Ctrl Pts',(0.203414634707478,1.,-3.76242717936885));
#68672=CARTESIAN_POINT('Ctrl Pts',(0.203192390045164,1.,-3.7699207159487));
#68673=CARTESIAN_POINT('Ctrl Pts',(0.202854729699081,1.,-3.77793553476614));
#68674=CARTESIAN_POINT('Ctrl Pts',(0.20239426051216,1.,-3.78609175019242));
#68675=CARTESIAN_POINT('Ctrl Pts',(0.201807533800837,1.,-3.7940835418736));
#68676=CARTESIAN_POINT('Ctrl Pts',(0.201097756307326,1.,-3.80175247447337));
#68677=CARTESIAN_POINT('Ctrl Pts',(0.200274679433364,1.,-3.80909529318669));
#68678=CARTESIAN_POINT('Ctrl Pts',(0.199351525297447,1.,-3.81620203429815));
#68679=CARTESIAN_POINT('Ctrl Pts',(0.198342616900486,1.,-3.82321127349016));
#68680=CARTESIAN_POINT('Ctrl Pts',(0.197260935827361,1.,-3.83026221776456));
#68681=CARTESIAN_POINT('Ctrl Pts',(0.196115198971859,1.,-3.83743910616195));
#68682=CARTESIAN_POINT('Ctrl Pts',(0.19490900946022,1.,-3.84475203346977));
#68683=CARTESIAN_POINT('Ctrl Pts',(0.193642806777723,1.,-3.85216762263966));
#68684=CARTESIAN_POINT('Ctrl Pts',(0.19231515304497,1.,-3.85962774407633));
#68685=CARTESIAN_POINT('Ctrl Pts',(0.19092419041862,1.,-3.86707158624783));
#68686=CARTESIAN_POINT('Ctrl Pts',(0.189469253358272,1.,-3.87445976418412));
#68687=CARTESIAN_POINT('Ctrl Pts',(0.187951632512685,1.,-3.88178563496228));
#68688=CARTESIAN_POINT('Ctrl Pts',(0.18637372498528,1.,-3.88906196725848));
#68689=CARTESIAN_POINT('Ctrl Pts',(0.184738537728043,1.,-3.89631300742646));
#68690=CARTESIAN_POINT('Ctrl Pts',(0.18304908199319,1.,-3.90356488555132));
#68691=CARTESIAN_POINT('Ctrl Pts',(0.181307740731785,1.,-3.91083557557175));
#68692=CARTESIAN_POINT('Ctrl Pts',(0.179515885822881,1.,-3.91812876180926));
#68693=CARTESIAN_POINT('Ctrl Pts',(0.177674246152317,1.,-3.92543942697655));
#68694=CARTESIAN_POINT('Ctrl Pts',(0.175783136893868,1.,-3.93275726771042));
#68695=CARTESIAN_POINT('Ctrl Pts',(0.173842734974609,1.,-3.94007083096217));
#68696=CARTESIAN_POINT('Ctrl Pts',(0.17185335536924,1.,-3.94737164900868));
#68697=CARTESIAN_POINT('Ctrl Pts',(0.169815666374139,1.,-3.95465744665268));
#68698=CARTESIAN_POINT('Ctrl Pts',(0.167730547023319,1.,-3.96192990160296));
#68699=CARTESIAN_POINT('Ctrl Pts',(0.165598992851102,1.,-3.96919313621407));
#68700=CARTESIAN_POINT('Ctrl Pts',(0.163422004609999,1.,-3.97645194630943));
#68701=CARTESIAN_POINT('Ctrl Pts',(0.161200482186084,1.,-3.98371010319872));
#68702=CARTESIAN_POINT('Ctrl Pts',(0.158935123982793,1.,-3.99096873945878));
#68703=CARTESIAN_POINT('Ctrl Pts',(0.156626481393734,1.,-3.99822717425893));
#68704=CARTESIAN_POINT('Ctrl Pts',(0.15427500487231,1.,-4.00548360245319));
#68705=CARTESIAN_POINT('Ctrl Pts',(0.15188109402291,1.,-4.01273584234689));
#68706=CARTESIAN_POINT('Ctrl Pts',(0.149445144968707,1.,-4.01998203715564));
#68707=CARTESIAN_POINT('Ctrl Pts',(0.146967602878994,1.,-4.02722143146994));
#68708=CARTESIAN_POINT('Ctrl Pts',(0.144448947038344,1.,-4.03445411510333));
#68709=CARTESIAN_POINT('Ctrl Pts',(0.1418896714855,1.,-4.04168069633781));
#68710=CARTESIAN_POINT('Ctrl Pts',(0.139290267180057,1.,-4.04890199238036));
#68711=CARTESIAN_POINT('Ctrl Pts',(0.136651205046119,1.,-4.05611873400172));
#68712=CARTESIAN_POINT('Ctrl Pts',(0.133972916144245,1.,-4.06333121018596));
#68713=CARTESIAN_POINT('Ctrl Pts',(0.13125579354894,1.,-4.0705393152874));
#68714=CARTESIAN_POINT('Ctrl Pts',(0.128500200484837,1.,-4.07774270738954));
#68715=CARTESIAN_POINT('Ctrl Pts',(0.12570647682254,1.,-4.08494093372377));
#68716=CARTESIAN_POINT('Ctrl Pts',(0.122874946249107,1.,-4.09213355850756));
#68717=CARTESIAN_POINT('Ctrl Pts',(0.120005924388124,1.,-4.09932031767002));
#68718=CARTESIAN_POINT('Ctrl Pts',(0.117099722731648,1.,-4.10650113381833));
#68719=CARTESIAN_POINT('Ctrl Pts',(0.114156649609545,1.,-4.11367603924961));
#68720=CARTESIAN_POINT('Ctrl Pts',(0.111177012683346,1.,-4.1208451250225));
#68721=CARTESIAN_POINT('Ctrl Pts',(0.108161120528369,1.,-4.12800848371504));
#68722=CARTESIAN_POINT('Ctrl Pts',(0.105109286538945,1.,-4.13516614458895));
#68723=CARTESIAN_POINT('Ctrl Pts',(0.102021826577584,1.,-4.14231804939538));
#68724=CARTESIAN_POINT('Ctrl Pts',(0.0988990478901223,1.,-4.14946408918485));
#68725=CARTESIAN_POINT('Ctrl Pts',(0.0957412403298004,1.,-4.15660412653577));
#68726=CARTESIAN_POINT('Ctrl Pts',(0.0925486672167528,1.,-4.16373802265839));
#68727=CARTESIAN_POINT('Ctrl Pts',(0.0893215560848647,1.,-4.17086566490794));
#68728=CARTESIAN_POINT('Ctrl Pts',(0.0860600915549394,1.,-4.17798698668094));
#68729=CARTESIAN_POINT('Ctrl Pts',(0.0827644164385676,1.,-4.18510195327123));
#68730=CARTESIAN_POINT('Ctrl Pts',(0.0801005887114317,1.,-4.19078883320504));
#68731=CARTESIAN_POINT('Ctrl Pts',(0.0780873956242395,1.,-4.19505112859416));
#68732=CARTESIAN_POINT('Ctrl Pts',(0.0767384596141462,1.,-4.1978913862118));
#68733=CARTESIAN_POINT('Ctrl Pts',(0.0760622897878244,1.,-4.19931119685982));
#68734=CARTESIAN_POINT('Origin',(0.0760622897878244,0.,-4.19931119685982));
#68735=CARTESIAN_POINT('',(-0.0760622897878238,1.,-4.19931119685982));
#68736=CARTESIAN_POINT('Origin',(0.,0.,0.));
#68737=CARTESIAN_POINT('',(0.385112848330761,1.,-3.73017266276651));
#68738=CARTESIAN_POINT('Origin',(0.,1.,0.));
#68739=CARTESIAN_POINT('Ctrl Pts',(0.385112848330762,1.,-3.73017266276651));
#68740=CARTESIAN_POINT('Ctrl Pts',(0.385112848330762,0.666666666666667,
-3.73017266276651));
#68741=CARTESIAN_POINT('Ctrl Pts',(0.385112848330762,0.333333333333333,
-3.73017266276651));
#68742=CARTESIAN_POINT('Ctrl Pts',(0.385112848330762,-0.333333333333333,
-3.73017266276651));
#68743=CARTESIAN_POINT('Ctrl Pts',(0.385112848330762,-0.666666666666667,
-3.73017266276651));
#68744=CARTESIAN_POINT('Ctrl Pts',(0.385112848330762,-1.,-3.73017266276651));
#68745=CARTESIAN_POINT('Ctrl Pts',(0.581791163835815,-1.,-4.15950947128175));
#68746=CARTESIAN_POINT('Ctrl Pts',(0.581791163835815,1.,-4.15950947128175));
#68747=CARTESIAN_POINT('Ctrl Pts',(0.580901211463535,-1.,-4.1582129171283));
#68748=CARTESIAN_POINT('Ctrl Pts',(0.580901211463535,1.,-4.1582129171283));
#68749=CARTESIAN_POINT('Ctrl Pts',(0.579124568914235,-1.,-4.15561864788576));
#68750=CARTESIAN_POINT('Ctrl Pts',(0.579124568914235,1.,-4.15561864788576));
#68751=CARTESIAN_POINT('Ctrl Pts',(0.576469391676688,-1.,-4.151723761217));
#68752=CARTESIAN_POINT('Ctrl Pts',(0.576469391676688,1.,-4.151723761217));
#68753=CARTESIAN_POINT('Ctrl Pts',(0.572948736069522,-1.,-4.14652361068081));
#68754=CARTESIAN_POINT('Ctrl Pts',(0.572948736069522,1.,-4.14652361068081));
#68755=CARTESIAN_POINT('Ctrl Pts',(0.568580610189774,-1.,-4.14001179830547));
#68756=CARTESIAN_POINT('Ctrl Pts',(0.568580610189774,1.,-4.14001179830547));
#68757=CARTESIAN_POINT('Ctrl Pts',(0.564245279537148,-1.,-4.13348835727104));
#68758=CARTESIAN_POINT('Ctrl Pts',(0.564245279537148,1.,-4.13348835727104));
#68759=CARTESIAN_POINT('Ctrl Pts',(0.559942890594773,-1.,-4.12695329951961));
#68760=CARTESIAN_POINT('Ctrl Pts',(0.559942890594773,1.,-4.12695329951961));
#68761=CARTESIAN_POINT('Ctrl Pts',(0.555673636129977,-1.,-4.12040666195664));
#68762=CARTESIAN_POINT('Ctrl Pts',(0.555673636129977,1.,-4.12040666195664));
#68763=CARTESIAN_POINT('Ctrl Pts',(0.551437758497032,-1.,-4.11384852024721));
#68764=CARTESIAN_POINT('Ctrl Pts',(0.551437758497032,1.,-4.11384852024721));
#68765=CARTESIAN_POINT('Ctrl Pts',(0.547235539485636,-1.,-4.10727897027977));
#68766=CARTESIAN_POINT('Ctrl Pts',(0.547235539485636,1.,-4.10727897027977));
#68767=CARTESIAN_POINT('Ctrl Pts',(0.543067286877757,-1.,-4.10069810243979));
#68768=CARTESIAN_POINT('Ctrl Pts',(0.543067286877757,1.,-4.10069810243979));
#68769=CARTESIAN_POINT('Ctrl Pts',(0.538933321179755,-1.,-4.09410597627));
#68770=CARTESIAN_POINT('Ctrl Pts',(0.538933321179755,1.,-4.09410597627));
#68771=CARTESIAN_POINT('Ctrl Pts',(0.534833963477273,-1.,-4.08750259988885));
#68772=CARTESIAN_POINT('Ctrl Pts',(0.534833963477273,1.,-4.08750259988885));
#68773=CARTESIAN_POINT('Ctrl Pts',(0.53076951872857,-1.,-4.08088789536836));
#68774=CARTESIAN_POINT('Ctrl Pts',(0.53076951872857,1.,-4.08088789536836));
#68775=CARTESIAN_POINT('Ctrl Pts',(0.526740277227498,-1.,-4.07426172299847));
#68776=CARTESIAN_POINT('Ctrl Pts',(0.526740277227498,1.,-4.07426172299847));
#68777=CARTESIAN_POINT('Ctrl Pts',(0.522746528603107,-1.,-4.06762394471314));
#68778=CARTESIAN_POINT('Ctrl Pts',(0.522746528603107,1.,-4.06762394471314));
#68779=CARTESIAN_POINT('Ctrl Pts',(0.518788572336923,-1.,-4.06097448038013));
#68780=CARTESIAN_POINT('Ctrl Pts',(0.518788572336923,1.,-4.06097448038013));
#68781=CARTESIAN_POINT('Ctrl Pts',(0.514866728193016,-1.,-4.05431335771199));
#68782=CARTESIAN_POINT('Ctrl Pts',(0.514866728193016,1.,-4.05431335771199));
#68783=CARTESIAN_POINT('Ctrl Pts',(0.51098134921897,-1.,-4.04764078815447));
#68784=CARTESIAN_POINT('Ctrl Pts',(0.51098134921897,1.,-4.04764078815447));
#68785=CARTESIAN_POINT('Ctrl Pts',(0.507132823288136,-1.,-4.04095715148915));
#68786=CARTESIAN_POINT('Ctrl Pts',(0.507132823288136,1.,-4.04095715148915));
#68787=CARTESIAN_POINT('Ctrl Pts',(0.503321556915346,-1.,-4.03426284174272));
#68788=CARTESIAN_POINT('Ctrl Pts',(0.503321556915346,1.,-4.03426284174272));
#68789=CARTESIAN_POINT('Ctrl Pts',(0.499547962340821,-1.,-4.02755813980101));
#68790=CARTESIAN_POINT('Ctrl Pts',(0.499547962340821,1.,-4.02755813980101));
#68791=CARTESIAN_POINT('Ctrl Pts',(0.495812444326251,-1.,-4.02084308851832));
#68792=CARTESIAN_POINT('Ctrl Pts',(0.495812444326251,1.,-4.02084308851832));
#68793=CARTESIAN_POINT('Ctrl Pts',(0.492115383418018,-1.,-4.01411733503546));
#68794=CARTESIAN_POINT('Ctrl Pts',(0.492115383418018,1.,-4.01411733503546));
#68795=CARTESIAN_POINT('Ctrl Pts',(0.488457130424633,-1.,-4.0073800839099));
#68796=CARTESIAN_POINT('Ctrl Pts',(0.488457130424633,1.,-4.0073800839099));
#68797=CARTESIAN_POINT('Ctrl Pts',(0.484838042421834,-1.,-4.00063045119288));
#68798=CARTESIAN_POINT('Ctrl Pts',(0.484838042421834,1.,-4.00063045119288));
#68799=CARTESIAN_POINT('Ctrl Pts',(0.481258512209675,-1.,-3.99386775880679));
#68800=CARTESIAN_POINT('Ctrl Pts',(0.481258512209675,1.,-3.99386775880679));
#68801=CARTESIAN_POINT('Ctrl Pts',(0.477718999122027,-1.,-3.98709184306738));
#68802=CARTESIAN_POINT('Ctrl Pts',(0.477718999122027,1.,-3.98709184306738));
#68803=CARTESIAN_POINT('Ctrl Pts',(0.474220061019509,-1.,-3.98030338044409));
#68804=CARTESIAN_POINT('Ctrl Pts',(0.474220061019509,1.,-3.98030338044409));
#68805=CARTESIAN_POINT('Ctrl Pts',(0.470762379613439,-1.,-3.97350414289392));
#68806=CARTESIAN_POINT('Ctrl Pts',(0.470762379613439,1.,-3.97350414289392));
#68807=CARTESIAN_POINT('Ctrl Pts',(0.467346690880643,-1.,-3.9666962227393));
#68808=CARTESIAN_POINT('Ctrl Pts',(0.467346690880643,1.,-3.9666962227393));
#68809=CARTESIAN_POINT('Ctrl Pts',(0.463973722115733,-1.,-3.95988133243538));
#68810=CARTESIAN_POINT('Ctrl Pts',(0.463973722115733,1.,-3.95988133243538));
#68811=CARTESIAN_POINT('Ctrl Pts',(0.460644124429121,-1.,-3.95306005817364));
#68812=CARTESIAN_POINT('Ctrl Pts',(0.460644124429121,1.,-3.95306005817364));
#68813=CARTESIAN_POINT('Ctrl Pts',(0.457358410451682,-1.,-3.94623117206678));
#68814=CARTESIAN_POINT('Ctrl Pts',(0.457358410451682,1.,-3.94623117206678));
#68815=CARTESIAN_POINT('Ctrl Pts',(0.454116879027584,-1.,-3.93939080846298));
#68816=CARTESIAN_POINT('Ctrl Pts',(0.454116879027584,1.,-3.93939080846298));
#68817=CARTESIAN_POINT('Ctrl Pts',(0.450919768356348,-1.,-3.93253407403123));
#68818=CARTESIAN_POINT('Ctrl Pts',(0.450919768356348,1.,-3.93253407403123));
#68819=CARTESIAN_POINT('Ctrl Pts',(0.447767416837292,-1.,-3.92565674143416));
#68820=CARTESIAN_POINT('Ctrl Pts',(0.447767416837292,1.,-3.92565674143416));
#68821=CARTESIAN_POINT('Ctrl Pts',(0.44466043023059,-1.,-3.91875701610719));
#68822=CARTESIAN_POINT('Ctrl Pts',(0.44466043023059,1.,-3.91875701610719));
#68823=CARTESIAN_POINT('Ctrl Pts',(0.441599824524054,-1.,-3.91183704069153));
#68824=CARTESIAN_POINT('Ctrl Pts',(0.441599824524054,1.,-3.91183704069153));
#68825=CARTESIAN_POINT('Ctrl Pts',(0.438587235458249,-1.,-3.90490512938563));
#68826=CARTESIAN_POINT('Ctrl Pts',(0.438587235458249,1.,-3.90490512938563));
#68827=CARTESIAN_POINT('Ctrl Pts',(0.435624629433527,-1.,-3.89797256655462));
#68828=CARTESIAN_POINT('Ctrl Pts',(0.435624629433527,1.,-3.89797256655462));
#68829=CARTESIAN_POINT('Ctrl Pts',(0.432713929544458,-1.,-3.89104947940611));
#68830=CARTESIAN_POINT('Ctrl Pts',(0.432713929544458,1.,-3.89104947940611));
#68831=CARTESIAN_POINT('Ctrl Pts',(0.429856640579741,-1.,-3.88414070943341));
#68832=CARTESIAN_POINT('Ctrl Pts',(0.429856640579741,1.,-3.88414070943341));
#68833=CARTESIAN_POINT('Ctrl Pts',(0.427053541173457,-1.,-3.87724240306597));
#68834=CARTESIAN_POINT('Ctrl Pts',(0.427053541173457,1.,-3.87724240306597));
#68835=CARTESIAN_POINT('Ctrl Pts',(0.42430417319511,-1.,-3.87033643487851));
#68836=CARTESIAN_POINT('Ctrl Pts',(0.42430417319511,1.,-3.87033643487851));
#68837=CARTESIAN_POINT('Ctrl Pts',(0.421607423177534,-1.,-3.86339652542709));
#68838=CARTESIAN_POINT('Ctrl Pts',(0.421607423177534,1.,-3.86339652542709));
#68839=CARTESIAN_POINT('Ctrl Pts',(0.418962468086773,-1.,-3.85639825647996));
#68840=CARTESIAN_POINT('Ctrl Pts',(0.418962468086773,1.,-3.85639825647996));
#68841=CARTESIAN_POINT('Ctrl Pts',(0.416369678052906,-1.,-3.84932864157497));
#68842=CARTESIAN_POINT('Ctrl Pts',(0.416369678052906,1.,-3.84932864157497));
#68843=CARTESIAN_POINT('Ctrl Pts',(0.413831367016748,-1.,-3.84219403994762));
#68844=CARTESIAN_POINT('Ctrl Pts',(0.413831367016748,1.,-3.84219403994762));
#68845=CARTESIAN_POINT('Ctrl Pts',(0.411353038798518,-1.,-3.83503345578698));
#68846=CARTESIAN_POINT('Ctrl Pts',(0.411353038798518,1.,-3.83503345578698));
#68847=CARTESIAN_POINT('Ctrl Pts',(0.408942371447459,-1.,-3.82790724256471));
#68848=CARTESIAN_POINT('Ctrl Pts',(0.408942371447459,1.,-3.82790724256471));
#68849=CARTESIAN_POINT('Ctrl Pts',(0.406607038258985,-1.,-3.8208730391381));
#68850=CARTESIAN_POINT('Ctrl Pts',(0.406607038258985,1.,-3.8208730391381));
#68851=CARTESIAN_POINT('Ctrl Pts',(0.404352694628273,-1.,-3.81396374287793));
#68852=CARTESIAN_POINT('Ctrl Pts',(0.404352694628273,1.,-3.81396374287793));
#68853=CARTESIAN_POINT('Ctrl Pts',(0.402181320148435,-1.,-3.80716881962728));
#68854=CARTESIAN_POINT('Ctrl Pts',(0.402181320148435,1.,-3.80716881962728));
#68855=CARTESIAN_POINT('Ctrl Pts',(0.4000883465046,-1.,-3.80040370384546));
#68856=CARTESIAN_POINT('Ctrl Pts',(0.4000883465046,1.,-3.80040370384546));
#68857=CARTESIAN_POINT('Ctrl Pts',(0.398064818683969,-1.,-3.7935288716329));
#68858=CARTESIAN_POINT('Ctrl Pts',(0.398064818683969,1.,-3.7935288716329));
#68859=CARTESIAN_POINT('Ctrl Pts',(0.39610320533484,-1.,-3.78640521279313));
#68860=CARTESIAN_POINT('Ctrl Pts',(0.39610320533484,1.,-3.78640521279313));
#68861=CARTESIAN_POINT('Ctrl Pts',(0.394202481011499,-1.,-3.77894173114283));
#68862=CARTESIAN_POINT('Ctrl Pts',(0.394202481011499,1.,-3.77894173114283));
#68863=CARTESIAN_POINT('Ctrl Pts',(0.392372786223432,-1.,-3.77114011595967));
#68864=CARTESIAN_POINT('Ctrl Pts',(0.392372786223432,1.,-3.77114011595967));
#68865=CARTESIAN_POINT('Ctrl Pts',(0.390642072979559,-1.,-3.76315635033257));
#68866=CARTESIAN_POINT('Ctrl Pts',(0.390642072979559,1.,-3.76315635033257));
#68867=CARTESIAN_POINT('Ctrl Pts',(0.389054775898701,-1.,-3.75529302895152));
#68868=CARTESIAN_POINT('Ctrl Pts',(0.389054775898701,1.,-3.75529302895152));
#68869=CARTESIAN_POINT('Ctrl Pts',(0.387663020050836,-1.,-3.74792651696654));
#68870=CARTESIAN_POINT('Ctrl Pts',(0.387663020050836,1.,-3.74792651696654));
#68871=CARTESIAN_POINT('Ctrl Pts',(0.386519576222251,-1.,-3.74144965781276));
#68872=CARTESIAN_POINT('Ctrl Pts',(0.386519576222251,1.,-3.74144965781276));
#68873=CARTESIAN_POINT('Ctrl Pts',(0.385670806454565,-1.,-3.73621371845318));
#68874=CARTESIAN_POINT('Ctrl Pts',(0.385670806454565,1.,-3.73621371845318));
#68875=CARTESIAN_POINT('Ctrl Pts',(0.385147887988951,-1.,-3.73245705638843));
#68876=CARTESIAN_POINT('Ctrl Pts',(0.385147887988951,1.,-3.73245705638843));
#68877=CARTESIAN_POINT('Ctrl Pts',(0.385001870183213,-1.,-3.73072465900175));
#68878=CARTESIAN_POINT('Ctrl Pts',(0.385001870183213,1.,-3.73072465900175));
#68879=CARTESIAN_POINT('Ctrl Pts',(0.385047711603462,-1.,-3.73015851028356));
#68880=CARTESIAN_POINT('Ctrl Pts',(0.385047711603462,1.,-3.73015851028356));
#68881=CARTESIAN_POINT('Ctrl Pts',(0.385147278814642,-1.,-3.73010668803042));
#68882=CARTESIAN_POINT('Ctrl Pts',(0.385147278814642,1.,-3.73010668803042));
#68883=CARTESIAN_POINT('Ctrl Pts',(0.385214314776329,-1.,-3.73016218570874));
#68884=CARTESIAN_POINT('Ctrl Pts',(0.385214314776329,1.,-3.73016218570874));
#68885=CARTESIAN_POINT('',(0.581791163835815,1.,-4.15950947128175));
#68886=CARTESIAN_POINT('Ctrl Pts',(0.581791163835815,1.,-4.15950947128175));
#68887=CARTESIAN_POINT('Ctrl Pts',(0.580901211463535,1.,-4.1582129171283));
#68888=CARTESIAN_POINT('Ctrl Pts',(0.579124568914235,1.,-4.15561864788576));
#68889=CARTESIAN_POINT('Ctrl Pts',(0.576469391676688,1.,-4.151723761217));
#68890=CARTESIAN_POINT('Ctrl Pts',(0.572948736069522,1.,-4.14652361068081));
#68891=CARTESIAN_POINT('Ctrl Pts',(0.568580610189774,1.,-4.14001179830547));
#68892=CARTESIAN_POINT('Ctrl Pts',(0.564245279537148,1.,-4.13348835727104));
#68893=CARTESIAN_POINT('Ctrl Pts',(0.559942890594773,1.,-4.12695329951961));
#68894=CARTESIAN_POINT('Ctrl Pts',(0.555673636129977,1.,-4.12040666195664));
#68895=CARTESIAN_POINT('Ctrl Pts',(0.551437758497032,1.,-4.11384852024721));
#68896=CARTESIAN_POINT('Ctrl Pts',(0.547235539485636,1.,-4.10727897027977));
#68897=CARTESIAN_POINT('Ctrl Pts',(0.543067286877757,1.,-4.10069810243979));
#68898=CARTESIAN_POINT('Ctrl Pts',(0.538933321179755,1.,-4.09410597627));
#68899=CARTESIAN_POINT('Ctrl Pts',(0.534833963477273,1.,-4.08750259988885));
#68900=CARTESIAN_POINT('Ctrl Pts',(0.53076951872857,1.,-4.08088789536836));
#68901=CARTESIAN_POINT('Ctrl Pts',(0.526740277227498,1.,-4.07426172299847));
#68902=CARTESIAN_POINT('Ctrl Pts',(0.522746528603107,1.,-4.06762394471314));
#68903=CARTESIAN_POINT('Ctrl Pts',(0.518788572336923,1.,-4.06097448038013));
#68904=CARTESIAN_POINT('Ctrl Pts',(0.514866728193016,1.,-4.05431335771199));
#68905=CARTESIAN_POINT('Ctrl Pts',(0.51098134921897,1.,-4.04764078815447));
#68906=CARTESIAN_POINT('Ctrl Pts',(0.507132823288136,1.,-4.04095715148915));
#68907=CARTESIAN_POINT('Ctrl Pts',(0.503321556915346,1.,-4.03426284174272));
#68908=CARTESIAN_POINT('Ctrl Pts',(0.499547962340821,1.,-4.02755813980101));
#68909=CARTESIAN_POINT('Ctrl Pts',(0.495812444326251,1.,-4.02084308851832));
#68910=CARTESIAN_POINT('Ctrl Pts',(0.492115383418018,1.,-4.01411733503546));
#68911=CARTESIAN_POINT('Ctrl Pts',(0.488457130424633,1.,-4.0073800839099));
#68912=CARTESIAN_POINT('Ctrl Pts',(0.484838042421834,1.,-4.00063045119288));
#68913=CARTESIAN_POINT('Ctrl Pts',(0.481258512209675,1.,-3.99386775880679));
#68914=CARTESIAN_POINT('Ctrl Pts',(0.477718999122027,1.,-3.98709184306738));
#68915=CARTESIAN_POINT('Ctrl Pts',(0.474220061019509,1.,-3.98030338044409));
#68916=CARTESIAN_POINT('Ctrl Pts',(0.470762379613439,1.,-3.97350414289392));
#68917=CARTESIAN_POINT('Ctrl Pts',(0.467346690880643,1.,-3.9666962227393));
#68918=CARTESIAN_POINT('Ctrl Pts',(0.463973722115733,1.,-3.95988133243538));
#68919=CARTESIAN_POINT('Ctrl Pts',(0.460644124429121,1.,-3.95306005817364));
#68920=CARTESIAN_POINT('Ctrl Pts',(0.457358410451682,1.,-3.94623117206678));
#68921=CARTESIAN_POINT('Ctrl Pts',(0.454116879027584,1.,-3.93939080846298));
#68922=CARTESIAN_POINT('Ctrl Pts',(0.450919768356348,1.,-3.93253407403123));
#68923=CARTESIAN_POINT('Ctrl Pts',(0.447767416837292,1.,-3.92565674143416));
#68924=CARTESIAN_POINT('Ctrl Pts',(0.44466043023059,1.,-3.91875701610719));
#68925=CARTESIAN_POINT('Ctrl Pts',(0.441599824524054,1.,-3.91183704069153));
#68926=CARTESIAN_POINT('Ctrl Pts',(0.438587235458249,1.,-3.90490512938563));
#68927=CARTESIAN_POINT('Ctrl Pts',(0.435624629433527,1.,-3.89797256655462));
#68928=CARTESIAN_POINT('Ctrl Pts',(0.432713929544458,1.,-3.89104947940611));
#68929=CARTESIAN_POINT('Ctrl Pts',(0.429856640579741,1.,-3.88414070943341));
#68930=CARTESIAN_POINT('Ctrl Pts',(0.427053541173457,1.,-3.87724240306597));
#68931=CARTESIAN_POINT('Ctrl Pts',(0.42430417319511,1.,-3.87033643487851));
#68932=CARTESIAN_POINT('Ctrl Pts',(0.421607423177534,1.,-3.86339652542709));
#68933=CARTESIAN_POINT('Ctrl Pts',(0.418962468086773,1.,-3.85639825647996));
#68934=CARTESIAN_POINT('Ctrl Pts',(0.416369678052906,1.,-3.84932864157497));
#68935=CARTESIAN_POINT('Ctrl Pts',(0.413831367016748,1.,-3.84219403994762));
#68936=CARTESIAN_POINT('Ctrl Pts',(0.411353038798518,1.,-3.83503345578698));
#68937=CARTESIAN_POINT('Ctrl Pts',(0.408942371447459,1.,-3.82790724256471));
#68938=CARTESIAN_POINT('Ctrl Pts',(0.406607038258985,1.,-3.8208730391381));
#68939=CARTESIAN_POINT('Ctrl Pts',(0.404352694628273,1.,-3.81396374287793));
#68940=CARTESIAN_POINT('Ctrl Pts',(0.402181320148435,1.,-3.80716881962728));
#68941=CARTESIAN_POINT('Ctrl Pts',(0.4000883465046,1.,-3.80040370384546));
#68942=CARTESIAN_POINT('Ctrl Pts',(0.398064818683969,1.,-3.7935288716329));
#68943=CARTESIAN_POINT('Ctrl Pts',(0.39610320533484,1.,-3.78640521279313));
#68944=CARTESIAN_POINT('Ctrl Pts',(0.394202481011499,1.,-3.77894173114283));
#68945=CARTESIAN_POINT('Ctrl Pts',(0.392372786223432,1.,-3.77114011595967));
#68946=CARTESIAN_POINT('Ctrl Pts',(0.390642072979559,1.,-3.76315635033257));
#68947=CARTESIAN_POINT('Ctrl Pts',(0.389054775898701,1.,-3.75529302895152));
#68948=CARTESIAN_POINT('Ctrl Pts',(0.387663020050836,1.,-3.74792651696654));
#68949=CARTESIAN_POINT('Ctrl Pts',(0.386519576222251,1.,-3.74144965781276));
#68950=CARTESIAN_POINT('Ctrl Pts',(0.385670806454565,1.,-3.73621371845318));
#68951=CARTESIAN_POINT('Ctrl Pts',(0.385187124634206,1.,-3.73273893363406));
#68952=CARTESIAN_POINT('Ctrl Pts',(0.385031656499163,1.,-3.73106082862548));
#68953=CARTESIAN_POINT('Ctrl Pts',(0.385037797881504,1.,-3.73040527621055));
#68954=CARTESIAN_POINT('Ctrl Pts',(0.385087139000374,1.,-3.73021431755274));
#68955=CARTESIAN_POINT('Ctrl Pts',(0.385112848330761,1.,-3.73017266276651));
#68956=CARTESIAN_POINT('',(0.581791163835815,0.,-4.15950947128175));
#68957=CARTESIAN_POINT('Ctrl Pts',(0.786322922920599,-1.,-3.66663282329846));
#68958=CARTESIAN_POINT('Ctrl Pts',(0.786322922920599,1.,-3.66663282329846));
#68959=CARTESIAN_POINT('Ctrl Pts',(0.786369528183326,-1.,-3.66655932661986));
#68960=CARTESIAN_POINT('Ctrl Pts',(0.786369528183326,1.,-3.66655932661986));
#68961=CARTESIAN_POINT('Ctrl Pts',(0.786480236185696,-1.,-3.66657784455334));
#68962=CARTESIAN_POINT('Ctrl Pts',(0.786480236185696,1.,-3.66657784455334));
#68963=CARTESIAN_POINT('Ctrl Pts',(0.786698783542764,-1.,-3.66710211820482));
#68964=CARTESIAN_POINT('Ctrl Pts',(0.786698783542764,1.,-3.66710211820482));
#68965=CARTESIAN_POINT('Ctrl Pts',(0.787095252590501,-1.,-3.66879484801113));
#68966=CARTESIAN_POINT('Ctrl Pts',(0.787095252590501,1.,-3.66879484801113));
#68967=CARTESIAN_POINT('Ctrl Pts',(0.787758799995742,-1.,-3.67252923663655));
#68968=CARTESIAN_POINT('Ctrl Pts',(0.787758799995742,1.,-3.67252923663655));
#68969=CARTESIAN_POINT('Ctrl Pts',(0.788569566220285,-1.,-3.67777119516252));
#68970=CARTESIAN_POINT('Ctrl Pts',(0.788569566220285,1.,-3.67777119516252));
#68971=CARTESIAN_POINT('Ctrl Pts',(0.789483546064386,-1.,-3.68428439783905));
#68972=CARTESIAN_POINT('Ctrl Pts',(0.789483546064386,1.,-3.68428439783905));
#68973=CARTESIAN_POINT('Ctrl Pts',(0.790436284988787,-1.,-3.69172044327364));
#68974=CARTESIAN_POINT('Ctrl Pts',(0.790436284988787,1.,-3.69172044327364));
#68975=CARTESIAN_POINT('Ctrl Pts',(0.79135657569598,-1.,-3.69968940808721));
#68976=CARTESIAN_POINT('Ctrl Pts',(0.79135657569598,1.,-3.69968940808721));
#68977=CARTESIAN_POINT('Ctrl Pts',(0.792177688845817,-1.,-3.70781724021806));
#68978=CARTESIAN_POINT('Ctrl Pts',(0.792177688845817,1.,-3.70781724021806));
#68979=CARTESIAN_POINT('Ctrl Pts',(0.792848377370287,-1.,-3.71580242396124));
#68980=CARTESIAN_POINT('Ctrl Pts',(0.792848377370287,1.,-3.71580242396124));
#68981=CARTESIAN_POINT('Ctrl Pts',(0.793347023784204,-1.,-3.72348797293734));
#68982=CARTESIAN_POINT('Ctrl Pts',(0.793347023784204,1.,-3.72348797293734));
#68983=CARTESIAN_POINT('Ctrl Pts',(0.793682750269684,-1.,-3.73086914695805));
#68984=CARTESIAN_POINT('Ctrl Pts',(0.793682750269684,1.,-3.73086914695805));
#68985=CARTESIAN_POINT('Ctrl Pts',(0.793882700937016,-1.,-3.73803280541687));
#68986=CARTESIAN_POINT('Ctrl Pts',(0.793882700937016,1.,-3.73803280541687));
#68987=CARTESIAN_POINT('Ctrl Pts',(0.793982700459951,-1.,-3.74511357728861));
#68988=CARTESIAN_POINT('Ctrl Pts',(0.793982700459951,1.,-3.74511357728861));
#68989=CARTESIAN_POINT('Ctrl Pts',(0.794017347371377,-1.,-3.75224692493864));
#68990=CARTESIAN_POINT('Ctrl Pts',(0.794017347371377,1.,-3.75224692493864));
#68991=CARTESIAN_POINT('Ctrl Pts',(0.794008429134907,-1.,-3.75951468666257));
#68992=CARTESIAN_POINT('Ctrl Pts',(0.794008429134907,1.,-3.75951468666257));
#68993=CARTESIAN_POINT('Ctrl Pts',(0.793961083688991,-1.,-3.76692626931111));
#68994=CARTESIAN_POINT('Ctrl Pts',(0.793961083688991,1.,-3.76692626931111));
#68995=CARTESIAN_POINT('Ctrl Pts',(0.793870523787407,-1.,-3.77444863801212));
#68996=CARTESIAN_POINT('Ctrl Pts',(0.793870523787407,1.,-3.77444863801212));
#68997=CARTESIAN_POINT('Ctrl Pts',(0.7937262357813,-1.,-3.78202460377598));
#68998=CARTESIAN_POINT('Ctrl Pts',(0.7937262357813,1.,-3.78202460377598));
#68999=CARTESIAN_POINT('Ctrl Pts',(0.793516871680993,-1.,-3.78959439439235));
#69000=CARTESIAN_POINT('Ctrl Pts',(0.793516871680993,1.,-3.78959439439235));
#69001=CARTESIAN_POINT('Ctrl Pts',(0.793235612973273,-1.,-3.79711921389897));
#69002=CARTESIAN_POINT('Ctrl Pts',(0.793235612973273,1.,-3.79711921389897));
#69003=CARTESIAN_POINT('Ctrl Pts',(0.792882695234777,-1.,-3.80459229925637));
#69004=CARTESIAN_POINT('Ctrl Pts',(0.792882695234777,1.,-3.80459229925637));
#69005=CARTESIAN_POINT('Ctrl Pts',(0.792462483517634,-1.,-3.81202588694756));
#69006=CARTESIAN_POINT('Ctrl Pts',(0.792462483517634,1.,-3.81202588694756));
#69007=CARTESIAN_POINT('Ctrl Pts',(0.791981740718634,-1.,-3.81944345442249));
#69008=CARTESIAN_POINT('Ctrl Pts',(0.791981740718634,1.,-3.81944345442249));
#69009=CARTESIAN_POINT('Ctrl Pts',(0.791447528662369,-1.,-3.82687033899792));
#69010=CARTESIAN_POINT('Ctrl Pts',(0.791447528662369,1.,-3.82687033899792));
#69011=CARTESIAN_POINT('Ctrl Pts',(0.7908650127053,-1.,-3.83432392054786));
#69012=CARTESIAN_POINT('Ctrl Pts',(0.7908650127053,1.,-3.83432392054786));
#69013=CARTESIAN_POINT('Ctrl Pts',(0.790236124191242,-1.,-3.84180762342454));
#69014=CARTESIAN_POINT('Ctrl Pts',(0.790236124191242,1.,-3.84180762342454));
#69015=CARTESIAN_POINT('Ctrl Pts',(0.789560798155582,-1.,-3.84931637808894));
#69016=CARTESIAN_POINT('Ctrl Pts',(0.789560798155582,1.,-3.84931637808894));
#69017=CARTESIAN_POINT('Ctrl Pts',(0.788837734090671,-1.,-3.85683995872529));
#69018=CARTESIAN_POINT('Ctrl Pts',(0.788837734090671,1.,-3.85683995872529));
#69019=CARTESIAN_POINT('Ctrl Pts',(0.788065315093777,-1.,-3.86436702561345));
#69020=CARTESIAN_POINT('Ctrl Pts',(0.788065315093777,1.,-3.86436702561345));
#69021=CARTESIAN_POINT('Ctrl Pts',(0.787242527617999,-1.,-3.87188916600912));
#69022=CARTESIAN_POINT('Ctrl Pts',(0.787242527617999,1.,-3.87188916600912));
#69023=CARTESIAN_POINT('Ctrl Pts',(0.786369675812608,-1.,-3.8794040281819));
#69024=CARTESIAN_POINT('Ctrl Pts',(0.786369675812608,1.,-3.8794040281819));
#69025=CARTESIAN_POINT('Ctrl Pts',(0.78544789034073,-1.,-3.88691313167398));
#69026=CARTESIAN_POINT('Ctrl Pts',(0.78544789034073,1.,-3.88691313167398));
#69027=CARTESIAN_POINT('Ctrl Pts',(0.784478799358336,-1.,-3.89442039235103));
#69028=CARTESIAN_POINT('Ctrl Pts',(0.784478799358336,1.,-3.89442039235103));
#69029=CARTESIAN_POINT('Ctrl Pts',(0.783464141529081,-1.,-3.9019303904397));
#69030=CARTESIAN_POINT('Ctrl Pts',(0.783464141529081,1.,-3.9019303904397));
#69031=CARTESIAN_POINT('Ctrl Pts',(0.782405395622764,-1.,-3.90944671004542));
#69032=CARTESIAN_POINT('Ctrl Pts',(0.782405395622764,1.,-3.90944671004542));
#69033=CARTESIAN_POINT('Ctrl Pts',(0.781303428618366,-1.,-3.91697036054676));
#69034=CARTESIAN_POINT('Ctrl Pts',(0.781303428618366,1.,-3.91697036054676));
#69035=CARTESIAN_POINT('Ctrl Pts',(0.780158678615542,-1.,-3.92450058323823));
#69036=CARTESIAN_POINT('Ctrl Pts',(0.780158678615542,1.,-3.92450058323823));
#69037=CARTESIAN_POINT('Ctrl Pts',(0.77897130813482,-1.,-3.93203552473174));
#69038=CARTESIAN_POINT('Ctrl Pts',(0.77897130813482,1.,-3.93203552473174));
#69039=CARTESIAN_POINT('Ctrl Pts',(0.777741370568558,-1.,-3.93957296768103));
#69040=CARTESIAN_POINT('Ctrl Pts',(0.777741370568558,1.,-3.93957296768103));
#69041=CARTESIAN_POINT('Ctrl Pts',(0.776468966697921,-1.,-3.94711101619447));
#69042=CARTESIAN_POINT('Ctrl Pts',(0.776468966697921,1.,-3.94711101619447));
#69043=CARTESIAN_POINT('Ctrl Pts',(0.775154418039351,-1.,-3.9546488545231));
#69044=CARTESIAN_POINT('Ctrl Pts',(0.775154418039351,1.,-3.9546488545231));
#69045=CARTESIAN_POINT('Ctrl Pts',(0.773798212026565,-1.,-3.96218649639807));
#69046=CARTESIAN_POINT('Ctrl Pts',(0.773798212026565,1.,-3.96218649639807));
#69047=CARTESIAN_POINT('Ctrl Pts',(0.772400931772136,-1.,-3.96972446532772));
#69048=CARTESIAN_POINT('Ctrl Pts',(0.772400931772136,1.,-3.96972446532772));
#69049=CARTESIAN_POINT('Ctrl Pts',(0.77096319003047,-1.,-3.97726349165488));
#69050=CARTESIAN_POINT('Ctrl Pts',(0.77096319003047,1.,-3.97726349165488));
#69051=CARTESIAN_POINT('Ctrl Pts',(0.769485566245544,-1.,-3.98480422348451));
#69052=CARTESIAN_POINT('Ctrl Pts',(0.769485566245544,1.,-3.98480422348451));
#69053=CARTESIAN_POINT('Ctrl Pts',(0.767968531377914,-1.,-3.9923468788101));
#69054=CARTESIAN_POINT('Ctrl Pts',(0.767968531377914,1.,-3.9923468788101));
#69055=CARTESIAN_POINT('Ctrl Pts',(0.766412457136063,-1.,-3.99989129179622));
#69056=CARTESIAN_POINT('Ctrl Pts',(0.766412457136063,1.,-3.99989129179622));
#69057=CARTESIAN_POINT('Ctrl Pts',(0.764817648785197,-1.,-4.00743706791509));
#69058=CARTESIAN_POINT('Ctrl Pts',(0.764817648785197,1.,-4.00743706791509));
#69059=CARTESIAN_POINT('Ctrl Pts',(0.763184371182935,-1.,-4.01498370680496));
#69060=CARTESIAN_POINT('Ctrl Pts',(0.763184371182935,1.,-4.01498370680496));
#69061=CARTESIAN_POINT('Ctrl Pts',(0.761512875859804,-1.,-4.02253072741268));
#69062=CARTESIAN_POINT('Ctrl Pts',(0.761512875859804,1.,-4.02253072741268));
#69063=CARTESIAN_POINT('Ctrl Pts',(0.759803433243751,-1.,-4.03007781954412));
#69064=CARTESIAN_POINT('Ctrl Pts',(0.759803433243751,1.,-4.03007781954412));
#69065=CARTESIAN_POINT('Ctrl Pts',(0.758056338884944,-1.,-4.03762485803119));
#69066=CARTESIAN_POINT('Ctrl Pts',(0.758056338884944,1.,-4.03762485803119));
#69067=CARTESIAN_POINT('Ctrl Pts',(0.75627190236958,-1.,-4.04517182653997));
#69068=CARTESIAN_POINT('Ctrl Pts',(0.75627190236958,1.,-4.04517182653997));
#69069=CARTESIAN_POINT('Ctrl Pts',(0.754450441816078,-1.,-4.05271876687915));
#69070=CARTESIAN_POINT('Ctrl Pts',(0.754450441816078,1.,-4.05271876687915));
#69071=CARTESIAN_POINT('Ctrl Pts',(0.752592276483072,-1.,-4.06026572221515));
#69072=CARTESIAN_POINT('Ctrl Pts',(0.752592276483072,1.,-4.06026572221515));
#69073=CARTESIAN_POINT('Ctrl Pts',(0.750697720484036,-1.,-4.06781267242378));
#69074=CARTESIAN_POINT('Ctrl Pts',(0.750697720484036,1.,-4.06781267242378));
#69075=CARTESIAN_POINT('Ctrl Pts',(0.748767076680557,-1.,-4.07535951056152));
#69076=CARTESIAN_POINT('Ctrl Pts',(0.748767076680557,1.,-4.07535951056152));
#69077=CARTESIAN_POINT('Ctrl Pts',(0.746800631492315,-1.,-4.08290608095642));
#69078=CARTESIAN_POINT('Ctrl Pts',(0.746800631492315,1.,-4.08290608095642));
#69079=CARTESIAN_POINT('Ctrl Pts',(0.7447986497065,-1.,-4.09045220253573));
#69080=CARTESIAN_POINT('Ctrl Pts',(0.7447986497065,1.,-4.09045220253573));
#69081=CARTESIAN_POINT('Ctrl Pts',(0.742761369689841,-1.,-4.09799769702611));
#69082=CARTESIAN_POINT('Ctrl Pts',(0.742761369689841,1.,-4.09799769702611));
#69083=CARTESIAN_POINT('Ctrl Pts',(0.740688998553376,-1.,-4.10554241757547));
#69084=CARTESIAN_POINT('Ctrl Pts',(0.740688998553376,1.,-4.10554241757547));
#69085=CARTESIAN_POINT('Ctrl Pts',(0.738581708225843,-1.,-4.11308626951927));
#69086=CARTESIAN_POINT('Ctrl Pts',(0.738581708225843,1.,-4.11308626951927));
#69087=CARTESIAN_POINT('Ctrl Pts',(0.736439634331344,-1.,-4.120629196238));
#69088=CARTESIAN_POINT('Ctrl Pts',(0.736439634331344,1.,-4.120629196238));
#69089=CARTESIAN_POINT('Ctrl Pts',(0.734698226764092,-1.,-4.12666277570844));
#69090=CARTESIAN_POINT('Ctrl Pts',(0.734698226764092,1.,-4.12666277570844));
#69091=CARTESIAN_POINT('Ctrl Pts',(0.733376589323546,-1.,-4.13118752795207));
#69092=CARTESIAN_POINT('Ctrl Pts',(0.733376589323546,1.,-4.13118752795207));
#69093=CARTESIAN_POINT('Ctrl Pts',(0.732488575135159,-1.,-4.1342038373684));
#69094=CARTESIAN_POINT('Ctrl Pts',(0.732488575135159,1.,-4.1342038373684));
#69095=CARTESIAN_POINT('Ctrl Pts',(0.73204283740062,-1.,-4.13571194405636));
#69096=CARTESIAN_POINT('Ctrl Pts',(0.73204283740062,1.,-4.13571194405636));
#69097=CARTESIAN_POINT('',(0.786422660831986,1.,-3.66661143271685));
#69098=CARTESIAN_POINT('Ctrl Pts',(0.786422660831985,-1.,-3.66661143271685));
#69099=CARTESIAN_POINT('Ctrl Pts',(0.786422660831985,-0.666666666666667,
-3.66661143271685));
#69100=CARTESIAN_POINT('Ctrl Pts',(0.786422660831985,-0.333333333333333,
-3.66661143271685));
#69101=CARTESIAN_POINT('Ctrl Pts',(0.786422660831985,0.333333333333333,
-3.66661143271685));
#69102=CARTESIAN_POINT('Ctrl Pts',(0.786422660831985,0.666666666666667,
-3.66661143271685));
#69103=CARTESIAN_POINT('Ctrl Pts',(0.786422660831985,1.,-3.66661143271685));
#69104=CARTESIAN_POINT('',(0.73204283740062,1.,-4.13571194405636));
#69105=CARTESIAN_POINT('',(0.73204283740062,0.,-4.13571194405636));
#69106=CARTESIAN_POINT('Ctrl Pts',(0.786422660831986,1.,-3.66661143271685));
#69107=CARTESIAN_POINT('Ctrl Pts',(0.786459983895432,1.,-3.6666431041522));
#69108=CARTESIAN_POINT('Ctrl Pts',(0.786565919558984,1.,-3.66680946938293));
#69109=CARTESIAN_POINT('Ctrl Pts',(0.786774337198062,1.,-3.66743103898702));
#69110=CARTESIAN_POINT('Ctrl Pts',(0.787145041181546,1.,-3.66907505398677));
#69111=CARTESIAN_POINT('Ctrl Pts',(0.787758799995742,1.,-3.67252923663655));
#69112=CARTESIAN_POINT('Ctrl Pts',(0.788569566220285,1.,-3.67777119516252));
#69113=CARTESIAN_POINT('Ctrl Pts',(0.789483546064386,1.,-3.68428439783905));
#69114=CARTESIAN_POINT('Ctrl Pts',(0.790436284988787,1.,-3.69172044327364));
#69115=CARTESIAN_POINT('Ctrl Pts',(0.79135657569598,1.,-3.69968940808721));
#69116=CARTESIAN_POINT('Ctrl Pts',(0.792177688845817,1.,-3.70781724021806));
#69117=CARTESIAN_POINT('Ctrl Pts',(0.792848377370287,1.,-3.71580242396124));
#69118=CARTESIAN_POINT('Ctrl Pts',(0.793347023784204,1.,-3.72348797293734));
#69119=CARTESIAN_POINT('Ctrl Pts',(0.793682750269684,1.,-3.73086914695805));
#69120=CARTESIAN_POINT('Ctrl Pts',(0.793882700937016,1.,-3.73803280541687));
#69121=CARTESIAN_POINT('Ctrl Pts',(0.793982700459951,1.,-3.74511357728861));
#69122=CARTESIAN_POINT('Ctrl Pts',(0.794017347371377,1.,-3.75224692493864));
#69123=CARTESIAN_POINT('Ctrl Pts',(0.794008429134907,1.,-3.75951468666257));
#69124=CARTESIAN_POINT('Ctrl Pts',(0.793961083688991,1.,-3.76692626931111));
#69125=CARTESIAN_POINT('Ctrl Pts',(0.793870523787407,1.,-3.77444863801212));
#69126=CARTESIAN_POINT('Ctrl Pts',(0.7937262357813,1.,-3.78202460377598));
#69127=CARTESIAN_POINT('Ctrl Pts',(0.793516871680993,1.,-3.78959439439235));
#69128=CARTESIAN_POINT('Ctrl Pts',(0.793235612973273,1.,-3.79711921389897));
#69129=CARTESIAN_POINT('Ctrl Pts',(0.792882695234777,1.,-3.80459229925637));
#69130=CARTESIAN_POINT('Ctrl Pts',(0.792462483517634,1.,-3.81202588694756));
#69131=CARTESIAN_POINT('Ctrl Pts',(0.791981740718634,1.,-3.81944345442249));
#69132=CARTESIAN_POINT('Ctrl Pts',(0.791447528662369,1.,-3.82687033899792));
#69133=CARTESIAN_POINT('Ctrl Pts',(0.7908650127053,1.,-3.83432392054786));
#69134=CARTESIAN_POINT('Ctrl Pts',(0.790236124191242,1.,-3.84180762342454));
#69135=CARTESIAN_POINT('Ctrl Pts',(0.789560798155582,1.,-3.84931637808894));
#69136=CARTESIAN_POINT('Ctrl Pts',(0.788837734090671,1.,-3.85683995872529));
#69137=CARTESIAN_POINT('Ctrl Pts',(0.788065315093777,1.,-3.86436702561345));
#69138=CARTESIAN_POINT('Ctrl Pts',(0.787242527617999,1.,-3.87188916600912));
#69139=CARTESIAN_POINT('Ctrl Pts',(0.786369675812608,1.,-3.8794040281819));
#69140=CARTESIAN_POINT('Ctrl Pts',(0.78544789034073,1.,-3.88691313167398));
#69141=CARTESIAN_POINT('Ctrl Pts',(0.784478799358336,1.,-3.89442039235103));
#69142=CARTESIAN_POINT('Ctrl Pts',(0.783464141529081,1.,-3.9019303904397));
#69143=CARTESIAN_POINT('Ctrl Pts',(0.782405395622764,1.,-3.90944671004542));
#69144=CARTESIAN_POINT('Ctrl Pts',(0.781303428618366,1.,-3.91697036054676));
#69145=CARTESIAN_POINT('Ctrl Pts',(0.780158678615542,1.,-3.92450058323823));
#69146=CARTESIAN_POINT('Ctrl Pts',(0.77897130813482,1.,-3.93203552473174));
#69147=CARTESIAN_POINT('Ctrl Pts',(0.777741370568558,1.,-3.93957296768103));
#69148=CARTESIAN_POINT('Ctrl Pts',(0.776468966697921,1.,-3.94711101619447));
#69149=CARTESIAN_POINT('Ctrl Pts',(0.775154418039351,1.,-3.9546488545231));
#69150=CARTESIAN_POINT('Ctrl Pts',(0.773798212026565,1.,-3.96218649639807));
#69151=CARTESIAN_POINT('Ctrl Pts',(0.772400931772136,1.,-3.96972446532772));
#69152=CARTESIAN_POINT('Ctrl Pts',(0.77096319003047,1.,-3.97726349165488));
#69153=CARTESIAN_POINT('Ctrl Pts',(0.769485566245544,1.,-3.98480422348451));
#69154=CARTESIAN_POINT('Ctrl Pts',(0.767968531377914,1.,-3.9923468788101));
#69155=CARTESIAN_POINT('Ctrl Pts',(0.766412457136063,1.,-3.99989129179622));
#69156=CARTESIAN_POINT('Ctrl Pts',(0.764817648785197,1.,-4.00743706791509));
#69157=CARTESIAN_POINT('Ctrl Pts',(0.763184371182935,1.,-4.01498370680496));
#69158=CARTESIAN_POINT('Ctrl Pts',(0.761512875859804,1.,-4.02253072741268));
#69159=CARTESIAN_POINT('Ctrl Pts',(0.759803433243751,1.,-4.03007781954412));
#69160=CARTESIAN_POINT('Ctrl Pts',(0.758056338884944,1.,-4.03762485803119));
#69161=CARTESIAN_POINT('Ctrl Pts',(0.75627190236958,1.,-4.04517182653997));
#69162=CARTESIAN_POINT('Ctrl Pts',(0.754450441816078,1.,-4.05271876687915));
#69163=CARTESIAN_POINT('Ctrl Pts',(0.752592276483072,1.,-4.06026572221515));
#69164=CARTESIAN_POINT('Ctrl Pts',(0.750697720484036,1.,-4.06781267242378));
#69165=CARTESIAN_POINT('Ctrl Pts',(0.748767076680557,1.,-4.07535951056152));
#69166=CARTESIAN_POINT('Ctrl Pts',(0.746800631492315,1.,-4.08290608095642));
#69167=CARTESIAN_POINT('Ctrl Pts',(0.7447986497065,1.,-4.09045220253573));
#69168=CARTESIAN_POINT('Ctrl Pts',(0.742761369689841,1.,-4.09799769702611));
#69169=CARTESIAN_POINT('Ctrl Pts',(0.740688998553376,1.,-4.10554241757547));
#69170=CARTESIAN_POINT('Ctrl Pts',(0.738581708225843,1.,-4.11308626951927));
#69171=CARTESIAN_POINT('Ctrl Pts',(0.736439634331344,1.,-4.120629196238));
#69172=CARTESIAN_POINT('Ctrl Pts',(0.734698226764092,1.,-4.12666277570844));
#69173=CARTESIAN_POINT('Ctrl Pts',(0.733376589323546,1.,-4.13118752795207));
#69174=CARTESIAN_POINT('Ctrl Pts',(0.732488575135159,1.,-4.1342038373684));
#69175=CARTESIAN_POINT('Ctrl Pts',(0.73204283740062,1.,-4.13571194405636));
#69176=CARTESIAN_POINT('Origin',(0.73204283740062,0.,-4.13571194405636));
#69177=CARTESIAN_POINT('',(0.581791163835815,1.,-4.15950947128175));
#69178=CARTESIAN_POINT('Origin',(0.,0.,0.));
#69179=CARTESIAN_POINT('',(0.963899035117248,1.,-3.62400312501245));
#69180=CARTESIAN_POINT('Origin',(0.,1.,0.));
#69181=CARTESIAN_POINT('Ctrl Pts',(0.963899035117248,1.,-3.62400312501246));
#69182=CARTESIAN_POINT('Ctrl Pts',(0.963899035117248,0.666666666666667,
-3.62400312501246));
#69183=CARTESIAN_POINT('Ctrl Pts',(0.963899035117248,0.333333333333333,
-3.62400312501246));
#69184=CARTESIAN_POINT('Ctrl Pts',(0.963899035117248,-0.333333333333333,
-3.62400312501246));
#69185=CARTESIAN_POINT('Ctrl Pts',(0.963899035117249,-0.666666666666667,
-3.62400312501246));
#69186=CARTESIAN_POINT('Ctrl Pts',(0.963899035117249,-1.,-3.62400312501246));
#69187=CARTESIAN_POINT('Ctrl Pts',(1.22531898815164,-1.,-4.01728681790024));
#69188=CARTESIAN_POINT('Ctrl Pts',(1.22531898815164,1.,-4.01728681790024));
#69189=CARTESIAN_POINT('Ctrl Pts',(1.22423716681447,-1.,-4.0161454457032));
#69190=CARTESIAN_POINT('Ctrl Pts',(1.22423716681447,1.,-4.0161454457032));
#69191=CARTESIAN_POINT('Ctrl Pts',(1.22207656456199,-1.,-4.01386104434674));
#69192=CARTESIAN_POINT('Ctrl Pts',(1.22207656456199,1.,-4.01386104434674));
#69193=CARTESIAN_POINT('Ctrl Pts',(1.21884478244983,-1.,-4.01042947142681));
#69194=CARTESIAN_POINT('Ctrl Pts',(1.21884478244983,1.,-4.01042947142681));
#69195=CARTESIAN_POINT('Ctrl Pts',(1.21455398918813,-1.,-4.00584409524937));
#69196=CARTESIAN_POINT('Ctrl Pts',(1.21455398918813,1.,-4.00584409524937));
#69197=CARTESIAN_POINT('Ctrl Pts',(1.20922097030107,-1.,-4.00009577952534));
#69198=CARTESIAN_POINT('Ctrl Pts',(1.20922097030107,1.,-4.00009577952534));
#69199=CARTESIAN_POINT('Ctrl Pts',(1.2039185237544,-1.,-3.99433084800649));
#69200=CARTESIAN_POINT('Ctrl Pts',(1.2039185237544,1.,-3.99433084800649));
#69201=CARTESIAN_POINT('Ctrl Pts',(1.19864679609596,-1.,-3.98854928957287));
#69202=CARTESIAN_POINT('Ctrl Pts',(1.19864679609596,1.,-3.98854928957287));
#69203=CARTESIAN_POINT('Ctrl Pts',(1.19340598349307,-1.,-3.98275111052015));
#69204=CARTESIAN_POINT('Ctrl Pts',(1.19340598349307,1.,-3.98275111052015));
#69205=CARTESIAN_POINT('Ctrl Pts',(1.18819633715285,-1.,-3.97693634766926));
#69206=CARTESIAN_POINT('Ctrl Pts',(1.18819633715285,1.,-3.97693634766926));
#69207=CARTESIAN_POINT('Ctrl Pts',(1.18301815039596,-1.,-3.9711050516465));
#69208=CARTESIAN_POINT('Ctrl Pts',(1.18301815039596,1.,-3.9711050516465));
#69209=CARTESIAN_POINT('Ctrl Pts',(1.17787174135445,-1.,-3.96525726357682));
#69210=CARTESIAN_POINT('Ctrl Pts',(1.17787174135445,1.,-3.96525726357682));
#69211=CARTESIAN_POINT('Ctrl Pts',(1.17275743590327,-1.,-3.95939299213164));
#69212=CARTESIAN_POINT('Ctrl Pts',(1.17275743590327,1.,-3.95939299213164));
#69213=CARTESIAN_POINT('Ctrl Pts',(1.16767555244495,-1.,-3.95351219510062));
#69214=CARTESIAN_POINT('Ctrl Pts',(1.16767555244495,1.,-3.95351219510062));
#69215=CARTESIAN_POINT('Ctrl Pts',(1.16262637999261,-1.,-3.9476147478092));
#69216=CARTESIAN_POINT('Ctrl Pts',(1.16262637999261,1.,-3.9476147478092));
#69217=CARTESIAN_POINT('Ctrl Pts',(1.1576101834106,-1.,-3.94170046685542));
#69218=CARTESIAN_POINT('Ctrl Pts',(1.1576101834106,1.,-3.94170046685542));
#69219=CARTESIAN_POINT('Ctrl Pts',(1.1526272271639,-1.,-3.9357691705651));
#69220=CARTESIAN_POINT('Ctrl Pts',(1.1526272271639,1.,-3.9357691705651));
#69221=CARTESIAN_POINT('Ctrl Pts',(1.14767779451147,-1.,-3.92982073294334));
#69222=CARTESIAN_POINT('Ctrl Pts',(1.14767779451147,1.,-3.92982073294334));
#69223=CARTESIAN_POINT('Ctrl Pts',(1.14276220561575,-1.,-3.92385513133937));
#69224=CARTESIAN_POINT('Ctrl Pts',(1.14276220561575,1.,-3.92385513133937));
#69225=CARTESIAN_POINT('Ctrl Pts',(1.13788084225511,-1.,-3.91787251936688));
#69226=CARTESIAN_POINT('Ctrl Pts',(1.13788084225511,1.,-3.91787251936688));
#69227=CARTESIAN_POINT('Ctrl Pts',(1.13303414693849,-1.,-3.91187321145495));
#69228=CARTESIAN_POINT('Ctrl Pts',(1.13303414693849,1.,-3.91187321145495));
#69229=CARTESIAN_POINT('Ctrl Pts',(1.12822258281518,-1.,-3.90585753318622));
#69230=CARTESIAN_POINT('Ctrl Pts',(1.12822258281518,1.,-3.90585753318622));
#69231=CARTESIAN_POINT('Ctrl Pts',(1.12344660099029,-1.,-3.89982569749978));
#69232=CARTESIAN_POINT('Ctrl Pts',(1.12344660099029,1.,-3.89982569749978));
#69233=CARTESIAN_POINT('Ctrl Pts',(1.11870660794609,-1.,-3.89377768340362));
#69234=CARTESIAN_POINT('Ctrl Pts',(1.11870660794609,1.,-3.89377768340362));
#69235=CARTESIAN_POINT('Ctrl Pts',(1.11400292434447,-1.,-3.88771308285229));
#69236=CARTESIAN_POINT('Ctrl Pts',(1.11400292434447,1.,-3.88771308285229));
#69237=CARTESIAN_POINT('Ctrl Pts',(1.10933577224029,-1.,-3.88163105531791));
#69238=CARTESIAN_POINT('Ctrl Pts',(1.10933577224029,1.,-3.88163105531791));
#69239=CARTESIAN_POINT('Ctrl Pts',(1.10470536603303,-1.,-3.87553067187566));
#69240=CARTESIAN_POINT('Ctrl Pts',(1.10470536603303,1.,-3.87553067187566));
#69241=CARTESIAN_POINT('Ctrl Pts',(1.10011198761202,-1.,-3.86941120134872));
#69242=CARTESIAN_POINT('Ctrl Pts',(1.10011198761202,1.,-3.86941120134872));
#69243=CARTESIAN_POINT('Ctrl Pts',(1.09555606505012,-1.,-3.86327241021242));
#69244=CARTESIAN_POINT('Ctrl Pts',(1.09555606505012,1.,-3.86327241021242));
#69245=CARTESIAN_POINT('Ctrl Pts',(1.09103825516288,-1.,-3.85711487933911));
#69246=CARTESIAN_POINT('Ctrl Pts',(1.09103825516288,1.,-3.85711487933911));
#69247=CARTESIAN_POINT('Ctrl Pts',(1.08655950846377,-1.,-3.85094025222691));
#69248=CARTESIAN_POINT('Ctrl Pts',(1.08655950846377,1.,-3.85094025222691));
#69249=CARTESIAN_POINT('Ctrl Pts',(1.08212087917986,-1.,-3.84475048030615));
#69250=CARTESIAN_POINT('Ctrl Pts',(1.08212087917986,1.,-3.84475048030615));
#69251=CARTESIAN_POINT('Ctrl Pts',(1.07772335353856,-1.,-3.83854714117486));
#69252=CARTESIAN_POINT('Ctrl Pts',(1.07772335353856,1.,-3.83854714117486));
#69253=CARTESIAN_POINT('Ctrl Pts',(1.0733676663346,-1.,-3.83233071195145));
#69254=CARTESIAN_POINT('Ctrl Pts',(1.0733676663346,1.,-3.83233071195145));
#69255=CARTESIAN_POINT('Ctrl Pts',(1.0690541318036,-1.,-3.82609989967278));
#69256=CARTESIAN_POINT('Ctrl Pts',(1.0690541318036,1.,-3.82609989967278));
#69257=CARTESIAN_POINT('Ctrl Pts',(1.06478244038931,-1.,-3.81985083953012));
#69258=CARTESIAN_POINT('Ctrl Pts',(1.06478244038931,1.,-3.81985083953012));
#69259=CARTESIAN_POINT('Ctrl Pts',(1.06055206187298,-1.,-3.81357866117485));
#69260=CARTESIAN_POINT('Ctrl Pts',(1.06055206187298,1.,-3.81357866117485));
#69261=CARTESIAN_POINT('Ctrl Pts',(1.05636266918643,-1.,-3.80727913637784));
#69262=CARTESIAN_POINT('Ctrl Pts',(1.05636266918643,1.,-3.80727913637784));
#69263=CARTESIAN_POINT('Ctrl Pts',(1.05221457990015,-1.,-3.80095039790678));
#69264=CARTESIAN_POINT('Ctrl Pts',(1.05221457990015,1.,-3.80095039790678));
#69265=CARTESIAN_POINT('Ctrl Pts',(1.04810913267641,-1.,-3.79459440308793));
#69266=CARTESIAN_POINT('Ctrl Pts',(1.04810913267641,1.,-3.79459440308793));
#69267=CARTESIAN_POINT('Ctrl Pts',(1.04404924374426,-1.,-3.78821910787195));
#69268=CARTESIAN_POINT('Ctrl Pts',(1.04404924374426,1.,-3.78821910787195));
#69269=CARTESIAN_POINT('Ctrl Pts',(1.04003862055804,-1.,-3.78183535008192));
#69270=CARTESIAN_POINT('Ctrl Pts',(1.04003862055804,1.,-3.78183535008192));
#69271=CARTESIAN_POINT('Ctrl Pts',(1.03608074678013,-1.,-3.77545283140445));
#69272=CARTESIAN_POINT('Ctrl Pts',(1.03608074678013,1.,-3.77545283140445));
#69273=CARTESIAN_POINT('Ctrl Pts',(1.0321778660492,-1.,-3.76907609832522));
#69274=CARTESIAN_POINT('Ctrl Pts',(1.0321778660492,1.,-3.76907609832522));
#69275=CARTESIAN_POINT('Ctrl Pts',(1.02833014458181,-1.,-3.76270122291232));
#69276=CARTESIAN_POINT('Ctrl Pts',(1.02833014458181,1.,-3.76270122291232));
#69277=CARTESIAN_POINT('Ctrl Pts',(1.0245342944466,-1.,-3.75631037456194));
#69278=CARTESIAN_POINT('Ctrl Pts',(1.0245342944466,1.,-3.75631037456194));
#69279=CARTESIAN_POINT('Ctrl Pts',(1.02078510487428,-1.,-3.74987777155834));
#69280=CARTESIAN_POINT('Ctrl Pts',(1.02078510487428,1.,-3.74987777155834));
#69281=CARTESIAN_POINT('Ctrl Pts',(1.01707794311079,-1.,-3.74337942504959));
#69282=CARTESIAN_POINT('Ctrl Pts',(1.01707794311079,1.,-3.74337942504959));
#69283=CARTESIAN_POINT('Ctrl Pts',(1.01341114319903,-1.,-3.73680245055734));
#69284=CARTESIAN_POINT('Ctrl Pts',(1.01341114319903,1.,-3.73680245055734));
#69285=CARTESIAN_POINT('Ctrl Pts',(1.00978798539496,-1.,-3.73015276704426));
#69286=CARTESIAN_POINT('Ctrl Pts',(1.00978798539496,1.,-3.73015276704426));
#69287=CARTESIAN_POINT('Ctrl Pts',(1.0062200073571,-1.,-3.72346803750596));
#69288=CARTESIAN_POINT('Ctrl Pts',(1.0062200073571,1.,-3.72346803750596));
#69289=CARTESIAN_POINT('Ctrl Pts',(1.00272423396822,-1.,-3.71680667125119));
#69290=CARTESIAN_POINT('Ctrl Pts',(1.00272423396822,1.,-3.71680667125119));
#69291=CARTESIAN_POINT('Ctrl Pts',(0.99931726075653,-1.,-3.71022439713938));
#69292=CARTESIAN_POINT('Ctrl Pts',(0.99931726075653,1.,-3.71022439713938));
#69293=CARTESIAN_POINT('Ctrl Pts',(0.996009819772518,-1.,-3.70375282282138));
#69294=CARTESIAN_POINT('Ctrl Pts',(0.996009819772518,1.,-3.70375282282138));
#69295=CARTESIAN_POINT('Ctrl Pts',(0.99280221833201,-1.,-3.69738123415662));
#69296=CARTESIAN_POINT('Ctrl Pts',(0.99280221833201,1.,-3.69738123415662));
#69297=CARTESIAN_POINT('Ctrl Pts',(0.989676715398558,-1.,-3.69102682138847));
#69298=CARTESIAN_POINT('Ctrl Pts',(0.989676715398558,1.,-3.69102682138847));
#69299=CARTESIAN_POINT('Ctrl Pts',(0.986602639863837,-1.,-3.68455317926068));
#69300=CARTESIAN_POINT('Ctrl Pts',(0.986602639863837,1.,-3.68455317926068));
#69301=CARTESIAN_POINT('Ctrl Pts',(0.983550791470419,-1.,-3.67782408841715));
#69302=CARTESIAN_POINT('Ctrl Pts',(0.983550791470419,1.,-3.67782408841715));
#69303=CARTESIAN_POINT('Ctrl Pts',(0.980505922458267,-1.,-3.67074983340361));
#69304=CARTESIAN_POINT('Ctrl Pts',(0.980505922458267,1.,-3.67074983340361));
#69305=CARTESIAN_POINT('Ctrl Pts',(0.977478312751618,-1.,-3.66333049637475));
#69306=CARTESIAN_POINT('Ctrl Pts',(0.977478312751618,1.,-3.66333049637475));
#69307=CARTESIAN_POINT('Ctrl Pts',(0.974519971354848,-1.,-3.65571576735126));
#69308=CARTESIAN_POINT('Ctrl Pts',(0.974519971354848,1.,-3.65571576735126));
#69309=CARTESIAN_POINT('Ctrl Pts',(0.971722122061341,-1.,-3.64819756447455));
#69310=CARTESIAN_POINT('Ctrl Pts',(0.971722122061341,1.,-3.64819756447455));
#69311=CARTESIAN_POINT('Ctrl Pts',(0.969195124675865,-1.,-3.64113946505766));
#69312=CARTESIAN_POINT('Ctrl Pts',(0.969195124675865,1.,-3.64113946505766));
#69313=CARTESIAN_POINT('Ctrl Pts',(0.967052554541385,-1.,-3.63492122081143));
#69314=CARTESIAN_POINT('Ctrl Pts',(0.967052554541385,1.,-3.63492122081143));
#69315=CARTESIAN_POINT('Ctrl Pts',(0.965395153165293,-1.,-3.62988252139846));
#69316=CARTESIAN_POINT('Ctrl Pts',(0.965395153165293,1.,-3.62988252139846));
#69317=CARTESIAN_POINT('Ctrl Pts',(0.964291001273287,-1.,-3.62625391254797));
#69318=CARTESIAN_POINT('Ctrl Pts',(0.964291001273287,1.,-3.62625391254797));
#69319=CARTESIAN_POINT('Ctrl Pts',(0.963875774530619,-1.,-3.6245656860652));
#69320=CARTESIAN_POINT('Ctrl Pts',(0.963875774530619,1.,-3.6245656860652));
#69321=CARTESIAN_POINT('Ctrl Pts',(0.963832486395051,-1.,-3.62399933639915));
#69322=CARTESIAN_POINT('Ctrl Pts',(0.963832486395051,1.,-3.62399933639915));
#69323=CARTESIAN_POINT('Ctrl Pts',(0.963922720982193,-1.,-3.62393257642052));
#69324=CARTESIAN_POINT('Ctrl Pts',(0.963922720982193,1.,-3.62393257642052));
#69325=CARTESIAN_POINT('Ctrl Pts',(0.963997613369571,-1.,-3.62397690409552));
#69326=CARTESIAN_POINT('Ctrl Pts',(0.963997613369571,1.,-3.62397690409552));
#69327=CARTESIAN_POINT('',(1.22531898815164,1.,-4.01728681790024));
#69328=CARTESIAN_POINT('Ctrl Pts',(1.22531898815164,1.,-4.01728681790024));
#69329=CARTESIAN_POINT('Ctrl Pts',(1.22423716681447,1.,-4.0161454457032));
#69330=CARTESIAN_POINT('Ctrl Pts',(1.22207656456199,1.,-4.01386104434674));
#69331=CARTESIAN_POINT('Ctrl Pts',(1.21884478244983,1.,-4.01042947142681));
#69332=CARTESIAN_POINT('Ctrl Pts',(1.21455398918813,1.,-4.00584409524937));
#69333=CARTESIAN_POINT('Ctrl Pts',(1.20922097030107,1.,-4.00009577952534));
#69334=CARTESIAN_POINT('Ctrl Pts',(1.2039185237544,1.,-3.99433084800649));
#69335=CARTESIAN_POINT('Ctrl Pts',(1.19864679609596,1.,-3.98854928957287));
#69336=CARTESIAN_POINT('Ctrl Pts',(1.19340598349307,1.,-3.98275111052015));
#69337=CARTESIAN_POINT('Ctrl Pts',(1.18819633715285,1.,-3.97693634766926));
#69338=CARTESIAN_POINT('Ctrl Pts',(1.18301815039596,1.,-3.9711050516465));
#69339=CARTESIAN_POINT('Ctrl Pts',(1.17787174135445,1.,-3.96525726357682));
#69340=CARTESIAN_POINT('Ctrl Pts',(1.17275743590327,1.,-3.95939299213164));
#69341=CARTESIAN_POINT('Ctrl Pts',(1.16767555244495,1.,-3.95351219510062));
#69342=CARTESIAN_POINT('Ctrl Pts',(1.16262637999261,1.,-3.9476147478092));
#69343=CARTESIAN_POINT('Ctrl Pts',(1.1576101834106,1.,-3.94170046685542));
#69344=CARTESIAN_POINT('Ctrl Pts',(1.1526272271639,1.,-3.9357691705651));
#69345=CARTESIAN_POINT('Ctrl Pts',(1.14767779451147,1.,-3.92982073294334));
#69346=CARTESIAN_POINT('Ctrl Pts',(1.14276220561575,1.,-3.92385513133937));
#69347=CARTESIAN_POINT('Ctrl Pts',(1.13788084225511,1.,-3.91787251936688));
#69348=CARTESIAN_POINT('Ctrl Pts',(1.13303414693849,1.,-3.91187321145495));
#69349=CARTESIAN_POINT('Ctrl Pts',(1.12822258281518,1.,-3.90585753318622));
#69350=CARTESIAN_POINT('Ctrl Pts',(1.12344660099029,1.,-3.89982569749978));
#69351=CARTESIAN_POINT('Ctrl Pts',(1.11870660794609,1.,-3.89377768340362));
#69352=CARTESIAN_POINT('Ctrl Pts',(1.11400292434447,1.,-3.88771308285229));
#69353=CARTESIAN_POINT('Ctrl Pts',(1.10933577224029,1.,-3.88163105531791));
#69354=CARTESIAN_POINT('Ctrl Pts',(1.10470536603303,1.,-3.87553067187566));
#69355=CARTESIAN_POINT('Ctrl Pts',(1.10011198761202,1.,-3.86941120134872));
#69356=CARTESIAN_POINT('Ctrl Pts',(1.09555606505012,1.,-3.86327241021242));
#69357=CARTESIAN_POINT('Ctrl Pts',(1.09103825516288,1.,-3.85711487933911));
#69358=CARTESIAN_POINT('Ctrl Pts',(1.08655950846377,1.,-3.85094025222691));
#69359=CARTESIAN_POINT('Ctrl Pts',(1.08212087917986,1.,-3.84475048030615));
#69360=CARTESIAN_POINT('Ctrl Pts',(1.07772335353856,1.,-3.83854714117486));
#69361=CARTESIAN_POINT('Ctrl Pts',(1.0733676663346,1.,-3.83233071195145));
#69362=CARTESIAN_POINT('Ctrl Pts',(1.0690541318036,1.,-3.82609989967278));
#69363=CARTESIAN_POINT('Ctrl Pts',(1.06478244038931,1.,-3.81985083953012));
#69364=CARTESIAN_POINT('Ctrl Pts',(1.06055206187298,1.,-3.81357866117485));
#69365=CARTESIAN_POINT('Ctrl Pts',(1.05636266918643,1.,-3.80727913637784));
#69366=CARTESIAN_POINT('Ctrl Pts',(1.05221457990015,1.,-3.80095039790678));
#69367=CARTESIAN_POINT('Ctrl Pts',(1.04810913267641,1.,-3.79459440308793));
#69368=CARTESIAN_POINT('Ctrl Pts',(1.04404924374426,1.,-3.78821910787195));
#69369=CARTESIAN_POINT('Ctrl Pts',(1.04003862055804,1.,-3.78183535008192));
#69370=CARTESIAN_POINT('Ctrl Pts',(1.03608074678013,1.,-3.77545283140445));
#69371=CARTESIAN_POINT('Ctrl Pts',(1.0321778660492,1.,-3.76907609832522));
#69372=CARTESIAN_POINT('Ctrl Pts',(1.02833014458181,1.,-3.76270122291232));
#69373=CARTESIAN_POINT('Ctrl Pts',(1.0245342944466,1.,-3.75631037456194));
#69374=CARTESIAN_POINT('Ctrl Pts',(1.02078510487428,1.,-3.74987777155834));
#69375=CARTESIAN_POINT('Ctrl Pts',(1.01707794311079,1.,-3.74337942504959));
#69376=CARTESIAN_POINT('Ctrl Pts',(1.01341114319903,1.,-3.73680245055734));
#69377=CARTESIAN_POINT('Ctrl Pts',(1.00978798539496,1.,-3.73015276704426));
#69378=CARTESIAN_POINT('Ctrl Pts',(1.0062200073571,1.,-3.72346803750596));
#69379=CARTESIAN_POINT('Ctrl Pts',(1.00272423396822,1.,-3.71680667125119));
#69380=CARTESIAN_POINT('Ctrl Pts',(0.99931726075653,1.,-3.71022439713938));
#69381=CARTESIAN_POINT('Ctrl Pts',(0.996009819772518,1.,-3.70375282282138));
#69382=CARTESIAN_POINT('Ctrl Pts',(0.99280221833201,1.,-3.69738123415662));
#69383=CARTESIAN_POINT('Ctrl Pts',(0.989676715398558,1.,-3.69102682138847));
#69384=CARTESIAN_POINT('Ctrl Pts',(0.986602639863837,1.,-3.68455317926068));
#69385=CARTESIAN_POINT('Ctrl Pts',(0.983550791470419,1.,-3.67782408841715));
#69386=CARTESIAN_POINT('Ctrl Pts',(0.980505922458267,1.,-3.67074983340361));
#69387=CARTESIAN_POINT('Ctrl Pts',(0.977478312751618,1.,-3.66333049637475));
#69388=CARTESIAN_POINT('Ctrl Pts',(0.974519971354848,1.,-3.65571576735126));
#69389=CARTESIAN_POINT('Ctrl Pts',(0.971722122061341,1.,-3.64819756447455));
#69390=CARTESIAN_POINT('Ctrl Pts',(0.969195124675865,1.,-3.64113946505766));
#69391=CARTESIAN_POINT('Ctrl Pts',(0.967052554541385,1.,-3.63492122081143));
#69392=CARTESIAN_POINT('Ctrl Pts',(0.965395153165293,1.,-3.62988252139846));
#69393=CARTESIAN_POINT('Ctrl Pts',(0.964373850166457,1.,-3.62652618145335));
#69394=CARTESIAN_POINT('Ctrl Pts',(0.963957782642843,1.,-3.62489305727662));
#69395=CARTESIAN_POINT('Ctrl Pts',(0.963861297423241,1.,-3.62424461507588));
#69396=CARTESIAN_POINT('Ctrl Pts',(0.963880158555582,1.,-3.6240482887845));
#69397=CARTESIAN_POINT('Ctrl Pts',(0.963899035117249,1.,-3.62400312501246));
#69398=CARTESIAN_POINT('',(1.22531898815164,0.,-4.01728681790024));
#69399=CARTESIAN_POINT('Ctrl Pts',(1.35022972712301,-1.,-3.49848248301936));
#69400=CARTESIAN_POINT('Ctrl Pts',(1.35022972712301,1.,-3.49848248301936));
#69401=CARTESIAN_POINT('Ctrl Pts',(1.35026426118402,-1.,-3.4984026005375));
#69402=CARTESIAN_POINT('Ctrl Pts',(1.35026426118402,1.,-3.4984026005375));
#69403=CARTESIAN_POINT('Ctrl Pts',(1.35037650303019,-1.,-3.49840357193736));
#69404=CARTESIAN_POINT('Ctrl Pts',(1.35037650303019,1.,-3.49840357193736));
#69405=CARTESIAN_POINT('Ctrl Pts',(1.35067437417483,-1.,-3.49888720257132));
#69406=CARTESIAN_POINT('Ctrl Pts',(1.35067437417483,1.,-3.49888720257132));
#69407=CARTESIAN_POINT('Ctrl Pts',(1.3513307633124,-1.,-3.5004970706414));
#69408=CARTESIAN_POINT('Ctrl Pts',(1.3513307633124,1.,-3.5004970706414));
#69409=CARTESIAN_POINT('Ctrl Pts',(1.35257032843486,-1.,-3.50408168106261));
#69410=CARTESIAN_POINT('Ctrl Pts',(1.35257032843486,1.,-3.50408168106261));
#69411=CARTESIAN_POINT('Ctrl Pts',(1.35419113575956,-1.,-3.50913227059999));
#69412=CARTESIAN_POINT('Ctrl Pts',(1.35419113575956,1.,-3.50913227059999));
#69413=CARTESIAN_POINT('Ctrl Pts',(1.35611275237152,-1.,-3.51542230699556));
#69414=CARTESIAN_POINT('Ctrl Pts',(1.35611275237152,1.,-3.51542230699556));
#69415=CARTESIAN_POINT('Ctrl Pts',(1.35821701528836,-1.,-3.52261776116748));
#69416=CARTESIAN_POINT('Ctrl Pts',(1.35821701528836,1.,-3.52261776116748));
#69417=CARTESIAN_POINT('Ctrl Pts',(1.36037259643734,-1.,-3.530344649616));
#69418=CARTESIAN_POINT('Ctrl Pts',(1.36037259643734,1.,-3.530344649616));
#69419=CARTESIAN_POINT('Ctrl Pts',(1.36245507339307,-1.,-3.53824396424961));
#69420=CARTESIAN_POINT('Ctrl Pts',(1.36245507339307,1.,-3.53824396424961));
#69421=CARTESIAN_POINT('Ctrl Pts',(1.36436666257597,-1.,-3.54602591832973));
#69422=CARTESIAN_POINT('Ctrl Pts',(1.36436666257597,1.,-3.54602591832973));
#69423=CARTESIAN_POINT('Ctrl Pts',(1.3660614545677,-1.,-3.55353883995949));
#69424=CARTESIAN_POINT('Ctrl Pts',(1.3660614545677,1.,-3.55353883995949));
#69425=CARTESIAN_POINT('Ctrl Pts',(1.36754771771233,-1.,-3.56077662028649));
#69426=CARTESIAN_POINT('Ctrl Pts',(1.36754771771233,1.,-3.56077662028649));
#69427=CARTESIAN_POINT('Ctrl Pts',(1.36886584973389,-1.,-3.5678208030466));
#69428=CARTESIAN_POINT('Ctrl Pts',(1.36886584973389,1.,-3.5678208030466));
#69429=CARTESIAN_POINT('Ctrl Pts',(1.37007229485659,-1.,-3.57479875549486));
#69430=CARTESIAN_POINT('Ctrl Pts',(1.37007229485659,1.,-3.57479875549486));
#69431=CARTESIAN_POINT('Ctrl Pts',(1.37122241663062,-1.,-3.58183885982715));
#69432=CARTESIAN_POINT('Ctrl Pts',(1.37122241663062,1.,-3.58183885982715));
#69433=CARTESIAN_POINT('Ctrl Pts',(1.37235053660976,-1.,-3.58901853846365));
#69434=CARTESIAN_POINT('Ctrl Pts',(1.37235053660976,1.,-3.58901853846365));
#69435=CARTESIAN_POINT('Ctrl Pts',(1.37346320103157,-1.,-3.59634627869048));
#69436=CARTESIAN_POINT('Ctrl Pts',(1.37346320103157,1.,-3.59634627869048));
#69437=CARTESIAN_POINT('Ctrl Pts',(1.37455051379623,-1.,-3.60379020123988));
#69438=CARTESIAN_POINT('Ctrl Pts',(1.37455051379623,1.,-3.60379020123988));
#69439=CARTESIAN_POINT('Ctrl Pts',(1.37559314436634,-1.,-3.61129546591064));
#69440=CARTESIAN_POINT('Ctrl Pts',(1.37559314436634,1.,-3.61129546591064));
#69441=CARTESIAN_POINT('Ctrl Pts',(1.37657053403107,-1.,-3.61880481160421));
#69442=CARTESIAN_POINT('Ctrl Pts',(1.37657053403107,1.,-3.61880481160421));
#69443=CARTESIAN_POINT('Ctrl Pts',(1.37746987919881,-1.,-3.62628098665145));
#69444=CARTESIAN_POINT('Ctrl Pts',(1.37746987919881,1.,-3.62628098665145));
#69445=CARTESIAN_POINT('Ctrl Pts',(1.37829035457339,-1.,-3.63371727442486));
#69446=CARTESIAN_POINT('Ctrl Pts',(1.37829035457339,1.,-3.63371727442486));
#69447=CARTESIAN_POINT('Ctrl Pts',(1.37903818567359,-1.,-3.64112507791141));
#69448=CARTESIAN_POINT('Ctrl Pts',(1.37903818567359,1.,-3.64112507791141));
#69449=CARTESIAN_POINT('Ctrl Pts',(1.37972372481603,-1.,-3.64852652756456));
#69450=CARTESIAN_POINT('Ctrl Pts',(1.37972372481603,1.,-3.64852652756456));
#69451=CARTESIAN_POINT('Ctrl Pts',(1.38035791051212,-1.,-3.6559455440439));
#69452=CARTESIAN_POINT('Ctrl Pts',(1.38035791051212,1.,-3.6559455440439));
#69453=CARTESIAN_POINT('Ctrl Pts',(1.38094856333552,-1.,-3.66339848520857));
#69454=CARTESIAN_POINT('Ctrl Pts',(1.38094856333552,1.,-3.66339848520857));
#69455=CARTESIAN_POINT('Ctrl Pts',(1.38149812653868,-1.,-3.67088843112262));
#69456=CARTESIAN_POINT('Ctrl Pts',(1.38149812653868,1.,-3.67088843112262));
#69457=CARTESIAN_POINT('Ctrl Pts',(1.3820057429062,-1.,-3.67841038482414));
#69458=CARTESIAN_POINT('Ctrl Pts',(1.3820057429062,1.,-3.67841038482414));
#69459=CARTESIAN_POINT('Ctrl Pts',(1.38246852827182,-1.,-3.68595444983838));
#69460=CARTESIAN_POINT('Ctrl Pts',(1.38246852827182,1.,-3.68595444983838));
#69461=CARTESIAN_POINT('Ctrl Pts',(1.3828831117165,-1.,-3.69350967899526));
#69462=CARTESIAN_POINT('Ctrl Pts',(1.3828831117165,1.,-3.69350967899526));
#69463=CARTESIAN_POINT('Ctrl Pts',(1.38324717612865,-1.,-3.701067921679));
#69464=CARTESIAN_POINT('Ctrl Pts',(1.38324717612865,1.,-3.701067921679));
#69465=CARTESIAN_POINT('Ctrl Pts',(1.38356065402124,-1.,-3.70862680753347));
#69466=CARTESIAN_POINT('Ctrl Pts',(1.38356065402124,1.,-3.70862680753347));
#69467=CARTESIAN_POINT('Ctrl Pts',(1.38382489984586,-1.,-3.7161876605181));
#69468=CARTESIAN_POINT('Ctrl Pts',(1.38382489984586,1.,-3.7161876605181));
#69469=CARTESIAN_POINT('Ctrl Pts',(1.3840421342895,-1.,-3.72375409358803));
#69470=CARTESIAN_POINT('Ctrl Pts',(1.3840421342895,1.,-3.72375409358803));
#69471=CARTESIAN_POINT('Ctrl Pts',(1.38421479111531,-1.,-3.73133035859282));
#69472=CARTESIAN_POINT('Ctrl Pts',(1.38421479111531,1.,-3.73133035859282));
#69473=CARTESIAN_POINT('Ctrl Pts',(1.38434489156458,-1.,-3.73891976418104));
#69474=CARTESIAN_POINT('Ctrl Pts',(1.38434489156458,1.,-3.73891976418104));
#69475=CARTESIAN_POINT('Ctrl Pts',(1.38443344984394,-1.,-3.74652317167876));
#69476=CARTESIAN_POINT('Ctrl Pts',(1.38443344984394,1.,-3.74652317167876));
#69477=CARTESIAN_POINT('Ctrl Pts',(1.38448077997163,-1.,-3.7541397631875));
#69478=CARTESIAN_POINT('Ctrl Pts',(1.38448077997163,1.,-3.7541397631875));
#69479=CARTESIAN_POINT('Ctrl Pts',(1.3844867525335,-1.,-3.76176768271367));
#69480=CARTESIAN_POINT('Ctrl Pts',(1.3844867525335,1.,-3.76176768271367));
#69481=CARTESIAN_POINT('Ctrl Pts',(1.38445107339518,-1.,-3.76940473185779));
#69482=CARTESIAN_POINT('Ctrl Pts',(1.38445107339518,1.,-3.76940473185779));
#69483=CARTESIAN_POINT('Ctrl Pts',(1.38437354551428,-1.,-3.77704902230418));
#69484=CARTESIAN_POINT('Ctrl Pts',(1.38437354551428,1.,-3.77704902230418));
#69485=CARTESIAN_POINT('Ctrl Pts',(1.38425435883756,-1.,-3.78469969805082));
#69486=CARTESIAN_POINT('Ctrl Pts',(1.38425435883756,1.,-3.78469969805082));
#69487=CARTESIAN_POINT('Ctrl Pts',(1.38409399694566,-1.,-3.79235669640841));
#69488=CARTESIAN_POINT('Ctrl Pts',(1.38409399694566,1.,-3.79235669640841));
#69489=CARTESIAN_POINT('Ctrl Pts',(1.38389311766682,-1.,-3.80002044322111));
#69490=CARTESIAN_POINT('Ctrl Pts',(1.38389311766682,1.,-3.80002044322111));
#69491=CARTESIAN_POINT('Ctrl Pts',(1.3836524404622,-1.,-3.80769156398411));
#69492=CARTESIAN_POINT('Ctrl Pts',(1.3836524404622,1.,-3.80769156398411));
#69493=CARTESIAN_POINT('Ctrl Pts',(1.38337263902782,-1.,-3.81537060817811));
#69494=CARTESIAN_POINT('Ctrl Pts',(1.38337263902782,1.,-3.81537060817811));
#69495=CARTESIAN_POINT('Ctrl Pts',(1.38305421262763,-1.,-3.82305771743829));
#69496=CARTESIAN_POINT('Ctrl Pts',(1.38305421262763,1.,-3.82305771743829));
#69497=CARTESIAN_POINT('Ctrl Pts',(1.38269750245138,-1.,-3.8307526698229));
#69498=CARTESIAN_POINT('Ctrl Pts',(1.38269750245138,1.,-3.8307526698229));
#69499=CARTESIAN_POINT('Ctrl Pts',(1.38230274828821,-1.,-3.83845502790746));
#69500=CARTESIAN_POINT('Ctrl Pts',(1.38230274828821,1.,-3.83845502790746));
#69501=CARTESIAN_POINT('Ctrl Pts',(1.38187013346109,-1.,-3.84616425605764));
#69502=CARTESIAN_POINT('Ctrl Pts',(1.38187013346109,1.,-3.84616425605764));
#69503=CARTESIAN_POINT('Ctrl Pts',(1.38139983115049,-1.,-3.85387983979481));
#69504=CARTESIAN_POINT('Ctrl Pts',(1.38139983115049,1.,-3.85387983979481));
#69505=CARTESIAN_POINT('Ctrl Pts',(1.38089205992989,-1.,-3.86160143043959));
#69506=CARTESIAN_POINT('Ctrl Pts',(1.38089205992989,1.,-3.86160143043959));
#69507=CARTESIAN_POINT('Ctrl Pts',(1.38034709213014,-1.,-3.86932885813068));
#69508=CARTESIAN_POINT('Ctrl Pts',(1.38034709213014,1.,-3.86932885813068));
#69509=CARTESIAN_POINT('Ctrl Pts',(1.37976523097073,-1.,-3.87706205830532));
#69510=CARTESIAN_POINT('Ctrl Pts',(1.37976523097073,1.,-3.87706205830532));
#69511=CARTESIAN_POINT('Ctrl Pts',(1.37914679719383,-1.,-3.88480102249278));
#69512=CARTESIAN_POINT('Ctrl Pts',(1.37914679719383,1.,-3.88480102249278));
#69513=CARTESIAN_POINT('Ctrl Pts',(1.3784921128802,-1.,-3.89254574338496));
#69514=CARTESIAN_POINT('Ctrl Pts',(1.3784921128802,1.,-3.89254574338496));
#69515=CARTESIAN_POINT('Ctrl Pts',(1.37780148512792,-1.,-3.90029615196727));
#69516=CARTESIAN_POINT('Ctrl Pts',(1.37780148512792,1.,-3.90029615196727));
#69517=CARTESIAN_POINT('Ctrl Pts',(1.3770751963402,-1.,-3.90805209523486));
#69518=CARTESIAN_POINT('Ctrl Pts',(1.3770751963402,1.,-3.90805209523486));
#69519=CARTESIAN_POINT('Ctrl Pts',(1.37631350505797,-1.,-3.91581337462644));
#69520=CARTESIAN_POINT('Ctrl Pts',(1.37631350505797,1.,-3.91581337462644));
#69521=CARTESIAN_POINT('Ctrl Pts',(1.37551664448242,-1.,-3.92357976987672));
#69522=CARTESIAN_POINT('Ctrl Pts',(1.37551664448242,1.,-3.92357976987672));
#69523=CARTESIAN_POINT('Ctrl Pts',(1.37468482215751,-1.,-3.93135106761844));
#69524=CARTESIAN_POINT('Ctrl Pts',(1.37468482215751,1.,-3.93135106761844));
#69525=CARTESIAN_POINT('Ctrl Pts',(1.37381821967165,-1.,-3.93912709040818));
#69526=CARTESIAN_POINT('Ctrl Pts',(1.37381821967165,1.,-3.93912709040818));
#69527=CARTESIAN_POINT('Ctrl Pts',(1.37291699202807,-1.,-3.94690771785133));
#69528=CARTESIAN_POINT('Ctrl Pts',(1.37291699202807,1.,-3.94690771785133));
#69529=CARTESIAN_POINT('Ctrl Pts',(1.37198126432386,-1.,-3.95469287280914));
#69530=CARTESIAN_POINT('Ctrl Pts',(1.37198126432386,1.,-3.95469287280914));
#69531=CARTESIAN_POINT('Ctrl Pts',(1.3712051561502,-1.,-3.96092458506535));
#69532=CARTESIAN_POINT('Ctrl Pts',(1.3712051561502,1.,-3.96092458506535));
#69533=CARTESIAN_POINT('Ctrl Pts',(1.37060761745635,-1.,-3.96560037974645));
#69534=CARTESIAN_POINT('Ctrl Pts',(1.37060761745635,1.,-3.96560037974645));
#69535=CARTESIAN_POINT('Ctrl Pts',(1.37020239094614,-1.,-3.9687184694131));
#69536=CARTESIAN_POINT('Ctrl Pts',(1.37020239094614,1.,-3.9687184694131));
#69537=CARTESIAN_POINT('Ctrl Pts',(1.36999806084572,-1.,-3.97027773754922));
#69538=CARTESIAN_POINT('Ctrl Pts',(1.36999806084572,1.,-3.97027773754922));
#69539=CARTESIAN_POINT('',(1.35032489087101,1.,-3.4984457533445));
#69540=CARTESIAN_POINT('Ctrl Pts',(1.35032489087101,-1.,-3.4984457533445));
#69541=CARTESIAN_POINT('Ctrl Pts',(1.35032489087101,-0.666666666666667,
-3.4984457533445));
#69542=CARTESIAN_POINT('Ctrl Pts',(1.35032489087101,-0.333333333333333,
-3.4984457533445));
#69543=CARTESIAN_POINT('Ctrl Pts',(1.35032489087101,0.333333333333333,-3.4984457533445));
#69544=CARTESIAN_POINT('Ctrl Pts',(1.35032489087101,0.666666666666667,-3.4984457533445));
#69545=CARTESIAN_POINT('Ctrl Pts',(1.35032489087101,1.,-3.4984457533445));
#69546=CARTESIAN_POINT('',(1.36999806084572,1.,-3.97027773754922));
#69547=CARTESIAN_POINT('',(1.36999806084572,0.,-3.97027773754922));
#69548=CARTESIAN_POINT('Ctrl Pts',(1.35032489087101,1.,-3.49844575334451));
#69549=CARTESIAN_POINT('Ctrl Pts',(1.35036670892966,1.,-3.49847119623846));
#69550=CARTESIAN_POINT('Ctrl Pts',(1.35049736560527,1.,-3.49861894124827));
#69551=CARTESIAN_POINT('Ctrl Pts',(1.35080045218587,1.,-3.49920025459723));
#69552=CARTESIAN_POINT('Ctrl Pts',(1.35142377279517,1.,-3.50076603816491));
#69553=CARTESIAN_POINT('Ctrl Pts',(1.35257032843486,1.,-3.50408168106261));
#69554=CARTESIAN_POINT('Ctrl Pts',(1.35419113575956,1.,-3.50913227059999));
#69555=CARTESIAN_POINT('Ctrl Pts',(1.35611275237152,1.,-3.51542230699556));
#69556=CARTESIAN_POINT('Ctrl Pts',(1.35821701528836,1.,-3.52261776116748));
#69557=CARTESIAN_POINT('Ctrl Pts',(1.36037259643734,1.,-3.530344649616));
#69558=CARTESIAN_POINT('Ctrl Pts',(1.36245507339307,1.,-3.53824396424961));
#69559=CARTESIAN_POINT('Ctrl Pts',(1.36436666257597,1.,-3.54602591832973));
#69560=CARTESIAN_POINT('Ctrl Pts',(1.3660614545677,1.,-3.55353883995949));
#69561=CARTESIAN_POINT('Ctrl Pts',(1.36754771771233,1.,-3.56077662028649));
#69562=CARTESIAN_POINT('Ctrl Pts',(1.36886584973389,1.,-3.5678208030466));
#69563=CARTESIAN_POINT('Ctrl Pts',(1.37007229485659,1.,-3.57479875549486));
#69564=CARTESIAN_POINT('Ctrl Pts',(1.37122241663062,1.,-3.58183885982715));
#69565=CARTESIAN_POINT('Ctrl Pts',(1.37235053660976,1.,-3.58901853846365));
#69566=CARTESIAN_POINT('Ctrl Pts',(1.37346320103157,1.,-3.59634627869048));
#69567=CARTESIAN_POINT('Ctrl Pts',(1.37455051379623,1.,-3.60379020123988));
#69568=CARTESIAN_POINT('Ctrl Pts',(1.37559314436634,1.,-3.61129546591064));
#69569=CARTESIAN_POINT('Ctrl Pts',(1.37657053403107,1.,-3.61880481160421));
#69570=CARTESIAN_POINT('Ctrl Pts',(1.37746987919881,1.,-3.62628098665145));
#69571=CARTESIAN_POINT('Ctrl Pts',(1.37829035457339,1.,-3.63371727442486));
#69572=CARTESIAN_POINT('Ctrl Pts',(1.37903818567359,1.,-3.64112507791141));
#69573=CARTESIAN_POINT('Ctrl Pts',(1.37972372481603,1.,-3.64852652756456));
#69574=CARTESIAN_POINT('Ctrl Pts',(1.38035791051212,1.,-3.6559455440439));
#69575=CARTESIAN_POINT('Ctrl Pts',(1.38094856333552,1.,-3.66339848520857));
#69576=CARTESIAN_POINT('Ctrl Pts',(1.38149812653868,1.,-3.67088843112262));
#69577=CARTESIAN_POINT('Ctrl Pts',(1.3820057429062,1.,-3.67841038482414));
#69578=CARTESIAN_POINT('Ctrl Pts',(1.38246852827182,1.,-3.68595444983838));
#69579=CARTESIAN_POINT('Ctrl Pts',(1.3828831117165,1.,-3.69350967899526));
#69580=CARTESIAN_POINT('Ctrl Pts',(1.38324717612865,1.,-3.701067921679));
#69581=CARTESIAN_POINT('Ctrl Pts',(1.38356065402124,1.,-3.70862680753347));
#69582=CARTESIAN_POINT('Ctrl Pts',(1.38382489984586,1.,-3.7161876605181));
#69583=CARTESIAN_POINT('Ctrl Pts',(1.3840421342895,1.,-3.72375409358803));
#69584=CARTESIAN_POINT('Ctrl Pts',(1.38421479111531,1.,-3.73133035859282));
#69585=CARTESIAN_POINT('Ctrl Pts',(1.38434489156458,1.,-3.73891976418104));
#69586=CARTESIAN_POINT('Ctrl Pts',(1.38443344984394,1.,-3.74652317167876));
#69587=CARTESIAN_POINT('Ctrl Pts',(1.38448077997163,1.,-3.7541397631875));
#69588=CARTESIAN_POINT('Ctrl Pts',(1.3844867525335,1.,-3.76176768271367));
#69589=CARTESIAN_POINT('Ctrl Pts',(1.38445107339518,1.,-3.76940473185779));
#69590=CARTESIAN_POINT('Ctrl Pts',(1.38437354551428,1.,-3.77704902230418));
#69591=CARTESIAN_POINT('Ctrl Pts',(1.38425435883756,1.,-3.78469969805082));
#69592=CARTESIAN_POINT('Ctrl Pts',(1.38409399694566,1.,-3.79235669640841));
#69593=CARTESIAN_POINT('Ctrl Pts',(1.38389311766682,1.,-3.80002044322111));
#69594=CARTESIAN_POINT('Ctrl Pts',(1.3836524404622,1.,-3.80769156398411));
#69595=CARTESIAN_POINT('Ctrl Pts',(1.38337263902782,1.,-3.81537060817811));
#69596=CARTESIAN_POINT('Ctrl Pts',(1.38305421262763,1.,-3.82305771743829));
#69597=CARTESIAN_POINT('Ctrl Pts',(1.38269750245138,1.,-3.8307526698229));
#69598=CARTESIAN_POINT('Ctrl Pts',(1.38230274828821,1.,-3.83845502790746));
#69599=CARTESIAN_POINT('Ctrl Pts',(1.38187013346109,1.,-3.84616425605764));
#69600=CARTESIAN_POINT('Ctrl Pts',(1.38139983115049,1.,-3.85387983979481));
#69601=CARTESIAN_POINT('Ctrl Pts',(1.38089205992989,1.,-3.86160143043959));
#69602=CARTESIAN_POINT('Ctrl Pts',(1.38034709213014,1.,-3.86932885813068));
#69603=CARTESIAN_POINT('Ctrl Pts',(1.37976523097073,1.,-3.87706205830532));
#69604=CARTESIAN_POINT('Ctrl Pts',(1.37914679719383,1.,-3.88480102249278));
#69605=CARTESIAN_POINT('Ctrl Pts',(1.3784921128802,1.,-3.89254574338496));
#69606=CARTESIAN_POINT('Ctrl Pts',(1.37780148512792,1.,-3.90029615196727));
#69607=CARTESIAN_POINT('Ctrl Pts',(1.3770751963402,1.,-3.90805209523486));
#69608=CARTESIAN_POINT('Ctrl Pts',(1.37631350505797,1.,-3.91581337462644));
#69609=CARTESIAN_POINT('Ctrl Pts',(1.37551664448242,1.,-3.92357976987672));
#69610=CARTESIAN_POINT('Ctrl Pts',(1.37468482215751,1.,-3.93135106761844));
#69611=CARTESIAN_POINT('Ctrl Pts',(1.37381821967165,1.,-3.93912709040818));
#69612=CARTESIAN_POINT('Ctrl Pts',(1.37291699202807,1.,-3.94690771785133));
#69613=CARTESIAN_POINT('Ctrl Pts',(1.37198126432386,1.,-3.95469287280914));
#69614=CARTESIAN_POINT('Ctrl Pts',(1.3712051561502,1.,-3.96092458506535));
#69615=CARTESIAN_POINT('Ctrl Pts',(1.37060761745635,1.,-3.96560037974645));
#69616=CARTESIAN_POINT('Ctrl Pts',(1.37020239094614,1.,-3.9687184694131));
#69617=CARTESIAN_POINT('Ctrl Pts',(1.36999806084572,1.,-3.97027773754922));
#69618=CARTESIAN_POINT('Origin',(1.36999806084572,0.,-3.97027773754922));
#69619=CARTESIAN_POINT('',(1.22531898815164,1.,-4.01728681790024));
#69620=CARTESIAN_POINT('Origin',(0.,0.,0.));
#69621=CARTESIAN_POINT('',(1.51895082866166,1.,-3.42859860294378));
#69622=CARTESIAN_POINT('Origin',(0.,1.,0.));
#69623=CARTESIAN_POINT('Ctrl Pts',(1.51895082866166,1.,-3.42859860294378));
#69624=CARTESIAN_POINT('Ctrl Pts',(1.51895082866166,0.666666666666667,-3.42859860294378));
#69625=CARTESIAN_POINT('Ctrl Pts',(1.51895082866166,0.333333333333333,-3.42859860294378));
#69626=CARTESIAN_POINT('Ctrl Pts',(1.51895082866166,-0.333333333333333,
-3.42859860294378));
#69627=CARTESIAN_POINT('Ctrl Pts',(1.51895082866166,-0.666666666666667,
-3.42859860294378));
#69628=CARTESIAN_POINT('Ctrl Pts',(1.51895082866166,-1.,-3.42859860294378));
#69629=CARTESIAN_POINT('Ctrl Pts',(1.83867539237861,-1.,-3.77614523045147));
#69630=CARTESIAN_POINT('Ctrl Pts',(1.83867539237861,1.,-3.77614523045147));
#69631=CARTESIAN_POINT('Ctrl Pts',(1.83742834010821,-1.,-3.77518714458232));
#69632=CARTESIAN_POINT('Ctrl Pts',(1.83742834010821,1.,-3.77518714458232));
#69633=CARTESIAN_POINT('Ctrl Pts',(1.83493697935064,-1.,-3.77326886065484));
#69634=CARTESIAN_POINT('Ctrl Pts',(1.83493697935064,1.,-3.77326886065484));
#69635=CARTESIAN_POINT('Ctrl Pts',(1.83120816956515,-1.,-3.77038509819777));
#69636=CARTESIAN_POINT('Ctrl Pts',(1.83120816956515,1.,-3.77038509819777));
#69637=CARTESIAN_POINT('Ctrl Pts',(1.82625289221933,-1.,-3.76652740355856));
#69638=CARTESIAN_POINT('Ctrl Pts',(1.82625289221933,1.,-3.76652740355856));
#69639=CARTESIAN_POINT('Ctrl Pts',(1.82008629694924,-1.,-3.76168412709652));
#69640=CARTESIAN_POINT('Ctrl Pts',(1.82008629694924,1.,-3.76168412709652));
#69641=CARTESIAN_POINT('Ctrl Pts',(1.81394729834032,-1.,-3.75681965683995));
#69642=CARTESIAN_POINT('Ctrl Pts',(1.81394729834032,1.,-3.75681965683995));
#69643=CARTESIAN_POINT('Ctrl Pts',(1.80783603939662,-1.,-3.75193395888069));
#69644=CARTESIAN_POINT('Ctrl Pts',(1.80783603939662,1.,-3.75193395888069));
#69645=CARTESIAN_POINT('Ctrl Pts',(1.80175271485519,-1.,-3.74702700874954));
#69646=CARTESIAN_POINT('Ctrl Pts',(1.80175271485519,1.,-3.74702700874954));
#69647=CARTESIAN_POINT('Ctrl Pts',(1.79569757859041,-1.,-3.74209880351667));
#69648=CARTESIAN_POINT('Ctrl Pts',(1.79569757859041,1.,-3.74209880351667));
#69649=CARTESIAN_POINT('Ctrl Pts',(1.78967092823139,-1.,-3.73714934729962));
#69650=CARTESIAN_POINT('Ctrl Pts',(1.78967092823139,1.,-3.73714934729962));
#69651=CARTESIAN_POINT('Ctrl Pts',(1.78367308442682,-1.,-3.73217863095022));
#69652=CARTESIAN_POINT('Ctrl Pts',(1.78367308442682,1.,-3.73217863095022));
#69653=CARTESIAN_POINT('Ctrl Pts',(1.77770437039606,-1.,-3.72718661205504));
#69654=CARTESIAN_POINT('Ctrl Pts',(1.77770437039606,1.,-3.72718661205504));
#69655=CARTESIAN_POINT('Ctrl Pts',(1.77176509401846,-1.,-3.72217319911429));
#69656=CARTESIAN_POINT('Ctrl Pts',(1.77176509401846,1.,-3.72217319911429));
#69657=CARTESIAN_POINT('Ctrl Pts',(1.76585552124549,-1.,-3.71713822377676));
#69658=CARTESIAN_POINT('Ctrl Pts',(1.76585552124549,1.,-3.71713822377676));
#69659=CARTESIAN_POINT('Ctrl Pts',(1.75997588499021,-1.,-3.71208146346455));
#69660=CARTESIAN_POINT('Ctrl Pts',(1.75997588499021,1.,-3.71208146346455));
#69661=CARTESIAN_POINT('Ctrl Pts',(1.75412641804148,-1.,-3.70700269736876));
#69662=CARTESIAN_POINT('Ctrl Pts',(1.75412641804148,1.,-3.70700269736876));
#69663=CARTESIAN_POINT('Ctrl Pts',(1.74830738046092,-1.,-3.70190175673422));
#69664=CARTESIAN_POINT('Ctrl Pts',(1.74830738046092,1.,-3.70190175673422));
#69665=CARTESIAN_POINT('Ctrl Pts',(1.74251908492589,-1.,-3.6967785691046));
#69666=CARTESIAN_POINT('Ctrl Pts',(1.74251908492589,1.,-3.6967785691046));
#69667=CARTESIAN_POINT('Ctrl Pts',(1.73676193254493,-1.,-3.69163322647906));
#69668=CARTESIAN_POINT('Ctrl Pts',(1.73676193254493,1.,-3.69163322647906));
#69669=CARTESIAN_POINT('Ctrl Pts',(1.73103640956647,-1.,-3.68646597019188));
#69670=CARTESIAN_POINT('Ctrl Pts',(1.73103640956647,1.,-3.68646597019188));
#69671=CARTESIAN_POINT('Ctrl Pts',(1.72534302437003,-1.,-3.68127704936472));
#69672=CARTESIAN_POINT('Ctrl Pts',(1.72534302437003,1.,-3.68127704936472));
#69673=CARTESIAN_POINT('Ctrl Pts',(1.71968225581787,-1.,-3.67606660374665));
#69674=CARTESIAN_POINT('Ctrl Pts',(1.71968225581787,1.,-3.67606660374665));
#69675=CARTESIAN_POINT('Ctrl Pts',(1.71405450210392,-1.,-3.67083454901629));
#69676=CARTESIAN_POINT('Ctrl Pts',(1.71405450210392,1.,-3.67083454901629));
#69677=CARTESIAN_POINT('Ctrl Pts',(1.70846001610983,-1.,-3.6655804319893));
#69678=CARTESIAN_POINT('Ctrl Pts',(1.70846001610983,1.,-3.6655804319893));
#69679=CARTESIAN_POINT('Ctrl Pts',(1.70289888566904,-1.,-3.6603033877491));
#69680=CARTESIAN_POINT('Ctrl Pts',(1.70289888566904,1.,-3.6603033877491));
#69681=CARTESIAN_POINT('Ctrl Pts',(1.69737117722558,-1.,-3.65500246526798));
#69682=CARTESIAN_POINT('Ctrl Pts',(1.69737117722558,1.,-3.65500246526798));
#69683=CARTESIAN_POINT('Ctrl Pts',(1.691877054817,-1.,-3.64967689827393));
#69684=CARTESIAN_POINT('Ctrl Pts',(1.691877054817,1.,-3.64967689827393));
#69685=CARTESIAN_POINT('Ctrl Pts',(1.68641690471455,-1.,-3.64432638915199));
#69686=CARTESIAN_POINT('Ctrl Pts',(1.68641690471455,1.,-3.64432638915199));
#69687=CARTESIAN_POINT('Ctrl Pts',(1.68099146651577,-1.,-3.63895140887443));
#69688=CARTESIAN_POINT('Ctrl Pts',(1.68099146651577,1.,-3.63895140887443));
#69689=CARTESIAN_POINT('Ctrl Pts',(1.67560193613145,-1.,-3.63355343201211));
#69690=CARTESIAN_POINT('Ctrl Pts',(1.67560193613145,1.,-3.63355343201211));
#69691=CARTESIAN_POINT('Ctrl Pts',(1.67024966008037,-1.,-3.62813422105257));
#69692=CARTESIAN_POINT('Ctrl Pts',(1.67024966008037,1.,-3.62813422105257));
#69693=CARTESIAN_POINT('Ctrl Pts',(1.66493585923853,-1.,-3.62269517989104));
#69694=CARTESIAN_POINT('Ctrl Pts',(1.66493585923853,1.,-3.62269517989104));
#69695=CARTESIAN_POINT('Ctrl Pts',(1.65966133399186,-1.,-3.61723666482457));
#69696=CARTESIAN_POINT('Ctrl Pts',(1.65966133399186,1.,-3.61723666482457));
#69697=CARTESIAN_POINT('Ctrl Pts',(1.65442619244327,-1.,-3.61175734965129));
#69698=CARTESIAN_POINT('Ctrl Pts',(1.65442619244327,1.,-3.61175734965129));
#69699=CARTESIAN_POINT('Ctrl Pts',(1.64922952425833,-1.,-3.60625346556992));
#69700=CARTESIAN_POINT('Ctrl Pts',(1.64922952425833,1.,-3.60625346556992));
#69701=CARTESIAN_POINT('Ctrl Pts',(1.6440700438558,-1.,-3.6007202851384));
#69702=CARTESIAN_POINT('Ctrl Pts',(1.6440700438558,1.,-3.6007202851384));
#69703=CARTESIAN_POINT('Ctrl Pts',(1.63894676675349,-1.,-3.59515368334887));
#69704=CARTESIAN_POINT('Ctrl Pts',(1.63894676675349,1.,-3.59515368334887));
#69705=CARTESIAN_POINT('Ctrl Pts',(1.63385971451259,-1.,-3.58955176627876));
#69706=CARTESIAN_POINT('Ctrl Pts',(1.63385971451259,1.,-3.58955176627876));
#69707=CARTESIAN_POINT('Ctrl Pts',(1.62881051550748,-1.,-3.5839162577435));
#69708=CARTESIAN_POINT('Ctrl Pts',(1.62881051550748,1.,-3.5839162577435));
#69709=CARTESIAN_POINT('Ctrl Pts',(1.62380329464851,-1.,-3.57825455954405));
#69710=CARTESIAN_POINT('Ctrl Pts',(1.62380329464851,1.,-3.57825455954405));
#69711=CARTESIAN_POINT('Ctrl Pts',(1.61884340915412,-1.,-3.57257679609826));
#69712=CARTESIAN_POINT('Ctrl Pts',(1.61884340915412,1.,-3.57257679609826));
#69713=CARTESIAN_POINT('Ctrl Pts',(1.61393581747522,-1.,-3.56689200468404));
#69714=CARTESIAN_POINT('Ctrl Pts',(1.61393581747522,1.,-3.56689200468404));
#69715=CARTESIAN_POINT('Ctrl Pts',(1.60908344685459,-1.,-3.56120432482986));
#69716=CARTESIAN_POINT('Ctrl Pts',(1.60908344685459,1.,-3.56120432482986));
#69717=CARTESIAN_POINT('Ctrl Pts',(1.60428584699848,-1.,-3.55550985096117));
#69718=CARTESIAN_POINT('Ctrl Pts',(1.60428584699848,1.,-3.55550985096117));
#69719=CARTESIAN_POINT('Ctrl Pts',(1.59953698113444,-1.,-3.54979148634426));
#69720=CARTESIAN_POINT('Ctrl Pts',(1.59953698113444,1.,-3.54979148634426));
#69721=CARTESIAN_POINT('Ctrl Pts',(1.5948276694975,-1.,-3.544024581823));
#69722=CARTESIAN_POINT('Ctrl Pts',(1.5948276694975,1.,-3.544024581823));
#69723=CARTESIAN_POINT('Ctrl Pts',(1.59014958368725,-1.,-3.53818616861045));
#69724=CARTESIAN_POINT('Ctrl Pts',(1.59014958368725,1.,-3.53818616861045));
#69725=CARTESIAN_POINT('Ctrl Pts',(1.58549906268083,-1.,-3.53226378147068));
#69726=CARTESIAN_POINT('Ctrl Pts',(1.58549906268083,1.,-3.53226378147068));
#69727=CARTESIAN_POINT('Ctrl Pts',(1.58088027227856,-1.,-3.52626275334899));
#69728=CARTESIAN_POINT('Ctrl Pts',(1.58088027227856,1.,-3.52626275334899));
#69729=CARTESIAN_POINT('Ctrl Pts',(1.5763104998818,-1.,-3.52021847865961));
#69730=CARTESIAN_POINT('Ctrl Pts',(1.5763104998818,1.,-3.52021847865961));
#69731=CARTESIAN_POINT('Ctrl Pts',(1.57181569799774,-1.,-3.51418598431733));
#69732=CARTESIAN_POINT('Ctrl Pts',(1.57181569799774,1.,-3.51418598431733));
#69733=CARTESIAN_POINT('Ctrl Pts',(1.56742097575041,-1.,-3.50821771695427));
#69734=CARTESIAN_POINT('Ctrl Pts',(1.56742097575041,1.,-3.50821771695427));
#69735=CARTESIAN_POINT('Ctrl Pts',(1.56314187758689,-1.,-3.50234321621607));
#69736=CARTESIAN_POINT('Ctrl Pts',(1.56314187758689,1.,-3.50234321621607));
#69737=CARTESIAN_POINT('Ctrl Pts',(1.55897703097859,-1.,-3.49655185179623));
#69738=CARTESIAN_POINT('Ctrl Pts',(1.55897703097859,1.,-3.49655185179623));
#69739=CARTESIAN_POINT('Ctrl Pts',(1.5548959590107,-1.,-3.49076460877317));
#69740=CARTESIAN_POINT('Ctrl Pts',(1.5548959590107,1.,-3.49076460877317));
#69741=CARTESIAN_POINT('Ctrl Pts',(1.55084702970382,-1.,-3.48485155928414));
#69742=CARTESIAN_POINT('Ctrl Pts',(1.55084702970382,1.,-3.48485155928414));
#69743=CARTESIAN_POINT('Ctrl Pts',(1.54678009290206,-1.,-3.47868272898599));
#69744=CARTESIAN_POINT('Ctrl Pts',(1.54678009290206,1.,-3.47868272898599));
#69745=CARTESIAN_POINT('Ctrl Pts',(1.54266605398152,-1.,-3.47217189224576));
#69746=CARTESIAN_POINT('Ctrl Pts',(1.54266605398152,1.,-3.47217189224576));
#69747=CARTESIAN_POINT('Ctrl Pts',(1.53851507915533,-1.,-3.46531752207222));
#69748=CARTESIAN_POINT('Ctrl Pts',(1.53851507915533,1.,-3.46531752207222));
#69749=CARTESIAN_POINT('Ctrl Pts',(1.53440195378902,-1.,-3.45825932955273));
#69750=CARTESIAN_POINT('Ctrl Pts',(1.53440195378902,1.,-3.45825932955273));
#69751=CARTESIAN_POINT('Ctrl Pts',(1.530462444618,-1.,-3.45127136828667));
#69752=CARTESIAN_POINT('Ctrl Pts',(1.530462444618,1.,-3.45127136828667));
#69753=CARTESIAN_POINT('Ctrl Pts',(1.52686242875717,-1.,-3.44469547527));
#69754=CARTESIAN_POINT('Ctrl Pts',(1.52686242875717,1.,-3.44469547527));
#69755=CARTESIAN_POINT('Ctrl Pts',(1.52377348950429,-1.,-3.43888895974182));
#69756=CARTESIAN_POINT('Ctrl Pts',(1.52377348950429,1.,-3.43888895974182));
#69757=CARTESIAN_POINT('Ctrl Pts',(1.52134826724227,-1.,-3.43417156977749));
#69758=CARTESIAN_POINT('Ctrl Pts',(1.52134826724227,1.,-3.43417156977749));
#69759=CARTESIAN_POINT('Ctrl Pts',(1.51969006980792,-1.,-3.43076036253384));
#69760=CARTESIAN_POINT('Ctrl Pts',(1.51969006980792,1.,-3.43076036253384));
#69761=CARTESIAN_POINT('Ctrl Pts',(1.51901585838879,-1.,-3.42915787669388));
#69762=CARTESIAN_POINT('Ctrl Pts',(1.51901585838879,1.,-3.42915787669388));
#69763=CARTESIAN_POINT('Ctrl Pts',(1.51888450659497,-1.,-3.42860527148835));
#69764=CARTESIAN_POINT('Ctrl Pts',(1.51888450659497,1.,-3.42860527148835));
#69765=CARTESIAN_POINT('Ctrl Pts',(1.51896318668306,-1.,-3.42852521763648));
#69766=CARTESIAN_POINT('Ctrl Pts',(1.51896318668306,1.,-3.42852521763648));
#69767=CARTESIAN_POINT('Ctrl Pts',(1.519044091397,-1.,-3.42855728381368));
#69768=CARTESIAN_POINT('Ctrl Pts',(1.519044091397,1.,-3.42855728381368));
#69769=CARTESIAN_POINT('',(1.83867539237861,1.,-3.77614523045147));
#69770=CARTESIAN_POINT('Ctrl Pts',(1.83867539237861,1.,-3.77614523045147));
#69771=CARTESIAN_POINT('Ctrl Pts',(1.83742834010821,1.,-3.77518714458232));
#69772=CARTESIAN_POINT('Ctrl Pts',(1.83493697935064,1.,-3.77326886065484));
#69773=CARTESIAN_POINT('Ctrl Pts',(1.83120816956515,1.,-3.77038509819777));
#69774=CARTESIAN_POINT('Ctrl Pts',(1.82625289221933,1.,-3.76652740355856));
#69775=CARTESIAN_POINT('Ctrl Pts',(1.82008629694924,1.,-3.76168412709652));
#69776=CARTESIAN_POINT('Ctrl Pts',(1.81394729834032,1.,-3.75681965683995));
#69777=CARTESIAN_POINT('Ctrl Pts',(1.80783603939662,1.,-3.75193395888069));
#69778=CARTESIAN_POINT('Ctrl Pts',(1.80175271485519,1.,-3.74702700874954));
#69779=CARTESIAN_POINT('Ctrl Pts',(1.79569757859041,1.,-3.74209880351667));
#69780=CARTESIAN_POINT('Ctrl Pts',(1.78967092823139,1.,-3.73714934729962));
#69781=CARTESIAN_POINT('Ctrl Pts',(1.78367308442682,1.,-3.73217863095022));
#69782=CARTESIAN_POINT('Ctrl Pts',(1.77770437039606,1.,-3.72718661205504));
#69783=CARTESIAN_POINT('Ctrl Pts',(1.77176509401846,1.,-3.72217319911429));
#69784=CARTESIAN_POINT('Ctrl Pts',(1.76585552124549,1.,-3.71713822377676));
#69785=CARTESIAN_POINT('Ctrl Pts',(1.75997588499021,1.,-3.71208146346455));
#69786=CARTESIAN_POINT('Ctrl Pts',(1.75412641804148,1.,-3.70700269736876));
#69787=CARTESIAN_POINT('Ctrl Pts',(1.74830738046092,1.,-3.70190175673422));
#69788=CARTESIAN_POINT('Ctrl Pts',(1.74251908492589,1.,-3.6967785691046));
#69789=CARTESIAN_POINT('Ctrl Pts',(1.73676193254493,1.,-3.69163322647906));
#69790=CARTESIAN_POINT('Ctrl Pts',(1.73103640956647,1.,-3.68646597019188));
#69791=CARTESIAN_POINT('Ctrl Pts',(1.72534302437003,1.,-3.68127704936472));
#69792=CARTESIAN_POINT('Ctrl Pts',(1.71968225581787,1.,-3.67606660374665));
#69793=CARTESIAN_POINT('Ctrl Pts',(1.71405450210392,1.,-3.67083454901629));
#69794=CARTESIAN_POINT('Ctrl Pts',(1.70846001610983,1.,-3.6655804319893));
#69795=CARTESIAN_POINT('Ctrl Pts',(1.70289888566904,1.,-3.6603033877491));
#69796=CARTESIAN_POINT('Ctrl Pts',(1.69737117722558,1.,-3.65500246526798));
#69797=CARTESIAN_POINT('Ctrl Pts',(1.691877054817,1.,-3.64967689827393));
#69798=CARTESIAN_POINT('Ctrl Pts',(1.68641690471455,1.,-3.64432638915199));
#69799=CARTESIAN_POINT('Ctrl Pts',(1.68099146651577,1.,-3.63895140887443));
#69800=CARTESIAN_POINT('Ctrl Pts',(1.67560193613145,1.,-3.63355343201211));
#69801=CARTESIAN_POINT('Ctrl Pts',(1.67024966008037,1.,-3.62813422105257));
#69802=CARTESIAN_POINT('Ctrl Pts',(1.66493585923853,1.,-3.62269517989104));
#69803=CARTESIAN_POINT('Ctrl Pts',(1.65966133399186,1.,-3.61723666482457));
#69804=CARTESIAN_POINT('Ctrl Pts',(1.65442619244327,1.,-3.61175734965129));
#69805=CARTESIAN_POINT('Ctrl Pts',(1.64922952425833,1.,-3.60625346556992));
#69806=CARTESIAN_POINT('Ctrl Pts',(1.6440700438558,1.,-3.6007202851384));
#69807=CARTESIAN_POINT('Ctrl Pts',(1.63894676675349,1.,-3.59515368334887));
#69808=CARTESIAN_POINT('Ctrl Pts',(1.63385971451259,1.,-3.58955176627876));
#69809=CARTESIAN_POINT('Ctrl Pts',(1.62881051550748,1.,-3.5839162577435));
#69810=CARTESIAN_POINT('Ctrl Pts',(1.62380329464851,1.,-3.57825455954405));
#69811=CARTESIAN_POINT('Ctrl Pts',(1.61884340915412,1.,-3.57257679609826));
#69812=CARTESIAN_POINT('Ctrl Pts',(1.61393581747522,1.,-3.56689200468404));
#69813=CARTESIAN_POINT('Ctrl Pts',(1.60908344685459,1.,-3.56120432482986));
#69814=CARTESIAN_POINT('Ctrl Pts',(1.60428584699848,1.,-3.55550985096117));
#69815=CARTESIAN_POINT('Ctrl Pts',(1.59953698113444,1.,-3.54979148634426));
#69816=CARTESIAN_POINT('Ctrl Pts',(1.5948276694975,1.,-3.544024581823));
#69817=CARTESIAN_POINT('Ctrl Pts',(1.59014958368725,1.,-3.53818616861045));
#69818=CARTESIAN_POINT('Ctrl Pts',(1.58549906268083,1.,-3.53226378147068));
#69819=CARTESIAN_POINT('Ctrl Pts',(1.58088027227856,1.,-3.52626275334899));
#69820=CARTESIAN_POINT('Ctrl Pts',(1.5763104998818,1.,-3.52021847865961));
#69821=CARTESIAN_POINT('Ctrl Pts',(1.57181569799774,1.,-3.51418598431733));
#69822=CARTESIAN_POINT('Ctrl Pts',(1.56742097575041,1.,-3.50821771695427));
#69823=CARTESIAN_POINT('Ctrl Pts',(1.56314187758689,1.,-3.50234321621607));
#69824=CARTESIAN_POINT('Ctrl Pts',(1.55897703097859,1.,-3.49655185179623));
#69825=CARTESIAN_POINT('Ctrl Pts',(1.5548959590107,1.,-3.49076460877317));
#69826=CARTESIAN_POINT('Ctrl Pts',(1.55084702970382,1.,-3.48485155928414));
#69827=CARTESIAN_POINT('Ctrl Pts',(1.54678009290206,1.,-3.47868272898599));
#69828=CARTESIAN_POINT('Ctrl Pts',(1.54266605398152,1.,-3.47217189224576));
#69829=CARTESIAN_POINT('Ctrl Pts',(1.53851507915533,1.,-3.46531752207222));
#69830=CARTESIAN_POINT('Ctrl Pts',(1.53440195378902,1.,-3.45825932955273));
#69831=CARTESIAN_POINT('Ctrl Pts',(1.530462444618,1.,-3.45127136828667));
#69832=CARTESIAN_POINT('Ctrl Pts',(1.52686242875717,1.,-3.44469547527));
#69833=CARTESIAN_POINT('Ctrl Pts',(1.52377348950429,1.,-3.43888895974182));
#69834=CARTESIAN_POINT('Ctrl Pts',(1.52134826724227,1.,-3.43417156977749));
#69835=CARTESIAN_POINT('Ctrl Pts',(1.5198144909343,1.,-3.43101631893491));
#69836=CARTESIAN_POINT('Ctrl Pts',(1.51914806898539,1.,-3.42946838852728));
#69837=CARTESIAN_POINT('Ctrl Pts',(1.51895133295017,1.,-3.42884302333978));
#69838=CARTESIAN_POINT('Ctrl Pts',(1.51893924967231,1.,-3.42864616361967));
#69839=CARTESIAN_POINT('Ctrl Pts',(1.51895082866166,1.,-3.42859860294378));
#69840=CARTESIAN_POINT('',(1.83867539237861,0.,-3.77614523045147));
#69841=CARTESIAN_POINT('Ctrl Pts',(1.8808893942881,-1.,-3.24418789321065));
#69842=CARTESIAN_POINT('Ctrl Pts',(1.8808893942881,1.,-3.24418789321065));
#69843=CARTESIAN_POINT('Ctrl Pts',(1.8809110068042,-1.,-3.24410359189733));
#69844=CARTESIAN_POINT('Ctrl Pts',(1.8809110068042,1.,-3.24410359189733));
#69845=CARTESIAN_POINT('Ctrl Pts',(1.8810220187274,-1.,-3.24408699284449));
#69846=CARTESIAN_POINT('Ctrl Pts',(1.8810220187274,1.,-3.24408699284449));
#69847=CARTESIAN_POINT('Ctrl Pts',(1.88139187908347,-1.,-3.24451807186964));
#69848=CARTESIAN_POINT('Ctrl Pts',(1.88139187908347,1.,-3.24451807186964));
#69849=CARTESIAN_POINT('Ctrl Pts',(1.88229202583187,-1.,-3.24600543790876));
#69850=CARTESIAN_POINT('Ctrl Pts',(1.88229202583187,1.,-3.24600543790876));
#69851=CARTESIAN_POINT('Ctrl Pts',(1.88407708646435,-1.,-3.24935200512055));
#69852=CARTESIAN_POINT('Ctrl Pts',(1.88407708646435,1.,-3.24935200512055));
#69853=CARTESIAN_POINT('Ctrl Pts',(1.88646802523372,-1.,-3.25408686339298));
#69854=CARTESIAN_POINT('Ctrl Pts',(1.88646802523372,1.,-3.25408686339298));
#69855=CARTESIAN_POINT('Ctrl Pts',(1.88934996203508,-1.,-3.2599988519361));
#69856=CARTESIAN_POINT('Ctrl Pts',(1.88934996203508,1.,-3.2599988519361));
#69857=CARTESIAN_POINT('Ctrl Pts',(1.89255393500769,-1.,-3.2667765388833));
#69858=CARTESIAN_POINT('Ctrl Pts',(1.89255393500769,1.,-3.2667765388833));
#69859=CARTESIAN_POINT('Ctrl Pts',(1.89589172903662,-1.,-3.27407108932908));
#69860=CARTESIAN_POINT('Ctrl Pts',(1.89589172903662,1.,-3.27407108932908));
#69861=CARTESIAN_POINT('Ctrl Pts',(1.89918429230424,-1.,-3.28154737912287));
#69862=CARTESIAN_POINT('Ctrl Pts',(1.89918429230424,1.,-3.28154737912287));
#69863=CARTESIAN_POINT('Ctrl Pts',(1.9022897124757,-1.,-3.28893448600364));
#69864=CARTESIAN_POINT('Ctrl Pts',(1.9022897124757,1.,-3.28893448600364));
#69865=CARTESIAN_POINT('Ctrl Pts',(1.9051389186417,-1.,-3.29608978722258));
#69866=CARTESIAN_POINT('Ctrl Pts',(1.9051389186417,1.,-3.29608978722258));
#69867=CARTESIAN_POINT('Ctrl Pts',(1.90773912171424,-1.,-3.30300595568341));
#69868=CARTESIAN_POINT('Ctrl Pts',(1.90773912171424,1.,-3.30300595568341));
#69869=CARTESIAN_POINT('Ctrl Pts',(1.91014297830502,-1.,-3.30975721158694));
#69870=CARTESIAN_POINT('Ctrl Pts',(1.91014297830502,1.,-3.30975721158694));
#69871=CARTESIAN_POINT('Ctrl Pts',(1.91242616234459,-1.,-3.31646052426395));
#69872=CARTESIAN_POINT('Ctrl Pts',(1.91242616234459,1.,-3.31646052426395));
#69873=CARTESIAN_POINT('Ctrl Pts',(1.91466343916612,-1.,-3.32323403454507));
#69874=CARTESIAN_POINT('Ctrl Pts',(1.91466343916612,1.,-3.32323403454507));
#69875=CARTESIAN_POINT('Ctrl Pts',(1.91690081930297,-1.,-3.33014884257812));
#69876=CARTESIAN_POINT('Ctrl Pts',(1.91690081930297,1.,-3.33014884257812));
#69877=CARTESIAN_POINT('Ctrl Pts',(1.91914609610173,-1.,-3.33721230709948));
#69878=CARTESIAN_POINT('Ctrl Pts',(1.91914609610173,1.,-3.33721230709948));
#69879=CARTESIAN_POINT('Ctrl Pts',(1.92138450828378,-1.,-3.34439448941915));
#69880=CARTESIAN_POINT('Ctrl Pts',(1.92138450828378,1.,-3.34439448941915));
#69881=CARTESIAN_POINT('Ctrl Pts',(1.92358838440518,-1.,-3.35164424847207));
#69882=CARTESIAN_POINT('Ctrl Pts',(1.92358838440518,1.,-3.35164424847207));
#69883=CARTESIAN_POINT('Ctrl Pts',(1.92572846125763,-1.,-3.35890824422976));
#69884=CARTESIAN_POINT('Ctrl Pts',(1.92572846125763,1.,-3.35890824422976));
#69885=CARTESIAN_POINT('Ctrl Pts',(1.92778626543803,-1.,-3.36615168657597));
#69886=CARTESIAN_POINT('Ctrl Pts',(1.92778626543803,1.,-3.36615168657597));
#69887=CARTESIAN_POINT('Ctrl Pts',(1.92975993109897,-1.,-3.37336807068078));
#69888=CARTESIAN_POINT('Ctrl Pts',(1.92975993109897,1.,-3.37336807068078));
#69889=CARTESIAN_POINT('Ctrl Pts',(1.93165739093292,-1.,-3.38056768525577));
#69890=CARTESIAN_POINT('Ctrl Pts',(1.93165739093292,1.,-3.38056768525577));
#69891=CARTESIAN_POINT('Ctrl Pts',(1.93349233176794,-1.,-3.38777076883267));
#69892=CARTESIAN_POINT('Ctrl Pts',(1.93349233176794,1.,-3.38777076883267));
#69893=CARTESIAN_POINT('Ctrl Pts',(1.93527929945982,-1.,-3.39499923640789));
#69894=CARTESIAN_POINT('Ctrl Pts',(1.93527929945982,1.,-3.39499923640789));
#69895=CARTESIAN_POINT('Ctrl Pts',(1.93702857723089,-1.,-3.40226802104093));
#69896=CARTESIAN_POINT('Ctrl Pts',(1.93702857723089,1.,-3.40226802104093));
#69897=CARTESIAN_POINT('Ctrl Pts',(1.93874306008132,-1.,-3.40957978266623));
#69898=CARTESIAN_POINT('Ctrl Pts',(1.93874306008132,1.,-3.40957978266623));
#69899=CARTESIAN_POINT('Ctrl Pts',(1.94042111965237,-1.,-3.41692971994082));
#69900=CARTESIAN_POINT('Ctrl Pts',(1.94042111965237,1.,-3.41692971994082));
#69901=CARTESIAN_POINT('Ctrl Pts',(1.94205835913692,-1.,-3.42430850941497));
#69902=CARTESIAN_POINT('Ctrl Pts',(1.94205835913692,1.,-3.42430850941497));
#69903=CARTESIAN_POINT('Ctrl Pts',(1.94364973660285,-1.,-3.43170586602436));
#69904=CARTESIAN_POINT('Ctrl Pts',(1.94364973660285,1.,-3.43170586602436));
#69905=CARTESIAN_POINT('Ctrl Pts',(1.94519168842883,-1.,-3.43911410197693));
#69906=CARTESIAN_POINT('Ctrl Pts',(1.94519168842883,1.,-3.43911410197693));
#69907=CARTESIAN_POINT('Ctrl Pts',(1.94668377715332,-1.,-3.44653088665685));
#69908=CARTESIAN_POINT('Ctrl Pts',(1.94668377715332,1.,-3.44653088665685));
#69909=CARTESIAN_POINT('Ctrl Pts',(1.94812754766524,-1.,-3.45395731584051));
#69910=CARTESIAN_POINT('Ctrl Pts',(1.94812754766524,1.,-3.45395731584051));
#69911=CARTESIAN_POINT('Ctrl Pts',(1.94952575850196,-1.,-3.46139661060959));
#69912=CARTESIAN_POINT('Ctrl Pts',(1.94952575850196,1.,-3.46139661060959));
#69913=CARTESIAN_POINT('Ctrl Pts',(1.95088147859876,-1.,-3.4688525897419));
#69914=CARTESIAN_POINT('Ctrl Pts',(1.95088147859876,1.,-3.4688525897419));
#69915=CARTESIAN_POINT('Ctrl Pts',(1.95219722189878,-1.,-3.47632820495926));
#69916=CARTESIAN_POINT('Ctrl Pts',(1.95219722189878,1.,-3.47632820495926));
#69917=CARTESIAN_POINT('Ctrl Pts',(1.95347412486316,-1.,-3.48382414832649));
#69918=CARTESIAN_POINT('Ctrl Pts',(1.95347412486316,1.,-3.48382414832649));
#69919=CARTESIAN_POINT('Ctrl Pts',(1.95471236969653,-1.,-3.49133956289154));
#69920=CARTESIAN_POINT('Ctrl Pts',(1.95471236969653,1.,-3.49133956289154));
#69921=CARTESIAN_POINT('Ctrl Pts',(1.9559115382367,-1.,-3.49887263575602));
#69922=CARTESIAN_POINT('Ctrl Pts',(1.9559115382367,1.,-3.49887263575602));
#69923=CARTESIAN_POINT('Ctrl Pts',(1.95707099606513,-1.,-3.50642124159913));
#69924=CARTESIAN_POINT('Ctrl Pts',(1.95707099606513,1.,-3.50642124159913));
#69925=CARTESIAN_POINT('Ctrl Pts',(1.95819025316768,-1.,-3.51398354617773));
#69926=CARTESIAN_POINT('Ctrl Pts',(1.95819025316768,1.,-3.51398354617773));
#69927=CARTESIAN_POINT('Ctrl Pts',(1.95926936324436,-1.,-3.52155867431438));
#69928=CARTESIAN_POINT('Ctrl Pts',(1.95926936324436,1.,-3.52155867431438));
#69929=CARTESIAN_POINT('Ctrl Pts',(1.96030879411534,-1.,-3.52914648844289));
#69930=CARTESIAN_POINT('Ctrl Pts',(1.96030879411534,1.,-3.52914648844289));
#69931=CARTESIAN_POINT('Ctrl Pts',(1.96130926212661,-1.,-3.53674730625759));
#69932=CARTESIAN_POINT('Ctrl Pts',(1.96130926212661,1.,-3.53674730625759));
#69933=CARTESIAN_POINT('Ctrl Pts',(1.96227157573058,-1.,-3.54436163300425));
#69934=CARTESIAN_POINT('Ctrl Pts',(1.96227157573058,1.,-3.54436163300425));
#69935=CARTESIAN_POINT('Ctrl Pts',(1.96319648628667,-1.,-3.55198990600929));
#69936=CARTESIAN_POINT('Ctrl Pts',(1.96319648628667,1.,-3.55198990600929));
#69937=CARTESIAN_POINT('Ctrl Pts',(1.96408450906868,-1.,-3.55963218706201));
#69938=CARTESIAN_POINT('Ctrl Pts',(1.96408450906868,1.,-3.55963218706201));
#69939=CARTESIAN_POINT('Ctrl Pts',(1.96493594634643,-1.,-3.56728820357933));
#69940=CARTESIAN_POINT('Ctrl Pts',(1.96493594634643,1.,-3.56728820357933));
#69941=CARTESIAN_POINT('Ctrl Pts',(1.96575096652857,-1.,-3.57495748601088));
#69942=CARTESIAN_POINT('Ctrl Pts',(1.96575096652857,1.,-3.57495748601088));
#69943=CARTESIAN_POINT('Ctrl Pts',(1.9665296668894,-1.,-3.58263947663884));
#69944=CARTESIAN_POINT('Ctrl Pts',(1.9665296668894,1.,-3.58263947663884));
#69945=CARTESIAN_POINT('Ctrl Pts',(1.96727213799507,-1.,-3.5903336402273));
#69946=CARTESIAN_POINT('Ctrl Pts',(1.96727213799507,1.,-3.5903336402273));
#69947=CARTESIAN_POINT('Ctrl Pts',(1.96797854118257,-1.,-3.59803959819725));
#69948=CARTESIAN_POINT('Ctrl Pts',(1.96797854118257,1.,-3.59803959819725));
#69949=CARTESIAN_POINT('Ctrl Pts',(1.96864911885775,-1.,-3.60575714017676));
#69950=CARTESIAN_POINT('Ctrl Pts',(1.96864911885775,1.,-3.60575714017676));
#69951=CARTESIAN_POINT('Ctrl Pts',(1.96928416040712,-1.,-3.61348615496393));
#69952=CARTESIAN_POINT('Ctrl Pts',(1.96928416040712,1.,-3.61348615496393));
#69953=CARTESIAN_POINT('Ctrl Pts',(1.96988398129888,-1.,-3.62122658401722));
#69954=CARTESIAN_POINT('Ctrl Pts',(1.96988398129888,1.,-3.62122658401722));
#69955=CARTESIAN_POINT('Ctrl Pts',(1.97044889850518,-1.,-3.62897836973397));
#69956=CARTESIAN_POINT('Ctrl Pts',(1.97044889850518,1.,-3.62897836973397));
#69957=CARTESIAN_POINT('Ctrl Pts',(1.97097920454698,-1.,-3.63674139590853));
#69958=CARTESIAN_POINT('Ctrl Pts',(1.97097920454698,1.,-3.63674139590853));
#69959=CARTESIAN_POINT('Ctrl Pts',(1.97147515441539,-1.,-3.64451546724222));
#69960=CARTESIAN_POINT('Ctrl Pts',(1.97147515441539,1.,-3.64451546724222));
#69961=CARTESIAN_POINT('Ctrl Pts',(1.97193697240645,-1.,-3.65230034717364));
#69962=CARTESIAN_POINT('Ctrl Pts',(1.97193697240645,1.,-3.65230034717364));
#69963=CARTESIAN_POINT('Ctrl Pts',(1.97236485439317,-1.,-3.66009578166865));
#69964=CARTESIAN_POINT('Ctrl Pts',(1.97236485439317,1.,-3.66009578166865));
#69965=CARTESIAN_POINT('Ctrl Pts',(1.9727589719863,-1.,-3.66790152751984));
#69966=CARTESIAN_POINT('Ctrl Pts',(1.9727589719863,1.,-3.66790152751984));
#69967=CARTESIAN_POINT('Ctrl Pts',(1.97311947678035,-1.,-3.67571738106175));
#69968=CARTESIAN_POINT('Ctrl Pts',(1.97311947678035,1.,-3.67571738106175));
#69969=CARTESIAN_POINT('Ctrl Pts',(1.9734465030363,-1.,-3.68354319913416));
#69970=CARTESIAN_POINT('Ctrl Pts',(1.9734465030363,1.,-3.68354319913416));
#69971=CARTESIAN_POINT('Ctrl Pts',(1.97374016224397,-1.,-3.69137888597855));
#69972=CARTESIAN_POINT('Ctrl Pts',(1.97374016224397,1.,-3.69137888597855));
#69973=CARTESIAN_POINT('Ctrl Pts',(1.97394846382288,-1.,-3.69765528558292));
#69974=CARTESIAN_POINT('Ctrl Pts',(1.97394846382288,1.,-3.69765528558292));
#69975=CARTESIAN_POINT('Ctrl Pts',(1.97408973726149,-1.,-3.70236698911837));
#69976=CARTESIAN_POINT('Ctrl Pts',(1.97408973726149,1.,-3.70236698911837));
#69977=CARTESIAN_POINT('Ctrl Pts',(1.974177276451,-1.,-3.7055100813194));
#69978=CARTESIAN_POINT('Ctrl Pts',(1.974177276451,1.,-3.7055100813194));
#69979=CARTESIAN_POINT('Ctrl Pts',(1.97421938526992,-1.,-3.70708211654725));
#69980=CARTESIAN_POINT('Ctrl Pts',(1.97421938526992,1.,-3.70708211654725));
#69981=CARTESIAN_POINT('',(1.88097764062542,1.,-3.24413672884902));
#69982=CARTESIAN_POINT('Ctrl Pts',(1.88097764062541,-1.,-3.24413672884902));
#69983=CARTESIAN_POINT('Ctrl Pts',(1.88097764062541,-0.666666666666667,
-3.24413672884902));
#69984=CARTESIAN_POINT('Ctrl Pts',(1.88097764062541,-0.333333333333333,
-3.24413672884902));
#69985=CARTESIAN_POINT('Ctrl Pts',(1.88097764062541,0.333333333333333,-3.24413672884902));
#69986=CARTESIAN_POINT('Ctrl Pts',(1.88097764062541,0.666666666666667,-3.24413672884902));
#69987=CARTESIAN_POINT('Ctrl Pts',(1.88097764062541,1.,-3.24413672884902));
#69988=CARTESIAN_POINT('',(1.97421938526992,1.,-3.70708211654725));
#69989=CARTESIAN_POINT('',(1.97421938526992,0.,-3.70708211654725));
#69990=CARTESIAN_POINT('Ctrl Pts',(1.88097764062542,1.,-3.24413672884902));
#69991=CARTESIAN_POINT('Ctrl Pts',(1.88102292397987,1.,-3.24415531671311));
#69992=CARTESIAN_POINT('Ctrl Pts',(1.88117508446657,1.,-3.24428080352952));
#69993=CARTESIAN_POINT('Ctrl Pts',(1.88156537699118,1.,-3.24480754675942));
#69994=CARTESIAN_POINT('Ctrl Pts',(1.88242596600422,1.,-3.24625654410705));
#69995=CARTESIAN_POINT('Ctrl Pts',(1.88407708646435,1.,-3.24935200512055));
#69996=CARTESIAN_POINT('Ctrl Pts',(1.88646802523372,1.,-3.25408686339298));
#69997=CARTESIAN_POINT('Ctrl Pts',(1.88934996203508,1.,-3.2599988519361));
#69998=CARTESIAN_POINT('Ctrl Pts',(1.89255393500769,1.,-3.2667765388833));
#69999=CARTESIAN_POINT('Ctrl Pts',(1.89589172903662,1.,-3.27407108932908));
#70000=CARTESIAN_POINT('Ctrl Pts',(1.89918429230424,1.,-3.28154737912287));
#70001=CARTESIAN_POINT('Ctrl Pts',(1.9022897124757,1.,-3.28893448600364));
#70002=CARTESIAN_POINT('Ctrl Pts',(1.9051389186417,1.,-3.29608978722258));
#70003=CARTESIAN_POINT('Ctrl Pts',(1.90773912171424,1.,-3.30300595568341));
#70004=CARTESIAN_POINT('Ctrl Pts',(1.91014297830502,1.,-3.30975721158694));
#70005=CARTESIAN_POINT('Ctrl Pts',(1.91242616234459,1.,-3.31646052426395));
#70006=CARTESIAN_POINT('Ctrl Pts',(1.91466343916612,1.,-3.32323403454507));
#70007=CARTESIAN_POINT('Ctrl Pts',(1.91690081930297,1.,-3.33014884257812));
#70008=CARTESIAN_POINT('Ctrl Pts',(1.91914609610173,1.,-3.33721230709948));
#70009=CARTESIAN_POINT('Ctrl Pts',(1.92138450828378,1.,-3.34439448941915));
#70010=CARTESIAN_POINT('Ctrl Pts',(1.92358838440518,1.,-3.35164424847207));
#70011=CARTESIAN_POINT('Ctrl Pts',(1.92572846125763,1.,-3.35890824422976));
#70012=CARTESIAN_POINT('Ctrl Pts',(1.92778626543803,1.,-3.36615168657597));
#70013=CARTESIAN_POINT('Ctrl Pts',(1.92975993109897,1.,-3.37336807068078));
#70014=CARTESIAN_POINT('Ctrl Pts',(1.93165739093292,1.,-3.38056768525577));
#70015=CARTESIAN_POINT('Ctrl Pts',(1.93349233176794,1.,-3.38777076883267));
#70016=CARTESIAN_POINT('Ctrl Pts',(1.93527929945982,1.,-3.39499923640789));
#70017=CARTESIAN_POINT('Ctrl Pts',(1.93702857723089,1.,-3.40226802104093));
#70018=CARTESIAN_POINT('Ctrl Pts',(1.93874306008132,1.,-3.40957978266623));
#70019=CARTESIAN_POINT('Ctrl Pts',(1.94042111965237,1.,-3.41692971994082));
#70020=CARTESIAN_POINT('Ctrl Pts',(1.94205835913692,1.,-3.42430850941497));
#70021=CARTESIAN_POINT('Ctrl Pts',(1.94364973660285,1.,-3.43170586602436));
#70022=CARTESIAN_POINT('Ctrl Pts',(1.94519168842883,1.,-3.43911410197693));
#70023=CARTESIAN_POINT('Ctrl Pts',(1.94668377715332,1.,-3.44653088665685));
#70024=CARTESIAN_POINT('Ctrl Pts',(1.94812754766524,1.,-3.45395731584051));
#70025=CARTESIAN_POINT('Ctrl Pts',(1.94952575850196,1.,-3.46139661060959));
#70026=CARTESIAN_POINT('Ctrl Pts',(1.95088147859876,1.,-3.4688525897419));
#70027=CARTESIAN_POINT('Ctrl Pts',(1.95219722189878,1.,-3.47632820495926));
#70028=CARTESIAN_POINT('Ctrl Pts',(1.95347412486316,1.,-3.48382414832649));
#70029=CARTESIAN_POINT('Ctrl Pts',(1.95471236969653,1.,-3.49133956289154));
#70030=CARTESIAN_POINT('Ctrl Pts',(1.9559115382367,1.,-3.49887263575602));
#70031=CARTESIAN_POINT('Ctrl Pts',(1.95707099606513,1.,-3.50642124159913));
#70032=CARTESIAN_POINT('Ctrl Pts',(1.95819025316768,1.,-3.51398354617773));
#70033=CARTESIAN_POINT('Ctrl Pts',(1.95926936324436,1.,-3.52155867431438));
#70034=CARTESIAN_POINT('Ctrl Pts',(1.96030879411534,1.,-3.52914648844289));
#70035=CARTESIAN_POINT('Ctrl Pts',(1.96130926212661,1.,-3.53674730625759));
#70036=CARTESIAN_POINT('Ctrl Pts',(1.96227157573058,1.,-3.54436163300425));
#70037=CARTESIAN_POINT('Ctrl Pts',(1.96319648628667,1.,-3.55198990600929));
#70038=CARTESIAN_POINT('Ctrl Pts',(1.96408450906868,1.,-3.55963218706201));
#70039=CARTESIAN_POINT('Ctrl Pts',(1.96493594634643,1.,-3.56728820357933));
#70040=CARTESIAN_POINT('Ctrl Pts',(1.96575096652857,1.,-3.57495748601088));
#70041=CARTESIAN_POINT('Ctrl Pts',(1.9665296668894,1.,-3.58263947663884));
#70042=CARTESIAN_POINT('Ctrl Pts',(1.96727213799507,1.,-3.5903336402273));
#70043=CARTESIAN_POINT('Ctrl Pts',(1.96797854118257,1.,-3.59803959819725));
#70044=CARTESIAN_POINT('Ctrl Pts',(1.96864911885775,1.,-3.60575714017676));
#70045=CARTESIAN_POINT('Ctrl Pts',(1.96928416040712,1.,-3.61348615496393));
#70046=CARTESIAN_POINT('Ctrl Pts',(1.96988398129888,1.,-3.62122658401722));
#70047=CARTESIAN_POINT('Ctrl Pts',(1.97044889850518,1.,-3.62897836973397));
#70048=CARTESIAN_POINT('Ctrl Pts',(1.97097920454698,1.,-3.63674139590853));
#70049=CARTESIAN_POINT('Ctrl Pts',(1.97147515441539,1.,-3.64451546724222));
#70050=CARTESIAN_POINT('Ctrl Pts',(1.97193697240645,1.,-3.65230034717364));
#70051=CARTESIAN_POINT('Ctrl Pts',(1.97236485439317,1.,-3.66009578166865));
#70052=CARTESIAN_POINT('Ctrl Pts',(1.9727589719863,1.,-3.66790152751984));
#70053=CARTESIAN_POINT('Ctrl Pts',(1.97311947678035,1.,-3.67571738106175));
#70054=CARTESIAN_POINT('Ctrl Pts',(1.9734465030363,1.,-3.68354319913416));
#70055=CARTESIAN_POINT('Ctrl Pts',(1.97374016224397,1.,-3.69137888597855));
#70056=CARTESIAN_POINT('Ctrl Pts',(1.97394846382288,1.,-3.69765528558292));
#70057=CARTESIAN_POINT('Ctrl Pts',(1.97408973726149,1.,-3.70236698911837));
#70058=CARTESIAN_POINT('Ctrl Pts',(1.974177276451,1.,-3.7055100813194));
#70059=CARTESIAN_POINT('Ctrl Pts',(1.97421938526992,1.,-3.70708211654725));
#70060=CARTESIAN_POINT('Origin',(1.97421938526992,0.,-3.70708211654725));
#70061=CARTESIAN_POINT('',(1.83867539237861,1.,-3.77614523045147));
#70062=CARTESIAN_POINT('Origin',(0.,0.,0.));
#70063=CARTESIAN_POINT('',(2.03660101169564,1.,-3.14877060440425));
#70064=CARTESIAN_POINT('Origin',(0.,1.,0.));
#70065=CARTESIAN_POINT('Ctrl Pts',(2.03660101169564,1.,-3.14877060440425));
#70066=CARTESIAN_POINT('Ctrl Pts',(2.03660101169564,0.666666666666667,-3.14877060440425));
#70067=CARTESIAN_POINT('Ctrl Pts',(2.03660101169564,0.333333333333333,-3.14877060440425));
#70068=CARTESIAN_POINT('Ctrl Pts',(2.03660101169564,-0.333333333333333,
-3.14877060440425));
#70069=CARTESIAN_POINT('Ctrl Pts',(2.03660101169564,-0.666666666666667,
-3.14877060440425));
#70070=CARTESIAN_POINT('Ctrl Pts',(2.03660101169564,-1.,-3.14877060440425));
#70071=CARTESIAN_POINT('Ctrl Pts',(2.40675750623143,-1.,-3.44202241512147));
#70072=CARTESIAN_POINT('Ctrl Pts',(2.40675750623143,1.,-3.44202241512147));
#70073=CARTESIAN_POINT('Ctrl Pts',(2.40537592959345,-1.,-3.44127120683402));
#70074=CARTESIAN_POINT('Ctrl Pts',(2.40537592959345,1.,-3.44127120683402));
#70075=CARTESIAN_POINT('Ctrl Pts',(2.40261515590099,-1.,-3.43976627485223));
#70076=CARTESIAN_POINT('Ctrl Pts',(2.40261515590099,1.,-3.43976627485223));
#70077=CARTESIAN_POINT('Ctrl Pts',(2.39848113411428,-1.,-3.43750133066037));
#70078=CARTESIAN_POINT('Ctrl Pts',(2.39848113411428,1.,-3.43750133066037));
#70079=CARTESIAN_POINT('Ctrl Pts',(2.39298338805823,-1.,-3.43446630680436));
#70080=CARTESIAN_POINT('Ctrl Pts',(2.39298338805823,1.,-3.43446630680436));
#70081=CARTESIAN_POINT('Ctrl Pts',(2.38613505844641,-1.,-3.43064732714472));
#70082=CARTESIAN_POINT('Ctrl Pts',(2.38613505844641,1.,-3.43064732714472));
#70083=CARTESIAN_POINT('Ctrl Pts',(2.37931067029517,-1.,-3.42680309755241));
#70084=CARTESIAN_POINT('Ctrl Pts',(2.37931067029517,1.,-3.42680309755241));
#70085=CARTESIAN_POINT('Ctrl Pts',(2.37251035954351,-1.,-3.42293356216595));
#70086=CARTESIAN_POINT('Ctrl Pts',(2.37251035954351,1.,-3.42293356216595));
#70087=CARTESIAN_POINT('Ctrl Pts',(2.36573431470313,-1.,-3.41903866635384));
#70088=CARTESIAN_POINT('Ctrl Pts',(2.36573431470313,1.,-3.41903866635384));
#70089=CARTESIAN_POINT('Ctrl Pts',(2.35898278606449,-1.,-3.4151183675076));
#70090=CARTESIAN_POINT('Ctrl Pts',(2.35898278606449,1.,-3.4151183675076));
#70091=CARTESIAN_POINT('Ctrl Pts',(2.35225606823649,-1.,-3.41117262313464));
#70092=CARTESIAN_POINT('Ctrl Pts',(2.35225606823649,1.,-3.41117262313464));
#70093=CARTESIAN_POINT('Ctrl Pts',(2.34555447648901,-1.,-3.40720137403888));
#70094=CARTESIAN_POINT('Ctrl Pts',(2.34555447648901,1.,-3.40720137403888));
#70095=CARTESIAN_POINT('Ctrl Pts',(2.33887832342715,-1.,-3.40320452776646));
#70096=CARTESIAN_POINT('Ctrl Pts',(2.33887832342715,1.,-3.40320452776646));
#70097=CARTESIAN_POINT('Ctrl Pts',(2.33222789882601,-1.,-3.39918194578115));
#70098=CARTESIAN_POINT('Ctrl Pts',(2.33222789882601,1.,-3.39918194578115));
#70099=CARTESIAN_POINT('Ctrl Pts',(2.32560343902683,-1.,-3.39513342020045));
#70100=CARTESIAN_POINT('Ctrl Pts',(2.32560343902683,1.,-3.39513342020045));
#70101=CARTESIAN_POINT('Ctrl Pts',(2.31900513925627,-1.,-3.39105869475112));
#70102=CARTESIAN_POINT('Ctrl Pts',(2.31900513925627,1.,-3.39105869475112));
#70103=CARTESIAN_POINT('Ctrl Pts',(2.31243319489505,-1.,-3.38695751492659));
#70104=CARTESIAN_POINT('Ctrl Pts',(2.31243319489505,1.,-3.38695751492659));
#70105=CARTESIAN_POINT('Ctrl Pts',(2.30588783640389,-1.,-3.38282967336676));
#70106=CARTESIAN_POINT('Ctrl Pts',(2.30588783640389,1.,-3.38282967336676));
#70107=CARTESIAN_POINT('Ctrl Pts',(2.29936936127588,-1.,-3.37867504959382));
#70108=CARTESIAN_POINT('Ctrl Pts',(2.29936936127588,1.,-3.37867504959382));
#70109=CARTESIAN_POINT('Ctrl Pts',(2.2928781800731,-1.,-3.37449367172707));
#70110=CARTESIAN_POINT('Ctrl Pts',(2.2928781800731,1.,-3.37449367172707));
#70111=CARTESIAN_POINT('Ctrl Pts',(2.28641481081045,-1.,-3.37028570206357));
#70112=CARTESIAN_POINT('Ctrl Pts',(2.28641481081045,1.,-3.37028570206357));
#70113=CARTESIAN_POINT('Ctrl Pts',(2.27997979457968,-1.,-3.36605130712978));
#70114=CARTESIAN_POINT('Ctrl Pts',(2.27997979457968,1.,-3.36605130712978));
#70115=CARTESIAN_POINT('Ctrl Pts',(2.27357362620902,-1.,-3.36179055004369));
#70116=CARTESIAN_POINT('Ctrl Pts',(2.27357362620902,1.,-3.36179055004369));
#70117=CARTESIAN_POINT('Ctrl Pts',(2.26719668579921,-1.,-3.35750328523077));
#70118=CARTESIAN_POINT('Ctrl Pts',(2.26719668579921,1.,-3.35750328523077));
#70119=CARTESIAN_POINT('Ctrl Pts',(2.26084915222484,-1.,-3.35318902552676));
#70120=CARTESIAN_POINT('Ctrl Pts',(2.26084915222484,1.,-3.35318902552676));
#70121=CARTESIAN_POINT('Ctrl Pts',(2.25453097693524,-1.,-3.34884690292342));
#70122=CARTESIAN_POINT('Ctrl Pts',(2.25453097693524,1.,-3.34884690292342));
#70123=CARTESIAN_POINT('Ctrl Pts',(2.24824207678287,-1.,-3.34447596770768));
#70124=CARTESIAN_POINT('Ctrl Pts',(2.24824207678287,1.,-3.34447596770768));
#70125=CARTESIAN_POINT('Ctrl Pts',(2.24198249391437,-1.,-3.34007543738044));
#70126=CARTESIAN_POINT('Ctrl Pts',(2.24198249391437,1.,-3.34007543738044));
#70127=CARTESIAN_POINT('Ctrl Pts',(2.23575256328809,-1.,-3.33564495756478));
#70128=CARTESIAN_POINT('Ctrl Pts',(2.23575256328809,1.,-3.33564495756478));
#70129=CARTESIAN_POINT('Ctrl Pts',(2.22955308907221,-1.,-3.33118487773593));
#70130=CARTESIAN_POINT('Ctrl Pts',(2.22955308907221,1.,-3.33118487773593));
#70131=CARTESIAN_POINT('Ctrl Pts',(2.22338548312758,-1.,-3.32669646722871));
#70132=CARTESIAN_POINT('Ctrl Pts',(2.22338548312758,1.,-3.32669646722871));
#70133=CARTESIAN_POINT('Ctrl Pts',(2.21725135110889,-1.,-3.32218125618955));
#70134=CARTESIAN_POINT('Ctrl Pts',(2.21725135110889,1.,-3.32218125618955));
#70135=CARTESIAN_POINT('Ctrl Pts',(2.21115211847872,-1.,-3.31764044024231));
#70136=CARTESIAN_POINT('Ctrl Pts',(2.21115211847872,1.,-3.31764044024231));
#70137=CARTESIAN_POINT('Ctrl Pts',(2.20508863150608,-1.,-3.3130742460895));
#70138=CARTESIAN_POINT('Ctrl Pts',(2.20508863150608,1.,-3.3130742460895));
#70139=CARTESIAN_POINT('Ctrl Pts',(2.19906078949924,-1.,-3.30848134694597));
#70140=CARTESIAN_POINT('Ctrl Pts',(2.19906078949924,1.,-3.30848134694597));
#70141=CARTESIAN_POINT('Ctrl Pts',(2.19306710376112,-1.,-3.30385816281831));
#70142=CARTESIAN_POINT('Ctrl Pts',(2.19306710376112,1.,-3.30385816281831));
#70143=CARTESIAN_POINT('Ctrl Pts',(2.18710556500325,-1.,-3.29920022557635));
#70144=CARTESIAN_POINT('Ctrl Pts',(2.18710556500325,1.,-3.29920022557635));
#70145=CARTESIAN_POINT('Ctrl Pts',(2.18117455557062,-1.,-3.29450361500484));
#70146=CARTESIAN_POINT('Ctrl Pts',(2.18117455557062,1.,-3.29450361500484));
#70147=CARTESIAN_POINT('Ctrl Pts',(2.17527380048422,-1.,-3.28976645712566));
#70148=CARTESIAN_POINT('Ctrl Pts',(2.17527380048422,1.,-3.28976645712566));
#70149=CARTESIAN_POINT('Ctrl Pts',(2.16940517773459,-1.,-3.2849901997973));
#70150=CARTESIAN_POINT('Ctrl Pts',(2.16940517773459,1.,-3.2849901997973));
#70151=CARTESIAN_POINT('Ctrl Pts',(2.16357391934434,-1.,-3.28018150841414));
#70152=CARTESIAN_POINT('Ctrl Pts',(2.16357391934434,1.,-3.28018150841414));
#70153=CARTESIAN_POINT('Ctrl Pts',(2.15778690038359,-1.,-3.27534954469206));
#70154=CARTESIAN_POINT('Ctrl Pts',(2.15778690038359,1.,-3.27534954469206));
#70155=CARTESIAN_POINT('Ctrl Pts',(2.15205043199818,-1.,-3.27050245897244));
#70156=CARTESIAN_POINT('Ctrl Pts',(2.15205043199818,1.,-3.27050245897244));
#70157=CARTESIAN_POINT('Ctrl Pts',(2.14636805295663,-1.,-3.26564388189764));
#70158=CARTESIAN_POINT('Ctrl Pts',(2.14636805295663,1.,-3.26564388189764));
#70159=CARTESIAN_POINT('Ctrl Pts',(2.14073870754257,-1.,-3.26077002641868));
#70160=CARTESIAN_POINT('Ctrl Pts',(2.14073870754257,1.,-3.26077002641868));
#70161=CARTESIAN_POINT('Ctrl Pts',(2.13515375878786,-1.,-3.25586495065027));
#70162=CARTESIAN_POINT('Ctrl Pts',(2.13515375878786,1.,-3.25586495065027));
#70163=CARTESIAN_POINT('Ctrl Pts',(2.1296002839681,-1.,-3.25090574493994));
#70164=CARTESIAN_POINT('Ctrl Pts',(2.1296002839681,1.,-3.25090574493994));
#70165=CARTESIAN_POINT('Ctrl Pts',(2.12406646410943,-1.,-3.24587102613347));
#70166=CARTESIAN_POINT('Ctrl Pts',(2.12406646410943,1.,-3.24587102613347));
#70167=CARTESIAN_POINT('Ctrl Pts',(2.11854673326972,-1.,-3.24074905517282));
#70168=CARTESIAN_POINT('Ctrl Pts',(2.11854673326972,1.,-3.24074905517282));
#70169=CARTESIAN_POINT('Ctrl Pts',(2.11304604021784,-1.,-3.23554444767115));
#70170=CARTESIAN_POINT('Ctrl Pts',(2.11304604021784,1.,-3.23554444767115));
#70171=CARTESIAN_POINT('Ctrl Pts',(2.1075869964248,-1.,-3.23028945793334));
#70172=CARTESIAN_POINT('Ctrl Pts',(2.1075869964248,1.,-3.23028945793334));
#70173=CARTESIAN_POINT('Ctrl Pts',(2.10220384298533,-1.,-3.22503437553496));
#70174=CARTESIAN_POINT('Ctrl Pts',(2.10220384298533,1.,-3.22503437553496));
#70175=CARTESIAN_POINT('Ctrl Pts',(2.09692958434933,-1.,-3.21982707347067));
#70176=CARTESIAN_POINT('Ctrl Pts',(2.09692958434933,1.,-3.21982707347067));
#70177=CARTESIAN_POINT('Ctrl Pts',(2.0917841946046,-1.,-3.2146942960168));
#70178=CARTESIAN_POINT('Ctrl Pts',(2.0917841946046,1.,-3.2146942960168));
#70179=CARTESIAN_POINT('Ctrl Pts',(2.08676465517435,-1.,-3.20962575845433));
#70180=CARTESIAN_POINT('Ctrl Pts',(2.08676465517435,1.,-3.20962575845433));
#70181=CARTESIAN_POINT('Ctrl Pts',(2.08182850370816,-1.,-3.20454818630635));
#70182=CARTESIAN_POINT('Ctrl Pts',(2.08182850370816,1.,-3.20454818630635));
#70183=CARTESIAN_POINT('Ctrl Pts',(2.0769044187063,-1.,-3.19934132835879));
#70184=CARTESIAN_POINT('Ctrl Pts',(2.0769044187063,1.,-3.19934132835879));
#70185=CARTESIAN_POINT('Ctrl Pts',(2.07192253497765,-1.,-3.19388465568113));
#70186=CARTESIAN_POINT('Ctrl Pts',(2.07192253497765,1.,-3.19388465568113));
#70187=CARTESIAN_POINT('Ctrl Pts',(2.06684062744065,-1.,-3.18809755562297));
#70188=CARTESIAN_POINT('Ctrl Pts',(2.06684062744065,1.,-3.18809755562297));
#70189=CARTESIAN_POINT('Ctrl Pts',(2.06166849827143,-1.,-3.18197692964677));
#70190=CARTESIAN_POINT('Ctrl Pts',(2.06166849827143,1.,-3.18197692964677));
#70191=CARTESIAN_POINT('Ctrl Pts',(2.05650186773279,-1.,-3.17564906975592));
#70192=CARTESIAN_POINT('Ctrl Pts',(2.05650186773279,1.,-3.17564906975592));
#70193=CARTESIAN_POINT('Ctrl Pts',(2.05151770247452,-1.,-3.16936341689859));
#70194=CARTESIAN_POINT('Ctrl Pts',(2.05151770247452,1.,-3.16936341689859));
#70195=CARTESIAN_POINT('Ctrl Pts',(2.0469333124766,-1.,-3.16343165059235));
#70196=CARTESIAN_POINT('Ctrl Pts',(2.0469333124766,1.,-3.16343165059235));
#70197=CARTESIAN_POINT('Ctrl Pts',(2.04297406404132,-1.,-3.15817983946525));
#70198=CARTESIAN_POINT('Ctrl Pts',(2.04297406404132,1.,-3.15817983946525));
#70199=CARTESIAN_POINT('Ctrl Pts',(2.03984073791432,-1.,-3.1538999167466));
#70200=CARTESIAN_POINT('Ctrl Pts',(2.03984073791432,1.,-3.1538999167466));
#70201=CARTESIAN_POINT('Ctrl Pts',(2.03766932526171,-1.,-3.15079010635326));
#70202=CARTESIAN_POINT('Ctrl Pts',(2.03766932526171,1.,-3.15079010635326));
#70203=CARTESIAN_POINT('Ctrl Pts',(2.03675273048882,-1.,-3.14931281967585));
#70204=CARTESIAN_POINT('Ctrl Pts',(2.03675273048882,1.,-3.14931281967585));
#70205=CARTESIAN_POINT('Ctrl Pts',(2.03653654935384,-1.,-3.14878756590499));
#70206=CARTESIAN_POINT('Ctrl Pts',(2.03653654935384,1.,-3.14878756590499));
#70207=CARTESIAN_POINT('Ctrl Pts',(2.036601737578,-1.,-3.14869618937139));
#70208=CARTESIAN_POINT('Ctrl Pts',(2.036601737578,1.,-3.14869618937139));
#70209=CARTESIAN_POINT('Ctrl Pts',(2.03668666247593,-1.,-3.1487152044751));
#70210=CARTESIAN_POINT('Ctrl Pts',(2.03668666247593,1.,-3.1487152044751));
#70211=CARTESIAN_POINT('',(2.40675750623143,1.,-3.44202241512147));
#70212=CARTESIAN_POINT('Ctrl Pts',(2.40675750623143,1.,-3.44202241512147));
#70213=CARTESIAN_POINT('Ctrl Pts',(2.40537592959345,1.,-3.44127120683402));
#70214=CARTESIAN_POINT('Ctrl Pts',(2.40261515590099,1.,-3.43976627485223));
#70215=CARTESIAN_POINT('Ctrl Pts',(2.39848113411428,1.,-3.43750133066037));
#70216=CARTESIAN_POINT('Ctrl Pts',(2.39298338805823,1.,-3.43446630680436));
#70217=CARTESIAN_POINT('Ctrl Pts',(2.38613505844641,1.,-3.43064732714472));
#70218=CARTESIAN_POINT('Ctrl Pts',(2.37931067029517,1.,-3.42680309755241));
#70219=CARTESIAN_POINT('Ctrl Pts',(2.37251035954351,1.,-3.42293356216595));
#70220=CARTESIAN_POINT('Ctrl Pts',(2.36573431470313,1.,-3.41903866635384));
#70221=CARTESIAN_POINT('Ctrl Pts',(2.35898278606449,1.,-3.4151183675076));
#70222=CARTESIAN_POINT('Ctrl Pts',(2.35225606823649,1.,-3.41117262313464));
#70223=CARTESIAN_POINT('Ctrl Pts',(2.34555447648901,1.,-3.40720137403888));
#70224=CARTESIAN_POINT('Ctrl Pts',(2.33887832342715,1.,-3.40320452776646));
#70225=CARTESIAN_POINT('Ctrl Pts',(2.33222789882601,1.,-3.39918194578115));
#70226=CARTESIAN_POINT('Ctrl Pts',(2.32560343902683,1.,-3.39513342020045));
#70227=CARTESIAN_POINT('Ctrl Pts',(2.31900513925627,1.,-3.39105869475112));
#70228=CARTESIAN_POINT('Ctrl Pts',(2.31243319489505,1.,-3.38695751492659));
#70229=CARTESIAN_POINT('Ctrl Pts',(2.30588783640389,1.,-3.38282967336676));
#70230=CARTESIAN_POINT('Ctrl Pts',(2.29936936127588,1.,-3.37867504959382));
#70231=CARTESIAN_POINT('Ctrl Pts',(2.2928781800731,1.,-3.37449367172707));
#70232=CARTESIAN_POINT('Ctrl Pts',(2.28641481081045,1.,-3.37028570206357));
#70233=CARTESIAN_POINT('Ctrl Pts',(2.27997979457968,1.,-3.36605130712978));
#70234=CARTESIAN_POINT('Ctrl Pts',(2.27357362620902,1.,-3.36179055004369));
#70235=CARTESIAN_POINT('Ctrl Pts',(2.26719668579921,1.,-3.35750328523077));
#70236=CARTESIAN_POINT('Ctrl Pts',(2.26084915222484,1.,-3.35318902552676));
#70237=CARTESIAN_POINT('Ctrl Pts',(2.25453097693524,1.,-3.34884690292342));
#70238=CARTESIAN_POINT('Ctrl Pts',(2.24824207678287,1.,-3.34447596770768));
#70239=CARTESIAN_POINT('Ctrl Pts',(2.24198249391437,1.,-3.34007543738044));
#70240=CARTESIAN_POINT('Ctrl Pts',(2.23575256328809,1.,-3.33564495756478));
#70241=CARTESIAN_POINT('Ctrl Pts',(2.22955308907221,1.,-3.33118487773593));
#70242=CARTESIAN_POINT('Ctrl Pts',(2.22338548312758,1.,-3.32669646722871));
#70243=CARTESIAN_POINT('Ctrl Pts',(2.21725135110889,1.,-3.32218125618955));
#70244=CARTESIAN_POINT('Ctrl Pts',(2.21115211847872,1.,-3.31764044024231));
#70245=CARTESIAN_POINT('Ctrl Pts',(2.20508863150608,1.,-3.3130742460895));
#70246=CARTESIAN_POINT('Ctrl Pts',(2.19906078949924,1.,-3.30848134694597));
#70247=CARTESIAN_POINT('Ctrl Pts',(2.19306710376112,1.,-3.30385816281831));
#70248=CARTESIAN_POINT('Ctrl Pts',(2.18710556500325,1.,-3.29920022557635));
#70249=CARTESIAN_POINT('Ctrl Pts',(2.18117455557062,1.,-3.29450361500484));
#70250=CARTESIAN_POINT('Ctrl Pts',(2.17527380048422,1.,-3.28976645712566));
#70251=CARTESIAN_POINT('Ctrl Pts',(2.16940517773459,1.,-3.2849901997973));
#70252=CARTESIAN_POINT('Ctrl Pts',(2.16357391934434,1.,-3.28018150841414));
#70253=CARTESIAN_POINT('Ctrl Pts',(2.15778690038359,1.,-3.27534954469206));
#70254=CARTESIAN_POINT('Ctrl Pts',(2.15205043199818,1.,-3.27050245897244));
#70255=CARTESIAN_POINT('Ctrl Pts',(2.14636805295663,1.,-3.26564388189764));
#70256=CARTESIAN_POINT('Ctrl Pts',(2.14073870754257,1.,-3.26077002641868));
#70257=CARTESIAN_POINT('Ctrl Pts',(2.13515375878786,1.,-3.25586495065027));
#70258=CARTESIAN_POINT('Ctrl Pts',(2.1296002839681,1.,-3.25090574493994));
#70259=CARTESIAN_POINT('Ctrl Pts',(2.12406646410943,1.,-3.24587102613347));
#70260=CARTESIAN_POINT('Ctrl Pts',(2.11854673326972,1.,-3.24074905517282));
#70261=CARTESIAN_POINT('Ctrl Pts',(2.11304604021784,1.,-3.23554444767115));
#70262=CARTESIAN_POINT('Ctrl Pts',(2.1075869964248,1.,-3.23028945793334));
#70263=CARTESIAN_POINT('Ctrl Pts',(2.10220384298533,1.,-3.22503437553496));
#70264=CARTESIAN_POINT('Ctrl Pts',(2.09692958434933,1.,-3.21982707347067));
#70265=CARTESIAN_POINT('Ctrl Pts',(2.0917841946046,1.,-3.2146942960168));
#70266=CARTESIAN_POINT('Ctrl Pts',(2.08676465517435,1.,-3.20962575845433));
#70267=CARTESIAN_POINT('Ctrl Pts',(2.08182850370816,1.,-3.20454818630635));
#70268=CARTESIAN_POINT('Ctrl Pts',(2.0769044187063,1.,-3.19934132835879));
#70269=CARTESIAN_POINT('Ctrl Pts',(2.07192253497765,1.,-3.19388465568113));
#70270=CARTESIAN_POINT('Ctrl Pts',(2.06684062744065,1.,-3.18809755562297));
#70271=CARTESIAN_POINT('Ctrl Pts',(2.06166849827143,1.,-3.18197692964677));
#70272=CARTESIAN_POINT('Ctrl Pts',(2.05650186773279,1.,-3.17564906975592));
#70273=CARTESIAN_POINT('Ctrl Pts',(2.05151770247452,1.,-3.16936341689859));
#70274=CARTESIAN_POINT('Ctrl Pts',(2.0469333124766,1.,-3.16343165059235));
#70275=CARTESIAN_POINT('Ctrl Pts',(2.04297406404132,1.,-3.15817983946525));
#70276=CARTESIAN_POINT('Ctrl Pts',(2.03984073791432,1.,-3.1538999167466));
#70277=CARTESIAN_POINT('Ctrl Pts',(2.03783225496023,1.,-3.15102344775396));
#70278=CARTESIAN_POINT('Ctrl Pts',(2.03693188810614,1.,-3.14959882629936));
#70279=CARTESIAN_POINT('Ctrl Pts',(2.03663974554941,1.,-3.14901193669147));
#70280=CARTESIAN_POINT('Ctrl Pts',(2.03659701539175,1.,-3.1488193908823));
#70281=CARTESIAN_POINT('Ctrl Pts',(2.03660101169564,1.,-3.14877060440425));
#70282=CARTESIAN_POINT('',(2.40675750623143,0.,-3.44202241512147));
#70283=CARTESIAN_POINT('Ctrl Pts',(2.36523532225181,-1.,-2.91001063062876));
#70284=CARTESIAN_POINT('Ctrl Pts',(2.36523532225181,1.,-2.91001063062876));
#70285=CARTESIAN_POINT('Ctrl Pts',(2.36524348105112,-1.,-2.90992398626211));
#70286=CARTESIAN_POINT('Ctrl Pts',(2.36524348105112,1.,-2.90992398626211));
#70287=CARTESIAN_POINT('Ctrl Pts',(2.36535052956938,-1.,-2.90989022548032));
#70288=CARTESIAN_POINT('Ctrl Pts',(2.36535052956938,1.,-2.90989022548032));
#70289=CARTESIAN_POINT('Ctrl Pts',(2.36578327194741,-1.,-2.91025813830041));
#70290=CARTESIAN_POINT('Ctrl Pts',(2.36578327194741,1.,-2.91025813830041));
#70291=CARTESIAN_POINT('Ctrl Pts',(2.36690501170627,-1.,-2.9115863784204));
#70292=CARTESIAN_POINT('Ctrl Pts',(2.36690501170627,1.,-2.9115863784204));
#70293=CARTESIAN_POINT('Ctrl Pts',(2.36919161373173,-1.,-2.9146124988314));
#70294=CARTESIAN_POINT('Ctrl Pts',(2.36919161373173,1.,-2.9146124988314));
#70295=CARTESIAN_POINT('Ctrl Pts',(2.37229381109821,-1.,-2.91891503791411));
#70296=CARTESIAN_POINT('Ctrl Pts',(2.37229381109821,1.,-2.91891503791411));
#70297=CARTESIAN_POINT('Ctrl Pts',(2.3760651052403,-1.,-2.92430340582608));
#70298=CARTESIAN_POINT('Ctrl Pts',(2.3760651052403,1.,-2.92430340582608));
#70299=CARTESIAN_POINT('Ctrl Pts',(2.38028989582073,-1.,-2.93049643640206));
#70300=CARTESIAN_POINT('Ctrl Pts',(2.38028989582073,1.,-2.93049643640206));
#70301=CARTESIAN_POINT('Ctrl Pts',(2.38472771516311,-1.,-2.93717903280391));
#70302=CARTESIAN_POINT('Ctrl Pts',(2.38472771516311,1.,-2.93717903280391));
#70303=CARTESIAN_POINT('Ctrl Pts',(2.38914929090759,-1.,-2.94404820669076));
#70304=CARTESIAN_POINT('Ctrl Pts',(2.38914929090759,1.,-2.94404820669076));
#70305=CARTESIAN_POINT('Ctrl Pts',(2.39337207631667,-1.,-2.95085857128439));
#70306=CARTESIAN_POINT('Ctrl Pts',(2.39337207631667,1.,-2.95085857128439));
#70307=CARTESIAN_POINT('Ctrl Pts',(2.39730553974516,-1.,-2.95748006482942));
#70308=CARTESIAN_POINT('Ctrl Pts',(2.39730553974516,1.,-2.95748006482942));
#70309=CARTESIAN_POINT('Ctrl Pts',(2.4009556571164,-1.,-2.96390432240312));
#70310=CARTESIAN_POINT('Ctrl Pts',(2.4009556571164,1.,-2.96390432240312));
#70311=CARTESIAN_POINT('Ctrl Pts',(2.40438604734919,-1.,-2.9701964131236));
#70312=CARTESIAN_POINT('Ctrl Pts',(2.40438604734919,1.,-2.9701964131236));
#70313=CARTESIAN_POINT('Ctrl Pts',(2.40768975073713,-1.,-2.97646002822422));
#70314=CARTESIAN_POINT('Ctrl Pts',(2.40768975073713,1.,-2.97646002822422));
#70315=CARTESIAN_POINT('Ctrl Pts',(2.41095909342571,-1.,-2.98280015815107));
#70316=CARTESIAN_POINT('Ctrl Pts',(2.41095909342571,1.,-2.98280015815107));
#70317=CARTESIAN_POINT('Ctrl Pts',(2.41425064199586,-1.,-2.98927983005796));
#70318=CARTESIAN_POINT('Ctrl Pts',(2.41425064199586,1.,-2.98927983005796));
#70319=CARTESIAN_POINT('Ctrl Pts',(2.41757324500514,-1.,-2.99590509293503));
#70320=CARTESIAN_POINT('Ctrl Pts',(2.41757324500514,1.,-2.99590509293503));
#70321=CARTESIAN_POINT('Ctrl Pts',(2.42090763946779,-1.,-3.00264868585996));
#70322=CARTESIAN_POINT('Ctrl Pts',(2.42090763946779,1.,-3.00264868585996));
#70323=CARTESIAN_POINT('Ctrl Pts',(2.42421849439613,-1.,-3.00946442616659));
#70324=CARTESIAN_POINT('Ctrl Pts',(2.42421849439613,1.,-3.00946442616659));
#70325=CARTESIAN_POINT('Ctrl Pts',(2.42746856264168,-1.,-3.01630420830504));
#70326=CARTESIAN_POINT('Ctrl Pts',(2.42746856264168,1.,-3.01630420830504));
#70327=CARTESIAN_POINT('Ctrl Pts',(2.43063415586637,-1.,-3.02313656036004));
#70328=CARTESIAN_POINT('Ctrl Pts',(2.43063415586637,1.,-3.02313656036004));
#70329=CARTESIAN_POINT('Ctrl Pts',(2.43371241361488,-1.,-3.02995534946978));
#70330=CARTESIAN_POINT('Ctrl Pts',(2.43371241361488,1.,-3.02995534946978));
#70331=CARTESIAN_POINT('Ctrl Pts',(2.43671278042414,-1.,-3.03676949672822));
#70332=CARTESIAN_POINT('Ctrl Pts',(2.43671278042414,1.,-3.03676949672822));
#70333=CARTESIAN_POINT('Ctrl Pts',(2.43965194061857,-1.,-3.04359685040555));
#70334=CARTESIAN_POINT('Ctrl Pts',(2.43965194061857,1.,-3.04359685040555));
#70335=CARTESIAN_POINT('Ctrl Pts',(2.44254768923105,-1.,-3.05045678021504));
#70336=CARTESIAN_POINT('Ctrl Pts',(2.44254768923105,1.,-3.05045678021504));
#70337=CARTESIAN_POINT('Ctrl Pts',(2.44541251892556,-1.,-3.05736242671506));
#70338=CARTESIAN_POINT('Ctrl Pts',(2.44541251892556,1.,-3.05736242671506));
#70339=CARTESIAN_POINT('Ctrl Pts',(2.44824970516543,-1.,-3.06431596421405));
#70340=CARTESIAN_POINT('Ctrl Pts',(2.44824970516543,1.,-3.06431596421405));
#70341=CARTESIAN_POINT('Ctrl Pts',(2.45105688854422,-1.,-3.07131290521297));
#70342=CARTESIAN_POINT('Ctrl Pts',(2.45105688854422,1.,-3.07131290521297));
#70343=CARTESIAN_POINT('Ctrl Pts',(2.4538282678779,-1.,-3.07834472886139));
#70344=CARTESIAN_POINT('Ctrl Pts',(2.4538282678779,1.,-3.07834472886139));
#70345=CARTESIAN_POINT('Ctrl Pts',(2.45655725437039,-1.,-3.08540206545315));
#70346=CARTESIAN_POINT('Ctrl Pts',(2.45655725437039,1.,-3.08540206545315));
#70347=CARTESIAN_POINT('Ctrl Pts',(2.4592391256388,-1.,-3.09247787931887));
#70348=CARTESIAN_POINT('Ctrl Pts',(2.4592391256388,1.,-3.09247787931887));
#70349=CARTESIAN_POINT('Ctrl Pts',(2.46187308501884,-1.,-3.09956993697052));
#70350=CARTESIAN_POINT('Ctrl Pts',(2.46187308501884,1.,-3.09956993697052));
#70351=CARTESIAN_POINT('Ctrl Pts',(2.46446082979646,-1.,-3.1066790790198));
#70352=CARTESIAN_POINT('Ctrl Pts',(2.46446082979646,1.,-3.1066790790198));
#70353=CARTESIAN_POINT('Ctrl Pts',(2.46700558843506,-1.,-3.11380805536122));
#70354=CARTESIAN_POINT('Ctrl Pts',(2.46700558843506,1.,-3.11380805536122));
#70355=CARTESIAN_POINT('Ctrl Pts',(2.46951098947469,-1.,-3.12096015766983));
#70356=CARTESIAN_POINT('Ctrl Pts',(2.46951098947469,1.,-3.12096015766983));
#70357=CARTESIAN_POINT('Ctrl Pts',(2.47197997765871,-1.,-3.12813790805952));
#70358=CARTESIAN_POINT('Ctrl Pts',(2.47197997765871,1.,-3.12813790805952));
#70359=CARTESIAN_POINT('Ctrl Pts',(2.47441378371932,-1.,-3.13534181229295));
#70360=CARTESIAN_POINT('Ctrl Pts',(2.47441378371932,1.,-3.13534181229295));
#70361=CARTESIAN_POINT('Ctrl Pts',(2.47681245356109,-1.,-3.1425709954655));
#70362=CARTESIAN_POINT('Ctrl Pts',(2.47681245356109,1.,-3.1425709954655));
#70363=CARTESIAN_POINT('Ctrl Pts',(2.47917529057029,-1.,-3.14982373241352));
#70364=CARTESIAN_POINT('Ctrl Pts',(2.47917529057029,1.,-3.14982373241352));
#70365=CARTESIAN_POINT('Ctrl Pts',(2.48150133566571,-1.,-3.15709802322739));
#70366=CARTESIAN_POINT('Ctrl Pts',(2.48150133566571,1.,-3.15709802322739));
#70367=CARTESIAN_POINT('Ctrl Pts',(2.48378981792725,-1.,-3.16439213290161));
#70368=CARTESIAN_POINT('Ctrl Pts',(2.48378981792725,1.,-3.16439213290161));
#70369=CARTESIAN_POINT('Ctrl Pts',(2.48604065348587,-1.,-3.17170518863313));
#70370=CARTESIAN_POINT('Ctrl Pts',(2.48604065348587,1.,-3.17170518863313));
#70371=CARTESIAN_POINT('Ctrl Pts',(2.48825428288201,-1.,-3.17903698136622));
#70372=CARTESIAN_POINT('Ctrl Pts',(2.48825428288201,1.,-3.17903698136622));
#70373=CARTESIAN_POINT('Ctrl Pts',(2.49043146334059,-1.,-3.18638771282266));
#70374=CARTESIAN_POINT('Ctrl Pts',(2.49043146334059,1.,-3.18638771282266));
#70375=CARTESIAN_POINT('Ctrl Pts',(2.49257307239848,-1.,-3.19375775555798));
#70376=CARTESIAN_POINT('Ctrl Pts',(2.49257307239848,1.,-3.19375775555798));
#70377=CARTESIAN_POINT('Ctrl Pts',(2.49467992057755,-1.,-3.20114742397588));
#70378=CARTESIAN_POINT('Ctrl Pts',(2.49467992057755,1.,-3.20114742397588));
#70379=CARTESIAN_POINT('Ctrl Pts',(2.4967525264737,-1.,-3.20855669849836));
#70380=CARTESIAN_POINT('Ctrl Pts',(2.4967525264737,1.,-3.20855669849836));
#70381=CARTESIAN_POINT('Ctrl Pts',(2.4987911459939,-1.,-3.21598526261286));
#70382=CARTESIAN_POINT('Ctrl Pts',(2.4987911459939,1.,-3.21598526261286));
#70383=CARTESIAN_POINT('Ctrl Pts',(2.50079587201957,-1.,-3.22343262620503));
#70384=CARTESIAN_POINT('Ctrl Pts',(2.50079587201957,1.,-3.22343262620503));
#70385=CARTESIAN_POINT('Ctrl Pts',(2.50276671338111,-1.,-3.23089822320646));
#70386=CARTESIAN_POINT('Ctrl Pts',(2.50276671338111,1.,-3.23089822320646));
#70387=CARTESIAN_POINT('Ctrl Pts',(2.5047036758003,-1.,-3.23838151080319));
#70388=CARTESIAN_POINT('Ctrl Pts',(2.5047036758003,1.,-3.23838151080319));
#70389=CARTESIAN_POINT('Ctrl Pts',(2.506606859405,-1.,-3.24588208983849));
#70390=CARTESIAN_POINT('Ctrl Pts',(2.506606859405,1.,-3.24588208983849));
#70391=CARTESIAN_POINT('Ctrl Pts',(2.50847647070723,-1.,-3.25339971460982));
#70392=CARTESIAN_POINT('Ctrl Pts',(2.50847647070723,1.,-3.25339971460982));
#70393=CARTESIAN_POINT('Ctrl Pts',(2.51031277813486,-1.,-3.26093423001434));
#70394=CARTESIAN_POINT('Ctrl Pts',(2.51031277813486,1.,-3.26093423001434));
#70395=CARTESIAN_POINT('Ctrl Pts',(2.51211608411423,-1.,-3.26848552888116));
#70396=CARTESIAN_POINT('Ctrl Pts',(2.51211608411423,1.,-3.26848552888116));
#70397=CARTESIAN_POINT('Ctrl Pts',(2.513886692704,-1.,-3.27605350473142));
#70398=CARTESIAN_POINT('Ctrl Pts',(2.513886692704,1.,-3.27605350473142));
#70399=CARTESIAN_POINT('Ctrl Pts',(2.51562487464514,-1.,-3.28363799702982));
#70400=CARTESIAN_POINT('Ctrl Pts',(2.51562487464514,1.,-3.28363799702982));
#70401=CARTESIAN_POINT('Ctrl Pts',(2.51733085123797,-1.,-3.2912387729927));
#70402=CARTESIAN_POINT('Ctrl Pts',(2.51733085123797,1.,-3.2912387729927));
#70403=CARTESIAN_POINT('Ctrl Pts',(2.51900480701068,-1.,-3.29885556388353));
#70404=CARTESIAN_POINT('Ctrl Pts',(2.51900480701068,1.,-3.29885556388353));
#70405=CARTESIAN_POINT('Ctrl Pts',(2.52064689568511,-1.,-3.30648808815443));
#70406=CARTESIAN_POINT('Ctrl Pts',(2.52064689568511,1.,-3.30648808815443));
#70407=CARTESIAN_POINT('Ctrl Pts',(2.52225724871313,-1.,-3.31413607874645));
#70408=CARTESIAN_POINT('Ctrl Pts',(2.52225724871313,1.,-3.31413607874645));
#70409=CARTESIAN_POINT('Ctrl Pts',(2.5238359839626,-1.,-3.32179931078699));
#70410=CARTESIAN_POINT('Ctrl Pts',(2.5238359839626,1.,-3.32179931078699));
#70411=CARTESIAN_POINT('Ctrl Pts',(2.52538321164634,-1.,-3.32947762187533));
#70412=CARTESIAN_POINT('Ctrl Pts',(2.52538321164634,1.,-3.32947762187533));
#70413=CARTESIAN_POINT('Ctrl Pts',(2.52689902690158,-1.,-3.33717089999103));
#70414=CARTESIAN_POINT('Ctrl Pts',(2.52689902690158,1.,-3.33717089999103));
#70415=CARTESIAN_POINT('Ctrl Pts',(2.52808660915689,-1.,-3.34333744115511));
#70416=CARTESIAN_POINT('Ctrl Pts',(2.52808660915689,1.,-3.34333744115511));
#70417=CARTESIAN_POINT('Ctrl Pts',(2.52896321610703,-1.,-3.34796903576663));
#70418=CARTESIAN_POINT('Ctrl Pts',(2.52896321610703,1.,-3.34796903576663));
#70419=CARTESIAN_POINT('Ctrl Pts',(2.5295413654909,-1.,-3.35105973714072));
#70420=CARTESIAN_POINT('Ctrl Pts',(2.5295413654909,1.,-3.35105973714072));
#70421=CARTESIAN_POINT('Ctrl Pts',(2.52982887637028,-1.,-3.35260583073571));
#70422=CARTESIAN_POINT('Ctrl Pts',(2.52982887637028,1.,-3.35260583073571));
#70423=CARTESIAN_POINT('',(2.36531447826073,1.,-2.90994629141676));
#70424=CARTESIAN_POINT('Ctrl Pts',(2.36531447826073,-1.,-2.90994629141676));
#70425=CARTESIAN_POINT('Ctrl Pts',(2.36531447826073,-0.666666666666667,
-2.90994629141676));
#70426=CARTESIAN_POINT('Ctrl Pts',(2.36531447826073,-0.333333333333333,
-2.90994629141676));
#70427=CARTESIAN_POINT('Ctrl Pts',(2.36531447826073,0.333333333333333,-2.90994629141676));
#70428=CARTESIAN_POINT('Ctrl Pts',(2.36531447826074,0.666666666666667,-2.90994629141676));
#70429=CARTESIAN_POINT('Ctrl Pts',(2.36531447826074,1.,-2.90994629141676));
#70430=CARTESIAN_POINT('',(2.52982887637028,1.,-3.35260583073571));
#70431=CARTESIAN_POINT('',(2.52982887637028,0.,-3.35260583073571));
#70432=CARTESIAN_POINT('Ctrl Pts',(2.36531447826073,1.,-2.90994629141676));
#70433=CARTESIAN_POINT('Ctrl Pts',(2.36536211188453,1.,-2.90995756655606));
#70434=CARTESIAN_POINT('Ctrl Pts',(2.36553202948613,1.,-2.91005770527719));
#70435=CARTESIAN_POINT('Ctrl Pts',(2.36599991765749,1.,-2.91051690822156));
#70436=CARTESIAN_POINT('Ctrl Pts',(2.36707658451664,1.,-2.91181344022548));
#70437=CARTESIAN_POINT('Ctrl Pts',(2.36919161373173,1.,-2.9146124988314));
#70438=CARTESIAN_POINT('Ctrl Pts',(2.37229381109821,1.,-2.91891503791411));
#70439=CARTESIAN_POINT('Ctrl Pts',(2.3760651052403,1.,-2.92430340582608));
#70440=CARTESIAN_POINT('Ctrl Pts',(2.38028989582073,1.,-2.93049643640206));
#70441=CARTESIAN_POINT('Ctrl Pts',(2.38472771516311,1.,-2.93717903280391));
#70442=CARTESIAN_POINT('Ctrl Pts',(2.38914929090759,1.,-2.94404820669076));
#70443=CARTESIAN_POINT('Ctrl Pts',(2.39337207631667,1.,-2.95085857128439));
#70444=CARTESIAN_POINT('Ctrl Pts',(2.39730553974516,1.,-2.95748006482942));
#70445=CARTESIAN_POINT('Ctrl Pts',(2.4009556571164,1.,-2.96390432240312));
#70446=CARTESIAN_POINT('Ctrl Pts',(2.40438604734919,1.,-2.9701964131236));
#70447=CARTESIAN_POINT('Ctrl Pts',(2.40768975073713,1.,-2.97646002822422));
#70448=CARTESIAN_POINT('Ctrl Pts',(2.41095909342571,1.,-2.98280015815107));
#70449=CARTESIAN_POINT('Ctrl Pts',(2.41425064199586,1.,-2.98927983005796));
#70450=CARTESIAN_POINT('Ctrl Pts',(2.41757324500514,1.,-2.99590509293503));
#70451=CARTESIAN_POINT('Ctrl Pts',(2.42090763946779,1.,-3.00264868585996));
#70452=CARTESIAN_POINT('Ctrl Pts',(2.42421849439613,1.,-3.00946442616659));
#70453=CARTESIAN_POINT('Ctrl Pts',(2.42746856264168,1.,-3.01630420830504));
#70454=CARTESIAN_POINT('Ctrl Pts',(2.43063415586637,1.,-3.02313656036004));
#70455=CARTESIAN_POINT('Ctrl Pts',(2.43371241361488,1.,-3.02995534946978));
#70456=CARTESIAN_POINT('Ctrl Pts',(2.43671278042414,1.,-3.03676949672822));
#70457=CARTESIAN_POINT('Ctrl Pts',(2.43965194061857,1.,-3.04359685040555));
#70458=CARTESIAN_POINT('Ctrl Pts',(2.44254768923105,1.,-3.05045678021504));
#70459=CARTESIAN_POINT('Ctrl Pts',(2.44541251892556,1.,-3.05736242671506));
#70460=CARTESIAN_POINT('Ctrl Pts',(2.44824970516543,1.,-3.06431596421405));
#70461=CARTESIAN_POINT('Ctrl Pts',(2.45105688854422,1.,-3.07131290521297));
#70462=CARTESIAN_POINT('Ctrl Pts',(2.4538282678779,1.,-3.07834472886139));
#70463=CARTESIAN_POINT('Ctrl Pts',(2.45655725437039,1.,-3.08540206545315));
#70464=CARTESIAN_POINT('Ctrl Pts',(2.4592391256388,1.,-3.09247787931887));
#70465=CARTESIAN_POINT('Ctrl Pts',(2.46187308501884,1.,-3.09956993697052));
#70466=CARTESIAN_POINT('Ctrl Pts',(2.46446082979646,1.,-3.1066790790198));
#70467=CARTESIAN_POINT('Ctrl Pts',(2.46700558843506,1.,-3.11380805536122));
#70468=CARTESIAN_POINT('Ctrl Pts',(2.46951098947469,1.,-3.12096015766983));
#70469=CARTESIAN_POINT('Ctrl Pts',(2.47197997765871,1.,-3.12813790805952));
#70470=CARTESIAN_POINT('Ctrl Pts',(2.47441378371932,1.,-3.13534181229295));
#70471=CARTESIAN_POINT('Ctrl Pts',(2.47681245356109,1.,-3.1425709954655));
#70472=CARTESIAN_POINT('Ctrl Pts',(2.47917529057029,1.,-3.14982373241352));
#70473=CARTESIAN_POINT('Ctrl Pts',(2.48150133566571,1.,-3.15709802322739));
#70474=CARTESIAN_POINT('Ctrl Pts',(2.48378981792725,1.,-3.16439213290161));
#70475=CARTESIAN_POINT('Ctrl Pts',(2.48604065348587,1.,-3.17170518863313));
#70476=CARTESIAN_POINT('Ctrl Pts',(2.48825428288201,1.,-3.17903698136622));
#70477=CARTESIAN_POINT('Ctrl Pts',(2.49043146334059,1.,-3.18638771282266));
#70478=CARTESIAN_POINT('Ctrl Pts',(2.49257307239848,1.,-3.19375775555798));
#70479=CARTESIAN_POINT('Ctrl Pts',(2.49467992057755,1.,-3.20114742397588));
#70480=CARTESIAN_POINT('Ctrl Pts',(2.4967525264737,1.,-3.20855669849836));
#70481=CARTESIAN_POINT('Ctrl Pts',(2.4987911459939,1.,-3.21598526261286));
#70482=CARTESIAN_POINT('Ctrl Pts',(2.50079587201957,1.,-3.22343262620503));
#70483=CARTESIAN_POINT('Ctrl Pts',(2.50276671338111,1.,-3.23089822320646));
#70484=CARTESIAN_POINT('Ctrl Pts',(2.5047036758003,1.,-3.23838151080319));
#70485=CARTESIAN_POINT('Ctrl Pts',(2.506606859405,1.,-3.24588208983849));
#70486=CARTESIAN_POINT('Ctrl Pts',(2.50847647070723,1.,-3.25339971460982));
#70487=CARTESIAN_POINT('Ctrl Pts',(2.51031277813486,1.,-3.26093423001434));
#70488=CARTESIAN_POINT('Ctrl Pts',(2.51211608411423,1.,-3.26848552888116));
#70489=CARTESIAN_POINT('Ctrl Pts',(2.513886692704,1.,-3.27605350473142));
#70490=CARTESIAN_POINT('Ctrl Pts',(2.51562487464514,1.,-3.28363799702982));
#70491=CARTESIAN_POINT('Ctrl Pts',(2.51733085123797,1.,-3.2912387729927));
#70492=CARTESIAN_POINT('Ctrl Pts',(2.51900480701068,1.,-3.29885556388353));
#70493=CARTESIAN_POINT('Ctrl Pts',(2.52064689568511,1.,-3.30648808815443));
#70494=CARTESIAN_POINT('Ctrl Pts',(2.52225724871313,1.,-3.31413607874645));
#70495=CARTESIAN_POINT('Ctrl Pts',(2.5238359839626,1.,-3.32179931078699));
#70496=CARTESIAN_POINT('Ctrl Pts',(2.52538321164634,1.,-3.32947762187533));
#70497=CARTESIAN_POINT('Ctrl Pts',(2.52689902690158,1.,-3.33717089999103));
#70498=CARTESIAN_POINT('Ctrl Pts',(2.52808660915689,1.,-3.34333744115511));
#70499=CARTESIAN_POINT('Ctrl Pts',(2.52896321610703,1.,-3.34796903576663));
#70500=CARTESIAN_POINT('Ctrl Pts',(2.5295413654909,1.,-3.35105973714072));
#70501=CARTESIAN_POINT('Ctrl Pts',(2.52982887637028,1.,-3.35260583073571));
#70502=CARTESIAN_POINT('Origin',(2.52982887637028,0.,-3.35260583073571));
#70503=CARTESIAN_POINT('',(2.40675750623143,1.,-3.44202241512147));
#70504=CARTESIAN_POINT('Origin',(0.,0.,0.));
#70505=CARTESIAN_POINT('',(2.50410331873042,1.,-2.79140942341378));
#70506=CARTESIAN_POINT('Origin',(0.,1.,0.));
#70507=CARTESIAN_POINT('Ctrl Pts',(2.50410331873042,1.,-2.79140942341378));
#70508=CARTESIAN_POINT('Ctrl Pts',(2.50410331873042,0.666666666666667,-2.79140942341378));
#70509=CARTESIAN_POINT('Ctrl Pts',(2.50410331873042,0.333333333333333,-2.79140942341378));
#70510=CARTESIAN_POINT('Ctrl Pts',(2.50410331873042,-0.333333333333333,
-2.79140942341378));
#70511=CARTESIAN_POINT('Ctrl Pts',(2.50410331873042,-0.666666666666667,
-2.79140942341378));
#70512=CARTESIAN_POINT('Ctrl Pts',(2.50410331873042,-1.,-2.79140942341378));
#70513=CARTESIAN_POINT('Ctrl Pts',(2.91557726271063,-1.,-3.02314558451372));
#70514=CARTESIAN_POINT('Ctrl Pts',(2.91557726271063,1.,-3.02314558451372));
#70515=CARTESIAN_POINT('Ctrl Pts',(2.91409518070707,-1.,-3.02261975104912));
#70516=CARTESIAN_POINT('Ctrl Pts',(2.91409518070707,1.,-3.02261975104912));
#70517=CARTESIAN_POINT('Ctrl Pts',(2.91113297349052,-1.,-3.02156522743299));
#70518=CARTESIAN_POINT('Ctrl Pts',(2.91113297349052,1.,-3.02156522743299));
#70519=CARTESIAN_POINT('Ctrl Pts',(2.90669553303902,-1.,-3.01997487194926));
#70520=CARTESIAN_POINT('Ctrl Pts',(2.90669553303902,1.,-3.01997487194926));
#70521=CARTESIAN_POINT('Ctrl Pts',(2.90079069102661,-1.,-3.01783725123646));
#70522=CARTESIAN_POINT('Ctrl Pts',(2.90079069102661,1.,-3.01783725123646));
#70523=CARTESIAN_POINT('Ctrl Pts',(2.8934292556764,-1.,-3.01513660433291));
#70524=CARTESIAN_POINT('Ctrl Pts',(2.8934292556764,1.,-3.01513660433291));
#70525=CARTESIAN_POINT('Ctrl Pts',(2.88608751706796,-1.,-3.01240727309568));
#70526=CARTESIAN_POINT('Ctrl Pts',(2.88608751706796,1.,-3.01240727309568));
#70527=CARTESIAN_POINT('Ctrl Pts',(2.87876560072799,-1.,-3.0096491810855));
#70528=CARTESIAN_POINT('Ctrl Pts',(2.87876560072799,1.,-3.0096491810855));
#70529=CARTESIAN_POINT('Ctrl Pts',(2.87146368430104,-1.,-3.00686224485374));
#70530=CARTESIAN_POINT('Ctrl Pts',(2.87146368430104,1.,-3.00686224485374));
#70531=CARTESIAN_POINT('Ctrl Pts',(2.86418200833065,-1.,-3.00404638316245));
#70532=CARTESIAN_POINT('Ctrl Pts',(2.86418200833065,1.,-3.00404638316245));
#70533=CARTESIAN_POINT('Ctrl Pts',(2.85692085715129,-1.,-3.0012015079552));
#70534=CARTESIAN_POINT('Ctrl Pts',(2.85692085715129,1.,-3.0012015079552));
#70535=CARTESIAN_POINT('Ctrl Pts',(2.84968053289104,-1.,-2.99832751144566));
#70536=CARTESIAN_POINT('Ctrl Pts',(2.84968053289104,1.,-2.99832751144566));
#70537=CARTESIAN_POINT('Ctrl Pts',(2.84246132984334,-1.,-2.995424253416));
#70538=CARTESIAN_POINT('Ctrl Pts',(2.84246132984334,1.,-2.995424253416));
#70539=CARTESIAN_POINT('Ctrl Pts',(2.83526351254383,-1.,-2.99249155170479));
#70540=CARTESIAN_POINT('Ctrl Pts',(2.83526351254383,1.,-2.99249155170479));
#70541=CARTESIAN_POINT('Ctrl Pts',(2.82808728190402,-1.,-2.98952916401699));
#70542=CARTESIAN_POINT('Ctrl Pts',(2.82808728190402,1.,-2.98952916401699));
#70543=CARTESIAN_POINT('Ctrl Pts',(2.82093279065704,-1.,-2.98653680669434));
#70544=CARTESIAN_POINT('Ctrl Pts',(2.82093279065704,1.,-2.98653680669434));
#70545=CARTESIAN_POINT('Ctrl Pts',(2.81380019196454,-1.,-2.9835141977994));
#70546=CARTESIAN_POINT('Ctrl Pts',(2.81380019196454,1.,-2.9835141977994));
#70547=CARTESIAN_POINT('Ctrl Pts',(2.80668968101162,-1.,-2.98046109647299));
#70548=CARTESIAN_POINT('Ctrl Pts',(2.80668968101162,1.,-2.98046109647299));
#70549=CARTESIAN_POINT('Ctrl Pts',(2.79960153278186,-1.,-2.97737733718242));
#70550=CARTESIAN_POINT('Ctrl Pts',(2.79960153278186,1.,-2.97737733718242));
#70551=CARTESIAN_POINT('Ctrl Pts',(2.79253615718147,-1.,-2.97426288347475));
#70552=CARTESIAN_POINT('Ctrl Pts',(2.79253615718147,1.,-2.97426288347475));
#70553=CARTESIAN_POINT('Ctrl Pts',(2.78549409123657,-1.,-2.97111781461349));
#70554=CARTESIAN_POINT('Ctrl Pts',(2.78549409123657,1.,-2.97111781461349));
#70555=CARTESIAN_POINT('Ctrl Pts',(2.77847589542767,-1.,-2.9679422104295));
#70556=CARTESIAN_POINT('Ctrl Pts',(2.77847589542767,1.,-2.9679422104295));
#70557=CARTESIAN_POINT('Ctrl Pts',(2.77148206836464,-1.,-2.96473605585548));
#70558=CARTESIAN_POINT('Ctrl Pts',(2.77148206836464,1.,-2.96473605585548));
#70559=CARTESIAN_POINT('Ctrl Pts',(2.76451296269571,-1.,-2.96149914764832));
#70560=CARTESIAN_POINT('Ctrl Pts',(2.76451296269571,1.,-2.96149914764832));
#70561=CARTESIAN_POINT('Ctrl Pts',(2.75756867888393,-1.,-2.9582309766594));
#70562=CARTESIAN_POINT('Ctrl Pts',(2.75756867888393,1.,-2.9582309766594));
#70563=CARTESIAN_POINT('Ctrl Pts',(2.75064903318996,-1.,-2.95493069316211));
#70564=CARTESIAN_POINT('Ctrl Pts',(2.75064903318996,1.,-2.95493069316211));
#70565=CARTESIAN_POINT('Ctrl Pts',(2.7437537949221,-1.,-2.95159737214305));
#70566=CARTESIAN_POINT('Ctrl Pts',(2.7437537949221,1.,-2.95159737214305));
#70567=CARTESIAN_POINT('Ctrl Pts',(2.73688288329825,-1.,-2.94823023414381));
#70568=CARTESIAN_POINT('Ctrl Pts',(2.73688288329825,1.,-2.94823023414381));
#70569=CARTESIAN_POINT('Ctrl Pts',(2.73003657371613,-1.,-2.94482887675139));
#70570=CARTESIAN_POINT('Ctrl Pts',(2.73003657371613,1.,-2.94482887675139));
#70571=CARTESIAN_POINT('Ctrl Pts',(2.72321571511322,-1.,-2.94139351933882));
#70572=CARTESIAN_POINT('Ctrl Pts',(2.72321571511322,1.,-2.94139351933882));
#70573=CARTESIAN_POINT('Ctrl Pts',(2.71642190053575,-1.,-2.93792519474955));
#70574=CARTESIAN_POINT('Ctrl Pts',(2.71642190053575,1.,-2.93792519474955));
#70575=CARTESIAN_POINT('Ctrl Pts',(2.70965695523776,-1.,-2.93442516311168));
#70576=CARTESIAN_POINT('Ctrl Pts',(2.70965695523776,1.,-2.93442516311168));
#70577=CARTESIAN_POINT('Ctrl Pts',(2.70292247416881,-1.,-2.93089438233746));
#70578=CARTESIAN_POINT('Ctrl Pts',(2.70292247416881,1.,-2.93089438233746));
#70579=CARTESIAN_POINT('Ctrl Pts',(2.69621932864302,-1.,-2.92733294395268));
#70580=CARTESIAN_POINT('Ctrl Pts',(2.69621932864302,1.,-2.92733294395268));
#70581=CARTESIAN_POINT('Ctrl Pts',(2.68954721165342,-1.,-2.92373955325876));
#70582=CARTESIAN_POINT('Ctrl Pts',(2.68954721165342,1.,-2.92373955325876));
#70583=CARTESIAN_POINT('Ctrl Pts',(2.68290409279689,-1.,-2.92011090722152));
#70584=CARTESIAN_POINT('Ctrl Pts',(2.68290409279689,1.,-2.92011090722152));
#70585=CARTESIAN_POINT('Ctrl Pts',(2.67628728855309,-1.,-2.91644290704281));
#70586=CARTESIAN_POINT('Ctrl Pts',(2.67628728855309,1.,-2.91644290704281));
#70587=CARTESIAN_POINT('Ctrl Pts',(2.66969458792627,-1.,-2.91273193382876));
#70588=CARTESIAN_POINT('Ctrl Pts',(2.66969458792627,1.,-2.91273193382876));
#70589=CARTESIAN_POINT('Ctrl Pts',(2.66312542616808,-1.,-2.90897617968921));
#70590=CARTESIAN_POINT('Ctrl Pts',(2.66312542616808,1.,-2.90897617968921));
#70591=CARTESIAN_POINT('Ctrl Pts',(2.65658188464287,-1.,-2.90517678087467));
#70592=CARTESIAN_POINT('Ctrl Pts',(2.65658188464287,1.,-2.90517678087467));
#70593=CARTESIAN_POINT('Ctrl Pts',(2.65007017365576,-1.,-2.90133950224879));
#70594=CARTESIAN_POINT('Ctrl Pts',(2.65007017365576,1.,-2.90133950224879));
#70595=CARTESIAN_POINT('Ctrl Pts',(2.64359851684146,-1.,-2.89747231723361));
#70596=CARTESIAN_POINT('Ctrl Pts',(2.64359851684146,1.,-2.89747231723361));
#70597=CARTESIAN_POINT('Ctrl Pts',(2.63717442263944,-1.,-2.89358228854557));
#70598=CARTESIAN_POINT('Ctrl Pts',(2.63717442263944,1.,-2.89358228854557));
#70599=CARTESIAN_POINT('Ctrl Pts',(2.63080195420771,-1.,-2.88967244854243));
#70600=CARTESIAN_POINT('Ctrl Pts',(2.63080195420771,1.,-2.88967244854243));
#70601=CARTESIAN_POINT('Ctrl Pts',(2.62447947640253,-1.,-2.88573922195049));
#70602=CARTESIAN_POINT('Ctrl Pts',(2.62447947640253,1.,-2.88573922195049));
#70603=CARTESIAN_POINT('Ctrl Pts',(2.61819596473087,-1.,-2.88176821427502));
#70604=CARTESIAN_POINT('Ctrl Pts',(2.61819596473087,1.,-2.88176821427502));
#70605=CARTESIAN_POINT('Ctrl Pts',(2.61193507170928,-1.,-2.87773881947885));
#70606=CARTESIAN_POINT('Ctrl Pts',(2.61193507170928,1.,-2.87773881947885));
#70607=CARTESIAN_POINT('Ctrl Pts',(2.6056817788128,-1.,-2.87363176656475));
#70608=CARTESIAN_POINT('Ctrl Pts',(2.6056817788128,1.,-2.87363176656475));
#70609=CARTESIAN_POINT('Ctrl Pts',(2.59942875223202,-1.,-2.86943633170712));
#70610=CARTESIAN_POINT('Ctrl Pts',(2.59942875223202,1.,-2.86943633170712));
#70611=CARTESIAN_POINT('Ctrl Pts',(2.59318160184921,-1.,-2.86515629953528));
#70612=CARTESIAN_POINT('Ctrl Pts',(2.59318160184921,1.,-2.86515629953528));
#70613=CARTESIAN_POINT('Ctrl Pts',(2.5869677064356,-1.,-2.86081999003668));
#70614=CARTESIAN_POINT('Ctrl Pts',(2.5869677064356,1.,-2.86081999003668));
#70615=CARTESIAN_POINT('Ctrl Pts',(2.58082875254407,-1.,-2.85647171715147));
#70616=CARTESIAN_POINT('Ctrl Pts',(2.58082875254407,1.,-2.85647171715147));
#70617=CARTESIAN_POINT('Ctrl Pts',(2.57480482727128,-1.,-2.85215360144483));
#70618=CARTESIAN_POINT('Ctrl Pts',(2.57480482727128,1.,-2.85215360144483));
#70619=CARTESIAN_POINT('Ctrl Pts',(2.56891984251743,-1.,-2.84788893329091));
#70620=CARTESIAN_POINT('Ctrl Pts',(2.56891984251743,1.,-2.84788893329091));
#70621=CARTESIAN_POINT('Ctrl Pts',(2.56316920798489,-1.,-2.84366802680211));
#70622=CARTESIAN_POINT('Ctrl Pts',(2.56316920798489,1.,-2.84366802680211));
#70623=CARTESIAN_POINT('Ctrl Pts',(2.55749952145165,-1.,-2.83942515220699));
#70624=CARTESIAN_POINT('Ctrl Pts',(2.55749952145165,1.,-2.83942515220699));
#70625=CARTESIAN_POINT('Ctrl Pts',(2.55182152806964,-1.,-2.83505269592412));
#70626=CARTESIAN_POINT('Ctrl Pts',(2.55182152806964,1.,-2.83505269592412));
#70627=CARTESIAN_POINT('Ctrl Pts',(2.54604736792542,-1.,-2.83044254225794));
#70628=CARTESIAN_POINT('Ctrl Pts',(2.54604736792542,1.,-2.83044254225794));
#70629=CARTESIAN_POINT('Ctrl Pts',(2.54012272520141,-1.,-2.82552167649157));
#70630=CARTESIAN_POINT('Ctrl Pts',(2.54012272520141,1.,-2.82552167649157));
#70631=CARTESIAN_POINT('Ctrl Pts',(2.53405679667463,-1.,-2.82028550483744));
#70632=CARTESIAN_POINT('Ctrl Pts',(2.53405679667463,1.,-2.82028550483744));
#70633=CARTESIAN_POINT('Ctrl Pts',(2.52796388055457,-1.,-2.8148437904867));
#70634=CARTESIAN_POINT('Ctrl Pts',(2.52796388055457,1.,-2.8148437904867));
#70635=CARTESIAN_POINT('Ctrl Pts',(2.52205778589922,-1.,-2.80941521967234));
#70636=CARTESIAN_POINT('Ctrl Pts',(2.52205778589922,1.,-2.80941521967234));
#70637=CARTESIAN_POINT('Ctrl Pts',(2.51660190466067,-1.,-2.80427363984939));
#70638=CARTESIAN_POINT('Ctrl Pts',(2.51660190466067,1.,-2.80427363984939));
#70639=CARTESIAN_POINT('Ctrl Pts',(2.51186983687947,-1.,-2.79970585014308));
#70640=CARTESIAN_POINT('Ctrl Pts',(2.51186983687947,1.,-2.79970585014308));
#70641=CARTESIAN_POINT('Ctrl Pts',(2.50810555977564,-1.,-2.7959687805717));
#70642=CARTESIAN_POINT('Ctrl Pts',(2.50810555977564,1.,-2.7959687805717));
#70643=CARTESIAN_POINT('Ctrl Pts',(2.50547439929077,-1.,-2.79323694088143));
#70644=CARTESIAN_POINT('Ctrl Pts',(2.50547439929077,1.,-2.79323694088143));
#70645=CARTESIAN_POINT('Ctrl Pts',(2.50433799076945,-1.,-2.79192122906739));
#70646=CARTESIAN_POINT('Ctrl Pts',(2.50433799076945,1.,-2.79192122906739));
#70647=CARTESIAN_POINT('Ctrl Pts',(2.50404230339032,-1.,-2.79143626022225));
#70648=CARTESIAN_POINT('Ctrl Pts',(2.50404230339032,1.,-2.79143626022225));
#70649=CARTESIAN_POINT('Ctrl Pts',(2.50409239460011,-1.,-2.79133581100044));
#70650=CARTESIAN_POINT('Ctrl Pts',(2.50409239460011,1.,-2.79133581100044));
#70651=CARTESIAN_POINT('Ctrl Pts',(2.50417924854921,-1.,-2.79134130681569));
#70652=CARTESIAN_POINT('Ctrl Pts',(2.50417924854921,1.,-2.79134130681569));
#70653=CARTESIAN_POINT('',(2.91557726271063,1.,-3.02314558451372));
#70654=CARTESIAN_POINT('Ctrl Pts',(2.91557726271063,1.,-3.02314558451372));
#70655=CARTESIAN_POINT('Ctrl Pts',(2.91409518070707,1.,-3.02261975104912));
#70656=CARTESIAN_POINT('Ctrl Pts',(2.91113297349052,1.,-3.02156522743299));
#70657=CARTESIAN_POINT('Ctrl Pts',(2.90669553303902,1.,-3.01997487194926));
#70658=CARTESIAN_POINT('Ctrl Pts',(2.90079069102661,1.,-3.01783725123646));
#70659=CARTESIAN_POINT('Ctrl Pts',(2.8934292556764,1.,-3.01513660433291));
#70660=CARTESIAN_POINT('Ctrl Pts',(2.88608751706796,1.,-3.01240727309568));
#70661=CARTESIAN_POINT('Ctrl Pts',(2.87876560072799,1.,-3.0096491810855));
#70662=CARTESIAN_POINT('Ctrl Pts',(2.87146368430104,1.,-3.00686224485374));
#70663=CARTESIAN_POINT('Ctrl Pts',(2.86418200833065,1.,-3.00404638316245));
#70664=CARTESIAN_POINT('Ctrl Pts',(2.85692085715129,1.,-3.0012015079552));
#70665=CARTESIAN_POINT('Ctrl Pts',(2.84968053289104,1.,-2.99832751144566));
#70666=CARTESIAN_POINT('Ctrl Pts',(2.84246132984334,1.,-2.995424253416));
#70667=CARTESIAN_POINT('Ctrl Pts',(2.83526351254383,1.,-2.99249155170479));
#70668=CARTESIAN_POINT('Ctrl Pts',(2.82808728190402,1.,-2.98952916401699));
#70669=CARTESIAN_POINT('Ctrl Pts',(2.82093279065704,1.,-2.98653680669434));
#70670=CARTESIAN_POINT('Ctrl Pts',(2.81380019196454,1.,-2.9835141977994));
#70671=CARTESIAN_POINT('Ctrl Pts',(2.80668968101162,1.,-2.98046109647299));
#70672=CARTESIAN_POINT('Ctrl Pts',(2.79960153278186,1.,-2.97737733718242));
#70673=CARTESIAN_POINT('Ctrl Pts',(2.79253615718147,1.,-2.97426288347475));
#70674=CARTESIAN_POINT('Ctrl Pts',(2.78549409123657,1.,-2.97111781461349));
#70675=CARTESIAN_POINT('Ctrl Pts',(2.77847589542767,1.,-2.9679422104295));
#70676=CARTESIAN_POINT('Ctrl Pts',(2.77148206836464,1.,-2.96473605585548));
#70677=CARTESIAN_POINT('Ctrl Pts',(2.76451296269571,1.,-2.96149914764832));
#70678=CARTESIAN_POINT('Ctrl Pts',(2.75756867888393,1.,-2.9582309766594));
#70679=CARTESIAN_POINT('Ctrl Pts',(2.75064903318996,1.,-2.95493069316211));
#70680=CARTESIAN_POINT('Ctrl Pts',(2.7437537949221,1.,-2.95159737214305));
#70681=CARTESIAN_POINT('Ctrl Pts',(2.73688288329825,1.,-2.94823023414381));
#70682=CARTESIAN_POINT('Ctrl Pts',(2.73003657371613,1.,-2.94482887675139));
#70683=CARTESIAN_POINT('Ctrl Pts',(2.72321571511322,1.,-2.94139351933882));
#70684=CARTESIAN_POINT('Ctrl Pts',(2.71642190053575,1.,-2.93792519474955));
#70685=CARTESIAN_POINT('Ctrl Pts',(2.70965695523776,1.,-2.93442516311168));
#70686=CARTESIAN_POINT('Ctrl Pts',(2.70292247416881,1.,-2.93089438233746));
#70687=CARTESIAN_POINT('Ctrl Pts',(2.69621932864302,1.,-2.92733294395268));
#70688=CARTESIAN_POINT('Ctrl Pts',(2.68954721165342,1.,-2.92373955325876));
#70689=CARTESIAN_POINT('Ctrl Pts',(2.68290409279689,1.,-2.92011090722152));
#70690=CARTESIAN_POINT('Ctrl Pts',(2.67628728855309,1.,-2.91644290704281));
#70691=CARTESIAN_POINT('Ctrl Pts',(2.66969458792627,1.,-2.91273193382876));
#70692=CARTESIAN_POINT('Ctrl Pts',(2.66312542616808,1.,-2.90897617968921));
#70693=CARTESIAN_POINT('Ctrl Pts',(2.65658188464287,1.,-2.90517678087467));
#70694=CARTESIAN_POINT('Ctrl Pts',(2.65007017365576,1.,-2.90133950224879));
#70695=CARTESIAN_POINT('Ctrl Pts',(2.64359851684146,1.,-2.89747231723361));
#70696=CARTESIAN_POINT('Ctrl Pts',(2.63717442263944,1.,-2.89358228854557));
#70697=CARTESIAN_POINT('Ctrl Pts',(2.63080195420771,1.,-2.88967244854243));
#70698=CARTESIAN_POINT('Ctrl Pts',(2.62447947640253,1.,-2.88573922195049));
#70699=CARTESIAN_POINT('Ctrl Pts',(2.61819596473087,1.,-2.88176821427502));
#70700=CARTESIAN_POINT('Ctrl Pts',(2.61193507170928,1.,-2.87773881947885));
#70701=CARTESIAN_POINT('Ctrl Pts',(2.6056817788128,1.,-2.87363176656475));
#70702=CARTESIAN_POINT('Ctrl Pts',(2.59942875223202,1.,-2.86943633170712));
#70703=CARTESIAN_POINT('Ctrl Pts',(2.59318160184921,1.,-2.86515629953528));
#70704=CARTESIAN_POINT('Ctrl Pts',(2.5869677064356,1.,-2.86081999003668));
#70705=CARTESIAN_POINT('Ctrl Pts',(2.58082875254407,1.,-2.85647171715147));
#70706=CARTESIAN_POINT('Ctrl Pts',(2.57480482727128,1.,-2.85215360144483));
#70707=CARTESIAN_POINT('Ctrl Pts',(2.56891984251743,1.,-2.84788893329091));
#70708=CARTESIAN_POINT('Ctrl Pts',(2.56316920798489,1.,-2.84366802680211));
#70709=CARTESIAN_POINT('Ctrl Pts',(2.55749952145165,1.,-2.83942515220699));
#70710=CARTESIAN_POINT('Ctrl Pts',(2.55182152806964,1.,-2.83505269592412));
#70711=CARTESIAN_POINT('Ctrl Pts',(2.54604736792542,1.,-2.83044254225794));
#70712=CARTESIAN_POINT('Ctrl Pts',(2.54012272520141,1.,-2.82552167649157));
#70713=CARTESIAN_POINT('Ctrl Pts',(2.53405679667463,1.,-2.82028550483744));
#70714=CARTESIAN_POINT('Ctrl Pts',(2.52796388055457,1.,-2.8148437904867));
#70715=CARTESIAN_POINT('Ctrl Pts',(2.52205778589922,1.,-2.80941521967234));
#70716=CARTESIAN_POINT('Ctrl Pts',(2.51660190466067,1.,-2.80427363984939));
#70717=CARTESIAN_POINT('Ctrl Pts',(2.51186983687947,1.,-2.79970585014308));
#70718=CARTESIAN_POINT('Ctrl Pts',(2.50810555977564,1.,-2.7959687805717));
#70719=CARTESIAN_POINT('Ctrl Pts',(2.50567182569153,1.,-2.79344192164204));
#70720=CARTESIAN_POINT('Ctrl Pts',(2.50455968395235,1.,-2.79217568804874));
#70721=CARTESIAN_POINT('Ctrl Pts',(2.50417932839344,1.,-2.79164172519039));
#70722=CARTESIAN_POINT('Ctrl Pts',(2.50410700351427,1.,-2.79145823440899));
#70723=CARTESIAN_POINT('Ctrl Pts',(2.50410331873043,1.,-2.79140942341378));
#70724=CARTESIAN_POINT('',(2.91557726271063,0.,-3.02314558451372));
#70725=CARTESIAN_POINT('Ctrl Pts',(2.79134130681569,-1.,-2.50417924854921));
#70726=CARTESIAN_POINT('Ctrl Pts',(2.79134130681569,1.,-2.50417924854921));
#70727=CARTESIAN_POINT('Ctrl Pts',(2.7913358110015,-1.,-2.50409239460108));
#70728=CARTESIAN_POINT('Ctrl Pts',(2.7913358110015,1.,-2.50409239460108));
#70729=CARTESIAN_POINT('Ctrl Pts',(2.79143626022503,-1.,-2.50404230339286));
#70730=CARTESIAN_POINT('Ctrl Pts',(2.79143626022503,1.,-2.50404230339286));
#70731=CARTESIAN_POINT('Ctrl Pts',(2.79192122907148,-1.,-2.5043379907732));
#70732=CARTESIAN_POINT('Ctrl Pts',(2.79192122907148,1.,-2.5043379907732));
#70733=CARTESIAN_POINT('Ctrl Pts',(2.7932369408851,-1.,-2.50547439929414));
#70734=CARTESIAN_POINT('Ctrl Pts',(2.7932369408851,1.,-2.50547439929414));
#70735=CARTESIAN_POINT('Ctrl Pts',(2.79596878057287,-1.,-2.50810555977671));
#70736=CARTESIAN_POINT('Ctrl Pts',(2.79596878057287,1.,-2.50810555977671));
#70737=CARTESIAN_POINT('Ctrl Pts',(2.79970585014168,-1.,-2.51186983687818));
#70738=CARTESIAN_POINT('Ctrl Pts',(2.79970585014168,1.,-2.51186983687818));
#70739=CARTESIAN_POINT('Ctrl Pts',(2.80427363984653,-1.,-2.51660190465805));
#70740=CARTESIAN_POINT('Ctrl Pts',(2.80427363984653,1.,-2.51660190465805));
#70741=CARTESIAN_POINT('Ctrl Pts',(2.80941521966941,-1.,-2.52205778589653));
#70742=CARTESIAN_POINT('Ctrl Pts',(2.80941521966941,1.,-2.52205778589653));
#70743=CARTESIAN_POINT('Ctrl Pts',(2.81484379048475,-1.,-2.52796388055278));
#70744=CARTESIAN_POINT('Ctrl Pts',(2.81484379048475,1.,-2.52796388055278));
#70745=CARTESIAN_POINT('Ctrl Pts',(2.82028550483689,-1.,-2.53405679667412));
#70746=CARTESIAN_POINT('Ctrl Pts',(2.82028550483689,1.,-2.53405679667412));
#70747=CARTESIAN_POINT('Ctrl Pts',(2.8255216764922,-1.,-2.54012272520199));
#70748=CARTESIAN_POINT('Ctrl Pts',(2.8255216764922,1.,-2.54012272520199));
#70749=CARTESIAN_POINT('Ctrl Pts',(2.83044254225917,-1.,-2.54604736792655));
#70750=CARTESIAN_POINT('Ctrl Pts',(2.83044254225917,1.,-2.54604736792655));
#70751=CARTESIAN_POINT('Ctrl Pts',(2.83505269592536,-1.,-2.55182152807077));
#70752=CARTESIAN_POINT('Ctrl Pts',(2.83505269592536,1.,-2.55182152807077));
#70753=CARTESIAN_POINT('Ctrl Pts',(2.83942515220782,-1.,-2.55749952145241));
#70754=CARTESIAN_POINT('Ctrl Pts',(2.83942515220782,1.,-2.55749952145241));
#70755=CARTESIAN_POINT('Ctrl Pts',(2.84366802680237,-1.,-2.56316920798513));
#70756=CARTESIAN_POINT('Ctrl Pts',(2.84366802680237,1.,-2.56316920798513));
#70757=CARTESIAN_POINT('Ctrl Pts',(2.84788893329067,-1.,-2.56891984251721));
#70758=CARTESIAN_POINT('Ctrl Pts',(2.84788893329067,1.,-2.56891984251721));
#70759=CARTESIAN_POINT('Ctrl Pts',(2.85215360144431,-1.,-2.57480482727081));
#70760=CARTESIAN_POINT('Ctrl Pts',(2.85215360144431,1.,-2.57480482727081));
#70761=CARTESIAN_POINT('Ctrl Pts',(2.85647171715092,-1.,-2.58082875254357));
#70762=CARTESIAN_POINT('Ctrl Pts',(2.85647171715092,1.,-2.58082875254357));
#70763=CARTESIAN_POINT('Ctrl Pts',(2.86081999003629,-1.,-2.58696770643524));
#70764=CARTESIAN_POINT('Ctrl Pts',(2.86081999003629,1.,-2.58696770643524));
#70765=CARTESIAN_POINT('Ctrl Pts',(2.86515629953513,-1.,-2.59318160184908));
#70766=CARTESIAN_POINT('Ctrl Pts',(2.86515629953513,1.,-2.59318160184908));
#70767=CARTESIAN_POINT('Ctrl Pts',(2.86943633170722,-1.,-2.5994287522321));
#70768=CARTESIAN_POINT('Ctrl Pts',(2.86943633170722,1.,-2.5994287522321));
#70769=CARTESIAN_POINT('Ctrl Pts',(2.87363176656501,-1.,-2.60568177881303));
#70770=CARTESIAN_POINT('Ctrl Pts',(2.87363176656501,1.,-2.60568177881303));
#70771=CARTESIAN_POINT('Ctrl Pts',(2.87773881947915,-1.,-2.61193507170955));
#70772=CARTESIAN_POINT('Ctrl Pts',(2.87773881947915,1.,-2.61193507170955));
#70773=CARTESIAN_POINT('Ctrl Pts',(2.88176821427525,-1.,-2.61819596473108));
#70774=CARTESIAN_POINT('Ctrl Pts',(2.88176821427525,1.,-2.61819596473108));
#70775=CARTESIAN_POINT('Ctrl Pts',(2.88573922195059,-1.,-2.62447947640262));
#70776=CARTESIAN_POINT('Ctrl Pts',(2.88573922195059,1.,-2.62447947640262));
#70777=CARTESIAN_POINT('Ctrl Pts',(2.88967244854239,-1.,-2.63080195420767));
#70778=CARTESIAN_POINT('Ctrl Pts',(2.88967244854239,1.,-2.63080195420767));
#70779=CARTESIAN_POINT('Ctrl Pts',(2.89358228854544,-1.,-2.63717442263932));
#70780=CARTESIAN_POINT('Ctrl Pts',(2.89358228854544,1.,-2.63717442263932));
#70781=CARTESIAN_POINT('Ctrl Pts',(2.89747231723345,-1.,-2.64359851684131));
#70782=CARTESIAN_POINT('Ctrl Pts',(2.89747231723345,1.,-2.64359851684131));
#70783=CARTESIAN_POINT('Ctrl Pts',(2.90133950224867,-1.,-2.65007017365564));
#70784=CARTESIAN_POINT('Ctrl Pts',(2.90133950224867,1.,-2.65007017365564));
#70785=CARTESIAN_POINT('Ctrl Pts',(2.90517678087461,-1.,-2.65658188464282));
#70786=CARTESIAN_POINT('Ctrl Pts',(2.90517678087461,1.,-2.65658188464282));
#70787=CARTESIAN_POINT('Ctrl Pts',(2.90897617968923,-1.,-2.6631254261681));
#70788=CARTESIAN_POINT('Ctrl Pts',(2.90897617968923,1.,-2.6631254261681));
#70789=CARTESIAN_POINT('Ctrl Pts',(2.91273193382882,-1.,-2.66969458792631));
#70790=CARTESIAN_POINT('Ctrl Pts',(2.91273193382882,1.,-2.66969458792631));
#70791=CARTESIAN_POINT('Ctrl Pts',(2.91644290704285,-1.,-2.67628728855312));
#70792=CARTESIAN_POINT('Ctrl Pts',(2.91644290704285,1.,-2.67628728855312));
#70793=CARTESIAN_POINT('Ctrl Pts',(2.92011090722152,-1.,-2.68290409279688));
#70794=CARTESIAN_POINT('Ctrl Pts',(2.92011090722152,1.,-2.68290409279688));
#70795=CARTESIAN_POINT('Ctrl Pts',(2.92373955325875,-1.,-2.68954721165339));
#70796=CARTESIAN_POINT('Ctrl Pts',(2.92373955325875,1.,-2.68954721165339));
#70797=CARTESIAN_POINT('Ctrl Pts',(2.92733294395267,-1.,-2.69621932864301));
#70798=CARTESIAN_POINT('Ctrl Pts',(2.92733294395267,1.,-2.69621932864301));
#70799=CARTESIAN_POINT('Ctrl Pts',(2.93089438233749,-1.,-2.70292247416885));
#70800=CARTESIAN_POINT('Ctrl Pts',(2.93089438233749,1.,-2.70292247416885));
#70801=CARTESIAN_POINT('Ctrl Pts',(2.93442516311179,-1.,-2.70965695523787));
#70802=CARTESIAN_POINT('Ctrl Pts',(2.93442516311179,1.,-2.70965695523787));
#70803=CARTESIAN_POINT('Ctrl Pts',(2.93792519474972,-1.,-2.71642190053592));
#70804=CARTESIAN_POINT('Ctrl Pts',(2.93792519474972,1.,-2.71642190053592));
#70805=CARTESIAN_POINT('Ctrl Pts',(2.94139351933897,-1.,-2.72321571511337));
#70806=CARTESIAN_POINT('Ctrl Pts',(2.94139351933897,1.,-2.72321571511337));
#70807=CARTESIAN_POINT('Ctrl Pts',(2.94482887675143,-1.,-2.73003657371617));
#70808=CARTESIAN_POINT('Ctrl Pts',(2.94482887675143,1.,-2.73003657371617));
#70809=CARTESIAN_POINT('Ctrl Pts',(2.94823023414364,-1.,-2.73688288329808));
#70810=CARTESIAN_POINT('Ctrl Pts',(2.94823023414364,1.,-2.73688288329808));
#70811=CARTESIAN_POINT('Ctrl Pts',(2.95159737214266,-1.,-2.74375379492172));
#70812=CARTESIAN_POINT('Ctrl Pts',(2.95159737214266,1.,-2.74375379492172));
#70813=CARTESIAN_POINT('Ctrl Pts',(2.95493069316161,-1.,-2.75064903318947));
#70814=CARTESIAN_POINT('Ctrl Pts',(2.95493069316161,1.,-2.75064903318947));
#70815=CARTESIAN_POINT('Ctrl Pts',(2.95823097665896,-1.,-2.7575686788835));
#70816=CARTESIAN_POINT('Ctrl Pts',(2.95823097665896,1.,-2.7575686788835));
#70817=CARTESIAN_POINT('Ctrl Pts',(2.96149914764818,-1.,-2.76451296269557));
#70818=CARTESIAN_POINT('Ctrl Pts',(2.96149914764818,1.,-2.76451296269557));
#70819=CARTESIAN_POINT('Ctrl Pts',(2.96473605585583,-1.,-2.77148206836498));
#70820=CARTESIAN_POINT('Ctrl Pts',(2.96473605585583,1.,-2.77148206836498));
#70821=CARTESIAN_POINT('Ctrl Pts',(2.96794221043036,-1.,-2.7784758954285));
#70822=CARTESIAN_POINT('Ctrl Pts',(2.96794221043036,1.,-2.7784758954285));
#70823=CARTESIAN_POINT('Ctrl Pts',(2.97111781461465,-1.,-2.78549409123769));
#70824=CARTESIAN_POINT('Ctrl Pts',(2.97111781461465,1.,-2.78549409123769));
#70825=CARTESIAN_POINT('Ctrl Pts',(2.9742628834758,-1.,-2.79253615718248));
#70826=CARTESIAN_POINT('Ctrl Pts',(2.9742628834758,1.,-2.79253615718248));
#70827=CARTESIAN_POINT('Ctrl Pts',(2.97737733718287,-1.,-2.7996015327823));
#70828=CARTESIAN_POINT('Ctrl Pts',(2.97737733718287,1.,-2.7996015327823));
#70829=CARTESIAN_POINT('Ctrl Pts',(2.98046109647241,-1.,-2.80668968101106));
#70830=CARTESIAN_POINT('Ctrl Pts',(2.98046109647241,1.,-2.80668968101106));
#70831=CARTESIAN_POINT('Ctrl Pts',(2.98351419779767,-1.,-2.81380019196286));
#70832=CARTESIAN_POINT('Ctrl Pts',(2.98351419779767,1.,-2.81380019196286));
#70833=CARTESIAN_POINT('Ctrl Pts',(2.9865368066918,-1.,-2.82093279065457));
#70834=CARTESIAN_POINT('Ctrl Pts',(2.9865368066918,1.,-2.82093279065457));
#70835=CARTESIAN_POINT('Ctrl Pts',(2.98952916401446,-1.,-2.82808728190157));
#70836=CARTESIAN_POINT('Ctrl Pts',(2.98952916401446,1.,-2.82808728190157));
#70837=CARTESIAN_POINT('Ctrl Pts',(2.99249155170339,-1.,-2.83526351254248));
#70838=CARTESIAN_POINT('Ctrl Pts',(2.99249155170339,1.,-2.83526351254248));
#70839=CARTESIAN_POINT('Ctrl Pts',(2.99542425341685,-1.,-2.84246132984415));
#70840=CARTESIAN_POINT('Ctrl Pts',(2.99542425341685,1.,-2.84246132984415));
#70841=CARTESIAN_POINT('Ctrl Pts',(2.99832751144925,-1.,-2.84968053289451));
#70842=CARTESIAN_POINT('Ctrl Pts',(2.99832751144925,1.,-2.84968053289451));
#70843=CARTESIAN_POINT('Ctrl Pts',(3.00120150796095,-1.,-2.85692085715686));
#70844=CARTESIAN_POINT('Ctrl Pts',(3.00120150796095,1.,-2.85692085715686));
#70845=CARTESIAN_POINT('Ctrl Pts',(3.00404638316867,-1.,-2.86418200833667));
#70846=CARTESIAN_POINT('Ctrl Pts',(3.00404638316867,1.,-2.86418200833667));
#70847=CARTESIAN_POINT('Ctrl Pts',(3.00686224485784,-1.,-2.87146368430502));
#70848=CARTESIAN_POINT('Ctrl Pts',(3.00686224485784,1.,-2.87146368430502));
#70849=CARTESIAN_POINT('Ctrl Pts',(3.00964918108476,-1.,-2.87876560072727));
#70850=CARTESIAN_POINT('Ctrl Pts',(3.00964918108476,1.,-2.87876560072727));
#70851=CARTESIAN_POINT('Ctrl Pts',(3.01240727308829,-1.,-2.8860875170608));
#70852=CARTESIAN_POINT('Ctrl Pts',(3.01240727308829,1.,-2.8860875170608));
#70853=CARTESIAN_POINT('Ctrl Pts',(3.01513660431928,-1.,-2.89342925566321));
#70854=CARTESIAN_POINT('Ctrl Pts',(3.01513660431928,1.,-2.89342925566321));
#70855=CARTESIAN_POINT('Ctrl Pts',(3.01783725121981,-1.,-2.9007906910105));
#70856=CARTESIAN_POINT('Ctrl Pts',(3.01783725121981,1.,-2.9007906910105));
#70857=CARTESIAN_POINT('Ctrl Pts',(3.01997487193503,-1.,-2.90669553302526));
#70858=CARTESIAN_POINT('Ctrl Pts',(3.01997487193503,1.,-2.90669553302526));
#70859=CARTESIAN_POINT('Ctrl Pts',(3.02156522742431,-1.,-2.91113297348212));
#70860=CARTESIAN_POINT('Ctrl Pts',(3.02156522742431,1.,-2.91113297348212));
#70861=CARTESIAN_POINT('Ctrl Pts',(3.02261975104593,-1.,-2.91409518070399));
#70862=CARTESIAN_POINT('Ctrl Pts',(3.02261975104593,1.,-2.91409518070399));
#70863=CARTESIAN_POINT('Ctrl Pts',(3.02314558451372,-1.,-2.91557726271063));
#70864=CARTESIAN_POINT('Ctrl Pts',(3.02314558451372,1.,-2.91557726271063));
#70865=CARTESIAN_POINT('',(2.79140942341258,1.,-2.50410331873176));
#70866=CARTESIAN_POINT('Ctrl Pts',(2.79140942341258,-1.,-2.50410331873176));
#70867=CARTESIAN_POINT('Ctrl Pts',(2.79140942341258,-0.666666666666667,
-2.50410331873176));
#70868=CARTESIAN_POINT('Ctrl Pts',(2.79140942341258,-0.333333333333333,
-2.50410331873176));
#70869=CARTESIAN_POINT('Ctrl Pts',(2.79140942341258,0.333333333333333,-2.50410331873176));
#70870=CARTESIAN_POINT('Ctrl Pts',(2.79140942341258,0.666666666666667,-2.50410331873176));
#70871=CARTESIAN_POINT('Ctrl Pts',(2.79140942341258,1.,-2.50410331873176));
#70872=CARTESIAN_POINT('',(3.02314558451372,1.,-2.91557726271063));
#70873=CARTESIAN_POINT('',(3.02314558451372,0.,-2.91557726271063));
#70874=CARTESIAN_POINT('Ctrl Pts',(2.79140942341258,1.,-2.50410331873176));
#70875=CARTESIAN_POINT('Ctrl Pts',(2.79145823440781,1.,-2.50410700351493));
#70876=CARTESIAN_POINT('Ctrl Pts',(2.79164172518905,1.,-2.50417932839313));
#70877=CARTESIAN_POINT('Ctrl Pts',(2.79217568804755,1.,-2.50455968395146));
#70878=CARTESIAN_POINT('Ctrl Pts',(2.79344192164147,1.,-2.50567182569081));
#70879=CARTESIAN_POINT('Ctrl Pts',(2.79596878057287,1.,-2.50810555977671));
#70880=CARTESIAN_POINT('Ctrl Pts',(2.79970585014168,1.,-2.51186983687818));
#70881=CARTESIAN_POINT('Ctrl Pts',(2.80427363984653,1.,-2.51660190465805));
#70882=CARTESIAN_POINT('Ctrl Pts',(2.80941521966941,1.,-2.52205778589653));
#70883=CARTESIAN_POINT('Ctrl Pts',(2.81484379048475,1.,-2.52796388055278));
#70884=CARTESIAN_POINT('Ctrl Pts',(2.82028550483689,1.,-2.53405679667412));
#70885=CARTESIAN_POINT('Ctrl Pts',(2.8255216764922,1.,-2.54012272520199));
#70886=CARTESIAN_POINT('Ctrl Pts',(2.83044254225917,1.,-2.54604736792655));
#70887=CARTESIAN_POINT('Ctrl Pts',(2.83505269592536,1.,-2.55182152807077));
#70888=CARTESIAN_POINT('Ctrl Pts',(2.83942515220782,1.,-2.55749952145241));
#70889=CARTESIAN_POINT('Ctrl Pts',(2.84366802680237,1.,-2.56316920798513));
#70890=CARTESIAN_POINT('Ctrl Pts',(2.84788893329067,1.,-2.56891984251721));
#70891=CARTESIAN_POINT('Ctrl Pts',(2.85215360144431,1.,-2.57480482727081));
#70892=CARTESIAN_POINT('Ctrl Pts',(2.85647171715092,1.,-2.58082875254357));
#70893=CARTESIAN_POINT('Ctrl Pts',(2.86081999003629,1.,-2.58696770643524));
#70894=CARTESIAN_POINT('Ctrl Pts',(2.86515629953513,1.,-2.59318160184908));
#70895=CARTESIAN_POINT('Ctrl Pts',(2.86943633170722,1.,-2.5994287522321));
#70896=CARTESIAN_POINT('Ctrl Pts',(2.87363176656501,1.,-2.60568177881303));
#70897=CARTESIAN_POINT('Ctrl Pts',(2.87773881947915,1.,-2.61193507170955));
#70898=CARTESIAN_POINT('Ctrl Pts',(2.88176821427525,1.,-2.61819596473108));
#70899=CARTESIAN_POINT('Ctrl Pts',(2.88573922195059,1.,-2.62447947640262));
#70900=CARTESIAN_POINT('Ctrl Pts',(2.88967244854239,1.,-2.63080195420767));
#70901=CARTESIAN_POINT('Ctrl Pts',(2.89358228854544,1.,-2.63717442263932));
#70902=CARTESIAN_POINT('Ctrl Pts',(2.89747231723345,1.,-2.64359851684131));
#70903=CARTESIAN_POINT('Ctrl Pts',(2.90133950224867,1.,-2.65007017365564));
#70904=CARTESIAN_POINT('Ctrl Pts',(2.90517678087461,1.,-2.65658188464282));
#70905=CARTESIAN_POINT('Ctrl Pts',(2.90897617968923,1.,-2.6631254261681));
#70906=CARTESIAN_POINT('Ctrl Pts',(2.91273193382882,1.,-2.66969458792631));
#70907=CARTESIAN_POINT('Ctrl Pts',(2.91644290704285,1.,-2.67628728855312));
#70908=CARTESIAN_POINT('Ctrl Pts',(2.92011090722152,1.,-2.68290409279688));
#70909=CARTESIAN_POINT('Ctrl Pts',(2.92373955325875,1.,-2.68954721165339));
#70910=CARTESIAN_POINT('Ctrl Pts',(2.92733294395267,1.,-2.69621932864301));
#70911=CARTESIAN_POINT('Ctrl Pts',(2.93089438233749,1.,-2.70292247416885));
#70912=CARTESIAN_POINT('Ctrl Pts',(2.93442516311179,1.,-2.70965695523787));
#70913=CARTESIAN_POINT('Ctrl Pts',(2.93792519474972,1.,-2.71642190053592));
#70914=CARTESIAN_POINT('Ctrl Pts',(2.94139351933897,1.,-2.72321571511337));
#70915=CARTESIAN_POINT('Ctrl Pts',(2.94482887675143,1.,-2.73003657371617));
#70916=CARTESIAN_POINT('Ctrl Pts',(2.94823023414364,1.,-2.73688288329808));
#70917=CARTESIAN_POINT('Ctrl Pts',(2.95159737214266,1.,-2.74375379492172));
#70918=CARTESIAN_POINT('Ctrl Pts',(2.95493069316161,1.,-2.75064903318947));
#70919=CARTESIAN_POINT('Ctrl Pts',(2.95823097665896,1.,-2.7575686788835));
#70920=CARTESIAN_POINT('Ctrl Pts',(2.96149914764818,1.,-2.76451296269557));
#70921=CARTESIAN_POINT('Ctrl Pts',(2.96473605585583,1.,-2.77148206836498));
#70922=CARTESIAN_POINT('Ctrl Pts',(2.96794221043036,1.,-2.7784758954285));
#70923=CARTESIAN_POINT('Ctrl Pts',(2.97111781461465,1.,-2.78549409123769));
#70924=CARTESIAN_POINT('Ctrl Pts',(2.9742628834758,1.,-2.79253615718248));
#70925=CARTESIAN_POINT('Ctrl Pts',(2.97737733718287,1.,-2.7996015327823));
#70926=CARTESIAN_POINT('Ctrl Pts',(2.98046109647241,1.,-2.80668968101106));
#70927=CARTESIAN_POINT('Ctrl Pts',(2.98351419779767,1.,-2.81380019196286));
#70928=CARTESIAN_POINT('Ctrl Pts',(2.9865368066918,1.,-2.82093279065457));
#70929=CARTESIAN_POINT('Ctrl Pts',(2.98952916401446,1.,-2.82808728190157));
#70930=CARTESIAN_POINT('Ctrl Pts',(2.99249155170339,1.,-2.83526351254248));
#70931=CARTESIAN_POINT('Ctrl Pts',(2.99542425341685,1.,-2.84246132984415));
#70932=CARTESIAN_POINT('Ctrl Pts',(2.99832751144925,1.,-2.84968053289451));
#70933=CARTESIAN_POINT('Ctrl Pts',(3.00120150796095,1.,-2.85692085715686));
#70934=CARTESIAN_POINT('Ctrl Pts',(3.00404638316867,1.,-2.86418200833667));
#70935=CARTESIAN_POINT('Ctrl Pts',(3.00686224485784,1.,-2.87146368430502));
#70936=CARTESIAN_POINT('Ctrl Pts',(3.00964918108476,1.,-2.87876560072727));
#70937=CARTESIAN_POINT('Ctrl Pts',(3.01240727308829,1.,-2.8860875170608));
#70938=CARTESIAN_POINT('Ctrl Pts',(3.01513660431928,1.,-2.89342925566321));
#70939=CARTESIAN_POINT('Ctrl Pts',(3.01783725121981,1.,-2.9007906910105));
#70940=CARTESIAN_POINT('Ctrl Pts',(3.01997487193503,1.,-2.90669553302526));
#70941=CARTESIAN_POINT('Ctrl Pts',(3.02156522742431,1.,-2.91113297348212));
#70942=CARTESIAN_POINT('Ctrl Pts',(3.02261975104593,1.,-2.91409518070399));
#70943=CARTESIAN_POINT('Ctrl Pts',(3.02314558451372,1.,-2.91557726271063));
#70944=CARTESIAN_POINT('Origin',(3.02314558451372,0.,-2.91557726271063));
#70945=CARTESIAN_POINT('',(2.91557726271063,1.,-3.02314558451372));
#70946=CARTESIAN_POINT('Origin',(0.,0.,0.));
#70947=CARTESIAN_POINT('',(2.90994629141562,1.,-2.36531447826213));
#70948=CARTESIAN_POINT('Origin',(0.,1.,0.));
#70949=CARTESIAN_POINT('Ctrl Pts',(2.90994629141562,1.,-2.36531447826213));
#70950=CARTESIAN_POINT('Ctrl Pts',(2.90994629141562,0.666666666666667,-2.36531447826213));
#70951=CARTESIAN_POINT('Ctrl Pts',(2.90994629141562,0.333333333333333,-2.36531447826213));
#70952=CARTESIAN_POINT('Ctrl Pts',(2.90994629141562,-0.333333333333333,
-2.36531447826213));
#70953=CARTESIAN_POINT('Ctrl Pts',(2.90994629141562,-0.666666666666667,
-2.36531447826213));
#70954=CARTESIAN_POINT('Ctrl Pts',(2.90994629141562,-1.,-2.36531447826213));
#70955=CARTESIAN_POINT('Ctrl Pts',(3.35260583073571,-1.,-2.52982887637028));
#70956=CARTESIAN_POINT('Ctrl Pts',(3.35260583073571,1.,-2.52982887637028));
#70957=CARTESIAN_POINT('Ctrl Pts',(3.35105973714426,-1.,-2.52954136549357));
#70958=CARTESIAN_POINT('Ctrl Pts',(3.35105973714426,1.,-2.52954136549357));
#70959=CARTESIAN_POINT('Ctrl Pts',(3.34796903577628,-1.,-2.5289632161143));
#70960=CARTESIAN_POINT('Ctrl Pts',(3.34796903577628,1.,-2.5289632161143));
#70961=CARTESIAN_POINT('Ctrl Pts',(3.34333744117093,-1.,-2.52808660916879));
#70962=CARTESIAN_POINT('Ctrl Pts',(3.34333744117093,1.,-2.52808660916879));
#70963=CARTESIAN_POINT('Ctrl Pts',(3.33717090000955,-1.,-2.52689902691551));
#70964=CARTESIAN_POINT('Ctrl Pts',(3.33717090000955,1.,-2.52689902691551));
#70965=CARTESIAN_POINT('Ctrl Pts',(3.32947762189049,-1.,-2.52538321165774));
#70966=CARTESIAN_POINT('Ctrl Pts',(3.32947762189049,1.,-2.52538321165774));
#70967=CARTESIAN_POINT('Ctrl Pts',(3.32179931079521,-1.,-2.52383598396878));
#70968=CARTESIAN_POINT('Ctrl Pts',(3.32179931079521,1.,-2.52383598396878));
#70969=CARTESIAN_POINT('Ctrl Pts',(3.31413607874727,-1.,-2.52225724871375));
#70970=CARTESIAN_POINT('Ctrl Pts',(3.31413607874727,1.,-2.52225724871375));
#70971=CARTESIAN_POINT('Ctrl Pts',(3.30648808814986,-1.,-2.52064689568167));
#70972=CARTESIAN_POINT('Ctrl Pts',(3.30648808814986,1.,-2.52064689568167));
#70973=CARTESIAN_POINT('Ctrl Pts',(3.29885556387661,-1.,-2.51900480700548));
#70974=CARTESIAN_POINT('Ctrl Pts',(3.29885556387661,1.,-2.51900480700548));
#70975=CARTESIAN_POINT('Ctrl Pts',(3.2912387729863,-1.,-2.51733085123316));
#70976=CARTESIAN_POINT('Ctrl Pts',(3.2912387729863,1.,-2.51733085123316));
#70977=CARTESIAN_POINT('Ctrl Pts',(3.28363799702583,-1.,-2.51562487464215));
#70978=CARTESIAN_POINT('Ctrl Pts',(3.28363799702583,1.,-2.51562487464215));
#70979=CARTESIAN_POINT('Ctrl Pts',(3.27605350473048,-1.,-2.51388669270329));
#70980=CARTESIAN_POINT('Ctrl Pts',(3.27605350473048,1.,-2.51388669270329));
#70981=CARTESIAN_POINT('Ctrl Pts',(3.26848552888271,-1.,-2.51211608411539));
#70982=CARTESIAN_POINT('Ctrl Pts',(3.26848552888271,1.,-2.51211608411539));
#70983=CARTESIAN_POINT('Ctrl Pts',(3.26093423001716,-1.,-2.51031277813697));
#70984=CARTESIAN_POINT('Ctrl Pts',(3.26093423001716,1.,-2.51031277813697));
#70985=CARTESIAN_POINT('Ctrl Pts',(3.25339971461265,-1.,-2.50847647070936));
#70986=CARTESIAN_POINT('Ctrl Pts',(3.25339971461265,1.,-2.50847647070936));
#70987=CARTESIAN_POINT('Ctrl Pts',(3.24588208984042,-1.,-2.50660685940645));
#70988=CARTESIAN_POINT('Ctrl Pts',(3.24588208984042,1.,-2.50660685940645));
#70989=CARTESIAN_POINT('Ctrl Pts',(3.23838151080383,-1.,-2.50470367580078));
#70990=CARTESIAN_POINT('Ctrl Pts',(3.23838151080383,1.,-2.50470367580078));
#70991=CARTESIAN_POINT('Ctrl Pts',(3.23089822320596,-1.,-2.50276671338074));
#70992=CARTESIAN_POINT('Ctrl Pts',(3.23089822320596,1.,-2.50276671338074));
#70993=CARTESIAN_POINT('Ctrl Pts',(3.22343262620387,-1.,-2.5007958720187));
#70994=CARTESIAN_POINT('Ctrl Pts',(3.22343262620387,1.,-2.5007958720187));
#70995=CARTESIAN_POINT('Ctrl Pts',(3.21598526261157,-1.,-2.49879114599293));
#70996=CARTESIAN_POINT('Ctrl Pts',(3.21598526261157,1.,-2.49879114599293));
#70997=CARTESIAN_POINT('Ctrl Pts',(3.2085566984974,-1.,-2.49675252647298));
#70998=CARTESIAN_POINT('Ctrl Pts',(3.2085566984974,1.,-2.49675252647298));
#70999=CARTESIAN_POINT('Ctrl Pts',(3.20114742397549,-1.,-2.49467992057726));
#71000=CARTESIAN_POINT('Ctrl Pts',(3.20114742397549,1.,-2.49467992057726));
#71001=CARTESIAN_POINT('Ctrl Pts',(3.19375775555814,-1.,-2.4925730723986));
#71002=CARTESIAN_POINT('Ctrl Pts',(3.19375775555814,1.,-2.4925730723986));
#71003=CARTESIAN_POINT('Ctrl Pts',(3.18638771282315,-1.,-2.49043146334095));
#71004=CARTESIAN_POINT('Ctrl Pts',(3.18638771282315,1.,-2.49043146334095));
#71005=CARTESIAN_POINT('Ctrl Pts',(3.17903698136678,-1.,-2.48825428288243));
#71006=CARTESIAN_POINT('Ctrl Pts',(3.17903698136678,1.,-2.48825428288243));
#71007=CARTESIAN_POINT('Ctrl Pts',(3.17170518863357,-1.,-2.48604065348619));
#71008=CARTESIAN_POINT('Ctrl Pts',(3.17170518863357,1.,-2.48604065348619));
#71009=CARTESIAN_POINT('Ctrl Pts',(3.16439213290181,-1.,-2.48378981792739));
#71010=CARTESIAN_POINT('Ctrl Pts',(3.16439213290181,1.,-2.48378981792739));
#71011=CARTESIAN_POINT('Ctrl Pts',(3.15709802322735,-1.,-2.48150133566568));
#71012=CARTESIAN_POINT('Ctrl Pts',(3.15709802322735,1.,-2.48150133566568));
#71013=CARTESIAN_POINT('Ctrl Pts',(3.14982373241335,-1.,-2.47917529057016));
#71014=CARTESIAN_POINT('Ctrl Pts',(3.14982373241335,1.,-2.47917529057016));
#71015=CARTESIAN_POINT('Ctrl Pts',(3.14257099546531,-1.,-2.47681245356095));
#71016=CARTESIAN_POINT('Ctrl Pts',(3.14257099546531,1.,-2.47681245356095));
#71017=CARTESIAN_POINT('Ctrl Pts',(3.13534181229282,-1.,-2.47441378371923));
#71018=CARTESIAN_POINT('Ctrl Pts',(3.13534181229282,1.,-2.47441378371923));
#71019=CARTESIAN_POINT('Ctrl Pts',(3.12813790805948,-1.,-2.47197997765868));
#71020=CARTESIAN_POINT('Ctrl Pts',(3.12813790805948,1.,-2.47197997765868));
#71021=CARTESIAN_POINT('Ctrl Pts',(3.12096015766984,-1.,-2.4695109894747));
#71022=CARTESIAN_POINT('Ctrl Pts',(3.12096015766984,1.,-2.4695109894747));
#71023=CARTESIAN_POINT('Ctrl Pts',(3.11380805536124,-1.,-2.46700558843507));
#71024=CARTESIAN_POINT('Ctrl Pts',(3.11380805536124,1.,-2.46700558843507));
#71025=CARTESIAN_POINT('Ctrl Pts',(3.10667907901981,-1.,-2.46446082979645));
#71026=CARTESIAN_POINT('Ctrl Pts',(3.10667907901981,1.,-2.46446082979645));
#71027=CARTESIAN_POINT('Ctrl Pts',(3.09956993697048,-1.,-2.4618730850188));
#71028=CARTESIAN_POINT('Ctrl Pts',(3.09956993697048,1.,-2.4618730850188));
#71029=CARTESIAN_POINT('Ctrl Pts',(3.09247787931881,-1.,-2.45923912563875));
#71030=CARTESIAN_POINT('Ctrl Pts',(3.09247787931881,1.,-2.45923912563875));
#71031=CARTESIAN_POINT('Ctrl Pts',(3.08540206545313,-1.,-2.45655725437037));
#71032=CARTESIAN_POINT('Ctrl Pts',(3.08540206545313,1.,-2.45655725437037));
#71033=CARTESIAN_POINT('Ctrl Pts',(3.07834472886145,-1.,-2.45382826787795));
#71034=CARTESIAN_POINT('Ctrl Pts',(3.07834472886145,1.,-2.45382826787795));
#71035=CARTESIAN_POINT('Ctrl Pts',(3.0713129052131,-1.,-2.45105688854432));
#71036=CARTESIAN_POINT('Ctrl Pts',(3.0713129052131,1.,-2.45105688854432));
#71037=CARTESIAN_POINT('Ctrl Pts',(3.06431596421422,-1.,-2.44824970516558));
#71038=CARTESIAN_POINT('Ctrl Pts',(3.06431596421422,1.,-2.44824970516558));
#71039=CARTESIAN_POINT('Ctrl Pts',(3.05736242671521,-1.,-2.44541251892568));
#71040=CARTESIAN_POINT('Ctrl Pts',(3.05736242671521,1.,-2.44541251892568));
#71041=CARTESIAN_POINT('Ctrl Pts',(3.05045678021509,-1.,-2.44254768923109));
#71042=CARTESIAN_POINT('Ctrl Pts',(3.05045678021509,1.,-2.44254768923109));
#71043=CARTESIAN_POINT('Ctrl Pts',(3.04359685040545,-1.,-2.43965194061849));
#71044=CARTESIAN_POINT('Ctrl Pts',(3.04359685040545,1.,-2.43965194061849));
#71045=CARTESIAN_POINT('Ctrl Pts',(3.03676949672797,-1.,-2.43671278042394));
#71046=CARTESIAN_POINT('Ctrl Pts',(3.03676949672797,1.,-2.43671278042394));
#71047=CARTESIAN_POINT('Ctrl Pts',(3.02995534946946,-1.,-2.43371241361462));
#71048=CARTESIAN_POINT('Ctrl Pts',(3.02995534946946,1.,-2.43371241361462));
#71049=CARTESIAN_POINT('Ctrl Pts',(3.02313656035977,-1.,-2.43063415586615));
#71050=CARTESIAN_POINT('Ctrl Pts',(3.02313656035977,1.,-2.43063415586615));
#71051=CARTESIAN_POINT('Ctrl Pts',(3.01630420830493,-1.,-2.4274685626416));
#71052=CARTESIAN_POINT('Ctrl Pts',(3.01630420830493,1.,-2.4274685626416));
#71053=CARTESIAN_POINT('Ctrl Pts',(3.00946442616674,-1.,-2.42421849439625));
#71054=CARTESIAN_POINT('Ctrl Pts',(3.00946442616674,1.,-2.42421849439625));
#71055=CARTESIAN_POINT('Ctrl Pts',(3.00264868586038,-1.,-2.42090763946812));
#71056=CARTESIAN_POINT('Ctrl Pts',(3.00264868586038,1.,-2.42090763946812));
#71057=CARTESIAN_POINT('Ctrl Pts',(2.99590509293561,-1.,-2.4175732450056));
#71058=CARTESIAN_POINT('Ctrl Pts',(2.99590509293561,1.,-2.4175732450056));
#71059=CARTESIAN_POINT('Ctrl Pts',(2.98927983005851,-1.,-2.4142506419963));
#71060=CARTESIAN_POINT('Ctrl Pts',(2.98927983005851,1.,-2.4142506419963));
#71061=CARTESIAN_POINT('Ctrl Pts',(2.98280015815132,-1.,-2.41095909342591));
#71062=CARTESIAN_POINT('Ctrl Pts',(2.98280015815132,1.,-2.41095909342591));
#71063=CARTESIAN_POINT('Ctrl Pts',(2.97646002822395,-1.,-2.40768975073691));
#71064=CARTESIAN_POINT('Ctrl Pts',(2.97646002822395,1.,-2.40768975073691));
#71065=CARTESIAN_POINT('Ctrl Pts',(2.97019641312272,-1.,-2.40438604734848));
#71066=CARTESIAN_POINT('Ctrl Pts',(2.97019641312272,1.,-2.40438604734848));
#71067=CARTESIAN_POINT('Ctrl Pts',(2.9639043224018,-1.,-2.40095565711535));
#71068=CARTESIAN_POINT('Ctrl Pts',(2.9639043224018,1.,-2.40095565711535));
#71069=CARTESIAN_POINT('Ctrl Pts',(2.95748006482811,-1.,-2.39730553974412));
#71070=CARTESIAN_POINT('Ctrl Pts',(2.95748006482811,1.,-2.39730553974412));
#71071=CARTESIAN_POINT('Ctrl Pts',(2.95085857128372,-1.,-2.39337207631613));
#71072=CARTESIAN_POINT('Ctrl Pts',(2.95085857128372,1.,-2.39337207631613));
#71073=CARTESIAN_POINT('Ctrl Pts',(2.94404820669135,-1.,-2.38914929090806));
#71074=CARTESIAN_POINT('Ctrl Pts',(2.94404820669135,1.,-2.38914929090806));
#71075=CARTESIAN_POINT('Ctrl Pts',(2.93717903280599,-1.,-2.38472771516476));
#71076=CARTESIAN_POINT('Ctrl Pts',(2.93717903280599,1.,-2.38472771516476));
#71077=CARTESIAN_POINT('Ctrl Pts',(2.93049643640517,-1.,-2.3802898958232));
#71078=CARTESIAN_POINT('Ctrl Pts',(2.93049643640517,1.,-2.3802898958232));
#71079=CARTESIAN_POINT('Ctrl Pts',(2.92430340582912,-1.,-2.37606510524271));
#71080=CARTESIAN_POINT('Ctrl Pts',(2.92430340582912,1.,-2.37606510524271));
#71081=CARTESIAN_POINT('Ctrl Pts',(2.9189150379156,-1.,-2.37229381109939));
#71082=CARTESIAN_POINT('Ctrl Pts',(2.9189150379156,1.,-2.37229381109939));
#71083=CARTESIAN_POINT('Ctrl Pts',(2.91461249883016,-1.,-2.36919161373074));
#71084=CARTESIAN_POINT('Ctrl Pts',(2.91461249883016,1.,-2.36919161373074));
#71085=CARTESIAN_POINT('Ctrl Pts',(2.9115863784165,-1.,-2.36690501170317));
#71086=CARTESIAN_POINT('Ctrl Pts',(2.9115863784165,1.,-2.36690501170317));
#71087=CARTESIAN_POINT('Ctrl Pts',(2.91025813829606,-1.,-2.36578327194396));
#71088=CARTESIAN_POINT('Ctrl Pts',(2.91025813829606,1.,-2.36578327194396));
#71089=CARTESIAN_POINT('Ctrl Pts',(2.90989022547738,-1.,-2.36535052956704));
#71090=CARTESIAN_POINT('Ctrl Pts',(2.90989022547738,1.,-2.36535052956704));
#71091=CARTESIAN_POINT('Ctrl Pts',(2.90992398626098,-1.,-2.36524348105023));
#71092=CARTESIAN_POINT('Ctrl Pts',(2.90992398626098,1.,-2.36524348105023));
#71093=CARTESIAN_POINT('Ctrl Pts',(2.91001063062876,-1.,-2.36523532225181));
#71094=CARTESIAN_POINT('Ctrl Pts',(2.91001063062876,1.,-2.36523532225181));
#71095=CARTESIAN_POINT('',(3.35260583073571,1.,-2.52982887637028));
#71096=CARTESIAN_POINT('Ctrl Pts',(3.35260583073571,1.,-2.52982887637028));
#71097=CARTESIAN_POINT('Ctrl Pts',(3.35105973714426,1.,-2.52954136549357));
#71098=CARTESIAN_POINT('Ctrl Pts',(3.34796903577628,1.,-2.5289632161143));
#71099=CARTESIAN_POINT('Ctrl Pts',(3.34333744117093,1.,-2.52808660916879));
#71100=CARTESIAN_POINT('Ctrl Pts',(3.33717090000955,1.,-2.52689902691551));
#71101=CARTESIAN_POINT('Ctrl Pts',(3.32947762189049,1.,-2.52538321165774));
#71102=CARTESIAN_POINT('Ctrl Pts',(3.32179931079521,1.,-2.52383598396878));
#71103=CARTESIAN_POINT('Ctrl Pts',(3.31413607874727,1.,-2.52225724871375));
#71104=CARTESIAN_POINT('Ctrl Pts',(3.30648808814986,1.,-2.52064689568167));
#71105=CARTESIAN_POINT('Ctrl Pts',(3.29885556387661,1.,-2.51900480700548));
#71106=CARTESIAN_POINT('Ctrl Pts',(3.2912387729863,1.,-2.51733085123316));
#71107=CARTESIAN_POINT('Ctrl Pts',(3.28363799702583,1.,-2.51562487464215));
#71108=CARTESIAN_POINT('Ctrl Pts',(3.27605350473048,1.,-2.51388669270329));
#71109=CARTESIAN_POINT('Ctrl Pts',(3.26848552888271,1.,-2.51211608411539));
#71110=CARTESIAN_POINT('Ctrl Pts',(3.26093423001716,1.,-2.51031277813697));
#71111=CARTESIAN_POINT('Ctrl Pts',(3.25339971461265,1.,-2.50847647070936));
#71112=CARTESIAN_POINT('Ctrl Pts',(3.24588208984042,1.,-2.50660685940645));
#71113=CARTESIAN_POINT('Ctrl Pts',(3.23838151080383,1.,-2.50470367580078));
#71114=CARTESIAN_POINT('Ctrl Pts',(3.23089822320596,1.,-2.50276671338074));
#71115=CARTESIAN_POINT('Ctrl Pts',(3.22343262620387,1.,-2.5007958720187));
#71116=CARTESIAN_POINT('Ctrl Pts',(3.21598526261157,1.,-2.49879114599293));
#71117=CARTESIAN_POINT('Ctrl Pts',(3.2085566984974,1.,-2.49675252647298));
#71118=CARTESIAN_POINT('Ctrl Pts',(3.20114742397549,1.,-2.49467992057726));
#71119=CARTESIAN_POINT('Ctrl Pts',(3.19375775555814,1.,-2.4925730723986));
#71120=CARTESIAN_POINT('Ctrl Pts',(3.18638771282315,1.,-2.49043146334095));
#71121=CARTESIAN_POINT('Ctrl Pts',(3.17903698136678,1.,-2.48825428288243));
#71122=CARTESIAN_POINT('Ctrl Pts',(3.17170518863357,1.,-2.48604065348619));
#71123=CARTESIAN_POINT('Ctrl Pts',(3.16439213290181,1.,-2.48378981792739));
#71124=CARTESIAN_POINT('Ctrl Pts',(3.15709802322735,1.,-2.48150133566568));
#71125=CARTESIAN_POINT('Ctrl Pts',(3.14982373241335,1.,-2.47917529057016));
#71126=CARTESIAN_POINT('Ctrl Pts',(3.14257099546531,1.,-2.47681245356095));
#71127=CARTESIAN_POINT('Ctrl Pts',(3.13534181229282,1.,-2.47441378371923));
#71128=CARTESIAN_POINT('Ctrl Pts',(3.12813790805948,1.,-2.47197997765868));
#71129=CARTESIAN_POINT('Ctrl Pts',(3.12096015766984,1.,-2.4695109894747));
#71130=CARTESIAN_POINT('Ctrl Pts',(3.11380805536124,1.,-2.46700558843507));
#71131=CARTESIAN_POINT('Ctrl Pts',(3.10667907901981,1.,-2.46446082979645));
#71132=CARTESIAN_POINT('Ctrl Pts',(3.09956993697048,1.,-2.4618730850188));
#71133=CARTESIAN_POINT('Ctrl Pts',(3.09247787931881,1.,-2.45923912563875));
#71134=CARTESIAN_POINT('Ctrl Pts',(3.08540206545313,1.,-2.45655725437037));
#71135=CARTESIAN_POINT('Ctrl Pts',(3.07834472886145,1.,-2.45382826787795));
#71136=CARTESIAN_POINT('Ctrl Pts',(3.0713129052131,1.,-2.45105688854432));
#71137=CARTESIAN_POINT('Ctrl Pts',(3.06431596421422,1.,-2.44824970516558));
#71138=CARTESIAN_POINT('Ctrl Pts',(3.05736242671521,1.,-2.44541251892568));
#71139=CARTESIAN_POINT('Ctrl Pts',(3.05045678021509,1.,-2.44254768923109));
#71140=CARTESIAN_POINT('Ctrl Pts',(3.04359685040545,1.,-2.43965194061849));
#71141=CARTESIAN_POINT('Ctrl Pts',(3.03676949672797,1.,-2.43671278042394));
#71142=CARTESIAN_POINT('Ctrl Pts',(3.02995534946946,1.,-2.43371241361462));
#71143=CARTESIAN_POINT('Ctrl Pts',(3.02313656035977,1.,-2.43063415586615));
#71144=CARTESIAN_POINT('Ctrl Pts',(3.01630420830493,1.,-2.4274685626416));
#71145=CARTESIAN_POINT('Ctrl Pts',(3.00946442616674,1.,-2.42421849439625));
#71146=CARTESIAN_POINT('Ctrl Pts',(3.00264868586038,1.,-2.42090763946812));
#71147=CARTESIAN_POINT('Ctrl Pts',(2.99590509293561,1.,-2.4175732450056));
#71148=CARTESIAN_POINT('Ctrl Pts',(2.98927983005851,1.,-2.4142506419963));
#71149=CARTESIAN_POINT('Ctrl Pts',(2.98280015815132,1.,-2.41095909342591));
#71150=CARTESIAN_POINT('Ctrl Pts',(2.97646002822395,1.,-2.40768975073691));
#71151=CARTESIAN_POINT('Ctrl Pts',(2.97019641312272,1.,-2.40438604734848));
#71152=CARTESIAN_POINT('Ctrl Pts',(2.9639043224018,1.,-2.40095565711535));
#71153=CARTESIAN_POINT('Ctrl Pts',(2.95748006482811,1.,-2.39730553974412));
#71154=CARTESIAN_POINT('Ctrl Pts',(2.95085857128372,1.,-2.39337207631613));
#71155=CARTESIAN_POINT('Ctrl Pts',(2.94404820669135,1.,-2.38914929090806));
#71156=CARTESIAN_POINT('Ctrl Pts',(2.93717903280599,1.,-2.38472771516476));
#71157=CARTESIAN_POINT('Ctrl Pts',(2.93049643640517,1.,-2.3802898958232));
#71158=CARTESIAN_POINT('Ctrl Pts',(2.92430340582912,1.,-2.37606510524271));
#71159=CARTESIAN_POINT('Ctrl Pts',(2.9189150379156,1.,-2.37229381109939));
#71160=CARTESIAN_POINT('Ctrl Pts',(2.91461249883016,1.,-2.36919161373074));
#71161=CARTESIAN_POINT('Ctrl Pts',(2.91181344022628,1.,-2.36707658451709));
#71162=CARTESIAN_POINT('Ctrl Pts',(2.91051690822262,1.,-2.36599991765853));
#71163=CARTESIAN_POINT('Ctrl Pts',(2.9100577052777,1.,-2.36553202948741));
#71164=CARTESIAN_POINT('Ctrl Pts',(2.90995756655558,1.,-2.3653621118858));
#71165=CARTESIAN_POINT('Ctrl Pts',(2.90994629141562,1.,-2.36531447826213));
#71166=CARTESIAN_POINT('',(3.35260583073571,0.,-2.52982887637028));
#71167=CARTESIAN_POINT('Ctrl Pts',(3.1487152044751,-1.,-2.03668666247593));
#71168=CARTESIAN_POINT('Ctrl Pts',(3.1487152044751,1.,-2.03668666247593));
#71169=CARTESIAN_POINT('Ctrl Pts',(3.14869618937258,-1.,-2.03660173757879));
#71170=CARTESIAN_POINT('Ctrl Pts',(3.14869618937258,1.,-2.03660173757879));
#71171=CARTESIAN_POINT('Ctrl Pts',(3.14878756590812,-1.,-2.03653654935592));
#71172=CARTESIAN_POINT('Ctrl Pts',(3.14878756590812,1.,-2.03653654935592));
#71173=CARTESIAN_POINT('Ctrl Pts',(3.14931281968048,-1.,-2.03675273049189));
#71174=CARTESIAN_POINT('Ctrl Pts',(3.14931281968048,1.,-2.03675273049189));
#71175=CARTESIAN_POINT('Ctrl Pts',(3.15079010635742,-1.,-2.03766932526445));
#71176=CARTESIAN_POINT('Ctrl Pts',(3.15079010635742,1.,-2.03766932526445));
#71177=CARTESIAN_POINT('Ctrl Pts',(3.15389991674792,-1.,-2.03984073791519));
#71178=CARTESIAN_POINT('Ctrl Pts',(3.15389991674792,1.,-2.03984073791519));
#71179=CARTESIAN_POINT('Ctrl Pts',(3.15817983946367,-1.,-2.04297406404027));
#71180=CARTESIAN_POINT('Ctrl Pts',(3.15817983946367,1.,-2.04297406404027));
#71181=CARTESIAN_POINT('Ctrl Pts',(3.16343165058912,-1.,-2.04693331247446));
#71182=CARTESIAN_POINT('Ctrl Pts',(3.16343165058912,1.,-2.04693331247446));
#71183=CARTESIAN_POINT('Ctrl Pts',(3.16936341689527,-1.,-2.05151770247233));
#71184=CARTESIAN_POINT('Ctrl Pts',(3.16936341689527,1.,-2.05151770247233));
#71185=CARTESIAN_POINT('Ctrl Pts',(3.17564906975371,-1.,-2.05650186773132));
#71186=CARTESIAN_POINT('Ctrl Pts',(3.17564906975371,1.,-2.05650186773132));
#71187=CARTESIAN_POINT('Ctrl Pts',(3.18197692964614,-1.,-2.06166849827101));
#71188=CARTESIAN_POINT('Ctrl Pts',(3.18197692964614,1.,-2.06166849827101));
#71189=CARTESIAN_POINT('Ctrl Pts',(3.18809755562368,-1.,-2.06684062744112));
#71190=CARTESIAN_POINT('Ctrl Pts',(3.18809755562368,1.,-2.06684062744112));
#71191=CARTESIAN_POINT('Ctrl Pts',(3.19388465568252,-1.,-2.07192253497857));
#71192=CARTESIAN_POINT('Ctrl Pts',(3.19388465568252,1.,-2.07192253497857));
#71193=CARTESIAN_POINT('Ctrl Pts',(3.19934132836019,-1.,-2.07690441870722));
#71194=CARTESIAN_POINT('Ctrl Pts',(3.19934132836019,1.,-2.07690441870722));
#71195=CARTESIAN_POINT('Ctrl Pts',(3.2045481863073,-1.,-2.08182850370878));
#71196=CARTESIAN_POINT('Ctrl Pts',(3.2045481863073,1.,-2.08182850370878));
#71197=CARTESIAN_POINT('Ctrl Pts',(3.20962575845463,-1.,-2.08676465517455));
#71198=CARTESIAN_POINT('Ctrl Pts',(3.20962575845463,1.,-2.08676465517455));
#71199=CARTESIAN_POINT('Ctrl Pts',(3.21469429601654,-1.,-2.09178419460443));
#71200=CARTESIAN_POINT('Ctrl Pts',(3.21469429601654,1.,-2.09178419460443));
#71201=CARTESIAN_POINT('Ctrl Pts',(3.21982707347009,-1.,-2.09692958434895));
#71202=CARTESIAN_POINT('Ctrl Pts',(3.21982707347009,1.,-2.09692958434895));
#71203=CARTESIAN_POINT('Ctrl Pts',(3.22503437553434,-1.,-2.10220384298492));
#71204=CARTESIAN_POINT('Ctrl Pts',(3.22503437553434,1.,-2.10220384298492));
#71205=CARTESIAN_POINT('Ctrl Pts',(3.23028945793289,-1.,-2.10758699642451));
#71206=CARTESIAN_POINT('Ctrl Pts',(3.23028945793289,1.,-2.10758699642451));
#71207=CARTESIAN_POINT('Ctrl Pts',(3.23554444767099,-1.,-2.11304604021773));
#71208=CARTESIAN_POINT('Ctrl Pts',(3.23554444767099,1.,-2.11304604021773));
#71209=CARTESIAN_POINT('Ctrl Pts',(3.24074905517293,-1.,-2.11854673326979));
#71210=CARTESIAN_POINT('Ctrl Pts',(3.24074905517293,1.,-2.11854673326979));
#71211=CARTESIAN_POINT('Ctrl Pts',(3.24587102613376,-1.,-2.12406646410962));
#71212=CARTESIAN_POINT('Ctrl Pts',(3.24587102613376,1.,-2.12406646410962));
#71213=CARTESIAN_POINT('Ctrl Pts',(3.25090574494028,-1.,-2.12960028396832));
#71214=CARTESIAN_POINT('Ctrl Pts',(3.25090574494028,1.,-2.12960028396832));
#71215=CARTESIAN_POINT('Ctrl Pts',(3.25586495065054,-1.,-2.13515375878803));
#71216=CARTESIAN_POINT('Ctrl Pts',(3.25586495065054,1.,-2.13515375878803));
#71217=CARTESIAN_POINT('Ctrl Pts',(3.26077002641879,-1.,-2.14073870754264));
#71218=CARTESIAN_POINT('Ctrl Pts',(3.26077002641879,1.,-2.14073870754264));
#71219=CARTESIAN_POINT('Ctrl Pts',(3.26564388189759,-1.,-2.1463680529566));
#71220=CARTESIAN_POINT('Ctrl Pts',(3.26564388189759,1.,-2.1463680529566));
#71221=CARTESIAN_POINT('Ctrl Pts',(3.27050245897228,-1.,-2.15205043199808));
#71222=CARTESIAN_POINT('Ctrl Pts',(3.27050245897228,1.,-2.15205043199808));
#71223=CARTESIAN_POINT('Ctrl Pts',(3.27534954469187,-1.,-2.15778690038347));
#71224=CARTESIAN_POINT('Ctrl Pts',(3.27534954469187,1.,-2.15778690038347));
#71225=CARTESIAN_POINT('Ctrl Pts',(3.280181508414,-1.,-2.16357391934425));
#71226=CARTESIAN_POINT('Ctrl Pts',(3.280181508414,1.,-2.16357391934425));
#71227=CARTESIAN_POINT('Ctrl Pts',(3.28499019979724,-1.,-2.16940517773455));
#71228=CARTESIAN_POINT('Ctrl Pts',(3.28499019979724,1.,-2.16940517773455));
#71229=CARTESIAN_POINT('Ctrl Pts',(3.28976645712568,-1.,-2.17527380048423));
#71230=CARTESIAN_POINT('Ctrl Pts',(3.28976645712568,1.,-2.17527380048423));
#71231=CARTESIAN_POINT('Ctrl Pts',(3.2945036150049,-1.,-2.18117455557065));
#71232=CARTESIAN_POINT('Ctrl Pts',(3.2945036150049,1.,-2.18117455557065));
#71233=CARTESIAN_POINT('Ctrl Pts',(3.29920022557639,-1.,-2.18710556500327));
#71234=CARTESIAN_POINT('Ctrl Pts',(3.29920022557639,1.,-2.18710556500327));
#71235=CARTESIAN_POINT('Ctrl Pts',(3.30385816281831,-1.,-2.19306710376111));
#71236=CARTESIAN_POINT('Ctrl Pts',(3.30385816281831,1.,-2.19306710376111));
#71237=CARTESIAN_POINT('Ctrl Pts',(3.30848134694595,-1.,-2.19906078949923));
#71238=CARTESIAN_POINT('Ctrl Pts',(3.30848134694595,1.,-2.19906078949923));
#71239=CARTESIAN_POINT('Ctrl Pts',(3.31307424608949,-1.,-2.20508863150607));
#71240=CARTESIAN_POINT('Ctrl Pts',(3.31307424608949,1.,-2.20508863150607));
#71241=CARTESIAN_POINT('Ctrl Pts',(3.31764044024235,-1.,-2.21115211847875));
#71242=CARTESIAN_POINT('Ctrl Pts',(3.31764044024235,1.,-2.21115211847875));
#71243=CARTESIAN_POINT('Ctrl Pts',(3.32218125618968,-1.,-2.21725135110898));
#71244=CARTESIAN_POINT('Ctrl Pts',(3.32218125618968,1.,-2.21725135110898));
#71245=CARTESIAN_POINT('Ctrl Pts',(3.3266964672289,-1.,-2.22338548312772));
#71246=CARTESIAN_POINT('Ctrl Pts',(3.3266964672289,1.,-2.22338548312772));
#71247=CARTESIAN_POINT('Ctrl Pts',(3.33118487773611,-1.,-2.22955308907233));
#71248=CARTESIAN_POINT('Ctrl Pts',(3.33118487773611,1.,-2.22955308907233));
#71249=CARTESIAN_POINT('Ctrl Pts',(3.33564495756481,-1.,-2.23575256328812));
#71250=CARTESIAN_POINT('Ctrl Pts',(3.33564495756481,1.,-2.23575256328812));
#71251=CARTESIAN_POINT('Ctrl Pts',(3.34007543738025,-1.,-2.24198249391422));
#71252=CARTESIAN_POINT('Ctrl Pts',(3.34007543738025,1.,-2.24198249391422));
#71253=CARTESIAN_POINT('Ctrl Pts',(3.34447596770723,-1.,-2.24824207678256));
#71254=CARTESIAN_POINT('Ctrl Pts',(3.34447596770723,1.,-2.24824207678256));
#71255=CARTESIAN_POINT('Ctrl Pts',(3.34884690292285,-1.,-2.25453097693483));
#71256=CARTESIAN_POINT('Ctrl Pts',(3.34884690292285,1.,-2.25453097693483));
#71257=CARTESIAN_POINT('Ctrl Pts',(3.35318902552626,-1.,-2.26084915222449));
#71258=CARTESIAN_POINT('Ctrl Pts',(3.35318902552626,1.,-2.26084915222449));
#71259=CARTESIAN_POINT('Ctrl Pts',(3.35750328523061,-1.,-2.2671966857991));
#71260=CARTESIAN_POINT('Ctrl Pts',(3.35750328523061,1.,-2.2671966857991));
#71261=CARTESIAN_POINT('Ctrl Pts',(3.36179055004409,-1.,-2.2735736262093));
#71262=CARTESIAN_POINT('Ctrl Pts',(3.36179055004409,1.,-2.2735736262093));
#71263=CARTESIAN_POINT('Ctrl Pts',(3.36605130713076,-1.,-2.27997979458037));
#71264=CARTESIAN_POINT('Ctrl Pts',(3.36605130713076,1.,-2.27997979458037));
#71265=CARTESIAN_POINT('Ctrl Pts',(3.37028570206488,-1.,-2.28641481081137));
#71266=CARTESIAN_POINT('Ctrl Pts',(3.37028570206488,1.,-2.28641481081137));
#71267=CARTESIAN_POINT('Ctrl Pts',(3.37449367172826,-1.,-2.29287818007393));
#71268=CARTESIAN_POINT('Ctrl Pts',(3.37449367172826,1.,-2.29287818007393));
#71269=CARTESIAN_POINT('Ctrl Pts',(3.37867504959433,-1.,-2.29936936127624));
#71270=CARTESIAN_POINT('Ctrl Pts',(3.37867504959433,1.,-2.29936936127624));
#71271=CARTESIAN_POINT('Ctrl Pts',(3.3828296733661,-1.,-2.30588783640343));
#71272=CARTESIAN_POINT('Ctrl Pts',(3.3828296733661,1.,-2.30588783640343));
#71273=CARTESIAN_POINT('Ctrl Pts',(3.38695751492462,-1.,-2.31243319489367));
#71274=CARTESIAN_POINT('Ctrl Pts',(3.38695751492462,1.,-2.31243319489367));
#71275=CARTESIAN_POINT('Ctrl Pts',(3.39105869474822,-1.,-2.31900513925424));
#71276=CARTESIAN_POINT('Ctrl Pts',(3.39105869474822,1.,-2.31900513925424));
#71277=CARTESIAN_POINT('Ctrl Pts',(3.39513342019756,-1.,-2.3256034390248));
#71278=CARTESIAN_POINT('Ctrl Pts',(3.39513342019756,1.,-2.3256034390248));
#71279=CARTESIAN_POINT('Ctrl Pts',(3.39918194577956,-1.,-2.33222789882489));
#71280=CARTESIAN_POINT('Ctrl Pts',(3.39918194577956,1.,-2.33222789882489));
#71281=CARTESIAN_POINT('Ctrl Pts',(3.40320452776743,-1.,-2.33887832342782));
#71282=CARTESIAN_POINT('Ctrl Pts',(3.40320452776743,1.,-2.33887832342782));
#71283=CARTESIAN_POINT('Ctrl Pts',(3.40720137404297,-1.,-2.34555447649188));
#71284=CARTESIAN_POINT('Ctrl Pts',(3.40720137404297,1.,-2.34555447649188));
#71285=CARTESIAN_POINT('Ctrl Pts',(3.41117262314119,-1.,-2.35225606824109));
#71286=CARTESIAN_POINT('Ctrl Pts',(3.41117262314119,1.,-2.35225606824109));
#71287=CARTESIAN_POINT('Ctrl Pts',(3.41511836751469,-1.,-2.35898278606946));
#71288=CARTESIAN_POINT('Ctrl Pts',(3.41511836751469,1.,-2.35898278606946));
#71289=CARTESIAN_POINT('Ctrl Pts',(3.41903866635852,-1.,-2.36573431470642));
#71290=CARTESIAN_POINT('Ctrl Pts',(3.41903866635852,1.,-2.36573431470642));
#71291=CARTESIAN_POINT('Ctrl Pts',(3.42293356216511,-1.,-2.37251035954292));
#71292=CARTESIAN_POINT('Ctrl Pts',(3.42293356216511,1.,-2.37251035954292));
#71293=CARTESIAN_POINT('Ctrl Pts',(3.42680309754399,-1.,-2.37931067028926));
#71294=CARTESIAN_POINT('Ctrl Pts',(3.42680309754399,1.,-2.37931067028926));
#71295=CARTESIAN_POINT('Ctrl Pts',(3.43064732712919,-1.,-2.38613505843552));
#71296=CARTESIAN_POINT('Ctrl Pts',(3.43064732712919,1.,-2.38613505843552));
#71297=CARTESIAN_POINT('Ctrl Pts',(3.4344663067854,-1.,-2.39298338804493));
#71298=CARTESIAN_POINT('Ctrl Pts',(3.4344663067854,1.,-2.39298338804493));
#71299=CARTESIAN_POINT('Ctrl Pts',(3.43750133064416,-1.,-2.39848113410292));
#71300=CARTESIAN_POINT('Ctrl Pts',(3.43750133064416,1.,-2.39848113410292));
#71301=CARTESIAN_POINT('Ctrl Pts',(3.43976627484234,-1.,-2.40261515589405));
#71302=CARTESIAN_POINT('Ctrl Pts',(3.43976627484234,1.,-2.40261515589405));
#71303=CARTESIAN_POINT('Ctrl Pts',(3.44127120683039,-1.,-2.4053759295909));
#71304=CARTESIAN_POINT('Ctrl Pts',(3.44127120683039,1.,-2.4053759295909));
#71305=CARTESIAN_POINT('Ctrl Pts',(3.44202241512147,-1.,-2.40675750623143));
#71306=CARTESIAN_POINT('Ctrl Pts',(3.44202241512147,1.,-2.40675750623143));
#71307=CARTESIAN_POINT('',(3.14877060440327,1.,-2.03660101169715));
#71308=CARTESIAN_POINT('Ctrl Pts',(3.14877060440327,-1.,-2.03660101169715));
#71309=CARTESIAN_POINT('Ctrl Pts',(3.14877060440327,-0.666666666666667,
-2.03660101169715));
#71310=CARTESIAN_POINT('Ctrl Pts',(3.14877060440327,-0.333333333333333,
-2.03660101169715));
#71311=CARTESIAN_POINT('Ctrl Pts',(3.14877060440327,0.333333333333333,-2.03660101169715));
#71312=CARTESIAN_POINT('Ctrl Pts',(3.14877060440328,0.666666666666667,-2.03660101169714));
#71313=CARTESIAN_POINT('Ctrl Pts',(3.14877060440328,1.,-2.03660101169714));
#71314=CARTESIAN_POINT('',(3.44202241512147,1.,-2.40675750623143));
#71315=CARTESIAN_POINT('',(3.44202241512147,0.,-2.40675750623143));
#71316=CARTESIAN_POINT('Ctrl Pts',(3.14877060440327,1.,-2.03660101169715));
#71317=CARTESIAN_POINT('Ctrl Pts',(3.14881939088124,1.,-2.03659701539259));
#71318=CARTESIAN_POINT('Ctrl Pts',(3.1490119366901,1.,-2.03663974554932));
#71319=CARTESIAN_POINT('Ctrl Pts',(3.14959882629804,1.,-2.03693188810544));
#71320=CARTESIAN_POINT('Ctrl Pts',(3.15102344775328,1.,-2.03783225495961));
#71321=CARTESIAN_POINT('Ctrl Pts',(3.15389991674792,1.,-2.03984073791519));
#71322=CARTESIAN_POINT('Ctrl Pts',(3.15817983946367,1.,-2.04297406404027));
#71323=CARTESIAN_POINT('Ctrl Pts',(3.16343165058912,1.,-2.04693331247446));
#71324=CARTESIAN_POINT('Ctrl Pts',(3.16936341689527,1.,-2.05151770247233));
#71325=CARTESIAN_POINT('Ctrl Pts',(3.17564906975371,1.,-2.05650186773132));
#71326=CARTESIAN_POINT('Ctrl Pts',(3.18197692964614,1.,-2.06166849827101));
#71327=CARTESIAN_POINT('Ctrl Pts',(3.18809755562368,1.,-2.06684062744112));
#71328=CARTESIAN_POINT('Ctrl Pts',(3.19388465568252,1.,-2.07192253497857));
#71329=CARTESIAN_POINT('Ctrl Pts',(3.19934132836019,1.,-2.07690441870722));
#71330=CARTESIAN_POINT('Ctrl Pts',(3.2045481863073,1.,-2.08182850370878));
#71331=CARTESIAN_POINT('Ctrl Pts',(3.20962575845463,1.,-2.08676465517455));
#71332=CARTESIAN_POINT('Ctrl Pts',(3.21469429601654,1.,-2.09178419460443));
#71333=CARTESIAN_POINT('Ctrl Pts',(3.21982707347009,1.,-2.09692958434895));
#71334=CARTESIAN_POINT('Ctrl Pts',(3.22503437553434,1.,-2.10220384298492));
#71335=CARTESIAN_POINT('Ctrl Pts',(3.23028945793289,1.,-2.10758699642451));
#71336=CARTESIAN_POINT('Ctrl Pts',(3.23554444767099,1.,-2.11304604021773));
#71337=CARTESIAN_POINT('Ctrl Pts',(3.24074905517293,1.,-2.11854673326979));
#71338=CARTESIAN_POINT('Ctrl Pts',(3.24587102613376,1.,-2.12406646410962));
#71339=CARTESIAN_POINT('Ctrl Pts',(3.25090574494028,1.,-2.12960028396832));
#71340=CARTESIAN_POINT('Ctrl Pts',(3.25586495065054,1.,-2.13515375878803));
#71341=CARTESIAN_POINT('Ctrl Pts',(3.26077002641879,1.,-2.14073870754264));
#71342=CARTESIAN_POINT('Ctrl Pts',(3.26564388189759,1.,-2.1463680529566));
#71343=CARTESIAN_POINT('Ctrl Pts',(3.27050245897228,1.,-2.15205043199808));
#71344=CARTESIAN_POINT('Ctrl Pts',(3.27534954469187,1.,-2.15778690038347));
#71345=CARTESIAN_POINT('Ctrl Pts',(3.280181508414,1.,-2.16357391934425));
#71346=CARTESIAN_POINT('Ctrl Pts',(3.28499019979724,1.,-2.16940517773455));
#71347=CARTESIAN_POINT('Ctrl Pts',(3.28976645712568,1.,-2.17527380048423));
#71348=CARTESIAN_POINT('Ctrl Pts',(3.2945036150049,1.,-2.18117455557065));
#71349=CARTESIAN_POINT('Ctrl Pts',(3.29920022557639,1.,-2.18710556500327));
#71350=CARTESIAN_POINT('Ctrl Pts',(3.30385816281831,1.,-2.19306710376111));
#71351=CARTESIAN_POINT('Ctrl Pts',(3.30848134694595,1.,-2.19906078949923));
#71352=CARTESIAN_POINT('Ctrl Pts',(3.31307424608949,1.,-2.20508863150607));
#71353=CARTESIAN_POINT('Ctrl Pts',(3.31764044024235,1.,-2.21115211847875));
#71354=CARTESIAN_POINT('Ctrl Pts',(3.32218125618968,1.,-2.21725135110898));
#71355=CARTESIAN_POINT('Ctrl Pts',(3.3266964672289,1.,-2.22338548312772));
#71356=CARTESIAN_POINT('Ctrl Pts',(3.33118487773611,1.,-2.22955308907233));
#71357=CARTESIAN_POINT('Ctrl Pts',(3.33564495756481,1.,-2.23575256328812));
#71358=CARTESIAN_POINT('Ctrl Pts',(3.34007543738025,1.,-2.24198249391422));
#71359=CARTESIAN_POINT('Ctrl Pts',(3.34447596770723,1.,-2.24824207678256));
#71360=CARTESIAN_POINT('Ctrl Pts',(3.34884690292285,1.,-2.25453097693483));
#71361=CARTESIAN_POINT('Ctrl Pts',(3.35318902552626,1.,-2.26084915222449));
#71362=CARTESIAN_POINT('Ctrl Pts',(3.35750328523061,1.,-2.2671966857991));
#71363=CARTESIAN_POINT('Ctrl Pts',(3.36179055004409,1.,-2.2735736262093));
#71364=CARTESIAN_POINT('Ctrl Pts',(3.36605130713076,1.,-2.27997979458037));
#71365=CARTESIAN_POINT('Ctrl Pts',(3.37028570206488,1.,-2.28641481081137));
#71366=CARTESIAN_POINT('Ctrl Pts',(3.37449367172826,1.,-2.29287818007393));
#71367=CARTESIAN_POINT('Ctrl Pts',(3.37867504959433,1.,-2.29936936127624));
#71368=CARTESIAN_POINT('Ctrl Pts',(3.3828296733661,1.,-2.30588783640343));
#71369=CARTESIAN_POINT('Ctrl Pts',(3.38695751492462,1.,-2.31243319489367));
#71370=CARTESIAN_POINT('Ctrl Pts',(3.39105869474822,1.,-2.31900513925424));
#71371=CARTESIAN_POINT('Ctrl Pts',(3.39513342019756,1.,-2.3256034390248));
#71372=CARTESIAN_POINT('Ctrl Pts',(3.39918194577956,1.,-2.33222789882489));
#71373=CARTESIAN_POINT('Ctrl Pts',(3.40320452776743,1.,-2.33887832342782));
#71374=CARTESIAN_POINT('Ctrl Pts',(3.40720137404297,1.,-2.34555447649188));
#71375=CARTESIAN_POINT('Ctrl Pts',(3.41117262314119,1.,-2.35225606824109));
#71376=CARTESIAN_POINT('Ctrl Pts',(3.41511836751469,1.,-2.35898278606946));
#71377=CARTESIAN_POINT('Ctrl Pts',(3.41903866635852,1.,-2.36573431470642));
#71378=CARTESIAN_POINT('Ctrl Pts',(3.42293356216511,1.,-2.37251035954292));
#71379=CARTESIAN_POINT('Ctrl Pts',(3.42680309754399,1.,-2.37931067028926));
#71380=CARTESIAN_POINT('Ctrl Pts',(3.43064732712919,1.,-2.38613505843552));
#71381=CARTESIAN_POINT('Ctrl Pts',(3.4344663067854,1.,-2.39298338804493));
#71382=CARTESIAN_POINT('Ctrl Pts',(3.43750133064416,1.,-2.39848113410292));
#71383=CARTESIAN_POINT('Ctrl Pts',(3.43976627484234,1.,-2.40261515589405));
#71384=CARTESIAN_POINT('Ctrl Pts',(3.44127120683039,1.,-2.4053759295909));
#71385=CARTESIAN_POINT('Ctrl Pts',(3.44202241512147,1.,-2.40675750623143));
#71386=CARTESIAN_POINT('Origin',(3.44202241512147,0.,-2.40675750623143));
#71387=CARTESIAN_POINT('',(3.35260583073571,1.,-2.52982887637028));
#71388=CARTESIAN_POINT('Origin',(0.,0.,0.));
#71389=CARTESIAN_POINT('',(3.24413672884812,1.,-1.88097764062697));
#71390=CARTESIAN_POINT('Origin',(0.,1.,0.));
#71391=CARTESIAN_POINT('Ctrl Pts',(3.24413672884812,1.,-1.88097764062697));
#71392=CARTESIAN_POINT('Ctrl Pts',(3.24413672884812,0.666666666666667,-1.88097764062697));
#71393=CARTESIAN_POINT('Ctrl Pts',(3.24413672884812,0.333333333333333,-1.88097764062697));
#71394=CARTESIAN_POINT('Ctrl Pts',(3.24413672884812,-0.333333333333333,
-1.88097764062697));
#71395=CARTESIAN_POINT('Ctrl Pts',(3.24413672884812,-0.666666666666667,
-1.88097764062697));
#71396=CARTESIAN_POINT('Ctrl Pts',(3.24413672884812,-1.,-1.88097764062697));
#71397=CARTESIAN_POINT('Ctrl Pts',(3.70708211654725,-1.,-1.97421938526992));
#71398=CARTESIAN_POINT('Ctrl Pts',(3.70708211654725,1.,-1.97421938526992));
#71399=CARTESIAN_POINT('Ctrl Pts',(3.70551008132332,-1.,-1.97417727645308));
#71400=CARTESIAN_POINT('Ctrl Pts',(3.70551008132332,1.,-1.97417727645308));
#71401=CARTESIAN_POINT('Ctrl Pts',(3.70236698912904,-1.,-1.97408973726715));
#71402=CARTESIAN_POINT('Ctrl Pts',(3.70236698912904,1.,-1.97408973726715));
#71403=CARTESIAN_POINT('Ctrl Pts',(3.6976552856004,-1.,-1.97394846383216));
#71404=CARTESIAN_POINT('Ctrl Pts',(3.6976552856004,1.,-1.97394846383216));
#71405=CARTESIAN_POINT('Ctrl Pts',(3.69137888599902,-1.,-1.97374016225483));
#71406=CARTESIAN_POINT('Ctrl Pts',(3.69137888599902,1.,-1.97374016225483));
#71407=CARTESIAN_POINT('Ctrl Pts',(3.68354319915092,-1.,-1.97344650304519));
#71408=CARTESIAN_POINT('Ctrl Pts',(3.68354319915092,1.,-1.97344650304519));
#71409=CARTESIAN_POINT('Ctrl Pts',(3.67571738107084,-1.,-1.97311947678517));
#71410=CARTESIAN_POINT('Ctrl Pts',(3.67571738107084,1.,-1.97311947678517));
#71411=CARTESIAN_POINT('Ctrl Pts',(3.66790152752075,-1.,-1.97275897198678));
#71412=CARTESIAN_POINT('Ctrl Pts',(3.66790152752075,1.,-1.97275897198678));
#71413=CARTESIAN_POINT('Ctrl Pts',(3.6600957816636,-1.,-1.9723648543905));
#71414=CARTESIAN_POINT('Ctrl Pts',(3.6600957816636,1.,-1.9723648543905));
#71415=CARTESIAN_POINT('Ctrl Pts',(3.652300347166,-1.,-1.9719369724024));
#71416=CARTESIAN_POINT('Ctrl Pts',(3.652300347166,1.,-1.9719369724024));
#71417=CARTESIAN_POINT('Ctrl Pts',(3.64451546723514,-1.,-1.97147515441164));
#71418=CARTESIAN_POINT('Ctrl Pts',(3.64451546723514,1.,-1.97147515441164));
#71419=CARTESIAN_POINT('Ctrl Pts',(3.63674139590412,-1.,-1.97097920454464));
#71420=CARTESIAN_POINT('Ctrl Pts',(3.63674139590412,1.,-1.97097920454464));
#71421=CARTESIAN_POINT('Ctrl Pts',(3.62897836973293,-1.,-1.97044889850463));
#71422=CARTESIAN_POINT('Ctrl Pts',(3.62897836973293,1.,-1.97044889850463));
#71423=CARTESIAN_POINT('Ctrl Pts',(3.62122658401893,-1.,-1.96988398129978));
#71424=CARTESIAN_POINT('Ctrl Pts',(3.62122658401893,1.,-1.96988398129978));
#71425=CARTESIAN_POINT('Ctrl Pts',(3.61348615496704,-1.,-1.96928416040877));
#71426=CARTESIAN_POINT('Ctrl Pts',(3.61348615496704,1.,-1.96928416040877));
#71427=CARTESIAN_POINT('Ctrl Pts',(3.60575714017989,-1.,-1.9686491188594));
#71428=CARTESIAN_POINT('Ctrl Pts',(3.60575714017989,1.,-1.9686491188594));
#71429=CARTESIAN_POINT('Ctrl Pts',(3.59803959819938,-1.,-1.96797854118369));
#71430=CARTESIAN_POINT('Ctrl Pts',(3.59803959819938,1.,-1.96797854118369));
#71431=CARTESIAN_POINT('Ctrl Pts',(3.59033364022801,-1.,-1.96727213799544));
#71432=CARTESIAN_POINT('Ctrl Pts',(3.59033364022801,1.,-1.96727213799544));
#71433=CARTESIAN_POINT('Ctrl Pts',(3.58263947663829,-1.,-1.96652966688911));
#71434=CARTESIAN_POINT('Ctrl Pts',(3.58263947663829,1.,-1.96652966688911));
#71435=CARTESIAN_POINT('Ctrl Pts',(3.57495748600959,-1.,-1.96575096652789));
#71436=CARTESIAN_POINT('Ctrl Pts',(3.57495748600959,1.,-1.96575096652789));
#71437=CARTESIAN_POINT('Ctrl Pts',(3.56728820357791,-1.,-1.96493594634567));
#71438=CARTESIAN_POINT('Ctrl Pts',(3.56728820357791,1.,-1.96493594634567));
#71439=CARTESIAN_POINT('Ctrl Pts',(3.55963218706096,-1.,-1.96408450906812));
#71440=CARTESIAN_POINT('Ctrl Pts',(3.55963218706096,1.,-1.96408450906812));
#71441=CARTESIAN_POINT('Ctrl Pts',(3.55198990600886,-1.,-1.96319648628644));
#71442=CARTESIAN_POINT('Ctrl Pts',(3.55198990600886,1.,-1.96319648628644));
#71443=CARTESIAN_POINT('Ctrl Pts',(3.54436163300443,-1.,-1.96227157573067));
#71444=CARTESIAN_POINT('Ctrl Pts',(3.54436163300443,1.,-1.96227157573067));
#71445=CARTESIAN_POINT('Ctrl Pts',(3.53674730625813,-1.,-1.96130926212689));
#71446=CARTESIAN_POINT('Ctrl Pts',(3.53674730625813,1.,-1.96130926212689));
#71447=CARTESIAN_POINT('Ctrl Pts',(3.52914648844351,-1.,-1.96030879411566));
#71448=CARTESIAN_POINT('Ctrl Pts',(3.52914648844351,1.,-1.96030879411566));
#71449=CARTESIAN_POINT('Ctrl Pts',(3.52155867431486,-1.,-1.95926936324461));
#71450=CARTESIAN_POINT('Ctrl Pts',(3.52155867431486,1.,-1.95926936324461));
#71451=CARTESIAN_POINT('Ctrl Pts',(3.51398354617794,-1.,-1.95819025316779));
#71452=CARTESIAN_POINT('Ctrl Pts',(3.51398354617794,1.,-1.95819025316779));
#71453=CARTESIAN_POINT('Ctrl Pts',(3.50642124159909,-1.,-1.95707099606511));
#71454=CARTESIAN_POINT('Ctrl Pts',(3.50642124159909,1.,-1.95707099606511));
#71455=CARTESIAN_POINT('Ctrl Pts',(3.49887263575583,-1.,-1.95591153823661));
#71456=CARTESIAN_POINT('Ctrl Pts',(3.49887263575583,1.,-1.95591153823661));
#71457=CARTESIAN_POINT('Ctrl Pts',(3.49133956289133,-1.,-1.95471236969643));
#71458=CARTESIAN_POINT('Ctrl Pts',(3.49133956289133,1.,-1.95471236969643));
#71459=CARTESIAN_POINT('Ctrl Pts',(3.48382414832634,-1.,-1.95347412486309));
#71460=CARTESIAN_POINT('Ctrl Pts',(3.48382414832634,1.,-1.95347412486309));
#71461=CARTESIAN_POINT('Ctrl Pts',(3.47632820495921,-1.,-1.95219722189876));
#71462=CARTESIAN_POINT('Ctrl Pts',(3.47632820495921,1.,-1.95219722189876));
#71463=CARTESIAN_POINT('Ctrl Pts',(3.46885258974191,-1.,-1.95088147859877));
#71464=CARTESIAN_POINT('Ctrl Pts',(3.46885258974191,1.,-1.95088147859877));
#71465=CARTESIAN_POINT('Ctrl Pts',(3.46139661060962,-1.,-1.94952575850197));
#71466=CARTESIAN_POINT('Ctrl Pts',(3.46139661060962,1.,-1.94952575850197));
#71467=CARTESIAN_POINT('Ctrl Pts',(3.45395731584051,-1.,-1.94812754766524));
#71468=CARTESIAN_POINT('Ctrl Pts',(3.45395731584051,1.,-1.94812754766524));
#71469=CARTESIAN_POINT('Ctrl Pts',(3.44653088665681,-1.,-1.94668377715329));
#71470=CARTESIAN_POINT('Ctrl Pts',(3.44653088665681,1.,-1.94668377715329));
#71471=CARTESIAN_POINT('Ctrl Pts',(3.43911410197687,-1.,-1.94519168842879));
#71472=CARTESIAN_POINT('Ctrl Pts',(3.43911410197687,1.,-1.94519168842879));
#71473=CARTESIAN_POINT('Ctrl Pts',(3.43170586602434,-1.,-1.94364973660284));
#71474=CARTESIAN_POINT('Ctrl Pts',(3.43170586602434,1.,-1.94364973660284));
#71475=CARTESIAN_POINT('Ctrl Pts',(3.42430850941503,-1.,-1.94205835913696));
#71476=CARTESIAN_POINT('Ctrl Pts',(3.42430850941503,1.,-1.94205835913696));
#71477=CARTESIAN_POINT('Ctrl Pts',(3.41692971994096,-1.,-1.94042111965246));
#71478=CARTESIAN_POINT('Ctrl Pts',(3.41692971994096,1.,-1.94042111965246));
#71479=CARTESIAN_POINT('Ctrl Pts',(3.40957978266642,-1.,-1.93874306008143));
#71480=CARTESIAN_POINT('Ctrl Pts',(3.40957978266642,1.,-1.93874306008143));
#71481=CARTESIAN_POINT('Ctrl Pts',(3.40226802104109,-1.,-1.93702857723098));
#71482=CARTESIAN_POINT('Ctrl Pts',(3.40226802104109,1.,-1.93702857723098));
#71483=CARTESIAN_POINT('Ctrl Pts',(3.39499923640795,-1.,-1.93527929945985));
#71484=CARTESIAN_POINT('Ctrl Pts',(3.39499923640795,1.,-1.93527929945985));
#71485=CARTESIAN_POINT('Ctrl Pts',(3.38777076883256,-1.,-1.93349233176788));
#71486=CARTESIAN_POINT('Ctrl Pts',(3.38777076883256,1.,-1.93349233176788));
#71487=CARTESIAN_POINT('Ctrl Pts',(3.3805676852555,-1.,-1.93165739093276));
#71488=CARTESIAN_POINT('Ctrl Pts',(3.3805676852555,1.,-1.93165739093276));
#71489=CARTESIAN_POINT('Ctrl Pts',(3.37336807068043,-1.,-1.92975993109877));
#71490=CARTESIAN_POINT('Ctrl Pts',(3.37336807068043,1.,-1.92975993109877));
#71491=CARTESIAN_POINT('Ctrl Pts',(3.36615168657567,-1.,-1.92778626543786));
#71492=CARTESIAN_POINT('Ctrl Pts',(3.36615168657567,1.,-1.92778626543786));
#71493=CARTESIAN_POINT('Ctrl Pts',(3.35890824422965,-1.,-1.92572846125756));
#71494=CARTESIAN_POINT('Ctrl Pts',(3.35890824422965,1.,-1.92572846125756));
#71495=CARTESIAN_POINT('Ctrl Pts',(3.35164424847223,-1.,-1.92358838440528));
#71496=CARTESIAN_POINT('Ctrl Pts',(3.35164424847223,1.,-1.92358838440528));
#71497=CARTESIAN_POINT('Ctrl Pts',(3.34439448941961,-1.,-1.92138450828404));
#71498=CARTESIAN_POINT('Ctrl Pts',(3.34439448941961,1.,-1.92138450828404));
#71499=CARTESIAN_POINT('Ctrl Pts',(3.33721230710012,-1.,-1.9191460961021));
#71500=CARTESIAN_POINT('Ctrl Pts',(3.33721230710012,1.,-1.9191460961021));
#71501=CARTESIAN_POINT('Ctrl Pts',(3.33014884257873,-1.,-1.91690081930332));
#71502=CARTESIAN_POINT('Ctrl Pts',(3.33014884257873,1.,-1.91690081930332));
#71503=CARTESIAN_POINT('Ctrl Pts',(3.32323403454535,-1.,-1.91466343916628));
#71504=CARTESIAN_POINT('Ctrl Pts',(3.32323403454535,1.,-1.91466343916628));
#71505=CARTESIAN_POINT('Ctrl Pts',(3.31646052426364,-1.,-1.91242616234442));
#71506=CARTESIAN_POINT('Ctrl Pts',(3.31646052426364,1.,-1.91242616234442));
#71507=CARTESIAN_POINT('Ctrl Pts',(3.30975721158596,-1.,-1.91014297830446));
#71508=CARTESIAN_POINT('Ctrl Pts',(3.30975721158596,1.,-1.91014297830446));
#71509=CARTESIAN_POINT('Ctrl Pts',(3.30300595568195,-1.,-1.90773912171341));
#71510=CARTESIAN_POINT('Ctrl Pts',(3.30300595568195,1.,-1.90773912171341));
#71511=CARTESIAN_POINT('Ctrl Pts',(3.29608978722113,-1.,-1.90513891864087));
#71512=CARTESIAN_POINT('Ctrl Pts',(3.29608978722113,1.,-1.90513891864087));
#71513=CARTESIAN_POINT('Ctrl Pts',(3.2889344860029,-1.,-1.90228971247527));
#71514=CARTESIAN_POINT('Ctrl Pts',(3.2889344860029,1.,-1.90228971247527));
#71515=CARTESIAN_POINT('Ctrl Pts',(3.28154737912352,-1.,-1.89918429230462));
#71516=CARTESIAN_POINT('Ctrl Pts',(3.28154737912352,1.,-1.89918429230462));
#71517=CARTESIAN_POINT('Ctrl Pts',(3.27407108933139,-1.,-1.89589172903793));
#71518=CARTESIAN_POINT('Ctrl Pts',(3.27407108933139,1.,-1.89589172903793));
#71519=CARTESIAN_POINT('Ctrl Pts',(3.26677653888676,-1.,-1.89255393500965));
#71520=CARTESIAN_POINT('Ctrl Pts',(3.26677653888676,1.,-1.89255393500965));
#71521=CARTESIAN_POINT('Ctrl Pts',(3.25999885193947,-1.,-1.88934996203698));
#71522=CARTESIAN_POINT('Ctrl Pts',(3.25999885193947,1.,-1.88934996203698));
#71523=CARTESIAN_POINT('Ctrl Pts',(3.25408686339463,-1.,-1.88646802523466));
#71524=CARTESIAN_POINT('Ctrl Pts',(3.25408686339463,1.,-1.88646802523466));
#71525=CARTESIAN_POINT('Ctrl Pts',(3.24935200511918,-1.,-1.88407708646357));
#71526=CARTESIAN_POINT('Ctrl Pts',(3.24935200511918,1.,-1.88407708646357));
#71527=CARTESIAN_POINT('Ctrl Pts',(3.24600543790443,-1.,-1.88229202582941));
#71528=CARTESIAN_POINT('Ctrl Pts',(3.24600543790443,1.,-1.88229202582941));
#71529=CARTESIAN_POINT('Ctrl Pts',(3.24451807186481,-1.,-1.88139187908074));
#71530=CARTESIAN_POINT('Ctrl Pts',(3.24451807186481,1.,-1.88139187908074));
#71531=CARTESIAN_POINT('Ctrl Pts',(3.24408699284121,-1.,-1.88102201872555));
#71532=CARTESIAN_POINT('Ctrl Pts',(3.24408699284121,1.,-1.88102201872555));
#71533=CARTESIAN_POINT('Ctrl Pts',(3.24410359189609,-1.,-1.88091100680349));
#71534=CARTESIAN_POINT('Ctrl Pts',(3.24410359189609,1.,-1.88091100680349));
#71535=CARTESIAN_POINT('Ctrl Pts',(3.24418789321065,-1.,-1.8808893942881));
#71536=CARTESIAN_POINT('Ctrl Pts',(3.24418789321065,1.,-1.8808893942881));
#71537=CARTESIAN_POINT('',(3.70708211654725,1.,-1.97421938526992));
#71538=CARTESIAN_POINT('Ctrl Pts',(3.70708211654725,1.,-1.97421938526992));
#71539=CARTESIAN_POINT('Ctrl Pts',(3.70551008132332,1.,-1.97417727645308));
#71540=CARTESIAN_POINT('Ctrl Pts',(3.70236698912904,1.,-1.97408973726715));
#71541=CARTESIAN_POINT('Ctrl Pts',(3.6976552856004,1.,-1.97394846383216));
#71542=CARTESIAN_POINT('Ctrl Pts',(3.69137888599902,1.,-1.97374016225483));
#71543=CARTESIAN_POINT('Ctrl Pts',(3.68354319915092,1.,-1.97344650304519));
#71544=CARTESIAN_POINT('Ctrl Pts',(3.67571738107084,1.,-1.97311947678517));
#71545=CARTESIAN_POINT('Ctrl Pts',(3.66790152752075,1.,-1.97275897198678));
#71546=CARTESIAN_POINT('Ctrl Pts',(3.6600957816636,1.,-1.9723648543905));
#71547=CARTESIAN_POINT('Ctrl Pts',(3.652300347166,1.,-1.9719369724024));
#71548=CARTESIAN_POINT('Ctrl Pts',(3.64451546723514,1.,-1.97147515441164));
#71549=CARTESIAN_POINT('Ctrl Pts',(3.63674139590412,1.,-1.97097920454464));
#71550=CARTESIAN_POINT('Ctrl Pts',(3.62897836973293,1.,-1.97044889850463));
#71551=CARTESIAN_POINT('Ctrl Pts',(3.62122658401893,1.,-1.96988398129978));
#71552=CARTESIAN_POINT('Ctrl Pts',(3.61348615496704,1.,-1.96928416040877));
#71553=CARTESIAN_POINT('Ctrl Pts',(3.60575714017989,1.,-1.9686491188594));
#71554=CARTESIAN_POINT('Ctrl Pts',(3.59803959819938,1.,-1.96797854118369));
#71555=CARTESIAN_POINT('Ctrl Pts',(3.59033364022801,1.,-1.96727213799544));
#71556=CARTESIAN_POINT('Ctrl Pts',(3.58263947663829,1.,-1.96652966688911));
#71557=CARTESIAN_POINT('Ctrl Pts',(3.57495748600959,1.,-1.96575096652789));
#71558=CARTESIAN_POINT('Ctrl Pts',(3.56728820357791,1.,-1.96493594634567));
#71559=CARTESIAN_POINT('Ctrl Pts',(3.55963218706096,1.,-1.96408450906812));
#71560=CARTESIAN_POINT('Ctrl Pts',(3.55198990600886,1.,-1.96319648628644));
#71561=CARTESIAN_POINT('Ctrl Pts',(3.54436163300443,1.,-1.96227157573067));
#71562=CARTESIAN_POINT('Ctrl Pts',(3.53674730625813,1.,-1.96130926212689));
#71563=CARTESIAN_POINT('Ctrl Pts',(3.52914648844351,1.,-1.96030879411566));
#71564=CARTESIAN_POINT('Ctrl Pts',(3.52155867431486,1.,-1.95926936324461));
#71565=CARTESIAN_POINT('Ctrl Pts',(3.51398354617794,1.,-1.95819025316779));
#71566=CARTESIAN_POINT('Ctrl Pts',(3.50642124159909,1.,-1.95707099606511));
#71567=CARTESIAN_POINT('Ctrl Pts',(3.49887263575583,1.,-1.95591153823661));
#71568=CARTESIAN_POINT('Ctrl Pts',(3.49133956289133,1.,-1.95471236969643));
#71569=CARTESIAN_POINT('Ctrl Pts',(3.48382414832634,1.,-1.95347412486309));
#71570=CARTESIAN_POINT('Ctrl Pts',(3.47632820495921,1.,-1.95219722189876));
#71571=CARTESIAN_POINT('Ctrl Pts',(3.46885258974191,1.,-1.95088147859877));
#71572=CARTESIAN_POINT('Ctrl Pts',(3.46139661060962,1.,-1.94952575850197));
#71573=CARTESIAN_POINT('Ctrl Pts',(3.45395731584051,1.,-1.94812754766524));
#71574=CARTESIAN_POINT('Ctrl Pts',(3.44653088665681,1.,-1.94668377715329));
#71575=CARTESIAN_POINT('Ctrl Pts',(3.43911410197687,1.,-1.94519168842879));
#71576=CARTESIAN_POINT('Ctrl Pts',(3.43170586602434,1.,-1.94364973660284));
#71577=CARTESIAN_POINT('Ctrl Pts',(3.42430850941503,1.,-1.94205835913696));
#71578=CARTESIAN_POINT('Ctrl Pts',(3.41692971994096,1.,-1.94042111965246));
#71579=CARTESIAN_POINT('Ctrl Pts',(3.40957978266642,1.,-1.93874306008143));
#71580=CARTESIAN_POINT('Ctrl Pts',(3.40226802104109,1.,-1.93702857723098));
#71581=CARTESIAN_POINT('Ctrl Pts',(3.39499923640795,1.,-1.93527929945985));
#71582=CARTESIAN_POINT('Ctrl Pts',(3.38777076883256,1.,-1.93349233176788));
#71583=CARTESIAN_POINT('Ctrl Pts',(3.3805676852555,1.,-1.93165739093276));
#71584=CARTESIAN_POINT('Ctrl Pts',(3.37336807068043,1.,-1.92975993109877));
#71585=CARTESIAN_POINT('Ctrl Pts',(3.36615168657567,1.,-1.92778626543786));
#71586=CARTESIAN_POINT('Ctrl Pts',(3.35890824422965,1.,-1.92572846125756));
#71587=CARTESIAN_POINT('Ctrl Pts',(3.35164424847223,1.,-1.92358838440528));
#71588=CARTESIAN_POINT('Ctrl Pts',(3.34439448941961,1.,-1.92138450828404));
#71589=CARTESIAN_POINT('Ctrl Pts',(3.33721230710012,1.,-1.9191460961021));
#71590=CARTESIAN_POINT('Ctrl Pts',(3.33014884257873,1.,-1.91690081930332));
#71591=CARTESIAN_POINT('Ctrl Pts',(3.32323403454535,1.,-1.91466343916628));
#71592=CARTESIAN_POINT('Ctrl Pts',(3.31646052426364,1.,-1.91242616234442));
#71593=CARTESIAN_POINT('Ctrl Pts',(3.30975721158596,1.,-1.91014297830446));
#71594=CARTESIAN_POINT('Ctrl Pts',(3.30300595568195,1.,-1.90773912171341));
#71595=CARTESIAN_POINT('Ctrl Pts',(3.29608978722113,1.,-1.90513891864087));
#71596=CARTESIAN_POINT('Ctrl Pts',(3.2889344860029,1.,-1.90228971247527));
#71597=CARTESIAN_POINT('Ctrl Pts',(3.28154737912352,1.,-1.89918429230462));
#71598=CARTESIAN_POINT('Ctrl Pts',(3.27407108933139,1.,-1.89589172903793));
#71599=CARTESIAN_POINT('Ctrl Pts',(3.26677653888676,1.,-1.89255393500965));
#71600=CARTESIAN_POINT('Ctrl Pts',(3.25999885193947,1.,-1.88934996203698));
#71601=CARTESIAN_POINT('Ctrl Pts',(3.25408686339463,1.,-1.88646802523466));
#71602=CARTESIAN_POINT('Ctrl Pts',(3.24935200511918,1.,-1.88407708646357));
#71603=CARTESIAN_POINT('Ctrl Pts',(3.2462565441079,1.,-1.88242596600454));
#71604=CARTESIAN_POINT('Ctrl Pts',(3.24480754676064,1.,-1.88156537699203));
#71605=CARTESIAN_POINT('Ctrl Pts',(3.24428080353022,1.,-1.88117508446775));
#71606=CARTESIAN_POINT('Ctrl Pts',(3.24415531671284,1.,-1.8810229239812));
#71607=CARTESIAN_POINT('Ctrl Pts',(3.24413672884812,1.,-1.88097764062697));
#71608=CARTESIAN_POINT('',(3.70708211654725,0.,-1.97421938526992));
#71609=CARTESIAN_POINT('Ctrl Pts',(3.42855728381368,-1.,-1.519044091397));
#71610=CARTESIAN_POINT('Ctrl Pts',(3.42855728381368,1.,-1.519044091397));
#71611=CARTESIAN_POINT('Ctrl Pts',(3.42852521763778,-1.,-1.51896318668366));
#71612=CARTESIAN_POINT('Ctrl Pts',(3.42852521763778,1.,-1.51896318668366));
#71613=CARTESIAN_POINT('Ctrl Pts',(3.42860527149177,-1.,-1.51888450659652));
#71614=CARTESIAN_POINT('Ctrl Pts',(3.42860527149177,1.,-1.51888450659652));
#71615=CARTESIAN_POINT('Ctrl Pts',(3.42915787669893,-1.,-1.51901585839109));
#71616=CARTESIAN_POINT('Ctrl Pts',(3.42915787669893,1.,-1.51901585839109));
#71617=CARTESIAN_POINT('Ctrl Pts',(3.43076036253837,-1.,-1.51969006980999));
#71618=CARTESIAN_POINT('Ctrl Pts',(3.43076036253837,1.,-1.51969006980999));
#71619=CARTESIAN_POINT('Ctrl Pts',(3.43417156977893,-1.,-1.52134826724293));
#71620=CARTESIAN_POINT('Ctrl Pts',(3.43417156977893,1.,-1.52134826724293));
#71621=CARTESIAN_POINT('Ctrl Pts',(3.4388889597401,-1.,-1.5237734895035));
#71622=CARTESIAN_POINT('Ctrl Pts',(3.4388889597401,1.,-1.5237734895035));
#71623=CARTESIAN_POINT('Ctrl Pts',(3.44469547526647,-1.,-1.52686242875556));
#71624=CARTESIAN_POINT('Ctrl Pts',(3.44469547526647,1.,-1.52686242875556));
#71625=CARTESIAN_POINT('Ctrl Pts',(3.45127136828305,-1.,-1.53046244461635));
#71626=CARTESIAN_POINT('Ctrl Pts',(3.45127136828305,1.,-1.53046244461635));
#71627=CARTESIAN_POINT('Ctrl Pts',(3.45825932955032,-1.,-1.53440195378792));
#71628=CARTESIAN_POINT('Ctrl Pts',(3.45825932955032,1.,-1.53440195378792));
#71629=CARTESIAN_POINT('Ctrl Pts',(3.46531752207153,-1.,-1.53851507915502));
#71630=CARTESIAN_POINT('Ctrl Pts',(3.46531752207153,1.,-1.53851507915502));
#71631=CARTESIAN_POINT('Ctrl Pts',(3.47217189224653,-1.,-1.54266605398188));
#71632=CARTESIAN_POINT('Ctrl Pts',(3.47217189224653,1.,-1.54266605398188));
#71633=CARTESIAN_POINT('Ctrl Pts',(3.47868272898751,-1.,-1.54678009290276));
#71634=CARTESIAN_POINT('Ctrl Pts',(3.47868272898751,1.,-1.54678009290276));
#71635=CARTESIAN_POINT('Ctrl Pts',(3.48485155928567,-1.,-1.55084702970452));
#71636=CARTESIAN_POINT('Ctrl Pts',(3.48485155928567,1.,-1.55084702970452));
#71637=CARTESIAN_POINT('Ctrl Pts',(3.4907646087742,-1.,-1.55489595901116));
#71638=CARTESIAN_POINT('Ctrl Pts',(3.4907646087742,1.,-1.55489595901116));
#71639=CARTESIAN_POINT('Ctrl Pts',(3.49655185179655,-1.,-1.55897703097874));
#71640=CARTESIAN_POINT('Ctrl Pts',(3.49655185179655,1.,-1.55897703097874));
#71641=CARTESIAN_POINT('Ctrl Pts',(3.50234321621578,-1.,-1.56314187758675));
#71642=CARTESIAN_POINT('Ctrl Pts',(3.50234321621578,1.,-1.56314187758675));
#71643=CARTESIAN_POINT('Ctrl Pts',(3.50821771695363,-1.,-1.56742097575012));
#71644=CARTESIAN_POINT('Ctrl Pts',(3.50821771695363,1.,-1.56742097575012));
#71645=CARTESIAN_POINT('Ctrl Pts',(3.51418598431665,-1.,-1.57181569799743));
#71646=CARTESIAN_POINT('Ctrl Pts',(3.51418598431665,1.,-1.57181569799743));
#71647=CARTESIAN_POINT('Ctrl Pts',(3.52021847865912,-1.,-1.57631049988158));
#71648=CARTESIAN_POINT('Ctrl Pts',(3.52021847865912,1.,-1.57631049988158));
#71649=CARTESIAN_POINT('Ctrl Pts',(3.52626275334881,-1.,-1.58088027227848));
#71650=CARTESIAN_POINT('Ctrl Pts',(3.52626275334881,1.,-1.58088027227848));
#71651=CARTESIAN_POINT('Ctrl Pts',(3.5322637814708,-1.,-1.58549906268088));
#71652=CARTESIAN_POINT('Ctrl Pts',(3.5322637814708,1.,-1.58549906268088));
#71653=CARTESIAN_POINT('Ctrl Pts',(3.53818616861077,-1.,-1.59014958368739));
#71654=CARTESIAN_POINT('Ctrl Pts',(3.53818616861077,1.,-1.59014958368739));
#71655=CARTESIAN_POINT('Ctrl Pts',(3.54402458182337,-1.,-1.59482766949766));
#71656=CARTESIAN_POINT('Ctrl Pts',(3.54402458182337,1.,-1.59482766949766));
#71657=CARTESIAN_POINT('Ctrl Pts',(3.54979148634454,-1.,-1.59953698113457));
#71658=CARTESIAN_POINT('Ctrl Pts',(3.54979148634454,1.,-1.59953698113457));
#71659=CARTESIAN_POINT('Ctrl Pts',(3.55550985096129,-1.,-1.60428584699853));
#71660=CARTESIAN_POINT('Ctrl Pts',(3.55550985096129,1.,-1.60428584699853));
#71661=CARTESIAN_POINT('Ctrl Pts',(3.5612043248298,-1.,-1.60908344685457));
#71662=CARTESIAN_POINT('Ctrl Pts',(3.5612043248298,1.,-1.60908344685457));
#71663=CARTESIAN_POINT('Ctrl Pts',(3.56689200468387,-1.,-1.61393581747514));
#71664=CARTESIAN_POINT('Ctrl Pts',(3.56689200468387,1.,-1.61393581747514));
#71665=CARTESIAN_POINT('Ctrl Pts',(3.57257679609806,-1.,-1.61884340915404));
#71666=CARTESIAN_POINT('Ctrl Pts',(3.57257679609806,1.,-1.61884340915404));
#71667=CARTESIAN_POINT('Ctrl Pts',(3.5782545595439,-1.,-1.62380329464844));
#71668=CARTESIAN_POINT('Ctrl Pts',(3.5782545595439,1.,-1.62380329464844));
#71669=CARTESIAN_POINT('Ctrl Pts',(3.58391625774343,-1.,-1.62881051550745));
#71670=CARTESIAN_POINT('Ctrl Pts',(3.58391625774343,1.,-1.62881051550745));
#71671=CARTESIAN_POINT('Ctrl Pts',(3.58955176627879,-1.,-1.6338597145126));
#71672=CARTESIAN_POINT('Ctrl Pts',(3.58955176627879,1.,-1.6338597145126));
#71673=CARTESIAN_POINT('Ctrl Pts',(3.59515368334893,-1.,-1.63894676675352));
#71674=CARTESIAN_POINT('Ctrl Pts',(3.59515368334893,1.,-1.63894676675352));
#71675=CARTESIAN_POINT('Ctrl Pts',(3.60072028513845,-1.,-1.64407004385582));
#71676=CARTESIAN_POINT('Ctrl Pts',(3.60072028513845,1.,-1.64407004385582));
#71677=CARTESIAN_POINT('Ctrl Pts',(3.60625346556992,-1.,-1.64922952425832));
#71678=CARTESIAN_POINT('Ctrl Pts',(3.60625346556992,1.,-1.64922952425832));
#71679=CARTESIAN_POINT('Ctrl Pts',(3.61175734965127,-1.,-1.65442619244325));
#71680=CARTESIAN_POINT('Ctrl Pts',(3.61175734965127,1.,-1.65442619244325));
#71681=CARTESIAN_POINT('Ctrl Pts',(3.61723666482456,-1.,-1.65966133399186));
#71682=CARTESIAN_POINT('Ctrl Pts',(3.61723666482456,1.,-1.65966133399186));
#71683=CARTESIAN_POINT('Ctrl Pts',(3.62269517989109,-1.,-1.66493585923855));
#71684=CARTESIAN_POINT('Ctrl Pts',(3.62269517989109,1.,-1.66493585923855));
#71685=CARTESIAN_POINT('Ctrl Pts',(3.62813422105271,-1.,-1.67024966008045));
#71686=CARTESIAN_POINT('Ctrl Pts',(3.62813422105271,1.,-1.67024966008045));
#71687=CARTESIAN_POINT('Ctrl Pts',(3.63355343201232,-1.,-1.67560193613156));
#71688=CARTESIAN_POINT('Ctrl Pts',(3.63355343201232,1.,-1.67560193613156));
#71689=CARTESIAN_POINT('Ctrl Pts',(3.63895140887462,-1.,-1.68099146651586));
#71690=CARTESIAN_POINT('Ctrl Pts',(3.63895140887462,1.,-1.68099146651586));
#71691=CARTESIAN_POINT('Ctrl Pts',(3.64432638915203,-1.,-1.68641690471457));
#71692=CARTESIAN_POINT('Ctrl Pts',(3.64432638915203,1.,-1.68641690471457));
#71693=CARTESIAN_POINT('Ctrl Pts',(3.64967689827371,-1.,-1.69187705481689));
#71694=CARTESIAN_POINT('Ctrl Pts',(3.64967689827371,1.,-1.69187705481689));
#71695=CARTESIAN_POINT('Ctrl Pts',(3.65500246526749,-1.,-1.69737117722534));
#71696=CARTESIAN_POINT('Ctrl Pts',(3.65500246526749,1.,-1.69737117722534));
#71697=CARTESIAN_POINT('Ctrl Pts',(3.66030338774847,-1.,-1.70289888566873));
#71698=CARTESIAN_POINT('Ctrl Pts',(3.66030338774847,1.,-1.70289888566873));
#71699=CARTESIAN_POINT('Ctrl Pts',(3.66558043198876,-1.,-1.70846001610956));
#71700=CARTESIAN_POINT('Ctrl Pts',(3.66558043198876,1.,-1.70846001610956));
#71701=CARTESIAN_POINT('Ctrl Pts',(3.67083454901611,-1.,-1.71405450210384));
#71702=CARTESIAN_POINT('Ctrl Pts',(3.67083454901611,1.,-1.71405450210384));
#71703=CARTESIAN_POINT('Ctrl Pts',(3.67606660374709,-1.,-1.71968225581808));
#71704=CARTESIAN_POINT('Ctrl Pts',(3.67606660374709,1.,-1.71968225581808));
#71705=CARTESIAN_POINT('Ctrl Pts',(3.68127704936579,-1.,-1.72534302437056));
#71706=CARTESIAN_POINT('Ctrl Pts',(3.68127704936579,1.,-1.72534302437056));
#71707=CARTESIAN_POINT('Ctrl Pts',(3.68646597019332,-1.,-1.73103640956717));
#71708=CARTESIAN_POINT('Ctrl Pts',(3.68646597019332,1.,-1.73103640956717));
#71709=CARTESIAN_POINT('Ctrl Pts',(3.69163322648036,-1.,-1.73676193254557));
#71710=CARTESIAN_POINT('Ctrl Pts',(3.69163322648036,1.,-1.73676193254557));
#71711=CARTESIAN_POINT('Ctrl Pts',(3.69677856910517,-1.,-1.74251908492617));
#71712=CARTESIAN_POINT('Ctrl Pts',(3.69677856910517,1.,-1.74251908492617));
#71713=CARTESIAN_POINT('Ctrl Pts',(3.7019017567335,-1.,-1.74830738046057));
#71714=CARTESIAN_POINT('Ctrl Pts',(3.7019017567335,1.,-1.74830738046057));
#71715=CARTESIAN_POINT('Ctrl Pts',(3.70700269736659,-1.,-1.75412641804042));
#71716=CARTESIAN_POINT('Ctrl Pts',(3.70700269736659,1.,-1.75412641804042));
#71717=CARTESIAN_POINT('Ctrl Pts',(3.71208146346136,-1.,-1.75997588498865));
#71718=CARTESIAN_POINT('Ctrl Pts',(3.71208146346136,1.,-1.75997588498865));
#71719=CARTESIAN_POINT('Ctrl Pts',(3.71713822377359,-1.,-1.76585552124394));
#71720=CARTESIAN_POINT('Ctrl Pts',(3.71713822377359,1.,-1.76585552124394));
#71721=CARTESIAN_POINT('Ctrl Pts',(3.72217319911254,-1.,-1.77176509401761));
#71722=CARTESIAN_POINT('Ctrl Pts',(3.72217319911254,1.,-1.77176509401761));
#71723=CARTESIAN_POINT('Ctrl Pts',(3.72718661205609,-1.,-1.77770437039658));
#71724=CARTESIAN_POINT('Ctrl Pts',(3.72718661205609,1.,-1.77770437039658));
#71725=CARTESIAN_POINT('Ctrl Pts',(3.7321786309547,-1.,-1.78367308442901));
#71726=CARTESIAN_POINT('Ctrl Pts',(3.7321786309547,1.,-1.78367308442901));
#71727=CARTESIAN_POINT('Ctrl Pts',(3.73714934730681,-1.,-1.78967092823491));
#71728=CARTESIAN_POINT('Ctrl Pts',(3.73714934730681,1.,-1.78967092823491));
#71729=CARTESIAN_POINT('Ctrl Pts',(3.74209880352445,-1.,-1.79569757859422));
#71730=CARTESIAN_POINT('Ctrl Pts',(3.74209880352445,1.,-1.79569757859422));
#71731=CARTESIAN_POINT('Ctrl Pts',(3.74702700875467,-1.,-1.8017527148577));
#71732=CARTESIAN_POINT('Ctrl Pts',(3.74702700875467,1.,-1.8017527148577));
#71733=CARTESIAN_POINT('Ctrl Pts',(3.75193395887977,-1.,-1.80783603939617));
#71734=CARTESIAN_POINT('Ctrl Pts',(3.75193395887977,1.,-1.80783603939617));
#71735=CARTESIAN_POINT('Ctrl Pts',(3.75681965683071,-1.,-1.8139472983358));
#71736=CARTESIAN_POINT('Ctrl Pts',(3.75681965683071,1.,-1.8139472983358));
#71737=CARTESIAN_POINT('Ctrl Pts',(3.76168412707948,-1.,-1.82008629694091));
#71738=CARTESIAN_POINT('Ctrl Pts',(3.76168412707948,1.,-1.82008629694091));
#71739=CARTESIAN_POINT('Ctrl Pts',(3.76652740353775,-1.,-1.82625289220915));
#71740=CARTESIAN_POINT('Ctrl Pts',(3.76652740353775,1.,-1.82625289220915));
#71741=CARTESIAN_POINT('Ctrl Pts',(3.77038509817999,-1.,-1.83120816955646));
#71742=CARTESIAN_POINT('Ctrl Pts',(3.77038509817999,1.,-1.83120816955646));
#71743=CARTESIAN_POINT('Ctrl Pts',(3.77326886064398,-1.,-1.83493697934534));
#71744=CARTESIAN_POINT('Ctrl Pts',(3.77326886064398,1.,-1.83493697934534));
#71745=CARTESIAN_POINT('Ctrl Pts',(3.77518714457833,-1.,-1.83742834010626));
#71746=CARTESIAN_POINT('Ctrl Pts',(3.77518714457833,1.,-1.83742834010626));
#71747=CARTESIAN_POINT('Ctrl Pts',(3.77614523045147,-1.,-1.83867539237861));
#71748=CARTESIAN_POINT('Ctrl Pts',(3.77614523045147,1.,-1.83867539237861));
#71749=CARTESIAN_POINT('',(3.42859860294306,1.,-1.5189508286633));
#71750=CARTESIAN_POINT('Ctrl Pts',(3.42859860294306,-1.,-1.5189508286633));
#71751=CARTESIAN_POINT('Ctrl Pts',(3.42859860294306,-0.666666666666667,
-1.5189508286633));
#71752=CARTESIAN_POINT('Ctrl Pts',(3.42859860294306,-0.333333333333333,
-1.5189508286633));
#71753=CARTESIAN_POINT('Ctrl Pts',(3.42859860294306,0.333333333333333,-1.5189508286633));
#71754=CARTESIAN_POINT('Ctrl Pts',(3.42859860294306,0.666666666666667,-1.5189508286633));
#71755=CARTESIAN_POINT('Ctrl Pts',(3.42859860294306,1.,-1.5189508286633));
#71756=CARTESIAN_POINT('',(3.77614523045147,1.,-1.83867539237861));
#71757=CARTESIAN_POINT('',(3.77614523045147,0.,-1.83867539237861));
#71758=CARTESIAN_POINT('Ctrl Pts',(3.42859860294306,1.,-1.5189508286633));
#71759=CARTESIAN_POINT('Ctrl Pts',(3.42864616361875,1.,-1.51893924967331));
#71760=CARTESIAN_POINT('Ctrl Pts',(3.42884302333841,1.,-1.5189513329503));
#71761=CARTESIAN_POINT('Ctrl Pts',(3.42946838852588,1.,-1.51914806898491));
#71762=CARTESIAN_POINT('Ctrl Pts',(3.43101631893414,1.,-1.5198144909338));
#71763=CARTESIAN_POINT('Ctrl Pts',(3.43417156977893,1.,-1.52134826724293));
#71764=CARTESIAN_POINT('Ctrl Pts',(3.4388889597401,1.,-1.5237734895035));
#71765=CARTESIAN_POINT('Ctrl Pts',(3.44469547526647,1.,-1.52686242875556));
#71766=CARTESIAN_POINT('Ctrl Pts',(3.45127136828305,1.,-1.53046244461635));
#71767=CARTESIAN_POINT('Ctrl Pts',(3.45825932955032,1.,-1.53440195378792));
#71768=CARTESIAN_POINT('Ctrl Pts',(3.46531752207153,1.,-1.53851507915502));
#71769=CARTESIAN_POINT('Ctrl Pts',(3.47217189224653,1.,-1.54266605398188));
#71770=CARTESIAN_POINT('Ctrl Pts',(3.47868272898751,1.,-1.54678009290276));
#71771=CARTESIAN_POINT('Ctrl Pts',(3.48485155928567,1.,-1.55084702970452));
#71772=CARTESIAN_POINT('Ctrl Pts',(3.4907646087742,1.,-1.55489595901116));
#71773=CARTESIAN_POINT('Ctrl Pts',(3.49655185179655,1.,-1.55897703097874));
#71774=CARTESIAN_POINT('Ctrl Pts',(3.50234321621578,1.,-1.56314187758675));
#71775=CARTESIAN_POINT('Ctrl Pts',(3.50821771695363,1.,-1.56742097575012));
#71776=CARTESIAN_POINT('Ctrl Pts',(3.51418598431665,1.,-1.57181569799743));
#71777=CARTESIAN_POINT('Ctrl Pts',(3.52021847865912,1.,-1.57631049988158));
#71778=CARTESIAN_POINT('Ctrl Pts',(3.52626275334881,1.,-1.58088027227848));
#71779=CARTESIAN_POINT('Ctrl Pts',(3.5322637814708,1.,-1.58549906268088));
#71780=CARTESIAN_POINT('Ctrl Pts',(3.53818616861077,1.,-1.59014958368739));
#71781=CARTESIAN_POINT('Ctrl Pts',(3.54402458182337,1.,-1.59482766949766));
#71782=CARTESIAN_POINT('Ctrl Pts',(3.54979148634454,1.,-1.59953698113457));
#71783=CARTESIAN_POINT('Ctrl Pts',(3.55550985096129,1.,-1.60428584699853));
#71784=CARTESIAN_POINT('Ctrl Pts',(3.5612043248298,1.,-1.60908344685457));
#71785=CARTESIAN_POINT('Ctrl Pts',(3.56689200468387,1.,-1.61393581747514));
#71786=CARTESIAN_POINT('Ctrl Pts',(3.57257679609806,1.,-1.61884340915404));
#71787=CARTESIAN_POINT('Ctrl Pts',(3.5782545595439,1.,-1.62380329464844));
#71788=CARTESIAN_POINT('Ctrl Pts',(3.58391625774343,1.,-1.62881051550745));
#71789=CARTESIAN_POINT('Ctrl Pts',(3.58955176627879,1.,-1.6338597145126));
#71790=CARTESIAN_POINT('Ctrl Pts',(3.59515368334893,1.,-1.63894676675352));
#71791=CARTESIAN_POINT('Ctrl Pts',(3.60072028513845,1.,-1.64407004385582));
#71792=CARTESIAN_POINT('Ctrl Pts',(3.60625346556992,1.,-1.64922952425832));
#71793=CARTESIAN_POINT('Ctrl Pts',(3.61175734965127,1.,-1.65442619244325));
#71794=CARTESIAN_POINT('Ctrl Pts',(3.61723666482456,1.,-1.65966133399186));
#71795=CARTESIAN_POINT('Ctrl Pts',(3.62269517989109,1.,-1.66493585923855));
#71796=CARTESIAN_POINT('Ctrl Pts',(3.62813422105271,1.,-1.67024966008045));
#71797=CARTESIAN_POINT('Ctrl Pts',(3.63355343201232,1.,-1.67560193613156));
#71798=CARTESIAN_POINT('Ctrl Pts',(3.63895140887462,1.,-1.68099146651586));
#71799=CARTESIAN_POINT('Ctrl Pts',(3.64432638915203,1.,-1.68641690471457));
#71800=CARTESIAN_POINT('Ctrl Pts',(3.64967689827371,1.,-1.69187705481689));
#71801=CARTESIAN_POINT('Ctrl Pts',(3.65500246526749,1.,-1.69737117722534));
#71802=CARTESIAN_POINT('Ctrl Pts',(3.66030338774847,1.,-1.70289888566873));
#71803=CARTESIAN_POINT('Ctrl Pts',(3.66558043198876,1.,-1.70846001610956));
#71804=CARTESIAN_POINT('Ctrl Pts',(3.67083454901611,1.,-1.71405450210384));
#71805=CARTESIAN_POINT('Ctrl Pts',(3.67606660374709,1.,-1.71968225581808));
#71806=CARTESIAN_POINT('Ctrl Pts',(3.68127704936579,1.,-1.72534302437056));
#71807=CARTESIAN_POINT('Ctrl Pts',(3.68646597019332,1.,-1.73103640956717));
#71808=CARTESIAN_POINT('Ctrl Pts',(3.69163322648036,1.,-1.73676193254557));
#71809=CARTESIAN_POINT('Ctrl Pts',(3.69677856910517,1.,-1.74251908492617));
#71810=CARTESIAN_POINT('Ctrl Pts',(3.7019017567335,1.,-1.74830738046057));
#71811=CARTESIAN_POINT('Ctrl Pts',(3.70700269736659,1.,-1.75412641804042));
#71812=CARTESIAN_POINT('Ctrl Pts',(3.71208146346136,1.,-1.75997588498865));
#71813=CARTESIAN_POINT('Ctrl Pts',(3.71713822377359,1.,-1.76585552124394));
#71814=CARTESIAN_POINT('Ctrl Pts',(3.72217319911254,1.,-1.77176509401761));
#71815=CARTESIAN_POINT('Ctrl Pts',(3.72718661205609,1.,-1.77770437039658));
#71816=CARTESIAN_POINT('Ctrl Pts',(3.7321786309547,1.,-1.78367308442901));
#71817=CARTESIAN_POINT('Ctrl Pts',(3.73714934730681,1.,-1.78967092823491));
#71818=CARTESIAN_POINT('Ctrl Pts',(3.74209880352445,1.,-1.79569757859422));
#71819=CARTESIAN_POINT('Ctrl Pts',(3.74702700875467,1.,-1.8017527148577));
#71820=CARTESIAN_POINT('Ctrl Pts',(3.75193395887977,1.,-1.80783603939617));
#71821=CARTESIAN_POINT('Ctrl Pts',(3.75681965683071,1.,-1.8139472983358));
#71822=CARTESIAN_POINT('Ctrl Pts',(3.76168412707948,1.,-1.82008629694091));
#71823=CARTESIAN_POINT('Ctrl Pts',(3.76652740353775,1.,-1.82625289220915));
#71824=CARTESIAN_POINT('Ctrl Pts',(3.77038509817999,1.,-1.83120816955646));
#71825=CARTESIAN_POINT('Ctrl Pts',(3.77326886064398,1.,-1.83493697934534));
#71826=CARTESIAN_POINT('Ctrl Pts',(3.77518714457833,1.,-1.83742834010626));
#71827=CARTESIAN_POINT('Ctrl Pts',(3.77614523045147,1.,-1.83867539237861));
#71828=CARTESIAN_POINT('Origin',(3.77614523045147,0.,-1.83867539237861));
#71829=CARTESIAN_POINT('',(3.70708211654725,1.,-1.97421938526992));
#71830=CARTESIAN_POINT('Origin',(0.,0.,0.));
#71831=CARTESIAN_POINT('',(3.49844575334386,1.,-1.35032489087269));
#71832=CARTESIAN_POINT('Origin',(0.,1.,0.));
#71833=CARTESIAN_POINT('Ctrl Pts',(3.49844575334386,1.,-1.35032489087269));
#71834=CARTESIAN_POINT('Ctrl Pts',(3.49844575334386,0.666666666666667,-1.35032489087269));
#71835=CARTESIAN_POINT('Ctrl Pts',(3.49844575334386,0.333333333333333,-1.35032489087269));
#71836=CARTESIAN_POINT('Ctrl Pts',(3.49844575334386,-0.333333333333333,
-1.35032489087269));
#71837=CARTESIAN_POINT('Ctrl Pts',(3.49844575334386,-0.666666666666667,
-1.35032489087269));
#71838=CARTESIAN_POINT('Ctrl Pts',(3.49844575334386,-1.,-1.35032489087269));
#71839=CARTESIAN_POINT('Ctrl Pts',(3.97027773754922,-1.,-1.36999806084572));
#71840=CARTESIAN_POINT('Ctrl Pts',(3.97027773754922,1.,-1.36999806084572));
#71841=CARTESIAN_POINT('Ctrl Pts',(3.9687184694173,-1.,-1.37020239094758));
#71842=CARTESIAN_POINT('Ctrl Pts',(3.9687184694173,1.,-1.37020239094758));
#71843=CARTESIAN_POINT('Ctrl Pts',(3.96560037975788,-1.,-1.37060761746027));
#71844=CARTESIAN_POINT('Ctrl Pts',(3.96560037975788,1.,-1.37060761746027));
#71845=CARTESIAN_POINT('Ctrl Pts',(3.96092458508407,-1.,-1.37120515615663));
#71846=CARTESIAN_POINT('Ctrl Pts',(3.96092458508407,1.,-1.37120515615663));
#71847=CARTESIAN_POINT('Ctrl Pts',(3.95469287283105,-1.,-1.37198126433139));
#71848=CARTESIAN_POINT('Ctrl Pts',(3.95469287283105,1.,-1.37198126433139));
#71849=CARTESIAN_POINT('Ctrl Pts',(3.94690771786926,-1.,-1.37291699203423));
#71850=CARTESIAN_POINT('Ctrl Pts',(3.94690771786926,1.,-1.37291699203423));
#71851=CARTESIAN_POINT('Ctrl Pts',(3.93912709041791,-1.,-1.37381821967499));
#71852=CARTESIAN_POINT('Ctrl Pts',(3.93912709041791,1.,-1.37381821967499));
#71853=CARTESIAN_POINT('Ctrl Pts',(3.93135106761941,-1.,-1.37468482215784));
#71854=CARTESIAN_POINT('Ctrl Pts',(3.93135106761941,1.,-1.37468482215784));
#71855=CARTESIAN_POINT('Ctrl Pts',(3.92357976987132,-1.,-1.37551664448057));
#71856=CARTESIAN_POINT('Ctrl Pts',(3.92357976987132,1.,-1.37551664448057));
#71857=CARTESIAN_POINT('Ctrl Pts',(3.91581337461825,-1.,-1.37631350505516));
#71858=CARTESIAN_POINT('Ctrl Pts',(3.91581337461825,1.,-1.37631350505516));
#71859=CARTESIAN_POINT('Ctrl Pts',(3.90805209522729,-1.,-1.3770751963376));
#71860=CARTESIAN_POINT('Ctrl Pts',(3.90805209522729,1.,-1.3770751963376));
#71861=CARTESIAN_POINT('Ctrl Pts',(3.90029615196255,-1.,-1.3778014851263));
#71862=CARTESIAN_POINT('Ctrl Pts',(3.90029615196255,1.,-1.3778014851263));
#71863=CARTESIAN_POINT('Ctrl Pts',(3.89254574338385,-1.,-1.37849211287981));
#71864=CARTESIAN_POINT('Ctrl Pts',(3.89254574338385,1.,-1.37849211287981));
#71865=CARTESIAN_POINT('Ctrl Pts',(3.88480102249461,-1.,-1.37914679719446));
#71866=CARTESIAN_POINT('Ctrl Pts',(3.88480102249461,1.,-1.37914679719446));
#71867=CARTESIAN_POINT('Ctrl Pts',(3.87706205830865,-1.,-1.37976523097187));
#71868=CARTESIAN_POINT('Ctrl Pts',(3.87706205830865,1.,-1.37976523097187));
#71869=CARTESIAN_POINT('Ctrl Pts',(3.86932885813403,-1.,-1.38034709213129));
#71870=CARTESIAN_POINT('Ctrl Pts',(3.86932885813403,1.,-1.38034709213129));
#71871=CARTESIAN_POINT('Ctrl Pts',(3.86160143044187,-1.,-1.38089205993068));
#71872=CARTESIAN_POINT('Ctrl Pts',(3.86160143044187,1.,-1.38089205993068));
#71873=CARTESIAN_POINT('Ctrl Pts',(3.85387983979557,-1.,-1.38139983115075));
#71874=CARTESIAN_POINT('Ctrl Pts',(3.85387983979557,1.,-1.38139983115075));
#71875=CARTESIAN_POINT('Ctrl Pts',(3.84616425605705,-1.,-1.38187013346089));
#71876=CARTESIAN_POINT('Ctrl Pts',(3.84616425605705,1.,-1.38187013346089));
#71877=CARTESIAN_POINT('Ctrl Pts',(3.83845502790609,-1.,-1.38230274828774));
#71878=CARTESIAN_POINT('Ctrl Pts',(3.83845502790609,1.,-1.38230274828774));
#71879=CARTESIAN_POINT('Ctrl Pts',(3.83075266982138,-1.,-1.38269750245086));
#71880=CARTESIAN_POINT('Ctrl Pts',(3.83075266982138,1.,-1.38269750245086));
#71881=CARTESIAN_POINT('Ctrl Pts',(3.82305771743715,-1.,-1.38305421262724));
#71882=CARTESIAN_POINT('Ctrl Pts',(3.82305771743715,1.,-1.38305421262724));
#71883=CARTESIAN_POINT('Ctrl Pts',(3.81537060817765,-1.,-1.38337263902766));
#71884=CARTESIAN_POINT('Ctrl Pts',(3.81537060817765,1.,-1.38337263902766));
#71885=CARTESIAN_POINT('Ctrl Pts',(3.80769156398429,-1.,-1.38365244046226));
#71886=CARTESIAN_POINT('Ctrl Pts',(3.80769156398429,1.,-1.38365244046226));
#71887=CARTESIAN_POINT('Ctrl Pts',(3.80002044322169,-1.,-1.38389311766701));
#71888=CARTESIAN_POINT('Ctrl Pts',(3.80002044322169,1.,-1.38389311766701));
#71889=CARTESIAN_POINT('Ctrl Pts',(3.79235669640907,-1.,-1.38409399694589));
#71890=CARTESIAN_POINT('Ctrl Pts',(3.79235669640907,1.,-1.38409399694589));
#71891=CARTESIAN_POINT('Ctrl Pts',(3.78469969805134,-1.,-1.38425435883773));
#71892=CARTESIAN_POINT('Ctrl Pts',(3.78469969805134,1.,-1.38425435883773));
#71893=CARTESIAN_POINT('Ctrl Pts',(3.77704902230441,-1.,-1.38437354551435));
#71894=CARTESIAN_POINT('Ctrl Pts',(3.77704902230441,1.,-1.38437354551435));
#71895=CARTESIAN_POINT('Ctrl Pts',(3.76940473185775,-1.,-1.38445107339517));
#71896=CARTESIAN_POINT('Ctrl Pts',(3.76940473185775,1.,-1.38445107339517));
#71897=CARTESIAN_POINT('Ctrl Pts',(3.76176768271347,-1.,-1.38448675253343));
#71898=CARTESIAN_POINT('Ctrl Pts',(3.76176768271347,1.,-1.38448675253343));
#71899=CARTESIAN_POINT('Ctrl Pts',(3.75413976318727,-1.,-1.38448077997155));
#71900=CARTESIAN_POINT('Ctrl Pts',(3.75413976318727,1.,-1.38448077997155));
#71901=CARTESIAN_POINT('Ctrl Pts',(3.7465231716786,-1.,-1.38443344984389));
#71902=CARTESIAN_POINT('Ctrl Pts',(3.7465231716786,1.,-1.38443344984389));
#71903=CARTESIAN_POINT('Ctrl Pts',(3.73891976418099,-1.,-1.38434489156456));
#71904=CARTESIAN_POINT('Ctrl Pts',(3.73891976418099,1.,-1.38434489156456));
#71905=CARTESIAN_POINT('Ctrl Pts',(3.73133035859283,-1.,-1.38421479111531));
#71906=CARTESIAN_POINT('Ctrl Pts',(3.73133035859283,1.,-1.38421479111531));
#71907=CARTESIAN_POINT('Ctrl Pts',(3.72375409358805,-1.,-1.3840421342895));
#71908=CARTESIAN_POINT('Ctrl Pts',(3.72375409358805,1.,-1.3840421342895));
#71909=CARTESIAN_POINT('Ctrl Pts',(3.7161876605181,-1.,-1.38382489984585));
#71910=CARTESIAN_POINT('Ctrl Pts',(3.7161876605181,1.,-1.38382489984585));
#71911=CARTESIAN_POINT('Ctrl Pts',(3.70862680753343,-1.,-1.38356065402122));
#71912=CARTESIAN_POINT('Ctrl Pts',(3.70862680753343,1.,-1.38356065402122));
#71913=CARTESIAN_POINT('Ctrl Pts',(3.70106792167894,-1.,-1.38324717612862));
#71914=CARTESIAN_POINT('Ctrl Pts',(3.70106792167894,1.,-1.38324717612862));
#71915=CARTESIAN_POINT('Ctrl Pts',(3.69350967899523,-1.,-1.38288311171649));
#71916=CARTESIAN_POINT('Ctrl Pts',(3.69350967899523,1.,-1.38288311171649));
#71917=CARTESIAN_POINT('Ctrl Pts',(3.68595444983844,-1.,-1.38246852827185));
#71918=CARTESIAN_POINT('Ctrl Pts',(3.68595444983844,1.,-1.38246852827185));
#71919=CARTESIAN_POINT('Ctrl Pts',(3.6784103848243,-1.,-1.38200574290626));
#71920=CARTESIAN_POINT('Ctrl Pts',(3.6784103848243,1.,-1.38200574290626));
#71921=CARTESIAN_POINT('Ctrl Pts',(3.67088843112282,-1.,-1.38149812653876));
#71922=CARTESIAN_POINT('Ctrl Pts',(3.67088843112282,1.,-1.38149812653876));
#71923=CARTESIAN_POINT('Ctrl Pts',(3.66339848520874,-1.,-1.38094856333558));
#71924=CARTESIAN_POINT('Ctrl Pts',(3.66339848520874,1.,-1.38094856333558));
#71925=CARTESIAN_POINT('Ctrl Pts',(3.65594554404396,-1.,-1.38035791051215));
#71926=CARTESIAN_POINT('Ctrl Pts',(3.65594554404396,1.,-1.38035791051215));
#71927=CARTESIAN_POINT('Ctrl Pts',(3.64852652756444,-1.,-1.37972372481598));
#71928=CARTESIAN_POINT('Ctrl Pts',(3.64852652756444,1.,-1.37972372481598));
#71929=CARTESIAN_POINT('Ctrl Pts',(3.64112507791112,-1.,-1.37903818567347));
#71930=CARTESIAN_POINT('Ctrl Pts',(3.64112507791112,1.,-1.37903818567347));
#71931=CARTESIAN_POINT('Ctrl Pts',(3.63371727442448,-1.,-1.37829035457325));
#71932=CARTESIAN_POINT('Ctrl Pts',(3.63371727442448,1.,-1.37829035457325));
#71933=CARTESIAN_POINT('Ctrl Pts',(3.62628098665112,-1.,-1.37746987919868));
#71934=CARTESIAN_POINT('Ctrl Pts',(3.62628098665112,1.,-1.37746987919868));
#71935=CARTESIAN_POINT('Ctrl Pts',(3.61880481160408,-1.,-1.37657053403102));
#71936=CARTESIAN_POINT('Ctrl Pts',(3.61880481160408,1.,-1.37657053403102));
#71937=CARTESIAN_POINT('Ctrl Pts',(3.61129546591082,-1.,-1.37559314436641));
#71938=CARTESIAN_POINT('Ctrl Pts',(3.61129546591082,1.,-1.37559314436641));
#71939=CARTESIAN_POINT('Ctrl Pts',(3.60379020124038,-1.,-1.37455051379642));
#71940=CARTESIAN_POINT('Ctrl Pts',(3.60379020124038,1.,-1.37455051379642));
#71941=CARTESIAN_POINT('Ctrl Pts',(3.59634627869117,-1.,-1.37346320103184));
#71942=CARTESIAN_POINT('Ctrl Pts',(3.59634627869117,1.,-1.37346320103184));
#71943=CARTESIAN_POINT('Ctrl Pts',(3.5890185384643,-1.,-1.37235053661));
#71944=CARTESIAN_POINT('Ctrl Pts',(3.5890185384643,1.,-1.37235053661));
#71945=CARTESIAN_POINT('Ctrl Pts',(3.58183885982745,-1.,-1.37122241663073));
#71946=CARTESIAN_POINT('Ctrl Pts',(3.58183885982745,1.,-1.37122241663073));
#71947=CARTESIAN_POINT('Ctrl Pts',(3.57479875549453,-1.,-1.37007229485646));
#71948=CARTESIAN_POINT('Ctrl Pts',(3.57479875549453,1.,-1.37007229485646));
#71949=CARTESIAN_POINT('Ctrl Pts',(3.56782080304554,-1.,-1.36886584973349));
#71950=CARTESIAN_POINT('Ctrl Pts',(3.56782080304554,1.,-1.36886584973349));
#71951=CARTESIAN_POINT('Ctrl Pts',(3.56077662028492,-1.,-1.36754771771174));
#71952=CARTESIAN_POINT('Ctrl Pts',(3.56077662028492,1.,-1.36754771771174));
#71953=CARTESIAN_POINT('Ctrl Pts',(3.55353883995793,-1.,-1.36606145456711));
#71954=CARTESIAN_POINT('Ctrl Pts',(3.55353883995793,1.,-1.36606145456711));
#71955=CARTESIAN_POINT('Ctrl Pts',(3.54602591832893,-1.,-1.36436666257568));
#71956=CARTESIAN_POINT('Ctrl Pts',(3.54602591832893,1.,-1.36436666257568));
#71957=CARTESIAN_POINT('Ctrl Pts',(3.53824396425032,-1.,-1.36245507339334));
#71958=CARTESIAN_POINT('Ctrl Pts',(3.53824396425032,1.,-1.36245507339334));
#71959=CARTESIAN_POINT('Ctrl Pts',(3.53034464961849,-1.,-1.36037259643827));
#71960=CARTESIAN_POINT('Ctrl Pts',(3.53034464961849,1.,-1.36037259643827));
#71961=CARTESIAN_POINT('Ctrl Pts',(3.52261776117121,-1.,-1.35821701528975));
#71962=CARTESIAN_POINT('Ctrl Pts',(3.52261776117121,1.,-1.35821701528975));
#71963=CARTESIAN_POINT('Ctrl Pts',(3.51542230699919,-1.,-1.35611275237288));
#71964=CARTESIAN_POINT('Ctrl Pts',(3.51542230699919,1.,-1.35611275237288));
#71965=CARTESIAN_POINT('Ctrl Pts',(3.50913227060177,-1.,-1.35419113576022));
#71966=CARTESIAN_POINT('Ctrl Pts',(3.50913227060177,1.,-1.35419113576022));
#71967=CARTESIAN_POINT('Ctrl Pts',(3.50408168106113,-1.,-1.3525703284343));
#71968=CARTESIAN_POINT('Ctrl Pts',(3.50408168106113,1.,-1.3525703284343));
#71969=CARTESIAN_POINT('Ctrl Pts',(3.50049707063673,-1.,-1.35133076331065));
#71970=CARTESIAN_POINT('Ctrl Pts',(3.50049707063673,1.,-1.35133076331065));
#71971=CARTESIAN_POINT('Ctrl Pts',(3.49888720256612,-1.,-1.35067437417289));
#71972=CARTESIAN_POINT('Ctrl Pts',(3.49888720256612,1.,-1.35067437417289));
#71973=CARTESIAN_POINT('Ctrl Pts',(3.49840357193384,-1.,-1.35037650302887));
#71974=CARTESIAN_POINT('Ctrl Pts',(3.49840357193384,1.,-1.35037650302887));
#71975=CARTESIAN_POINT('Ctrl Pts',(3.49840260053616,-1.,-1.35026426118352));
#71976=CARTESIAN_POINT('Ctrl Pts',(3.49840260053616,1.,-1.35026426118352));
#71977=CARTESIAN_POINT('Ctrl Pts',(3.49848248301936,-1.,-1.35022972712301));
#71978=CARTESIAN_POINT('Ctrl Pts',(3.49848248301936,1.,-1.35022972712301));
#71979=CARTESIAN_POINT('',(3.97027773754922,1.,-1.36999806084572));
#71980=CARTESIAN_POINT('Ctrl Pts',(3.97027773754922,1.,-1.36999806084572));
#71981=CARTESIAN_POINT('Ctrl Pts',(3.9687184694173,1.,-1.37020239094758));
#71982=CARTESIAN_POINT('Ctrl Pts',(3.96560037975788,1.,-1.37060761746027));
#71983=CARTESIAN_POINT('Ctrl Pts',(3.96092458508407,1.,-1.37120515615663));
#71984=CARTESIAN_POINT('Ctrl Pts',(3.95469287283105,1.,-1.37198126433139));
#71985=CARTESIAN_POINT('Ctrl Pts',(3.94690771786926,1.,-1.37291699203423));
#71986=CARTESIAN_POINT('Ctrl Pts',(3.93912709041791,1.,-1.37381821967499));
#71987=CARTESIAN_POINT('Ctrl Pts',(3.93135106761941,1.,-1.37468482215784));
#71988=CARTESIAN_POINT('Ctrl Pts',(3.92357976987132,1.,-1.37551664448057));
#71989=CARTESIAN_POINT('Ctrl Pts',(3.91581337461825,1.,-1.37631350505516));
#71990=CARTESIAN_POINT('Ctrl Pts',(3.90805209522729,1.,-1.3770751963376));
#71991=CARTESIAN_POINT('Ctrl Pts',(3.90029615196255,1.,-1.3778014851263));
#71992=CARTESIAN_POINT('Ctrl Pts',(3.89254574338385,1.,-1.37849211287981));
#71993=CARTESIAN_POINT('Ctrl Pts',(3.88480102249461,1.,-1.37914679719446));
#71994=CARTESIAN_POINT('Ctrl Pts',(3.87706205830865,1.,-1.37976523097187));
#71995=CARTESIAN_POINT('Ctrl Pts',(3.86932885813403,1.,-1.38034709213129));
#71996=CARTESIAN_POINT('Ctrl Pts',(3.86160143044187,1.,-1.38089205993068));
#71997=CARTESIAN_POINT('Ctrl Pts',(3.85387983979557,1.,-1.38139983115075));
#71998=CARTESIAN_POINT('Ctrl Pts',(3.84616425605705,1.,-1.38187013346089));
#71999=CARTESIAN_POINT('Ctrl Pts',(3.83845502790609,1.,-1.38230274828774));
#72000=CARTESIAN_POINT('Ctrl Pts',(3.83075266982138,1.,-1.38269750245086));
#72001=CARTESIAN_POINT('Ctrl Pts',(3.82305771743715,1.,-1.38305421262724));
#72002=CARTESIAN_POINT('Ctrl Pts',(3.81537060817765,1.,-1.38337263902766));
#72003=CARTESIAN_POINT('Ctrl Pts',(3.80769156398429,1.,-1.38365244046226));
#72004=CARTESIAN_POINT('Ctrl Pts',(3.80002044322169,1.,-1.38389311766701));
#72005=CARTESIAN_POINT('Ctrl Pts',(3.79235669640907,1.,-1.38409399694589));
#72006=CARTESIAN_POINT('Ctrl Pts',(3.78469969805134,1.,-1.38425435883773));
#72007=CARTESIAN_POINT('Ctrl Pts',(3.77704902230441,1.,-1.38437354551435));
#72008=CARTESIAN_POINT('Ctrl Pts',(3.76940473185775,1.,-1.38445107339517));
#72009=CARTESIAN_POINT('Ctrl Pts',(3.76176768271347,1.,-1.38448675253343));
#72010=CARTESIAN_POINT('Ctrl Pts',(3.75413976318727,1.,-1.38448077997155));
#72011=CARTESIAN_POINT('Ctrl Pts',(3.7465231716786,1.,-1.38443344984389));
#72012=CARTESIAN_POINT('Ctrl Pts',(3.73891976418099,1.,-1.38434489156456));
#72013=CARTESIAN_POINT('Ctrl Pts',(3.73133035859283,1.,-1.38421479111531));
#72014=CARTESIAN_POINT('Ctrl Pts',(3.72375409358805,1.,-1.3840421342895));
#72015=CARTESIAN_POINT('Ctrl Pts',(3.7161876605181,1.,-1.38382489984585));
#72016=CARTESIAN_POINT('Ctrl Pts',(3.70862680753343,1.,-1.38356065402122));
#72017=CARTESIAN_POINT('Ctrl Pts',(3.70106792167894,1.,-1.38324717612862));
#72018=CARTESIAN_POINT('Ctrl Pts',(3.69350967899523,1.,-1.38288311171649));
#72019=CARTESIAN_POINT('Ctrl Pts',(3.68595444983844,1.,-1.38246852827185));
#72020=CARTESIAN_POINT('Ctrl Pts',(3.6784103848243,1.,-1.38200574290626));
#72021=CARTESIAN_POINT('Ctrl Pts',(3.67088843112282,1.,-1.38149812653876));
#72022=CARTESIAN_POINT('Ctrl Pts',(3.66339848520874,1.,-1.38094856333558));
#72023=CARTESIAN_POINT('Ctrl Pts',(3.65594554404396,1.,-1.38035791051215));
#72024=CARTESIAN_POINT('Ctrl Pts',(3.64852652756444,1.,-1.37972372481598));
#72025=CARTESIAN_POINT('Ctrl Pts',(3.64112507791112,1.,-1.37903818567347));
#72026=CARTESIAN_POINT('Ctrl Pts',(3.63371727442448,1.,-1.37829035457325));
#72027=CARTESIAN_POINT('Ctrl Pts',(3.62628098665112,1.,-1.37746987919868));
#72028=CARTESIAN_POINT('Ctrl Pts',(3.61880481160408,1.,-1.37657053403102));
#72029=CARTESIAN_POINT('Ctrl Pts',(3.61129546591082,1.,-1.37559314436641));
#72030=CARTESIAN_POINT('Ctrl Pts',(3.60379020124038,1.,-1.37455051379642));
#72031=CARTESIAN_POINT('Ctrl Pts',(3.59634627869117,1.,-1.37346320103184));
#72032=CARTESIAN_POINT('Ctrl Pts',(3.5890185384643,1.,-1.37235053661));
#72033=CARTESIAN_POINT('Ctrl Pts',(3.58183885982745,1.,-1.37122241663073));
#72034=CARTESIAN_POINT('Ctrl Pts',(3.57479875549453,1.,-1.37007229485646));
#72035=CARTESIAN_POINT('Ctrl Pts',(3.56782080304554,1.,-1.36886584973349));
#72036=CARTESIAN_POINT('Ctrl Pts',(3.56077662028492,1.,-1.36754771771174));
#72037=CARTESIAN_POINT('Ctrl Pts',(3.55353883995793,1.,-1.36606145456711));
#72038=CARTESIAN_POINT('Ctrl Pts',(3.54602591832893,1.,-1.36436666257568));
#72039=CARTESIAN_POINT('Ctrl Pts',(3.53824396425032,1.,-1.36245507339334));
#72040=CARTESIAN_POINT('Ctrl Pts',(3.53034464961849,1.,-1.36037259643827));
#72041=CARTESIAN_POINT('Ctrl Pts',(3.52261776117121,1.,-1.35821701528975));
#72042=CARTESIAN_POINT('Ctrl Pts',(3.51542230699919,1.,-1.35611275237288));
#72043=CARTESIAN_POINT('Ctrl Pts',(3.50913227060177,1.,-1.35419113576022));
#72044=CARTESIAN_POINT('Ctrl Pts',(3.50408168106113,1.,-1.3525703284343));
#72045=CARTESIAN_POINT('Ctrl Pts',(3.5007660381658,1.,-1.35142377279535));
#72046=CARTESIAN_POINT('Ctrl Pts',(3.49920025459856,1.,-1.35080045218652));
#72047=CARTESIAN_POINT('Ctrl Pts',(3.49861894124915,1.,-1.35049736560633));
#72048=CARTESIAN_POINT('Ctrl Pts',(3.49847119623841,1.,-1.35036670893102));
#72049=CARTESIAN_POINT('Ctrl Pts',(3.49844575334386,1.,-1.35032489087269));
#72050=CARTESIAN_POINT('',(3.97027773754922,0.,-1.36999806084572));
#72051=CARTESIAN_POINT('Ctrl Pts',(3.62397690409552,-1.,-0.963997613369571));
#72052=CARTESIAN_POINT('Ctrl Pts',(3.62397690409552,1.,-0.963997613369571));
#72053=CARTESIAN_POINT('Ctrl Pts',(3.62393257642191,-1.,-0.963922720982576));
#72054=CARTESIAN_POINT('Ctrl Pts',(3.62393257642191,1.,-0.963922720982576));
#72055=CARTESIAN_POINT('Ctrl Pts',(3.62399933640277,-1.,-0.963832486396056));
#72056=CARTESIAN_POINT('Ctrl Pts',(3.62399933640277,1.,-0.963832486396056));
#72057=CARTESIAN_POINT('Ctrl Pts',(3.62456568607055,-1.,-0.963875774532103));
#72058=CARTESIAN_POINT('Ctrl Pts',(3.62456568607055,1.,-0.963875774532103));
#72059=CARTESIAN_POINT('Ctrl Pts',(3.62625391255277,-1.,-0.964291001274619));
#72060=CARTESIAN_POINT('Ctrl Pts',(3.62625391255277,1.,-0.964291001274619));
#72061=CARTESIAN_POINT('Ctrl Pts',(3.62988252139998,-1.,-0.965395153165716));
#72062=CARTESIAN_POINT('Ctrl Pts',(3.62988252139998,1.,-0.965395153165716));
#72063=CARTESIAN_POINT('Ctrl Pts',(3.6349212208096,-1.,-0.967052554540878));
#72064=CARTESIAN_POINT('Ctrl Pts',(3.6349212208096,1.,-0.967052554540878));
#72065=CARTESIAN_POINT('Ctrl Pts',(3.64113946505393,-1.,-0.969195124674829));
#72066=CARTESIAN_POINT('Ctrl Pts',(3.64113946505393,1.,-0.969195124674829));
#72067=CARTESIAN_POINT('Ctrl Pts',(3.64819756447072,-1.,-0.971722122060278));
#72068=CARTESIAN_POINT('Ctrl Pts',(3.64819756447072,1.,-0.971722122060278));
#72069=CARTESIAN_POINT('Ctrl Pts',(3.6557157673487,-1.,-0.974519971354139));
#72070=CARTESIAN_POINT('Ctrl Pts',(3.6557157673487,1.,-0.974519971354139));
#72071=CARTESIAN_POINT('Ctrl Pts',(3.66333049637403,-1.,-0.977478312751416));
#72072=CARTESIAN_POINT('Ctrl Pts',(3.66333049637403,1.,-0.977478312751416));
#72073=CARTESIAN_POINT('Ctrl Pts',(3.67074983340444,-1.,-0.980505922458495));
#72074=CARTESIAN_POINT('Ctrl Pts',(3.67074983340444,1.,-0.980505922458495));
#72075=CARTESIAN_POINT('Ctrl Pts',(3.67782408841876,-1.,-0.983550791470865));
#72076=CARTESIAN_POINT('Ctrl Pts',(3.67782408841876,1.,-0.983550791470865));
#72077=CARTESIAN_POINT('Ctrl Pts',(3.6845531792623,-1.,-0.986602639864286));
#72078=CARTESIAN_POINT('Ctrl Pts',(3.6845531792623,1.,-0.986602639864286));
#72079=CARTESIAN_POINT('Ctrl Pts',(3.69102682138955,-1.,-0.989676715398859));
#72080=CARTESIAN_POINT('Ctrl Pts',(3.69102682138955,1.,-0.989676715398859));
#72081=CARTESIAN_POINT('Ctrl Pts',(3.69738123415696,-1.,-0.992802218332104));
#72082=CARTESIAN_POINT('Ctrl Pts',(3.69738123415696,1.,-0.992802218332104));
#72083=CARTESIAN_POINT('Ctrl Pts',(3.70375282282107,-1.,-0.996009819772432));
#72084=CARTESIAN_POINT('Ctrl Pts',(3.70375282282107,1.,-0.996009819772432));
#72085=CARTESIAN_POINT('Ctrl Pts',(3.7102243971387,-1.,-0.999317260756345));
#72086=CARTESIAN_POINT('Ctrl Pts',(3.7102243971387,1.,-0.999317260756345));
#72087=CARTESIAN_POINT('Ctrl Pts',(3.71680667125047,-1.,-1.00272423396802));
#72088=CARTESIAN_POINT('Ctrl Pts',(3.71680667125047,1.,-1.00272423396802));
#72089=CARTESIAN_POINT('Ctrl Pts',(3.72346803750544,-1.,-1.00622000735696));
#72090=CARTESIAN_POINT('Ctrl Pts',(3.72346803750544,1.,-1.00622000735696));
#72091=CARTESIAN_POINT('Ctrl Pts',(3.73015276704407,-1.,-1.00978798539491));
#72092=CARTESIAN_POINT('Ctrl Pts',(3.73015276704407,1.,-1.00978798539491));
#72093=CARTESIAN_POINT('Ctrl Pts',(3.73680245055747,-1.,-1.01341114319906));
#72094=CARTESIAN_POINT('Ctrl Pts',(3.73680245055747,1.,-1.01341114319906));
#72095=CARTESIAN_POINT('Ctrl Pts',(3.74337942504993,-1.,-1.01707794311088));
#72096=CARTESIAN_POINT('Ctrl Pts',(3.74337942504993,1.,-1.01707794311088));
#72097=CARTESIAN_POINT('Ctrl Pts',(3.74987777155873,-1.,-1.02078510487439));
#72098=CARTESIAN_POINT('Ctrl Pts',(3.74987777155873,1.,-1.02078510487439));
#72099=CARTESIAN_POINT('Ctrl Pts',(3.75631037456224,-1.,-1.02453429444668));
#72100=CARTESIAN_POINT('Ctrl Pts',(3.75631037456224,1.,-1.02453429444668));
#72101=CARTESIAN_POINT('Ctrl Pts',(3.76270122291245,-1.,-1.02833014458184));
#72102=CARTESIAN_POINT('Ctrl Pts',(3.76270122291245,1.,-1.02833014458184));
#72103=CARTESIAN_POINT('Ctrl Pts',(3.76907609832516,-1.,-1.03217786604919));
#72104=CARTESIAN_POINT('Ctrl Pts',(3.76907609832516,1.,-1.03217786604919));
#72105=CARTESIAN_POINT('Ctrl Pts',(3.77545283140427,-1.,-1.03608074678008));
#72106=CARTESIAN_POINT('Ctrl Pts',(3.77545283140427,1.,-1.03608074678008));
#72107=CARTESIAN_POINT('Ctrl Pts',(3.7818353500817,-1.,-1.04003862055798));
#72108=CARTESIAN_POINT('Ctrl Pts',(3.7818353500817,1.,-1.04003862055798));
#72109=CARTESIAN_POINT('Ctrl Pts',(3.78821910787179,-1.,-1.04404924374422));
#72110=CARTESIAN_POINT('Ctrl Pts',(3.78821910787179,1.,-1.04404924374422));
#72111=CARTESIAN_POINT('Ctrl Pts',(3.79459440308786,-1.,-1.04810913267639));
#72112=CARTESIAN_POINT('Ctrl Pts',(3.79459440308786,1.,-1.04810913267639));
#72113=CARTESIAN_POINT('Ctrl Pts',(3.80095039790681,-1.,-1.05221457990016));
#72114=CARTESIAN_POINT('Ctrl Pts',(3.80095039790681,1.,-1.05221457990016));
#72115=CARTESIAN_POINT('Ctrl Pts',(3.80727913637791,-1.,-1.05636266918644));
#72116=CARTESIAN_POINT('Ctrl Pts',(3.80727913637791,1.,-1.05636266918644));
#72117=CARTESIAN_POINT('Ctrl Pts',(3.8135786611749,-1.,-1.06055206187299));
#72118=CARTESIAN_POINT('Ctrl Pts',(3.8135786611749,1.,-1.06055206187299));
#72119=CARTESIAN_POINT('Ctrl Pts',(3.81985083953012,-1.,-1.0647824403893));
#72120=CARTESIAN_POINT('Ctrl Pts',(3.81985083953012,1.,-1.0647824403893));
#72121=CARTESIAN_POINT('Ctrl Pts',(3.82609989967276,-1.,-1.06905413180359));
#72122=CARTESIAN_POINT('Ctrl Pts',(3.82609989967276,1.,-1.06905413180359));
#72123=CARTESIAN_POINT('Ctrl Pts',(3.83233071195144,-1.,-1.07336766633459));
#72124=CARTESIAN_POINT('Ctrl Pts',(3.83233071195144,1.,-1.07336766633459));
#72125=CARTESIAN_POINT('Ctrl Pts',(3.83854714117491,-1.,-1.07772335353858));
#72126=CARTESIAN_POINT('Ctrl Pts',(3.83854714117491,1.,-1.07772335353858));
#72127=CARTESIAN_POINT('Ctrl Pts',(3.8447504803063,-1.,-1.08212087917991));
#72128=CARTESIAN_POINT('Ctrl Pts',(3.8447504803063,1.,-1.08212087917991));
#72129=CARTESIAN_POINT('Ctrl Pts',(3.85094025222713,-1.,-1.08655950846384));
#72130=CARTESIAN_POINT('Ctrl Pts',(3.85094025222713,1.,-1.08655950846384));
#72131=CARTESIAN_POINT('Ctrl Pts',(3.85711487933931,-1.,-1.09103825516294));
#72132=CARTESIAN_POINT('Ctrl Pts',(3.85711487933931,1.,-1.09103825516294));
#72133=CARTESIAN_POINT('Ctrl Pts',(3.86327241021247,-1.,-1.09555606505013));
#72134=CARTESIAN_POINT('Ctrl Pts',(3.86327241021247,1.,-1.09555606505013));
#72135=CARTESIAN_POINT('Ctrl Pts',(3.86941120134849,-1.,-1.10011198761195));
#72136=CARTESIAN_POINT('Ctrl Pts',(3.86941120134849,1.,-1.10011198761195));
#72137=CARTESIAN_POINT('Ctrl Pts',(3.87553067187514,-1.,-1.10470536603287));
#72138=CARTESIAN_POINT('Ctrl Pts',(3.87553067187514,1.,-1.10470536603287));
#72139=CARTESIAN_POINT('Ctrl Pts',(3.88163105531724,-1.,-1.10933577224008));
#72140=CARTESIAN_POINT('Ctrl Pts',(3.88163105531724,1.,-1.10933577224008));
#72141=CARTESIAN_POINT('Ctrl Pts',(3.88771308285171,-1.,-1.11400292434429));
#72142=CARTESIAN_POINT('Ctrl Pts',(3.88771308285171,1.,-1.11400292434429));
#72143=CARTESIAN_POINT('Ctrl Pts',(3.89377768340344,-1.,-1.11870660794603));
#72144=CARTESIAN_POINT('Ctrl Pts',(3.89377768340344,1.,-1.11870660794603));
#72145=CARTESIAN_POINT('Ctrl Pts',(3.89982569750025,-1.,-1.12344660099043));
#72146=CARTESIAN_POINT('Ctrl Pts',(3.89982569750025,1.,-1.12344660099043));
#72147=CARTESIAN_POINT('Ctrl Pts',(3.90585753318737,-1.,-1.12822258281553));
#72148=CARTESIAN_POINT('Ctrl Pts',(3.90585753318737,1.,-1.12822258281553));
#72149=CARTESIAN_POINT('Ctrl Pts',(3.91187321145649,-1.,-1.13303414693896));
#72150=CARTESIAN_POINT('Ctrl Pts',(3.91187321145649,1.,-1.13303414693896));
#72151=CARTESIAN_POINT('Ctrl Pts',(3.91787251936827,-1.,-1.13788084225554));
#72152=CARTESIAN_POINT('Ctrl Pts',(3.91787251936827,1.,-1.13788084225554));
#72153=CARTESIAN_POINT('Ctrl Pts',(3.92385513133997,-1.,-1.14276220561593));
#72154=CARTESIAN_POINT('Ctrl Pts',(3.92385513133997,1.,-1.14276220561593));
#72155=CARTESIAN_POINT('Ctrl Pts',(3.92982073294257,-1.,-1.14767779451124));
#72156=CARTESIAN_POINT('Ctrl Pts',(3.92982073294257,1.,-1.14767779451124));
#72157=CARTESIAN_POINT('Ctrl Pts',(3.9357691705628,-1.,-1.1526272271632));
#72158=CARTESIAN_POINT('Ctrl Pts',(3.9357691705628,1.,-1.1526272271632));
#72159=CARTESIAN_POINT('Ctrl Pts',(3.94170046685203,-1.,-1.15761018340956));
#72160=CARTESIAN_POINT('Ctrl Pts',(3.94170046685203,1.,-1.15761018340956));
#72161=CARTESIAN_POINT('Ctrl Pts',(3.94761474780583,-1.,-1.16262637999157));
#72162=CARTESIAN_POINT('Ctrl Pts',(3.94761474780583,1.,-1.16262637999157));
#72163=CARTESIAN_POINT('Ctrl Pts',(3.95351219509876,-1.,-1.16767555244438));
#72164=CARTESIAN_POINT('Ctrl Pts',(3.95351219509876,1.,-1.16767555244438));
#72165=CARTESIAN_POINT('Ctrl Pts',(3.95939299213276,-1.,-1.17275743590361));
#72166=CARTESIAN_POINT('Ctrl Pts',(3.95939299213276,1.,-1.17275743590361));
#72167=CARTESIAN_POINT('Ctrl Pts',(3.96525726358159,-1.,-1.17787174135592));
#72168=CARTESIAN_POINT('Ctrl Pts',(3.96525726358159,1.,-1.17787174135592));
#72169=CARTESIAN_POINT('Ctrl Pts',(3.97110505165415,-1.,-1.18301815039831));
#72170=CARTESIAN_POINT('Ctrl Pts',(3.97110505165415,1.,-1.18301815039831));
#72171=CARTESIAN_POINT('Ctrl Pts',(3.97693634767754,-1.,-1.18819633715539));
#72172=CARTESIAN_POINT('Ctrl Pts',(3.97693634767754,1.,-1.18819633715539));
#72173=CARTESIAN_POINT('Ctrl Pts',(3.98275111052561,-1.,-1.19340598349475));
#72174=CARTESIAN_POINT('Ctrl Pts',(3.98275111052561,1.,-1.19340598349475));
#72175=CARTESIAN_POINT('Ctrl Pts',(3.98854928957189,-1.,-1.19864679609566));
#72176=CARTESIAN_POINT('Ctrl Pts',(3.98854928957189,1.,-1.19864679609566));
#72177=CARTESIAN_POINT('Ctrl Pts',(3.99433084799666,-1.,-1.20391852375139));
#72178=CARTESIAN_POINT('Ctrl Pts',(3.99433084799666,1.,-1.20391852375139));
#72179=CARTESIAN_POINT('Ctrl Pts',(4.00009577950721,-1.,-1.20922097029551));
#72180=CARTESIAN_POINT('Ctrl Pts',(4.00009577950721,1.,-1.20922097029551));
#72181=CARTESIAN_POINT('Ctrl Pts',(4.00584409522722,-1.,-1.21455398918133));
#72182=CARTESIAN_POINT('Ctrl Pts',(4.00584409522722,1.,-1.21455398918133));
#72183=CARTESIAN_POINT('Ctrl Pts',(4.01042947140789,-1.,-1.21884478244403));
#72184=CARTESIAN_POINT('Ctrl Pts',(4.01042947140789,1.,-1.21884478244403));
#72185=CARTESIAN_POINT('Ctrl Pts',(4.01386104433519,-1.,-1.22207656455845));
#72186=CARTESIAN_POINT('Ctrl Pts',(4.01386104433519,1.,-1.22207656455845));
#72187=CARTESIAN_POINT('Ctrl Pts',(4.01614544569895,-1.,-1.22423716681317));
#72188=CARTESIAN_POINT('Ctrl Pts',(4.01614544569895,1.,-1.22423716681317));
#72189=CARTESIAN_POINT('Ctrl Pts',(4.01728681790024,-1.,-1.22531898815164));
#72190=CARTESIAN_POINT('Ctrl Pts',(4.01728681790024,1.,-1.22531898815164));
#72191=CARTESIAN_POINT('',(3.62400312501199,1.,-0.963899035118984));
#72192=CARTESIAN_POINT('Ctrl Pts',(3.62400312501199,-1.,-0.963899035118986));
#72193=CARTESIAN_POINT('Ctrl Pts',(3.62400312501199,-0.666666666666667,
-0.963899035118986));
#72194=CARTESIAN_POINT('Ctrl Pts',(3.62400312501199,-0.333333333333333,
-0.963899035118986));
#72195=CARTESIAN_POINT('Ctrl Pts',(3.62400312501199,0.333333333333333,-0.963899035118986));
#72196=CARTESIAN_POINT('Ctrl Pts',(3.62400312501199,0.666666666666667,-0.963899035118986));
#72197=CARTESIAN_POINT('Ctrl Pts',(3.62400312501199,1.,-0.963899035118986));
#72198=CARTESIAN_POINT('',(4.01728681790024,1.,-1.22531898815164));
#72199=CARTESIAN_POINT('',(4.01728681790024,0.,-1.22531898815164));
#72200=CARTESIAN_POINT('Ctrl Pts',(3.62400312501199,1.,-0.963899035118985));
#72201=CARTESIAN_POINT('Ctrl Pts',(3.62404828878374,1.,-0.963880158556713));
#72202=CARTESIAN_POINT('Ctrl Pts',(3.62424461507455,1.,-0.963861297423579));
#72203=CARTESIAN_POINT('Ctrl Pts',(3.62489305727516,1.,-0.96395778264259));
#72204=CARTESIAN_POINT('Ctrl Pts',(3.62652618145252,1.,-0.964373850166082));
#72205=CARTESIAN_POINT('Ctrl Pts',(3.62988252139998,1.,-0.965395153165716));
#72206=CARTESIAN_POINT('Ctrl Pts',(3.6349212208096,1.,-0.967052554540878));
#72207=CARTESIAN_POINT('Ctrl Pts',(3.64113946505393,1.,-0.969195124674829));
#72208=CARTESIAN_POINT('Ctrl Pts',(3.64819756447072,1.,-0.971722122060278));
#72209=CARTESIAN_POINT('Ctrl Pts',(3.6557157673487,1.,-0.974519971354139));
#72210=CARTESIAN_POINT('Ctrl Pts',(3.66333049637403,1.,-0.977478312751416));
#72211=CARTESIAN_POINT('Ctrl Pts',(3.67074983340444,1.,-0.980505922458495));
#72212=CARTESIAN_POINT('Ctrl Pts',(3.67782408841876,1.,-0.983550791470865));
#72213=CARTESIAN_POINT('Ctrl Pts',(3.6845531792623,1.,-0.986602639864286));
#72214=CARTESIAN_POINT('Ctrl Pts',(3.69102682138955,1.,-0.989676715398859));
#72215=CARTESIAN_POINT('Ctrl Pts',(3.69738123415696,1.,-0.992802218332104));
#72216=CARTESIAN_POINT('Ctrl Pts',(3.70375282282107,1.,-0.996009819772432));
#72217=CARTESIAN_POINT('Ctrl Pts',(3.7102243971387,1.,-0.999317260756345));
#72218=CARTESIAN_POINT('Ctrl Pts',(3.71680667125047,1.,-1.00272423396802));
#72219=CARTESIAN_POINT('Ctrl Pts',(3.72346803750544,1.,-1.00622000735696));
#72220=CARTESIAN_POINT('Ctrl Pts',(3.73015276704407,1.,-1.00978798539491));
#72221=CARTESIAN_POINT('Ctrl Pts',(3.73680245055747,1.,-1.01341114319906));
#72222=CARTESIAN_POINT('Ctrl Pts',(3.74337942504993,1.,-1.01707794311088));
#72223=CARTESIAN_POINT('Ctrl Pts',(3.74987777155873,1.,-1.02078510487439));
#72224=CARTESIAN_POINT('Ctrl Pts',(3.75631037456224,1.,-1.02453429444668));
#72225=CARTESIAN_POINT('Ctrl Pts',(3.76270122291245,1.,-1.02833014458184));
#72226=CARTESIAN_POINT('Ctrl Pts',(3.76907609832516,1.,-1.03217786604919));
#72227=CARTESIAN_POINT('Ctrl Pts',(3.77545283140427,1.,-1.03608074678008));
#72228=CARTESIAN_POINT('Ctrl Pts',(3.7818353500817,1.,-1.04003862055798));
#72229=CARTESIAN_POINT('Ctrl Pts',(3.78821910787179,1.,-1.04404924374422));
#72230=CARTESIAN_POINT('Ctrl Pts',(3.79459440308786,1.,-1.04810913267639));
#72231=CARTESIAN_POINT('Ctrl Pts',(3.80095039790681,1.,-1.05221457990016));
#72232=CARTESIAN_POINT('Ctrl Pts',(3.80727913637791,1.,-1.05636266918644));
#72233=CARTESIAN_POINT('Ctrl Pts',(3.8135786611749,1.,-1.06055206187299));
#72234=CARTESIAN_POINT('Ctrl Pts',(3.81985083953012,1.,-1.0647824403893));
#72235=CARTESIAN_POINT('Ctrl Pts',(3.82609989967276,1.,-1.06905413180359));
#72236=CARTESIAN_POINT('Ctrl Pts',(3.83233071195144,1.,-1.07336766633459));
#72237=CARTESIAN_POINT('Ctrl Pts',(3.83854714117491,1.,-1.07772335353858));
#72238=CARTESIAN_POINT('Ctrl Pts',(3.8447504803063,1.,-1.08212087917991));
#72239=CARTESIAN_POINT('Ctrl Pts',(3.85094025222713,1.,-1.08655950846384));
#72240=CARTESIAN_POINT('Ctrl Pts',(3.85711487933931,1.,-1.09103825516294));
#72241=CARTESIAN_POINT('Ctrl Pts',(3.86327241021247,1.,-1.09555606505013));
#72242=CARTESIAN_POINT('Ctrl Pts',(3.86941120134849,1.,-1.10011198761195));
#72243=CARTESIAN_POINT('Ctrl Pts',(3.87553067187514,1.,-1.10470536603287));
#72244=CARTESIAN_POINT('Ctrl Pts',(3.88163105531724,1.,-1.10933577224008));
#72245=CARTESIAN_POINT('Ctrl Pts',(3.88771308285171,1.,-1.11400292434429));
#72246=CARTESIAN_POINT('Ctrl Pts',(3.89377768340344,1.,-1.11870660794603));
#72247=CARTESIAN_POINT('Ctrl Pts',(3.89982569750025,1.,-1.12344660099043));
#72248=CARTESIAN_POINT('Ctrl Pts',(3.90585753318737,1.,-1.12822258281553));
#72249=CARTESIAN_POINT('Ctrl Pts',(3.91187321145649,1.,-1.13303414693896));
#72250=CARTESIAN_POINT('Ctrl Pts',(3.91787251936827,1.,-1.13788084225554));
#72251=CARTESIAN_POINT('Ctrl Pts',(3.92385513133997,1.,-1.14276220561593));
#72252=CARTESIAN_POINT('Ctrl Pts',(3.92982073294257,1.,-1.14767779451124));
#72253=CARTESIAN_POINT('Ctrl Pts',(3.9357691705628,1.,-1.1526272271632));
#72254=CARTESIAN_POINT('Ctrl Pts',(3.94170046685203,1.,-1.15761018340956));
#72255=CARTESIAN_POINT('Ctrl Pts',(3.94761474780583,1.,-1.16262637999157));
#72256=CARTESIAN_POINT('Ctrl Pts',(3.95351219509876,1.,-1.16767555244438));
#72257=CARTESIAN_POINT('Ctrl Pts',(3.95939299213276,1.,-1.17275743590361));
#72258=CARTESIAN_POINT('Ctrl Pts',(3.96525726358159,1.,-1.17787174135592));
#72259=CARTESIAN_POINT('Ctrl Pts',(3.97110505165415,1.,-1.18301815039831));
#72260=CARTESIAN_POINT('Ctrl Pts',(3.97693634767754,1.,-1.18819633715539));
#72261=CARTESIAN_POINT('Ctrl Pts',(3.98275111052561,1.,-1.19340598349475));
#72262=CARTESIAN_POINT('Ctrl Pts',(3.98854928957189,1.,-1.19864679609566));
#72263=CARTESIAN_POINT('Ctrl Pts',(3.99433084799666,1.,-1.20391852375139));
#72264=CARTESIAN_POINT('Ctrl Pts',(4.00009577950721,1.,-1.20922097029551));
#72265=CARTESIAN_POINT('Ctrl Pts',(4.00584409522722,1.,-1.21455398918133));
#72266=CARTESIAN_POINT('Ctrl Pts',(4.01042947140789,1.,-1.21884478244403));
#72267=CARTESIAN_POINT('Ctrl Pts',(4.01386104433519,1.,-1.22207656455845));
#72268=CARTESIAN_POINT('Ctrl Pts',(4.01614544569895,1.,-1.22423716681317));
#72269=CARTESIAN_POINT('Ctrl Pts',(4.01728681790024,1.,-1.22531898815164));
#72270=CARTESIAN_POINT('Origin',(4.01728681790024,0.,-1.22531898815164));
#72271=CARTESIAN_POINT('',(3.97027773754922,1.,-1.36999806084572));
#72272=CARTESIAN_POINT('Origin',(0.,0.,0.));
#72273=CARTESIAN_POINT('',(3.66661143271648,1.,-0.786422660833743));
#72274=CARTESIAN_POINT('Origin',(0.,1.,0.));
#72275=CARTESIAN_POINT('Ctrl Pts',(3.66661143271648,1.,-0.786422660833743));
#72276=CARTESIAN_POINT('Ctrl Pts',(3.66661143271648,0.666666666666667,-0.786422660833743));
#72277=CARTESIAN_POINT('Ctrl Pts',(3.66661143271648,0.333333333333333,-0.786422660833743));
#72278=CARTESIAN_POINT('Ctrl Pts',(3.66661143271648,-0.333333333333333,
-0.786422660833743));
#72279=CARTESIAN_POINT('Ctrl Pts',(3.66661143271648,-0.666666666666667,
-0.786422660833742));
#72280=CARTESIAN_POINT('Ctrl Pts',(3.66661143271648,-1.,-0.786422660833742));
#72281=CARTESIAN_POINT('Ctrl Pts',(4.13571194405636,-1.,-0.73204283740062));
#72282=CARTESIAN_POINT('Ctrl Pts',(4.13571194405636,1.,-0.73204283740062));
#72283=CARTESIAN_POINT('Ctrl Pts',(4.13420383737278,-1.,-0.732488575135926));
#72284=CARTESIAN_POINT('Ctrl Pts',(4.13420383737278,1.,-0.732488575135926));
#72285=CARTESIAN_POINT('Ctrl Pts',(4.13118752796397,-1.,-0.733376589325634));
#72286=CARTESIAN_POINT('Ctrl Pts',(4.13118752796397,1.,-0.733376589325634));
#72287=CARTESIAN_POINT('Ctrl Pts',(4.12666277572794,-1.,-0.734698226767513));
#72288=CARTESIAN_POINT('Ctrl Pts',(4.12666277572794,1.,-0.734698226767513));
#72289=CARTESIAN_POINT('Ctrl Pts',(4.12062919626082,-1.,-0.736439634335347));
#72290=CARTESIAN_POINT('Ctrl Pts',(4.12062919626082,1.,-0.736439634335347));
#72291=CARTESIAN_POINT('Ctrl Pts',(4.11308626953795,-1.,-0.738581708229119));
#72292=CARTESIAN_POINT('Ctrl Pts',(4.11308626953795,1.,-0.738581708229119));
#72293=CARTESIAN_POINT('Ctrl Pts',(4.1055424175856,-1.,-0.740688998555152));
#72294=CARTESIAN_POINT('Ctrl Pts',(4.1055424175856,1.,-0.740688998555152));
#72295=CARTESIAN_POINT('Ctrl Pts',(4.09799769702712,-1.,-0.742761369690018));
#72296=CARTESIAN_POINT('Ctrl Pts',(4.09799769702712,1.,-0.742761369690018));
#72297=CARTESIAN_POINT('Ctrl Pts',(4.09045220253011,-1.,-0.744798649705514));
#72298=CARTESIAN_POINT('Ctrl Pts',(4.09045220253011,1.,-0.744798649705514));
#72299=CARTESIAN_POINT('Ctrl Pts',(4.08290608094789,-1.,-0.746800631490822));
#72300=CARTESIAN_POINT('Ctrl Pts',(4.08290608094789,1.,-0.746800631490822));
#72301=CARTESIAN_POINT('Ctrl Pts',(4.07535951055363,-1.,-0.748767076679177));
#72302=CARTESIAN_POINT('Ctrl Pts',(4.07535951055363,1.,-0.748767076679177));
#72303=CARTESIAN_POINT('Ctrl Pts',(4.06781267241886,-1.,-0.750697720483176));
#72304=CARTESIAN_POINT('Ctrl Pts',(4.06781267241886,1.,-0.750697720483176));
#72305=CARTESIAN_POINT('Ctrl Pts',(4.06026572221399,-1.,-0.752592276482869));
#72306=CARTESIAN_POINT('Ctrl Pts',(4.06026572221399,1.,-0.752592276482869));
#72307=CARTESIAN_POINT('Ctrl Pts',(4.05271876688106,-1.,-0.754450441816412));
#72308=CARTESIAN_POINT('Ctrl Pts',(4.05271876688106,1.,-0.754450441816412));
#72309=CARTESIAN_POINT('Ctrl Pts',(4.04517182654344,-1.,-0.756271902370187));
#72310=CARTESIAN_POINT('Ctrl Pts',(4.04517182654344,1.,-0.756271902370187));
#72311=CARTESIAN_POINT('Ctrl Pts',(4.03762485803468,-1.,-0.758056338885554));
#72312=CARTESIAN_POINT('Ctrl Pts',(4.03762485803468,1.,-0.758056338885554));
#72313=CARTESIAN_POINT('Ctrl Pts',(4.0300778195465,-1.,-0.759803433244166));
#72314=CARTESIAN_POINT('Ctrl Pts',(4.0300778195465,1.,-0.759803433244166));
#72315=CARTESIAN_POINT('Ctrl Pts',(4.02253072741347,-1.,-0.761512875859942));
#72316=CARTESIAN_POINT('Ctrl Pts',(4.02253072741347,1.,-0.761512875859942));
#72317=CARTESIAN_POINT('Ctrl Pts',(4.01498370680434,-1.,-0.763184371182827));
#72318=CARTESIAN_POINT('Ctrl Pts',(4.01498370680434,1.,-0.763184371182827));
#72319=CARTESIAN_POINT('Ctrl Pts',(4.00743706791366,-1.,-0.764817648784947));
#72320=CARTESIAN_POINT('Ctrl Pts',(4.00743706791366,1.,-0.764817648784947));
#72321=CARTESIAN_POINT('Ctrl Pts',(3.99989129179464,-1.,-0.766412457135786));
#72322=CARTESIAN_POINT('Ctrl Pts',(3.99989129179464,1.,-0.766412457135786));
#72323=CARTESIAN_POINT('Ctrl Pts',(3.99234687880892,-1.,-0.767968531377708));
#72324=CARTESIAN_POINT('Ctrl Pts',(3.99234687880892,1.,-0.767968531377708));
#72325=CARTESIAN_POINT('Ctrl Pts',(3.98480422348403,-1.,-0.76948556624546));
#72326=CARTESIAN_POINT('Ctrl Pts',(3.98480422348403,1.,-0.76948556624546));
#72327=CARTESIAN_POINT('Ctrl Pts',(3.97726349165507,-1.,-0.770963190030504));
#72328=CARTESIAN_POINT('Ctrl Pts',(3.97726349165507,1.,-0.770963190030504));
#72329=CARTESIAN_POINT('Ctrl Pts',(3.96972446532832,-1.,-0.772400931772239));
#72330=CARTESIAN_POINT('Ctrl Pts',(3.96972446532832,1.,-0.772400931772239));
#72331=CARTESIAN_POINT('Ctrl Pts',(3.96218649639876,-1.,-0.773798212026683));
#72332=CARTESIAN_POINT('Ctrl Pts',(3.96218649639876,1.,-0.773798212026683));
#72333=CARTESIAN_POINT('Ctrl Pts',(3.95464885452364,-1.,-0.775154418039442));
#72334=CARTESIAN_POINT('Ctrl Pts',(3.95464885452364,1.,-0.775154418039442));
#72335=CARTESIAN_POINT('Ctrl Pts',(3.94711101619471,-1.,-0.77646896669796));
#72336=CARTESIAN_POINT('Ctrl Pts',(3.94711101619471,1.,-0.77646896669796));
#72337=CARTESIAN_POINT('Ctrl Pts',(3.93957296768098,-1.,-0.77774137056855));
#72338=CARTESIAN_POINT('Ctrl Pts',(3.93957296768098,1.,-0.77774137056855));
#72339=CARTESIAN_POINT('Ctrl Pts',(3.93203552473153,-1.,-0.778971308134786));
#72340=CARTESIAN_POINT('Ctrl Pts',(3.93203552473153,1.,-0.778971308134786));
#72341=CARTESIAN_POINT('Ctrl Pts',(3.92450058323799,-1.,-0.780158678615507));
#72342=CARTESIAN_POINT('Ctrl Pts',(3.92450058323799,1.,-0.780158678615507));
#72343=CARTESIAN_POINT('Ctrl Pts',(3.9169703605466,-1.,-0.781303428618344));
#72344=CARTESIAN_POINT('Ctrl Pts',(3.9169703605466,1.,-0.781303428618344));
#72345=CARTESIAN_POINT('Ctrl Pts',(3.90944671004536,-1.,-0.782405395622759));
#72346=CARTESIAN_POINT('Ctrl Pts',(3.90944671004536,1.,-0.782405395622759));
#72347=CARTESIAN_POINT('Ctrl Pts',(3.90193039043971,-1.,-0.783464141529083));
#72348=CARTESIAN_POINT('Ctrl Pts',(3.90193039043971,1.,-0.783464141529083));
#72349=CARTESIAN_POINT('Ctrl Pts',(3.89442039235105,-1.,-0.784478799358336));
#72350=CARTESIAN_POINT('Ctrl Pts',(3.89442039235105,1.,-0.784478799358336));
#72351=CARTESIAN_POINT('Ctrl Pts',(3.88691313167399,-1.,-0.785447890340723));
#72352=CARTESIAN_POINT('Ctrl Pts',(3.88691313167399,1.,-0.785447890340723));
#72353=CARTESIAN_POINT('Ctrl Pts',(3.87940402818186,-1.,-0.786369675812592));
#72354=CARTESIAN_POINT('Ctrl Pts',(3.87940402818186,1.,-0.786369675812592));
#72355=CARTESIAN_POINT('Ctrl Pts',(3.87188916600905,-1.,-0.787242527617981));
#72356=CARTESIAN_POINT('Ctrl Pts',(3.87188916600905,1.,-0.787242527617981));
#72357=CARTESIAN_POINT('Ctrl Pts',(3.86436702561342,-1.,-0.788065315093771));
#72358=CARTESIAN_POINT('Ctrl Pts',(3.86436702561342,1.,-0.788065315093771));
#72359=CARTESIAN_POINT('Ctrl Pts',(3.85683995872536,-1.,-0.788837734090688));
#72360=CARTESIAN_POINT('Ctrl Pts',(3.85683995872536,1.,-0.788837734090688));
#72361=CARTESIAN_POINT('Ctrl Pts',(3.8493163780891,-1.,-0.789560798155619));
#72362=CARTESIAN_POINT('Ctrl Pts',(3.8493163780891,1.,-0.789560798155619));
#72363=CARTESIAN_POINT('Ctrl Pts',(3.84180762342476,-1.,-0.790236124191289));
#72364=CARTESIAN_POINT('Ctrl Pts',(3.84180762342476,1.,-0.790236124191289));
#72365=CARTESIAN_POINT('Ctrl Pts',(3.83432392054804,-1.,-0.79086501270534));
#72366=CARTESIAN_POINT('Ctrl Pts',(3.83432392054804,1.,-0.79086501270534));
#72367=CARTESIAN_POINT('Ctrl Pts',(3.82687033899799,-1.,-0.791447528662381));
#72368=CARTESIAN_POINT('Ctrl Pts',(3.82687033899799,1.,-0.791447528662381));
#72369=CARTESIAN_POINT('Ctrl Pts',(3.81944345442237,-1.,-0.791981740718607));
#72370=CARTESIAN_POINT('Ctrl Pts',(3.81944345442237,1.,-0.791981740718607));
#72371=CARTESIAN_POINT('Ctrl Pts',(3.81202588694726,-1.,-0.792462483517568));
#72372=CARTESIAN_POINT('Ctrl Pts',(3.81202588694726,1.,-0.792462483517568));
#72373=CARTESIAN_POINT('Ctrl Pts',(3.80459229925598,-1.,-0.792882695234693));
#72374=CARTESIAN_POINT('Ctrl Pts',(3.80459229925598,1.,-0.792882695234693));
#72375=CARTESIAN_POINT('Ctrl Pts',(3.79711921389862,-1.,-0.793235612973201));
#72376=CARTESIAN_POINT('Ctrl Pts',(3.79711921389862,1.,-0.793235612973201));
#72377=CARTESIAN_POINT('Ctrl Pts',(3.78959439439222,-1.,-0.793516871680966));
#72378=CARTESIAN_POINT('Ctrl Pts',(3.78959439439222,1.,-0.793516871680966));
#72379=CARTESIAN_POINT('Ctrl Pts',(3.78202460377617,-1.,-0.79372623578134));
#72380=CARTESIAN_POINT('Ctrl Pts',(3.78202460377617,1.,-0.79372623578134));
#72381=CARTESIAN_POINT('Ctrl Pts',(3.77444863801264,-1.,-0.793870523787515));
#72382=CARTESIAN_POINT('Ctrl Pts',(3.77444863801264,1.,-0.793870523787515));
#72383=CARTESIAN_POINT('Ctrl Pts',(3.76692626931184,-1.,-0.793961083689141));
#72384=CARTESIAN_POINT('Ctrl Pts',(3.76692626931184,1.,-0.793961083689141));
#72385=CARTESIAN_POINT('Ctrl Pts',(3.75951468666325,-1.,-0.794008429135047));
#72386=CARTESIAN_POINT('Ctrl Pts',(3.75951468666325,1.,-0.794008429135047));
#72387=CARTESIAN_POINT('Ctrl Pts',(3.75224692493895,-1.,-0.794017347371441));
#72388=CARTESIAN_POINT('Ctrl Pts',(3.75224692493895,1.,-0.794017347371441));
#72389=CARTESIAN_POINT('Ctrl Pts',(3.74511357728827,-1.,-0.79398270045988));
#72390=CARTESIAN_POINT('Ctrl Pts',(3.74511357728827,1.,-0.79398270045988));
#72391=CARTESIAN_POINT('Ctrl Pts',(3.73803280541576,-1.,-0.793882700936791));
#72392=CARTESIAN_POINT('Ctrl Pts',(3.73803280541576,1.,-0.793882700936791));
#72393=CARTESIAN_POINT('Ctrl Pts',(3.7308691469564,-1.,-0.793682750269348));
#72394=CARTESIAN_POINT('Ctrl Pts',(3.7308691469564,1.,-0.793682750269348));
#72395=CARTESIAN_POINT('Ctrl Pts',(3.7234879729357,-1.,-0.793347023783871));
#72396=CARTESIAN_POINT('Ctrl Pts',(3.7234879729357,1.,-0.793347023783871));
#72397=CARTESIAN_POINT('Ctrl Pts',(3.7158024239604,-1.,-0.792848377370116));
#72398=CARTESIAN_POINT('Ctrl Pts',(3.7158024239604,1.,-0.792848377370116));
#72399=CARTESIAN_POINT('Ctrl Pts',(3.70781724021879,-1.,-0.792177688845968));
#72400=CARTESIAN_POINT('Ctrl Pts',(3.70781724021879,1.,-0.792177688845968));
#72401=CARTESIAN_POINT('Ctrl Pts',(3.69968940808982,-1.,-0.791356575696509));
#72402=CARTESIAN_POINT('Ctrl Pts',(3.69968940808982,1.,-0.791356575696509));
#72403=CARTESIAN_POINT('Ctrl Pts',(3.69172044327754,-1.,-0.79043628498958));
#72404=CARTESIAN_POINT('Ctrl Pts',(3.69172044327754,1.,-0.79043628498958));
#72405=CARTESIAN_POINT('Ctrl Pts',(3.68428439784285,-1.,-0.789483546065159));
#72406=CARTESIAN_POINT('Ctrl Pts',(3.68428439784285,1.,-0.789483546065159));
#72407=CARTESIAN_POINT('Ctrl Pts',(3.67777119516438,-1.,-0.788569566220663));
#72408=CARTESIAN_POINT('Ctrl Pts',(3.67777119516438,1.,-0.788569566220663));
#72409=CARTESIAN_POINT('Ctrl Pts',(3.672529236635,-1.,-0.787758799995427));
#72410=CARTESIAN_POINT('Ctrl Pts',(3.672529236635,1.,-0.787758799995427));
#72411=CARTESIAN_POINT('Ctrl Pts',(3.66879484800625,-1.,-0.787095252589508));
#72412=CARTESIAN_POINT('Ctrl Pts',(3.66879484800625,1.,-0.787095252589508));
#72413=CARTESIAN_POINT('Ctrl Pts',(3.66710211819938,-1.,-0.786698783541658));
#72414=CARTESIAN_POINT('Ctrl Pts',(3.66710211819938,1.,-0.786698783541658));
#72415=CARTESIAN_POINT('Ctrl Pts',(3.66657784454965,-1.,-0.786480236184947));
#72416=CARTESIAN_POINT('Ctrl Pts',(3.66657784454965,1.,-0.786480236184947));
#72417=CARTESIAN_POINT('Ctrl Pts',(3.66655932661846,-1.,-0.78636952818304));
#72418=CARTESIAN_POINT('Ctrl Pts',(3.66655932661846,1.,-0.78636952818304));
#72419=CARTESIAN_POINT('Ctrl Pts',(3.66663282329846,-1.,-0.786322922920599));
#72420=CARTESIAN_POINT('Ctrl Pts',(3.66663282329846,1.,-0.786322922920599));
#72421=CARTESIAN_POINT('',(4.13571194405636,1.,-0.73204283740062));
#72422=CARTESIAN_POINT('Ctrl Pts',(4.13571194405636,1.,-0.73204283740062));
#72423=CARTESIAN_POINT('Ctrl Pts',(4.13420383737278,1.,-0.732488575135926));
#72424=CARTESIAN_POINT('Ctrl Pts',(4.13118752796397,1.,-0.733376589325634));
#72425=CARTESIAN_POINT('Ctrl Pts',(4.12666277572794,1.,-0.734698226767513));
#72426=CARTESIAN_POINT('Ctrl Pts',(4.12062919626082,1.,-0.736439634335347));
#72427=CARTESIAN_POINT('Ctrl Pts',(4.11308626953795,1.,-0.738581708229119));
#72428=CARTESIAN_POINT('Ctrl Pts',(4.1055424175856,1.,-0.740688998555152));
#72429=CARTESIAN_POINT('Ctrl Pts',(4.09799769702712,1.,-0.742761369690018));
#72430=CARTESIAN_POINT('Ctrl Pts',(4.09045220253011,1.,-0.744798649705514));
#72431=CARTESIAN_POINT('Ctrl Pts',(4.08290608094789,1.,-0.746800631490822));
#72432=CARTESIAN_POINT('Ctrl Pts',(4.07535951055363,1.,-0.748767076679177));
#72433=CARTESIAN_POINT('Ctrl Pts',(4.06781267241886,1.,-0.750697720483176));
#72434=CARTESIAN_POINT('Ctrl Pts',(4.06026572221399,1.,-0.752592276482869));
#72435=CARTESIAN_POINT('Ctrl Pts',(4.05271876688106,1.,-0.754450441816412));
#72436=CARTESIAN_POINT('Ctrl Pts',(4.04517182654344,1.,-0.756271902370187));
#72437=CARTESIAN_POINT('Ctrl Pts',(4.03762485803468,1.,-0.758056338885554));
#72438=CARTESIAN_POINT('Ctrl Pts',(4.0300778195465,1.,-0.759803433244166));
#72439=CARTESIAN_POINT('Ctrl Pts',(4.02253072741347,1.,-0.761512875859942));
#72440=CARTESIAN_POINT('Ctrl Pts',(4.01498370680434,1.,-0.763184371182827));
#72441=CARTESIAN_POINT('Ctrl Pts',(4.00743706791366,1.,-0.764817648784947));
#72442=CARTESIAN_POINT('Ctrl Pts',(3.99989129179464,1.,-0.766412457135786));
#72443=CARTESIAN_POINT('Ctrl Pts',(3.99234687880892,1.,-0.767968531377708));
#72444=CARTESIAN_POINT('Ctrl Pts',(3.98480422348403,1.,-0.76948556624546));
#72445=CARTESIAN_POINT('Ctrl Pts',(3.97726349165507,1.,-0.770963190030504));
#72446=CARTESIAN_POINT('Ctrl Pts',(3.96972446532832,1.,-0.772400931772239));
#72447=CARTESIAN_POINT('Ctrl Pts',(3.96218649639876,1.,-0.773798212026683));
#72448=CARTESIAN_POINT('Ctrl Pts',(3.95464885452364,1.,-0.775154418039442));
#72449=CARTESIAN_POINT('Ctrl Pts',(3.94711101619471,1.,-0.77646896669796));
#72450=CARTESIAN_POINT('Ctrl Pts',(3.93957296768098,1.,-0.77774137056855));
#72451=CARTESIAN_POINT('Ctrl Pts',(3.93203552473153,1.,-0.778971308134786));
#72452=CARTESIAN_POINT('Ctrl Pts',(3.92450058323799,1.,-0.780158678615507));
#72453=CARTESIAN_POINT('Ctrl Pts',(3.9169703605466,1.,-0.781303428618344));
#72454=CARTESIAN_POINT('Ctrl Pts',(3.90944671004536,1.,-0.782405395622759));
#72455=CARTESIAN_POINT('Ctrl Pts',(3.90193039043971,1.,-0.783464141529083));
#72456=CARTESIAN_POINT('Ctrl Pts',(3.89442039235105,1.,-0.784478799358336));
#72457=CARTESIAN_POINT('Ctrl Pts',(3.88691313167399,1.,-0.785447890340723));
#72458=CARTESIAN_POINT('Ctrl Pts',(3.87940402818186,1.,-0.786369675812592));
#72459=CARTESIAN_POINT('Ctrl Pts',(3.87188916600905,1.,-0.787242527617981));
#72460=CARTESIAN_POINT('Ctrl Pts',(3.86436702561342,1.,-0.788065315093771));
#72461=CARTESIAN_POINT('Ctrl Pts',(3.85683995872536,1.,-0.788837734090688));
#72462=CARTESIAN_POINT('Ctrl Pts',(3.8493163780891,1.,-0.789560798155619));
#72463=CARTESIAN_POINT('Ctrl Pts',(3.84180762342476,1.,-0.790236124191289));
#72464=CARTESIAN_POINT('Ctrl Pts',(3.83432392054804,1.,-0.79086501270534));
#72465=CARTESIAN_POINT('Ctrl Pts',(3.82687033899799,1.,-0.791447528662381));
#72466=CARTESIAN_POINT('Ctrl Pts',(3.81944345442237,1.,-0.791981740718607));
#72467=CARTESIAN_POINT('Ctrl Pts',(3.81202588694726,1.,-0.792462483517568));
#72468=CARTESIAN_POINT('Ctrl Pts',(3.80459229925598,1.,-0.792882695234693));
#72469=CARTESIAN_POINT('Ctrl Pts',(3.79711921389862,1.,-0.793235612973201));
#72470=CARTESIAN_POINT('Ctrl Pts',(3.78959439439222,1.,-0.793516871680966));
#72471=CARTESIAN_POINT('Ctrl Pts',(3.78202460377617,1.,-0.79372623578134));
#72472=CARTESIAN_POINT('Ctrl Pts',(3.77444863801264,1.,-0.793870523787515));
#72473=CARTESIAN_POINT('Ctrl Pts',(3.76692626931184,1.,-0.793961083689141));
#72474=CARTESIAN_POINT('Ctrl Pts',(3.75951468666325,1.,-0.794008429135047));
#72475=CARTESIAN_POINT('Ctrl Pts',(3.75224692493895,1.,-0.794017347371441));
#72476=CARTESIAN_POINT('Ctrl Pts',(3.74511357728827,1.,-0.79398270045988));
#72477=CARTESIAN_POINT('Ctrl Pts',(3.73803280541576,1.,-0.793882700936791));
#72478=CARTESIAN_POINT('Ctrl Pts',(3.7308691469564,1.,-0.793682750269348));
#72479=CARTESIAN_POINT('Ctrl Pts',(3.7234879729357,1.,-0.793347023783871));
#72480=CARTESIAN_POINT('Ctrl Pts',(3.7158024239604,1.,-0.792848377370116));
#72481=CARTESIAN_POINT('Ctrl Pts',(3.70781724021879,1.,-0.792177688845968));
#72482=CARTESIAN_POINT('Ctrl Pts',(3.69968940808982,1.,-0.791356575696509));
#72483=CARTESIAN_POINT('Ctrl Pts',(3.69172044327754,1.,-0.79043628498958));
#72484=CARTESIAN_POINT('Ctrl Pts',(3.68428439784285,1.,-0.789483546065159));
#72485=CARTESIAN_POINT('Ctrl Pts',(3.67777119516438,1.,-0.788569566220663));
#72486=CARTESIAN_POINT('Ctrl Pts',(3.672529236635,1.,-0.787758799995427));
#72487=CARTESIAN_POINT('Ctrl Pts',(3.66907505398769,1.,-0.787145041181589));
#72488=CARTESIAN_POINT('Ctrl Pts',(3.66743103898844,1.,-0.7867743371985));
#72489=CARTESIAN_POINT('Ctrl Pts',(3.66680946938396,1.,-0.78656591955989));
#72490=CARTESIAN_POINT('Ctrl Pts',(3.66664310415236,1.,-0.786459983896781));
#72491=CARTESIAN_POINT('Ctrl Pts',(3.66661143271648,1.,-0.786422660833743));
#72492=CARTESIAN_POINT('',(4.13571194405636,0.,-0.73204283740062));
#72493=CARTESIAN_POINT('Origin',(4.15950947128175,0.,-0.581791163835815));
#72494=CARTESIAN_POINT('',(4.15950947128175,1.,-0.581791163835815));
#72495=CARTESIAN_POINT('',(4.13571194405636,1.,-0.73204283740062));
#72496=CARTESIAN_POINT('',(4.15950947128175,0.,-0.581791163835815));
#72497=CARTESIAN_POINT('Ctrl Pts',(3.73016218570874,-1.,-0.385214314776329));
#72498=CARTESIAN_POINT('Ctrl Pts',(3.73016218570874,1.,-0.385214314776329));
#72499=CARTESIAN_POINT('Ctrl Pts',(3.73010668803185,-1.,-0.385147278814804));
#72500=CARTESIAN_POINT('Ctrl Pts',(3.73010668803185,1.,-0.385147278814804));
#72501=CARTESIAN_POINT('Ctrl Pts',(3.73015851028729,-1.,-0.385047711603887));
#72502=CARTESIAN_POINT('Ctrl Pts',(3.73015851028729,1.,-0.385047711603887));
#72503=CARTESIAN_POINT('Ctrl Pts',(3.73072465900727,-1.,-0.385001870183842));
#72504=CARTESIAN_POINT('Ctrl Pts',(3.73072465900727,1.,-0.385001870183842));
#72505=CARTESIAN_POINT('Ctrl Pts',(3.73245705639337,-1.,-0.385147887989515));
#72506=CARTESIAN_POINT('Ctrl Pts',(3.73245705639337,1.,-0.385147887989515));
#72507=CARTESIAN_POINT('Ctrl Pts',(3.73621371845475,-1.,-0.385670806454744));
#72508=CARTESIAN_POINT('Ctrl Pts',(3.73621371845475,1.,-0.385670806454744));
#72509=CARTESIAN_POINT('Ctrl Pts',(3.74144965781088,-1.,-0.386519576222036));
#72510=CARTESIAN_POINT('Ctrl Pts',(3.74144965781088,1.,-0.386519576222036));
#72511=CARTESIAN_POINT('Ctrl Pts',(3.74792651696269,-1.,-0.387663020050396));
#72512=CARTESIAN_POINT('Ctrl Pts',(3.74792651696269,1.,-0.387663020050396));
#72513=CARTESIAN_POINT('Ctrl Pts',(3.75529302894757,-1.,-0.389054775898251));
#72514=CARTESIAN_POINT('Ctrl Pts',(3.75529302894757,1.,-0.389054775898251));
#72515=CARTESIAN_POINT('Ctrl Pts',(3.76315635032993,-1.,-0.390642072979259));
#72516=CARTESIAN_POINT('Ctrl Pts',(3.76315635032993,1.,-0.390642072979259));
#72517=CARTESIAN_POINT('Ctrl Pts',(3.77114011595892,-1.,-0.392372786223347));
#72518=CARTESIAN_POINT('Ctrl Pts',(3.77114011595892,1.,-0.392372786223347));
#72519=CARTESIAN_POINT('Ctrl Pts',(3.77894173114368,-1.,-0.394202481011595));
#72520=CARTESIAN_POINT('Ctrl Pts',(3.77894173114368,1.,-0.394202481011595));
#72521=CARTESIAN_POINT('Ctrl Pts',(3.78640521279479,-1.,-0.396103205335029));
#72522=CARTESIAN_POINT('Ctrl Pts',(3.78640521279479,1.,-0.396103205335029));
#72523=CARTESIAN_POINT('Ctrl Pts',(3.79352887163457,-1.,-0.398064818684159));
#72524=CARTESIAN_POINT('Ctrl Pts',(3.79352887163457,1.,-0.398064818684159));
#72525=CARTESIAN_POINT('Ctrl Pts',(3.80040370384659,-1.,-0.400088346504727));
#72526=CARTESIAN_POINT('Ctrl Pts',(3.80040370384659,1.,-0.400088346504727));
#72527=CARTESIAN_POINT('Ctrl Pts',(3.80716881962763,-1.,-0.402181320148475));
#72528=CARTESIAN_POINT('Ctrl Pts',(3.80716881962763,1.,-0.402181320148475));
#72529=CARTESIAN_POINT('Ctrl Pts',(3.81396374287762,-1.,-0.404352694628237));
#72530=CARTESIAN_POINT('Ctrl Pts',(3.81396374287762,1.,-0.404352694628237));
#72531=CARTESIAN_POINT('Ctrl Pts',(3.82087303913741,-1.,-0.406607038258907));
#72532=CARTESIAN_POINT('Ctrl Pts',(3.82087303913741,1.,-0.406607038258907));
#72533=CARTESIAN_POINT('Ctrl Pts',(3.82790724256397,-1.,-0.408942371447377));
#72534=CARTESIAN_POINT('Ctrl Pts',(3.82790724256397,1.,-0.408942371447377));
#72535=CARTESIAN_POINT('Ctrl Pts',(3.83503345578645,-1.,-0.41135303879846));
#72536=CARTESIAN_POINT('Ctrl Pts',(3.83503345578645,1.,-0.41135303879846));
#72537=CARTESIAN_POINT('Ctrl Pts',(3.84219403994742,-1.,-0.413831367016727));
#72538=CARTESIAN_POINT('Ctrl Pts',(3.84219403994742,1.,-0.413831367016727));
#72539=CARTESIAN_POINT('Ctrl Pts',(3.8493286415751,-1.,-0.41636967805292));
#72540=CARTESIAN_POINT('Ctrl Pts',(3.8493286415751,1.,-0.41636967805292));
#72541=CARTESIAN_POINT('Ctrl Pts',(3.85639825648031,-1.,-0.41896246808681));
#72542=CARTESIAN_POINT('Ctrl Pts',(3.85639825648031,1.,-0.41896246808681));
#72543=CARTESIAN_POINT('Ctrl Pts',(3.86339652542749,-1.,-0.421607423177576));
#72544=CARTESIAN_POINT('Ctrl Pts',(3.86339652542749,1.,-0.421607423177576));
#72545=CARTESIAN_POINT('Ctrl Pts',(3.87033643487882,-1.,-0.424304173195143));
#72546=CARTESIAN_POINT('Ctrl Pts',(3.87033643487882,1.,-0.424304173195143));
#72547=CARTESIAN_POINT('Ctrl Pts',(3.87724240306609,-1.,-0.427053541173469));
#72548=CARTESIAN_POINT('Ctrl Pts',(3.87724240306609,1.,-0.427053541173469));
#72549=CARTESIAN_POINT('Ctrl Pts',(3.88414070943334,-1.,-0.429856640579734));
#72550=CARTESIAN_POINT('Ctrl Pts',(3.88414070943334,1.,-0.429856640579734));
#72551=CARTESIAN_POINT('Ctrl Pts',(3.89104947940592,-1.,-0.43271392954444));
#72552=CARTESIAN_POINT('Ctrl Pts',(3.89104947940592,1.,-0.43271392954444));
#72553=CARTESIAN_POINT('Ctrl Pts',(3.8979725665544,-1.,-0.435624629433506));
#72554=CARTESIAN_POINT('Ctrl Pts',(3.8979725665544,1.,-0.435624629433506));
#72555=CARTESIAN_POINT('Ctrl Pts',(3.90490512938546,-1.,-0.438587235458234));
#72556=CARTESIAN_POINT('Ctrl Pts',(3.90490512938546,1.,-0.438587235458234));
#72557=CARTESIAN_POINT('Ctrl Pts',(3.91183704069146,-1.,-0.441599824524048));
#72558=CARTESIAN_POINT('Ctrl Pts',(3.91183704069146,1.,-0.441599824524048));
#72559=CARTESIAN_POINT('Ctrl Pts',(3.91875701610721,-1.,-0.444660430230593));
#72560=CARTESIAN_POINT('Ctrl Pts',(3.91875701610721,1.,-0.444660430230593));
#72561=CARTESIAN_POINT('Ctrl Pts',(3.92565674143424,-1.,-0.447767416837297));
#72562=CARTESIAN_POINT('Ctrl Pts',(3.92565674143424,1.,-0.447767416837297));
#72563=CARTESIAN_POINT('Ctrl Pts',(3.93253407403128,-1.,-0.450919768356347));
#72564=CARTESIAN_POINT('Ctrl Pts',(3.93253407403128,1.,-0.450919768356347));
#72565=CARTESIAN_POINT('Ctrl Pts',(3.93939080846298,-1.,-0.454116879027576));
#72566=CARTESIAN_POINT('Ctrl Pts',(3.93939080846298,1.,-0.454116879027576));
#72567=CARTESIAN_POINT('Ctrl Pts',(3.94623117206675,-1.,-0.457358410451674));
#72568=CARTESIAN_POINT('Ctrl Pts',(3.94623117206675,1.,-0.457358410451674));
#72569=CARTESIAN_POINT('Ctrl Pts',(3.95306005817363,-1.,-0.460644124429119));
#72570=CARTESIAN_POINT('Ctrl Pts',(3.95306005817363,1.,-0.460644124429119));
#72571=CARTESIAN_POINT('Ctrl Pts',(3.95988133243543,-1.,-0.463973722115745));
#72572=CARTESIAN_POINT('Ctrl Pts',(3.95988133243543,1.,-0.463973722115745));
#72573=CARTESIAN_POINT('Ctrl Pts',(3.96669622273946,-1.,-0.467346690880672));
#72574=CARTESIAN_POINT('Ctrl Pts',(3.96669622273946,1.,-0.467346690880672));
#72575=CARTESIAN_POINT('Ctrl Pts',(3.97350414289415,-1.,-0.470762379613478));
#72576=CARTESIAN_POINT('Ctrl Pts',(3.97350414289415,1.,-0.470762379613478));
#72577=CARTESIAN_POINT('Ctrl Pts',(3.9803033804443,-1.,-0.474220061019542));
#72578=CARTESIAN_POINT('Ctrl Pts',(3.9803033804443,1.,-0.474220061019542));
#72579=CARTESIAN_POINT('Ctrl Pts',(3.98709184306743,-1.,-0.477718999122033));
#72580=CARTESIAN_POINT('Ctrl Pts',(3.98709184306743,1.,-0.477718999122033));
#72581=CARTESIAN_POINT('Ctrl Pts',(3.99386775880655,-1.,-0.481258512209638));
#72582=CARTESIAN_POINT('Ctrl Pts',(3.99386775880655,1.,-0.481258512209638));
#72583=CARTESIAN_POINT('Ctrl Pts',(4.00063045119234,-1.,-0.484838042421754));
#72584=CARTESIAN_POINT('Ctrl Pts',(4.00063045119234,1.,-0.484838042421754));
#72585=CARTESIAN_POINT('Ctrl Pts',(4.0073800839092,-1.,-0.488457130424531));
#72586=CARTESIAN_POINT('Ctrl Pts',(4.0073800839092,1.,-0.488457130424531));
#72587=CARTESIAN_POINT('Ctrl Pts',(4.01411733503486,-1.,-0.492115383417931));
#72588=CARTESIAN_POINT('Ctrl Pts',(4.01411733503486,1.,-0.492115383417931));
#72589=CARTESIAN_POINT('Ctrl Pts',(4.02084308851813,-1.,-0.495812444326223));
#72590=CARTESIAN_POINT('Ctrl Pts',(4.02084308851813,1.,-0.495812444326223));
#72591=CARTESIAN_POINT('Ctrl Pts',(4.0275581398015,-1.,-0.49954796234089));
#72592=CARTESIAN_POINT('Ctrl Pts',(4.0275581398015,1.,-0.49954796234089));
#72593=CARTESIAN_POINT('Ctrl Pts',(4.0342628417439,-1.,-0.503321556915514));
#72594=CARTESIAN_POINT('Ctrl Pts',(4.0342628417439,1.,-0.503321556915514));
#72595=CARTESIAN_POINT('Ctrl Pts',(4.04095715149074,-1.,-0.507132823288362));
#72596=CARTESIAN_POINT('Ctrl Pts',(4.04095715149074,1.,-0.507132823288362));
#72597=CARTESIAN_POINT('Ctrl Pts',(4.04764078815591,-1.,-0.510981349219174));
#72598=CARTESIAN_POINT('Ctrl Pts',(4.04764078815591,1.,-0.510981349219174));
#72599=CARTESIAN_POINT('Ctrl Pts',(4.05431335771261,-1.,-0.514866728193104));
#72600=CARTESIAN_POINT('Ctrl Pts',(4.05431335771261,1.,-0.514866728193104));
#72601=CARTESIAN_POINT('Ctrl Pts',(4.06097448037934,-1.,-0.51878857233681));
#72602=CARTESIAN_POINT('Ctrl Pts',(4.06097448037934,1.,-0.51878857233681));
#72603=CARTESIAN_POINT('Ctrl Pts',(4.06762394471075,-1.,-0.522746528602768));
#72604=CARTESIAN_POINT('Ctrl Pts',(4.06762394471075,1.,-0.522746528602768));
#72605=CARTESIAN_POINT('Ctrl Pts',(4.07426172299496,-1.,-0.526740277227));
#72606=CARTESIAN_POINT('Ctrl Pts',(4.07426172299496,1.,-0.526740277227));
#72607=CARTESIAN_POINT('Ctrl Pts',(4.08088789536488,-1.,-0.530769518728076));
#72608=CARTESIAN_POINT('Ctrl Pts',(4.08088789536488,1.,-0.530769518728076));
#72609=CARTESIAN_POINT('Ctrl Pts',(4.08750259988693,-1.,-0.534833963477));
#72610=CARTESIAN_POINT('Ctrl Pts',(4.08750259988693,1.,-0.534833963477));
#72611=CARTESIAN_POINT('Ctrl Pts',(4.09410597627116,-1.,-0.538933321179921));
#72612=CARTESIAN_POINT('Ctrl Pts',(4.09410597627116,1.,-0.538933321179921));
#72613=CARTESIAN_POINT('Ctrl Pts',(4.10069810244473,-1.,-0.543067286878457));
#72614=CARTESIAN_POINT('Ctrl Pts',(4.10069810244473,1.,-0.543067286878457));
#72615=CARTESIAN_POINT('Ctrl Pts',(4.1072789702877,-1.,-0.54723553948676));
#72616=CARTESIAN_POINT('Ctrl Pts',(4.1072789702877,1.,-0.54723553948676));
#72617=CARTESIAN_POINT('Ctrl Pts',(4.11384852025578,-1.,-0.551437758498247));
#72618=CARTESIAN_POINT('Ctrl Pts',(4.11384852025578,1.,-0.551437758498247));
#72619=CARTESIAN_POINT('Ctrl Pts',(4.1204066619623,-1.,-0.555673636130778));
#72620=CARTESIAN_POINT('Ctrl Pts',(4.1204066619623,1.,-0.555673636130778));
#72621=CARTESIAN_POINT('Ctrl Pts',(4.12695329951859,-1.,-0.559942890594628));
#72622=CARTESIAN_POINT('Ctrl Pts',(4.12695329951859,1.,-0.559942890594628));
#72623=CARTESIAN_POINT('Ctrl Pts',(4.13348835726086,-1.,-0.564245279535706));
#72624=CARTESIAN_POINT('Ctrl Pts',(4.13348835726086,1.,-0.564245279535706));
#72625=CARTESIAN_POINT('Ctrl Pts',(4.14001179828669,-1.,-0.568580610187116));
#72626=CARTESIAN_POINT('Ctrl Pts',(4.14001179828669,1.,-0.568580610187116));
#72627=CARTESIAN_POINT('Ctrl Pts',(4.14652361065787,-1.,-0.572948736066277));
#72628=CARTESIAN_POINT('Ctrl Pts',(4.14652361065787,1.,-0.572948736066277));
#72629=CARTESIAN_POINT('Ctrl Pts',(4.1517237611974,-1.,-0.576469391673917));
#72630=CARTESIAN_POINT('Ctrl Pts',(4.1517237611974,1.,-0.576469391673917));
#72631=CARTESIAN_POINT('Ctrl Pts',(4.15561864787379,-1.,-0.579124568912544));
#72632=CARTESIAN_POINT('Ctrl Pts',(4.15561864787379,1.,-0.579124568912544));
#72633=CARTESIAN_POINT('Ctrl Pts',(4.15821291712391,-1.,-0.580901211462913));
#72634=CARTESIAN_POINT('Ctrl Pts',(4.15821291712391,1.,-0.580901211462913));
#72635=CARTESIAN_POINT('Ctrl Pts',(4.15950947128175,-1.,-0.581791163835815));
#72636=CARTESIAN_POINT('Ctrl Pts',(4.15950947128175,1.,-0.581791163835815));
#72637=CARTESIAN_POINT('',(3.73017266276632,1.,-0.385112848332548));
#72638=CARTESIAN_POINT('Ctrl Pts',(3.73017266276632,-1.,-0.385112848332549));
#72639=CARTESIAN_POINT('Ctrl Pts',(3.73017266276632,-0.666666666666667,
-0.385112848332549));
#72640=CARTESIAN_POINT('Ctrl Pts',(3.73017266276632,-0.333333333333333,
-0.385112848332549));
#72641=CARTESIAN_POINT('Ctrl Pts',(3.73017266276632,0.333333333333333,-0.385112848332549));
#72642=CARTESIAN_POINT('Ctrl Pts',(3.73017266276632,0.666666666666667,-0.38511284833255));
#72643=CARTESIAN_POINT('Ctrl Pts',(3.73017266276632,1.,-0.38511284833255));
#72644=CARTESIAN_POINT('Ctrl Pts',(3.73017266276632,1.,-0.385112848332549));
#72645=CARTESIAN_POINT('Ctrl Pts',(3.73021431755218,1.,-0.385087139001609));
#72646=CARTESIAN_POINT('Ctrl Pts',(3.73040527620929,1.,-0.385037797882046));
#72647=CARTESIAN_POINT('Ctrl Pts',(3.731060828624,1.,-0.385031656499142));
#72648=CARTESIAN_POINT('Ctrl Pts',(3.73273893363318,1.,-0.385187124633965));
#72649=CARTESIAN_POINT('Ctrl Pts',(3.73621371845475,1.,-0.385670806454744));
#72650=CARTESIAN_POINT('Ctrl Pts',(3.74144965781088,1.,-0.386519576222036));
#72651=CARTESIAN_POINT('Ctrl Pts',(3.74792651696269,1.,-0.387663020050396));
#72652=CARTESIAN_POINT('Ctrl Pts',(3.75529302894757,1.,-0.389054775898251));
#72653=CARTESIAN_POINT('Ctrl Pts',(3.76315635032993,1.,-0.390642072979259));
#72654=CARTESIAN_POINT('Ctrl Pts',(3.77114011595892,1.,-0.392372786223347));
#72655=CARTESIAN_POINT('Ctrl Pts',(3.77894173114368,1.,-0.394202481011595));
#72656=CARTESIAN_POINT('Ctrl Pts',(3.78640521279479,1.,-0.396103205335029));
#72657=CARTESIAN_POINT('Ctrl Pts',(3.79352887163457,1.,-0.398064818684159));
#72658=CARTESIAN_POINT('Ctrl Pts',(3.80040370384659,1.,-0.400088346504727));
#72659=CARTESIAN_POINT('Ctrl Pts',(3.80716881962763,1.,-0.402181320148475));
#72660=CARTESIAN_POINT('Ctrl Pts',(3.81396374287762,1.,-0.404352694628237));
#72661=CARTESIAN_POINT('Ctrl Pts',(3.82087303913741,1.,-0.406607038258907));
#72662=CARTESIAN_POINT('Ctrl Pts',(3.82790724256397,1.,-0.408942371447377));
#72663=CARTESIAN_POINT('Ctrl Pts',(3.83503345578645,1.,-0.41135303879846));
#72664=CARTESIAN_POINT('Ctrl Pts',(3.84219403994742,1.,-0.413831367016727));
#72665=CARTESIAN_POINT('Ctrl Pts',(3.8493286415751,1.,-0.41636967805292));
#72666=CARTESIAN_POINT('Ctrl Pts',(3.85639825648031,1.,-0.41896246808681));
#72667=CARTESIAN_POINT('Ctrl Pts',(3.86339652542749,1.,-0.421607423177576));
#72668=CARTESIAN_POINT('Ctrl Pts',(3.87033643487882,1.,-0.424304173195143));
#72669=CARTESIAN_POINT('Ctrl Pts',(3.87724240306609,1.,-0.427053541173469));
#72670=CARTESIAN_POINT('Ctrl Pts',(3.88414070943334,1.,-0.429856640579734));
#72671=CARTESIAN_POINT('Ctrl Pts',(3.89104947940592,1.,-0.43271392954444));
#72672=CARTESIAN_POINT('Ctrl Pts',(3.8979725665544,1.,-0.435624629433506));
#72673=CARTESIAN_POINT('Ctrl Pts',(3.90490512938546,1.,-0.438587235458234));
#72674=CARTESIAN_POINT('Ctrl Pts',(3.91183704069146,1.,-0.441599824524048));
#72675=CARTESIAN_POINT('Ctrl Pts',(3.91875701610721,1.,-0.444660430230593));
#72676=CARTESIAN_POINT('Ctrl Pts',(3.92565674143424,1.,-0.447767416837297));
#72677=CARTESIAN_POINT('Ctrl Pts',(3.93253407403128,1.,-0.450919768356347));
#72678=CARTESIAN_POINT('Ctrl Pts',(3.93939080846298,1.,-0.454116879027576));
#72679=CARTESIAN_POINT('Ctrl Pts',(3.94623117206675,1.,-0.457358410451674));
#72680=CARTESIAN_POINT('Ctrl Pts',(3.95306005817363,1.,-0.460644124429119));
#72681=CARTESIAN_POINT('Ctrl Pts',(3.95988133243543,1.,-0.463973722115745));
#72682=CARTESIAN_POINT('Ctrl Pts',(3.96669622273946,1.,-0.467346690880672));
#72683=CARTESIAN_POINT('Ctrl Pts',(3.97350414289415,1.,-0.470762379613478));
#72684=CARTESIAN_POINT('Ctrl Pts',(3.9803033804443,1.,-0.474220061019542));
#72685=CARTESIAN_POINT('Ctrl Pts',(3.98709184306743,1.,-0.477718999122033));
#72686=CARTESIAN_POINT('Ctrl Pts',(3.99386775880655,1.,-0.481258512209638));
#72687=CARTESIAN_POINT('Ctrl Pts',(4.00063045119234,1.,-0.484838042421754));
#72688=CARTESIAN_POINT('Ctrl Pts',(4.0073800839092,1.,-0.488457130424531));
#72689=CARTESIAN_POINT('Ctrl Pts',(4.01411733503486,1.,-0.492115383417931));
#72690=CARTESIAN_POINT('Ctrl Pts',(4.02084308851813,1.,-0.495812444326223));
#72691=CARTESIAN_POINT('Ctrl Pts',(4.0275581398015,1.,-0.49954796234089));
#72692=CARTESIAN_POINT('Ctrl Pts',(4.0342628417439,1.,-0.503321556915514));
#72693=CARTESIAN_POINT('Ctrl Pts',(4.04095715149074,1.,-0.507132823288362));
#72694=CARTESIAN_POINT('Ctrl Pts',(4.04764078815591,1.,-0.510981349219174));
#72695=CARTESIAN_POINT('Ctrl Pts',(4.05431335771261,1.,-0.514866728193104));
#72696=CARTESIAN_POINT('Ctrl Pts',(4.06097448037934,1.,-0.51878857233681));
#72697=CARTESIAN_POINT('Ctrl Pts',(4.06762394471075,1.,-0.522746528602768));
#72698=CARTESIAN_POINT('Ctrl Pts',(4.07426172299496,1.,-0.526740277227));
#72699=CARTESIAN_POINT('Ctrl Pts',(4.08088789536488,1.,-0.530769518728076));
#72700=CARTESIAN_POINT('Ctrl Pts',(4.08750259988693,1.,-0.534833963477));
#72701=CARTESIAN_POINT('Ctrl Pts',(4.09410597627116,1.,-0.538933321179921));
#72702=CARTESIAN_POINT('Ctrl Pts',(4.10069810244473,1.,-0.543067286878457));
#72703=CARTESIAN_POINT('Ctrl Pts',(4.1072789702877,1.,-0.54723553948676));
#72704=CARTESIAN_POINT('Ctrl Pts',(4.11384852025578,1.,-0.551437758498247));
#72705=CARTESIAN_POINT('Ctrl Pts',(4.1204066619623,1.,-0.555673636130778));
#72706=CARTESIAN_POINT('Ctrl Pts',(4.12695329951859,1.,-0.559942890594628));
#72707=CARTESIAN_POINT('Ctrl Pts',(4.13348835726086,1.,-0.564245279535706));
#72708=CARTESIAN_POINT('Ctrl Pts',(4.14001179828669,1.,-0.568580610187116));
#72709=CARTESIAN_POINT('Ctrl Pts',(4.14652361065787,1.,-0.572948736066277));
#72710=CARTESIAN_POINT('Ctrl Pts',(4.1517237611974,1.,-0.576469391673917));
#72711=CARTESIAN_POINT('Ctrl Pts',(4.15561864787379,1.,-0.579124568912544));
#72712=CARTESIAN_POINT('Ctrl Pts',(4.15821291712391,1.,-0.580901211462913));
#72713=CARTESIAN_POINT('Ctrl Pts',(4.15950947128175,1.,-0.581791163835815));
#72714=CARTESIAN_POINT('Origin',(0.,0.,0.));
#72715=CARTESIAN_POINT('',(3.74449296982994,1.,-0.203156094897896));
#72716=CARTESIAN_POINT('Origin',(0.,1.,0.));
#72717=CARTESIAN_POINT('Ctrl Pts',(3.74449296982994,1.,-0.203156094897896));
#72718=CARTESIAN_POINT('Ctrl Pts',(3.74449296982994,0.666666666666667,-0.203156094897896));
#72719=CARTESIAN_POINT('Ctrl Pts',(3.74449296982994,0.333333333333333,-0.203156094897896));
#72720=CARTESIAN_POINT('Ctrl Pts',(3.74449296982994,-0.333333333333333,
-0.203156094897896));
#72721=CARTESIAN_POINT('Ctrl Pts',(3.74449296982994,-0.666666666666667,
-0.203156094897895));
#72722=CARTESIAN_POINT('Ctrl Pts',(3.74449296982994,-1.,-0.203156094897895));
#72723=CARTESIAN_POINT('Ctrl Pts',(3.74449849461127,-1.,0.20305423869972));
#72724=CARTESIAN_POINT('Ctrl Pts',(3.74449849461127,1.,0.20305423869972));
#72725=CARTESIAN_POINT('Ctrl Pts',(3.7444331934681,-1.,0.203111767587923));
#72726=CARTESIAN_POINT('Ctrl Pts',(3.7444331934681,1.,0.203111767587923));
#72727=CARTESIAN_POINT('Ctrl Pts',(3.7444688019622,-1.,0.203218215748058));
#72728=CARTESIAN_POINT('Ctrl Pts',(3.7444688019622,1.,0.203218215748058));
#72729=CARTESIAN_POINT('Ctrl Pts',(3.74502080927395,-1.,0.203352057956297));
#72730=CARTESIAN_POINT('Ctrl Pts',(3.74502080927395,1.,0.203352057956297));
#72731=CARTESIAN_POINT('Ctrl Pts',(3.7467547201908,-1.,0.203478844530446));
#72732=CARTESIAN_POINT('Ctrl Pts',(3.7467547201908,1.,0.203478844530446));
#72733=CARTESIAN_POINT('Ctrl Pts',(3.75054693397875,-1.,0.203550035479166));
#72734=CARTESIAN_POINT('Ctrl Pts',(3.75054693397875,1.,0.203550035479166));
#72735=CARTESIAN_POINT('Ctrl Pts',(3.75585118707734,-1.,0.203530796848321));
#72736=CARTESIAN_POINT('Ctrl Pts',(3.75585118707734,1.,0.203530796848321));
#72737=CARTESIAN_POINT('Ctrl Pts',(3.76242717936885,-1.,0.203414634707478));
#72738=CARTESIAN_POINT('Ctrl Pts',(3.76242717936885,1.,0.203414634707478));
#72739=CARTESIAN_POINT('Ctrl Pts',(3.7699207159487,-1.,0.203192390045164));
#72740=CARTESIAN_POINT('Ctrl Pts',(3.7699207159487,1.,0.203192390045164));
#72741=CARTESIAN_POINT('Ctrl Pts',(3.77793553476614,-1.,0.20285472969908));
#72742=CARTESIAN_POINT('Ctrl Pts',(3.77793553476614,1.,0.20285472969908));
#72743=CARTESIAN_POINT('Ctrl Pts',(3.78609175019242,-1.,0.20239426051216));
#72744=CARTESIAN_POINT('Ctrl Pts',(3.78609175019242,1.,0.20239426051216));
#72745=CARTESIAN_POINT('Ctrl Pts',(3.7940835418736,-1.,0.201807533800837));
#72746=CARTESIAN_POINT('Ctrl Pts',(3.7940835418736,1.,0.201807533800837));
#72747=CARTESIAN_POINT('Ctrl Pts',(3.80175247447337,-1.,0.201097756307325));
#72748=CARTESIAN_POINT('Ctrl Pts',(3.80175247447337,1.,0.201097756307325));
#72749=CARTESIAN_POINT('Ctrl Pts',(3.80909529318669,-1.,0.200274679433364));
#72750=CARTESIAN_POINT('Ctrl Pts',(3.80909529318669,1.,0.200274679433364));
#72751=CARTESIAN_POINT('Ctrl Pts',(3.81620203429815,-1.,0.199351525297447));
#72752=CARTESIAN_POINT('Ctrl Pts',(3.81620203429815,1.,0.199351525297447));
#72753=CARTESIAN_POINT('Ctrl Pts',(3.82321127349016,-1.,0.198342616900486));
#72754=CARTESIAN_POINT('Ctrl Pts',(3.82321127349016,1.,0.198342616900486));
#72755=CARTESIAN_POINT('Ctrl Pts',(3.83026221776456,-1.,0.197260935827361));
#72756=CARTESIAN_POINT('Ctrl Pts',(3.83026221776456,1.,0.197260935827361));
#72757=CARTESIAN_POINT('Ctrl Pts',(3.83743910616195,-1.,0.196115198971858));
#72758=CARTESIAN_POINT('Ctrl Pts',(3.83743910616195,1.,0.196115198971858));
#72759=CARTESIAN_POINT('Ctrl Pts',(3.84475203346977,-1.,0.19490900946022));
#72760=CARTESIAN_POINT('Ctrl Pts',(3.84475203346977,1.,0.19490900946022));
#72761=CARTESIAN_POINT('Ctrl Pts',(3.85216762263966,-1.,0.193642806777722));
#72762=CARTESIAN_POINT('Ctrl Pts',(3.85216762263966,1.,0.193642806777722));
#72763=CARTESIAN_POINT('Ctrl Pts',(3.85962774407633,-1.,0.19231515304497));
#72764=CARTESIAN_POINT('Ctrl Pts',(3.85962774407633,1.,0.19231515304497));
#72765=CARTESIAN_POINT('Ctrl Pts',(3.86707158624783,-1.,0.190924190418619));
#72766=CARTESIAN_POINT('Ctrl Pts',(3.86707158624783,1.,0.190924190418619));
#72767=CARTESIAN_POINT('Ctrl Pts',(3.87445976418412,-1.,0.189469253358272));
#72768=CARTESIAN_POINT('Ctrl Pts',(3.87445976418412,1.,0.189469253358272));
#72769=CARTESIAN_POINT('Ctrl Pts',(3.88178563496228,-1.,0.187951632512684));
#72770=CARTESIAN_POINT('Ctrl Pts',(3.88178563496228,1.,0.187951632512684));
#72771=CARTESIAN_POINT('Ctrl Pts',(3.88906196725848,-1.,0.18637372498528));
#72772=CARTESIAN_POINT('Ctrl Pts',(3.88906196725848,1.,0.18637372498528));
#72773=CARTESIAN_POINT('Ctrl Pts',(3.89631300742646,-1.,0.184738537728042));
#72774=CARTESIAN_POINT('Ctrl Pts',(3.89631300742646,1.,0.184738537728042));
#72775=CARTESIAN_POINT('Ctrl Pts',(3.90356488555132,-1.,0.18304908199319));
#72776=CARTESIAN_POINT('Ctrl Pts',(3.90356488555132,1.,0.18304908199319));
#72777=CARTESIAN_POINT('Ctrl Pts',(3.91083557557175,-1.,0.181307740731785));
#72778=CARTESIAN_POINT('Ctrl Pts',(3.91083557557175,1.,0.181307740731785));
#72779=CARTESIAN_POINT('Ctrl Pts',(3.91812876180926,-1.,0.179515885822881));
#72780=CARTESIAN_POINT('Ctrl Pts',(3.91812876180926,1.,0.179515885822881));
#72781=CARTESIAN_POINT('Ctrl Pts',(3.92543942697655,-1.,0.177674246152317));
#72782=CARTESIAN_POINT('Ctrl Pts',(3.92543942697655,1.,0.177674246152317));
#72783=CARTESIAN_POINT('Ctrl Pts',(3.93275726771042,-1.,0.175783136893867));
#72784=CARTESIAN_POINT('Ctrl Pts',(3.93275726771042,1.,0.175783136893867));
#72785=CARTESIAN_POINT('Ctrl Pts',(3.94007083096217,-1.,0.173842734974609));
#72786=CARTESIAN_POINT('Ctrl Pts',(3.94007083096217,1.,0.173842734974609));
#72787=CARTESIAN_POINT('Ctrl Pts',(3.94737164900868,-1.,0.17185335536924));
#72788=CARTESIAN_POINT('Ctrl Pts',(3.94737164900868,1.,0.17185335536924));
#72789=CARTESIAN_POINT('Ctrl Pts',(3.95465744665268,-1.,0.169815666374138));
#72790=CARTESIAN_POINT('Ctrl Pts',(3.95465744665268,1.,0.169815666374138));
#72791=CARTESIAN_POINT('Ctrl Pts',(3.96192990160296,-1.,0.167730547023319));
#72792=CARTESIAN_POINT('Ctrl Pts',(3.96192990160296,1.,0.167730547023319));
#72793=CARTESIAN_POINT('Ctrl Pts',(3.96919313621407,-1.,0.165598992851102));
#72794=CARTESIAN_POINT('Ctrl Pts',(3.96919313621407,1.,0.165598992851102));
#72795=CARTESIAN_POINT('Ctrl Pts',(3.97645194630943,-1.,0.163422004609999));
#72796=CARTESIAN_POINT('Ctrl Pts',(3.97645194630943,1.,0.163422004609999));
#72797=CARTESIAN_POINT('Ctrl Pts',(3.98371010319872,-1.,0.161200482186084));
#72798=CARTESIAN_POINT('Ctrl Pts',(3.98371010319872,1.,0.161200482186084));
#72799=CARTESIAN_POINT('Ctrl Pts',(3.99096873945878,-1.,0.158935123982793));
#72800=CARTESIAN_POINT('Ctrl Pts',(3.99096873945878,1.,0.158935123982793));
#72801=CARTESIAN_POINT('Ctrl Pts',(3.99822717425893,-1.,0.156626481393734));
#72802=CARTESIAN_POINT('Ctrl Pts',(3.99822717425893,1.,0.156626481393734));
#72803=CARTESIAN_POINT('Ctrl Pts',(4.00548360245319,-1.,0.15427500487231));
#72804=CARTESIAN_POINT('Ctrl Pts',(4.00548360245319,1.,0.15427500487231));
#72805=CARTESIAN_POINT('Ctrl Pts',(4.01273584234689,-1.,0.15188109402291));
#72806=CARTESIAN_POINT('Ctrl Pts',(4.01273584234689,1.,0.15188109402291));
#72807=CARTESIAN_POINT('Ctrl Pts',(4.01998203715564,-1.,0.149445144968706));
#72808=CARTESIAN_POINT('Ctrl Pts',(4.01998203715564,1.,0.149445144968706));
#72809=CARTESIAN_POINT('Ctrl Pts',(4.02722143146994,-1.,0.146967602878994));
#72810=CARTESIAN_POINT('Ctrl Pts',(4.02722143146994,1.,0.146967602878994));
#72811=CARTESIAN_POINT('Ctrl Pts',(4.03445411510333,-1.,0.144448947038344));
#72812=CARTESIAN_POINT('Ctrl Pts',(4.03445411510333,1.,0.144448947038344));
#72813=CARTESIAN_POINT('Ctrl Pts',(4.04168069633781,-1.,0.1418896714855));
#72814=CARTESIAN_POINT('Ctrl Pts',(4.04168069633781,1.,0.1418896714855));
#72815=CARTESIAN_POINT('Ctrl Pts',(4.04890199238036,-1.,0.139290267180057));
#72816=CARTESIAN_POINT('Ctrl Pts',(4.04890199238036,1.,0.139290267180057));
#72817=CARTESIAN_POINT('Ctrl Pts',(4.05611873400172,-1.,0.136651205046119));
#72818=CARTESIAN_POINT('Ctrl Pts',(4.05611873400172,1.,0.136651205046119));
#72819=CARTESIAN_POINT('Ctrl Pts',(4.06333121018596,-1.,0.133972916144244));
#72820=CARTESIAN_POINT('Ctrl Pts',(4.06333121018596,1.,0.133972916144244));
#72821=CARTESIAN_POINT('Ctrl Pts',(4.0705393152874,-1.,0.13125579354894));
#72822=CARTESIAN_POINT('Ctrl Pts',(4.0705393152874,1.,0.13125579354894));
#72823=CARTESIAN_POINT('Ctrl Pts',(4.07774270738954,-1.,0.128500200484837));
#72824=CARTESIAN_POINT('Ctrl Pts',(4.07774270738954,1.,0.128500200484837));
#72825=CARTESIAN_POINT('Ctrl Pts',(4.08494093372377,-1.,0.125706476822539));
#72826=CARTESIAN_POINT('Ctrl Pts',(4.08494093372377,1.,0.125706476822539));
#72827=CARTESIAN_POINT('Ctrl Pts',(4.09213355850756,-1.,0.122874946249106));
#72828=CARTESIAN_POINT('Ctrl Pts',(4.09213355850756,1.,0.122874946249106));
#72829=CARTESIAN_POINT('Ctrl Pts',(4.09932031767002,-1.,0.120005924388124));
#72830=CARTESIAN_POINT('Ctrl Pts',(4.09932031767002,1.,0.120005924388124));
#72831=CARTESIAN_POINT('Ctrl Pts',(4.10650113381833,-1.,0.117099722731648));
#72832=CARTESIAN_POINT('Ctrl Pts',(4.10650113381833,1.,0.117099722731648));
#72833=CARTESIAN_POINT('Ctrl Pts',(4.11367603924961,-1.,0.114156649609545));
#72834=CARTESIAN_POINT('Ctrl Pts',(4.11367603924961,1.,0.114156649609545));
#72835=CARTESIAN_POINT('Ctrl Pts',(4.1208451250225,-1.,0.111177012683346));
#72836=CARTESIAN_POINT('Ctrl Pts',(4.1208451250225,1.,0.111177012683346));
#72837=CARTESIAN_POINT('Ctrl Pts',(4.12800848371504,-1.,0.108161120528369));
#72838=CARTESIAN_POINT('Ctrl Pts',(4.12800848371504,1.,0.108161120528369));
#72839=CARTESIAN_POINT('Ctrl Pts',(4.13516614458895,-1.,0.105109286538945));
#72840=CARTESIAN_POINT('Ctrl Pts',(4.13516614458895,1.,0.105109286538945));
#72841=CARTESIAN_POINT('Ctrl Pts',(4.14231804939538,-1.,0.102021826577583));
#72842=CARTESIAN_POINT('Ctrl Pts',(4.14231804939538,1.,0.102021826577583));
#72843=CARTESIAN_POINT('Ctrl Pts',(4.14946408918485,-1.,0.0988990478901221));
#72844=CARTESIAN_POINT('Ctrl Pts',(4.14946408918485,1.,0.0988990478901221));
#72845=CARTESIAN_POINT('Ctrl Pts',(4.15660412653577,-1.,0.0957412403298002));
#72846=CARTESIAN_POINT('Ctrl Pts',(4.15660412653577,1.,0.0957412403298002));
#72847=CARTESIAN_POINT('Ctrl Pts',(4.16373802265839,-1.,0.0925486672167526));
#72848=CARTESIAN_POINT('Ctrl Pts',(4.16373802265839,1.,0.0925486672167526));
#72849=CARTESIAN_POINT('Ctrl Pts',(4.17086566490794,-1.,0.0893215560848644));
#72850=CARTESIAN_POINT('Ctrl Pts',(4.17086566490794,1.,0.0893215560848644));
#72851=CARTESIAN_POINT('Ctrl Pts',(4.17798698668094,-1.,0.0860600915549391));
#72852=CARTESIAN_POINT('Ctrl Pts',(4.17798698668094,1.,0.0860600915549391));
#72853=CARTESIAN_POINT('Ctrl Pts',(4.18510195327123,-1.,0.0827644164385674));
#72854=CARTESIAN_POINT('Ctrl Pts',(4.18510195327123,1.,0.0827644164385674));
#72855=CARTESIAN_POINT('Ctrl Pts',(4.19078883320504,-1.,0.0801005887114315));
#72856=CARTESIAN_POINT('Ctrl Pts',(4.19078883320504,1.,0.0801005887114315));
#72857=CARTESIAN_POINT('Ctrl Pts',(4.19505112859416,-1.,0.0780873956242392));
#72858=CARTESIAN_POINT('Ctrl Pts',(4.19505112859416,1.,0.0780873956242392));
#72859=CARTESIAN_POINT('Ctrl Pts',(4.1978913862118,-1.,0.0767384596141459));
#72860=CARTESIAN_POINT('Ctrl Pts',(4.1978913862118,1.,0.0767384596141459));
#72861=CARTESIAN_POINT('Ctrl Pts',(4.19931119685982,-1.,0.0760622897878241));
#72862=CARTESIAN_POINT('Ctrl Pts',(4.19931119685982,1.,0.0760622897878241));
#72863=CARTESIAN_POINT('',(3.74449296983004,1.,0.2031560948961));
#72864=CARTESIAN_POINT('Ctrl Pts',(3.74449296983004,-1.,0.2031560948961));
#72865=CARTESIAN_POINT('Ctrl Pts',(3.74449296983004,-0.666666666666667,
0.2031560948961));
#72866=CARTESIAN_POINT('Ctrl Pts',(3.74449296983004,-0.333333333333333,
0.2031560948961));
#72867=CARTESIAN_POINT('Ctrl Pts',(3.74449296983004,0.333333333333333,0.2031560948961));
#72868=CARTESIAN_POINT('Ctrl Pts',(3.74449296983004,0.666666666666667,0.2031560948961));
#72869=CARTESIAN_POINT('Ctrl Pts',(3.74449296983004,1.,0.2031560948961));
#72870=CARTESIAN_POINT('',(4.19931119685982,1.,0.0760622897878241));
#72871=CARTESIAN_POINT('',(4.19931119685982,0.,0.0760622897878241));
#72872=CARTESIAN_POINT('Ctrl Pts',(3.74449296983004,1.,0.2031560948961));
#72873=CARTESIAN_POINT('Ctrl Pts',(3.74453008995092,1.,0.203188003946656));
#72874=CARTESIAN_POINT('Ctrl Pts',(3.74471097893845,1.,0.20326661011053));
#72875=CARTESIAN_POINT('Ctrl Pts',(3.74535749969115,1.,0.203375226874121));
#72876=CARTESIAN_POINT('Ctrl Pts',(3.74703926501752,1.,0.203484186269415));
#72877=CARTESIAN_POINT('Ctrl Pts',(3.75054693397875,1.,0.203550035479166));
#72878=CARTESIAN_POINT('Ctrl Pts',(3.75585118707734,1.,0.203530796848321));
#72879=CARTESIAN_POINT('Ctrl Pts',(3.76242717936885,1.,0.203414634707478));
#72880=CARTESIAN_POINT('Ctrl Pts',(3.7699207159487,1.,0.203192390045164));
#72881=CARTESIAN_POINT('Ctrl Pts',(3.77793553476614,1.,0.20285472969908));
#72882=CARTESIAN_POINT('Ctrl Pts',(3.78609175019242,1.,0.20239426051216));
#72883=CARTESIAN_POINT('Ctrl Pts',(3.7940835418736,1.,0.201807533800837));
#72884=CARTESIAN_POINT('Ctrl Pts',(3.80175247447337,1.,0.201097756307325));
#72885=CARTESIAN_POINT('Ctrl Pts',(3.80909529318669,1.,0.200274679433364));
#72886=CARTESIAN_POINT('Ctrl Pts',(3.81620203429815,1.,0.199351525297447));
#72887=CARTESIAN_POINT('Ctrl Pts',(3.82321127349016,1.,0.198342616900486));
#72888=CARTESIAN_POINT('Ctrl Pts',(3.83026221776456,1.,0.197260935827361));
#72889=CARTESIAN_POINT('Ctrl Pts',(3.83743910616195,1.,0.196115198971858));
#72890=CARTESIAN_POINT('Ctrl Pts',(3.84475203346977,1.,0.19490900946022));
#72891=CARTESIAN_POINT('Ctrl Pts',(3.85216762263966,1.,0.193642806777722));
#72892=CARTESIAN_POINT('Ctrl Pts',(3.85962774407633,1.,0.19231515304497));
#72893=CARTESIAN_POINT('Ctrl Pts',(3.86707158624783,1.,0.190924190418619));
#72894=CARTESIAN_POINT('Ctrl Pts',(3.87445976418412,1.,0.189469253358272));
#72895=CARTESIAN_POINT('Ctrl Pts',(3.88178563496228,1.,0.187951632512684));
#72896=CARTESIAN_POINT('Ctrl Pts',(3.88906196725848,1.,0.18637372498528));
#72897=CARTESIAN_POINT('Ctrl Pts',(3.89631300742646,1.,0.184738537728042));
#72898=CARTESIAN_POINT('Ctrl Pts',(3.90356488555132,1.,0.18304908199319));
#72899=CARTESIAN_POINT('Ctrl Pts',(3.91083557557175,1.,0.181307740731785));
#72900=CARTESIAN_POINT('Ctrl Pts',(3.91812876180926,1.,0.179515885822881));
#72901=CARTESIAN_POINT('Ctrl Pts',(3.92543942697655,1.,0.177674246152317));
#72902=CARTESIAN_POINT('Ctrl Pts',(3.93275726771042,1.,0.175783136893867));
#72903=CARTESIAN_POINT('Ctrl Pts',(3.94007083096217,1.,0.173842734974609));
#72904=CARTESIAN_POINT('Ctrl Pts',(3.94737164900868,1.,0.17185335536924));
#72905=CARTESIAN_POINT('Ctrl Pts',(3.95465744665268,1.,0.169815666374138));
#72906=CARTESIAN_POINT('Ctrl Pts',(3.96192990160296,1.,0.167730547023319));
#72907=CARTESIAN_POINT('Ctrl Pts',(3.96919313621407,1.,0.165598992851102));
#72908=CARTESIAN_POINT('Ctrl Pts',(3.97645194630943,1.,0.163422004609999));
#72909=CARTESIAN_POINT('Ctrl Pts',(3.98371010319872,1.,0.161200482186084));
#72910=CARTESIAN_POINT('Ctrl Pts',(3.99096873945878,1.,0.158935123982793));
#72911=CARTESIAN_POINT('Ctrl Pts',(3.99822717425893,1.,0.156626481393734));
#72912=CARTESIAN_POINT('Ctrl Pts',(4.00548360245319,1.,0.15427500487231));
#72913=CARTESIAN_POINT('Ctrl Pts',(4.01273584234689,1.,0.15188109402291));
#72914=CARTESIAN_POINT('Ctrl Pts',(4.01998203715564,1.,0.149445144968706));
#72915=CARTESIAN_POINT('Ctrl Pts',(4.02722143146994,1.,0.146967602878994));
#72916=CARTESIAN_POINT('Ctrl Pts',(4.03445411510333,1.,0.144448947038344));
#72917=CARTESIAN_POINT('Ctrl Pts',(4.04168069633781,1.,0.1418896714855));
#72918=CARTESIAN_POINT('Ctrl Pts',(4.04890199238036,1.,0.139290267180057));
#72919=CARTESIAN_POINT('Ctrl Pts',(4.05611873400172,1.,0.136651205046119));
#72920=CARTESIAN_POINT('Ctrl Pts',(4.06333121018596,1.,0.133972916144244));
#72921=CARTESIAN_POINT('Ctrl Pts',(4.0705393152874,1.,0.13125579354894));
#72922=CARTESIAN_POINT('Ctrl Pts',(4.07774270738954,1.,0.128500200484837));
#72923=CARTESIAN_POINT('Ctrl Pts',(4.08494093372377,1.,0.125706476822539));
#72924=CARTESIAN_POINT('Ctrl Pts',(4.09213355850756,1.,0.122874946249106));
#72925=CARTESIAN_POINT('Ctrl Pts',(4.09932031767002,1.,0.120005924388124));
#72926=CARTESIAN_POINT('Ctrl Pts',(4.10650113381833,1.,0.117099722731648));
#72927=CARTESIAN_POINT('Ctrl Pts',(4.11367603924961,1.,0.114156649609545));
#72928=CARTESIAN_POINT('Ctrl Pts',(4.1208451250225,1.,0.111177012683346));
#72929=CARTESIAN_POINT('Ctrl Pts',(4.12800848371504,1.,0.108161120528369));
#72930=CARTESIAN_POINT('Ctrl Pts',(4.13516614458895,1.,0.105109286538945));
#72931=CARTESIAN_POINT('Ctrl Pts',(4.14231804939538,1.,0.102021826577583));
#72932=CARTESIAN_POINT('Ctrl Pts',(4.14946408918485,1.,0.0988990478901221));
#72933=CARTESIAN_POINT('Ctrl Pts',(4.15660412653577,1.,0.0957412403298002));
#72934=CARTESIAN_POINT('Ctrl Pts',(4.16373802265839,1.,0.0925486672167526));
#72935=CARTESIAN_POINT('Ctrl Pts',(4.17086566490794,1.,0.0893215560848644));
#72936=CARTESIAN_POINT('Ctrl Pts',(4.17798698668094,1.,0.0860600915549391));
#72937=CARTESIAN_POINT('Ctrl Pts',(4.18510195327123,1.,0.0827644164385674));
#72938=CARTESIAN_POINT('Ctrl Pts',(4.19078883320504,1.,0.0801005887114315));
#72939=CARTESIAN_POINT('Ctrl Pts',(4.19505112859416,1.,0.0780873956242392));
#72940=CARTESIAN_POINT('Ctrl Pts',(4.1978913862118,1.,0.0767384596141459));
#72941=CARTESIAN_POINT('Ctrl Pts',(4.19931119685982,1.,0.0760622897878241));
#72942=CARTESIAN_POINT('Ctrl Pts',(4.19931119685982,-1.,-0.0760622897878241));
#72943=CARTESIAN_POINT('Ctrl Pts',(4.19931119685982,1.,-0.0760622897878241));
#72944=CARTESIAN_POINT('Ctrl Pts',(4.19789138621624,-1.,-0.07673845961422));
#72945=CARTESIAN_POINT('Ctrl Pts',(4.19789138621624,1.,-0.07673845961422));
#72946=CARTESIAN_POINT('Ctrl Pts',(4.19505112860624,-1.,-0.0780873956244407));
#72947=CARTESIAN_POINT('Ctrl Pts',(4.19505112860624,1.,-0.0780873956244407));
#72948=CARTESIAN_POINT('Ctrl Pts',(4.19078883322483,-1.,-0.0801005887117608));
#72949=CARTESIAN_POINT('Ctrl Pts',(4.19078883322483,1.,-0.0801005887117608));
#72950=CARTESIAN_POINT('Ctrl Pts',(4.1851019532944,-1.,-0.0827644164389515));
#72951=CARTESIAN_POINT('Ctrl Pts',(4.1851019532944,1.,-0.0827644164389515));
#72952=CARTESIAN_POINT('Ctrl Pts',(4.17798698669991,-1.,-0.086060091555252));
#72953=CARTESIAN_POINT('Ctrl Pts',(4.17798698669991,1.,-0.086060091555252));
#72954=CARTESIAN_POINT('Ctrl Pts',(4.17086566491823,-1.,-0.0893215560850332));
#72955=CARTESIAN_POINT('Ctrl Pts',(4.17086566491823,1.,-0.0893215560850332));
#72956=CARTESIAN_POINT('Ctrl Pts',(4.16373802265942,-1.,-0.0925486672167695));
#72957=CARTESIAN_POINT('Ctrl Pts',(4.16373802265942,1.,-0.0925486672167695));
#72958=CARTESIAN_POINT('Ctrl Pts',(4.15660412653006,-1.,-0.0957412403297072));
#72959=CARTESIAN_POINT('Ctrl Pts',(4.15660412653006,1.,-0.0957412403297072));
#72960=CARTESIAN_POINT('Ctrl Pts',(4.1494640891762,-1.,-0.0988990478899816));
#72961=CARTESIAN_POINT('Ctrl Pts',(4.1494640891762,1.,-0.0988990478899816));
#72962=CARTESIAN_POINT('Ctrl Pts',(4.14231804938737,-1.,-0.102021826577454));
#72963=CARTESIAN_POINT('Ctrl Pts',(4.14231804938737,1.,-0.102021826577454));
#72964=CARTESIAN_POINT('Ctrl Pts',(4.13516614458396,-1.,-0.105109286538864));
#72965=CARTESIAN_POINT('Ctrl Pts',(4.13516614458396,1.,-0.105109286538864));
#72966=CARTESIAN_POINT('Ctrl Pts',(4.12800848371386,-1.,-0.10816112052835));
#72967=CARTESIAN_POINT('Ctrl Pts',(4.12800848371386,1.,-0.10816112052835));
#72968=CARTESIAN_POINT('Ctrl Pts',(4.12084512502444,-1.,-0.111177012683378));
#72969=CARTESIAN_POINT('Ctrl Pts',(4.12084512502444,1.,-0.111177012683378));
#72970=CARTESIAN_POINT('Ctrl Pts',(4.11367603925313,-1.,-0.114156649609602));
#72971=CARTESIAN_POINT('Ctrl Pts',(4.11367603925313,1.,-0.114156649609602));
#72972=CARTESIAN_POINT('Ctrl Pts',(4.10650113382187,-1.,-0.117099722731705));
#72973=CARTESIAN_POINT('Ctrl Pts',(4.10650113382187,1.,-0.117099722731705));
#72974=CARTESIAN_POINT('Ctrl Pts',(4.09932031767243,-1.,-0.120005924388162));
#72975=CARTESIAN_POINT('Ctrl Pts',(4.09932031767243,1.,-0.120005924388162));
#72976=CARTESIAN_POINT('Ctrl Pts',(4.09213355850836,-1.,-0.122874946249119));
#72977=CARTESIAN_POINT('Ctrl Pts',(4.09213355850836,1.,-0.122874946249119));
#72978=CARTESIAN_POINT('Ctrl Pts',(4.08494093372315,-1.,-0.12570647682253));
#72979=CARTESIAN_POINT('Ctrl Pts',(4.08494093372315,1.,-0.12570647682253));
#72980=CARTESIAN_POINT('Ctrl Pts',(4.07774270738809,-1.,-0.128500200484814));
#72981=CARTESIAN_POINT('Ctrl Pts',(4.07774270738809,1.,-0.128500200484814));
#72982=CARTESIAN_POINT('Ctrl Pts',(4.07053931528579,-1.,-0.131255793548914));
#72983=CARTESIAN_POINT('Ctrl Pts',(4.07053931528579,1.,-0.131255793548914));
#72984=CARTESIAN_POINT('Ctrl Pts',(4.06333121018476,-1.,-0.133972916144225));
#72985=CARTESIAN_POINT('Ctrl Pts',(4.06333121018476,1.,-0.133972916144225));
#72986=CARTESIAN_POINT('Ctrl Pts',(4.05611873400122,-1.,-0.136651205046111));
#72987=CARTESIAN_POINT('Ctrl Pts',(4.05611873400122,1.,-0.136651205046111));
#72988=CARTESIAN_POINT('Ctrl Pts',(4.04890199238056,-1.,-0.13929026718006));
#72989=CARTESIAN_POINT('Ctrl Pts',(4.04890199238056,1.,-0.13929026718006));
#72990=CARTESIAN_POINT('Ctrl Pts',(4.04168069633842,-1.,-0.141889671485508));
#72991=CARTESIAN_POINT('Ctrl Pts',(4.04168069633842,1.,-0.141889671485508));
#72992=CARTESIAN_POINT('Ctrl Pts',(4.03445411510403,-1.,-0.144448947038352));
#72993=CARTESIAN_POINT('Ctrl Pts',(4.03445411510403,1.,-0.144448947038352));
#72994=CARTESIAN_POINT('Ctrl Pts',(4.02722143147048,-1.,-0.146967602878999));
#72995=CARTESIAN_POINT('Ctrl Pts',(4.02722143147048,1.,-0.146967602878999));
#72996=CARTESIAN_POINT('Ctrl Pts',(4.01998203715588,-1.,-0.149445144968708));
#72997=CARTESIAN_POINT('Ctrl Pts',(4.01998203715588,1.,-0.149445144968708));
#72998=CARTESIAN_POINT('Ctrl Pts',(4.01273584234684,-1.,-0.151881094022909));
#72999=CARTESIAN_POINT('Ctrl Pts',(4.01273584234684,1.,-0.151881094022909));
#73000=CARTESIAN_POINT('Ctrl Pts',(4.00548360245297,-1.,-0.15427500487231));
#73001=CARTESIAN_POINT('Ctrl Pts',(4.00548360245297,1.,-0.15427500487231));
#73002=CARTESIAN_POINT('Ctrl Pts',(3.99822717425869,-1.,-0.156626481393736));
#73003=CARTESIAN_POINT('Ctrl Pts',(3.99822717425869,1.,-0.156626481393736));
#73004=CARTESIAN_POINT('Ctrl Pts',(3.99096873945862,-1.,-0.158935123982796));
#73005=CARTESIAN_POINT('Ctrl Pts',(3.99096873945862,1.,-0.158935123982796));
#73006=CARTESIAN_POINT('Ctrl Pts',(3.98371010319866,-1.,-0.161200482186088));
#73007=CARTESIAN_POINT('Ctrl Pts',(3.98371010319866,1.,-0.161200482186088));
#73008=CARTESIAN_POINT('Ctrl Pts',(3.97645194630944,-1.,-0.163422004609999));
#73009=CARTESIAN_POINT('Ctrl Pts',(3.97645194630944,1.,-0.163422004609999));
#73010=CARTESIAN_POINT('Ctrl Pts',(3.9691931362141,-1.,-0.165598992851098));
#73011=CARTESIAN_POINT('Ctrl Pts',(3.9691931362141,1.,-0.165598992851098));
#73012=CARTESIAN_POINT('Ctrl Pts',(3.96192990160296,-1.,-0.167730547023312));
#73013=CARTESIAN_POINT('Ctrl Pts',(3.96192990160296,1.,-0.167730547023312));
#73014=CARTESIAN_POINT('Ctrl Pts',(3.95465744665263,-1.,-0.16981566637413));
#73015=CARTESIAN_POINT('Ctrl Pts',(3.95465744665263,1.,-0.16981566637413));
#73016=CARTESIAN_POINT('Ctrl Pts',(3.94737164900861,-1.,-0.171853355369233));
#73017=CARTESIAN_POINT('Ctrl Pts',(3.94737164900861,1.,-0.171853355369233));
#73018=CARTESIAN_POINT('Ctrl Pts',(3.94007083096214,-1.,-0.173842734974608));
#73019=CARTESIAN_POINT('Ctrl Pts',(3.94007083096214,1.,-0.173842734974608));
#73020=CARTESIAN_POINT('Ctrl Pts',(3.93275726771049,-1.,-0.175783136893873));
#73021=CARTESIAN_POINT('Ctrl Pts',(3.93275726771049,1.,-0.175783136893873));
#73022=CARTESIAN_POINT('Ctrl Pts',(3.92543942697672,-1.,-0.177674246152328));
#73023=CARTESIAN_POINT('Ctrl Pts',(3.92543942697672,1.,-0.177674246152328));
#73024=CARTESIAN_POINT('Ctrl Pts',(3.91812876180948,-1.,-0.179515885822895));
#73025=CARTESIAN_POINT('Ctrl Pts',(3.91812876180948,1.,-0.179515885822895));
#73026=CARTESIAN_POINT('Ctrl Pts',(3.91083557557193,-1.,-0.181307740731796));
#73027=CARTESIAN_POINT('Ctrl Pts',(3.91083557557193,1.,-0.181307740731796));
#73028=CARTESIAN_POINT('Ctrl Pts',(3.90356488555138,-1.,-0.183049081993193));
#73029=CARTESIAN_POINT('Ctrl Pts',(3.90356488555138,1.,-0.183049081993193));
#73030=CARTESIAN_POINT('Ctrl Pts',(3.89631300742633,-1.,-0.184738537728035));
#73031=CARTESIAN_POINT('Ctrl Pts',(3.89631300742633,1.,-0.184738537728035));
#73032=CARTESIAN_POINT('Ctrl Pts',(3.88906196725817,-1.,-0.186373724985263));
#73033=CARTESIAN_POINT('Ctrl Pts',(3.88906196725817,1.,-0.186373724985263));
#73034=CARTESIAN_POINT('Ctrl Pts',(3.88178563496187,-1.,-0.187951632512664));
#73035=CARTESIAN_POINT('Ctrl Pts',(3.88178563496187,1.,-0.187951632512664));
#73036=CARTESIAN_POINT('Ctrl Pts',(3.87445976418377,-1.,-0.189469253358255));
#73037=CARTESIAN_POINT('Ctrl Pts',(3.87445976418377,1.,-0.189469253358255));
#73038=CARTESIAN_POINT('Ctrl Pts',(3.8670715862477,-1.,-0.190924190418613));
#73039=CARTESIAN_POINT('Ctrl Pts',(3.8670715862477,1.,-0.190924190418613));
#73040=CARTESIAN_POINT('Ctrl Pts',(3.85962774407652,-1.,-0.19231515304498));
#73041=CARTESIAN_POINT('Ctrl Pts',(3.85962774407652,1.,-0.19231515304498));
#73042=CARTESIAN_POINT('Ctrl Pts',(3.85216762264019,-1.,-0.193642806777748));
#73043=CARTESIAN_POINT('Ctrl Pts',(3.85216762264019,1.,-0.193642806777748));
#73044=CARTESIAN_POINT('Ctrl Pts',(3.84475203347052,-1.,-0.194909009460255));
#73045=CARTESIAN_POINT('Ctrl Pts',(3.84475203347052,1.,-0.194909009460255));
#73046=CARTESIAN_POINT('Ctrl Pts',(3.83743910616265,-1.,-0.19611519897189));
#73047=CARTESIAN_POINT('Ctrl Pts',(3.83743910616265,1.,-0.19611519897189));
#73048=CARTESIAN_POINT('Ctrl Pts',(3.83026221776488,-1.,-0.197260935827375));
#73049=CARTESIAN_POINT('Ctrl Pts',(3.83026221776488,1.,-0.197260935827375));
#73050=CARTESIAN_POINT('Ctrl Pts',(3.82321127348981,-1.,-0.19834261690047));
#73051=CARTESIAN_POINT('Ctrl Pts',(3.82321127348981,1.,-0.19834261690047));
#73052=CARTESIAN_POINT('Ctrl Pts',(3.81620203429702,-1.,-0.199351525297397));
#73053=CARTESIAN_POINT('Ctrl Pts',(3.81620203429702,1.,-0.199351525297397));
#73054=CARTESIAN_POINT('Ctrl Pts',(3.80909529318501,-1.,-0.20027467943329));
#73055=CARTESIAN_POINT('Ctrl Pts',(3.80909529318501,1.,-0.20027467943329));
#73056=CARTESIAN_POINT('Ctrl Pts',(3.80175247447171,-1.,-0.201097756307252));
#73057=CARTESIAN_POINT('Ctrl Pts',(3.80175247447171,1.,-0.201097756307252));
#73058=CARTESIAN_POINT('Ctrl Pts',(3.79408354187274,-1.,-0.201807533800799));
#73059=CARTESIAN_POINT('Ctrl Pts',(3.79408354187274,1.,-0.201807533800799));
#73060=CARTESIAN_POINT('Ctrl Pts',(3.78609175019317,-1.,-0.202394260512193));
#73061=CARTESIAN_POINT('Ctrl Pts',(3.78609175019317,1.,-0.202394260512193));
#73062=CARTESIAN_POINT('Ctrl Pts',(3.77793553476879,-1.,-0.202854729699197));
#73063=CARTESIAN_POINT('Ctrl Pts',(3.77793553476879,1.,-0.202854729699197));
#73064=CARTESIAN_POINT('Ctrl Pts',(3.76992071595267,-1.,-0.203192390045338));
#73065=CARTESIAN_POINT('Ctrl Pts',(3.76992071595267,1.,-0.203192390045338));
#73066=CARTESIAN_POINT('Ctrl Pts',(3.76242717937273,-1.,-0.203414634707647));
#73067=CARTESIAN_POINT('Ctrl Pts',(3.76242717937273,1.,-0.203414634707647));
#73068=CARTESIAN_POINT('Ctrl Pts',(3.75585118707924,-1.,-0.203530796848404));
#73069=CARTESIAN_POINT('Ctrl Pts',(3.75585118707924,1.,-0.203530796848404));
#73070=CARTESIAN_POINT('Ctrl Pts',(3.75054693397716,-1.,-0.203550035479097));
#73071=CARTESIAN_POINT('Ctrl Pts',(3.75054693397716,1.,-0.203550035479097));
#73072=CARTESIAN_POINT('Ctrl Pts',(3.74675472018582,-1.,-0.20347884453023));
#73073=CARTESIAN_POINT('Ctrl Pts',(3.74675472018582,1.,-0.20347884453023));
#73074=CARTESIAN_POINT('Ctrl Pts',(3.7450208092684,-1.,-0.203352057956056));
#73075=CARTESIAN_POINT('Ctrl Pts',(3.7450208092684,1.,-0.203352057956056));
#73076=CARTESIAN_POINT('Ctrl Pts',(3.74446880195845,-1.,-0.203218215747895));
#73077=CARTESIAN_POINT('Ctrl Pts',(3.74446880195845,1.,-0.203218215747895));
#73078=CARTESIAN_POINT('Ctrl Pts',(3.74443319346666,-1.,-0.20311176758786));
#73079=CARTESIAN_POINT('Ctrl Pts',(3.74443319346666,1.,-0.20311176758786));
#73080=CARTESIAN_POINT('Ctrl Pts',(3.74449849461127,-1.,-0.20305423869972));
#73081=CARTESIAN_POINT('Ctrl Pts',(3.74449849461127,1.,-0.20305423869972));
#73082=CARTESIAN_POINT('',(4.19931119685982,1.,-0.0760622897878241));
#73083=CARTESIAN_POINT('Ctrl Pts',(4.19931119685982,1.,-0.0760622897878241));
#73084=CARTESIAN_POINT('Ctrl Pts',(4.19789138621624,1.,-0.07673845961422));
#73085=CARTESIAN_POINT('Ctrl Pts',(4.19505112860624,1.,-0.0780873956244407));
#73086=CARTESIAN_POINT('Ctrl Pts',(4.19078883322483,1.,-0.0801005887117608));
#73087=CARTESIAN_POINT('Ctrl Pts',(4.1851019532944,1.,-0.0827644164389515));
#73088=CARTESIAN_POINT('Ctrl Pts',(4.17798698669991,1.,-0.086060091555252));
#73089=CARTESIAN_POINT('Ctrl Pts',(4.17086566491823,1.,-0.0893215560850332));
#73090=CARTESIAN_POINT('Ctrl Pts',(4.16373802265942,1.,-0.0925486672167695));
#73091=CARTESIAN_POINT('Ctrl Pts',(4.15660412653006,1.,-0.0957412403297072));
#73092=CARTESIAN_POINT('Ctrl Pts',(4.1494640891762,1.,-0.0988990478899816));
#73093=CARTESIAN_POINT('Ctrl Pts',(4.14231804938737,1.,-0.102021826577454));
#73094=CARTESIAN_POINT('Ctrl Pts',(4.13516614458396,1.,-0.105109286538864));
#73095=CARTESIAN_POINT('Ctrl Pts',(4.12800848371386,1.,-0.10816112052835));
#73096=CARTESIAN_POINT('Ctrl Pts',(4.12084512502444,1.,-0.111177012683378));
#73097=CARTESIAN_POINT('Ctrl Pts',(4.11367603925313,1.,-0.114156649609602));
#73098=CARTESIAN_POINT('Ctrl Pts',(4.10650113382187,1.,-0.117099722731705));
#73099=CARTESIAN_POINT('Ctrl Pts',(4.09932031767243,1.,-0.120005924388162));
#73100=CARTESIAN_POINT('Ctrl Pts',(4.09213355850836,1.,-0.122874946249119));
#73101=CARTESIAN_POINT('Ctrl Pts',(4.08494093372315,1.,-0.12570647682253));
#73102=CARTESIAN_POINT('Ctrl Pts',(4.07774270738809,1.,-0.128500200484814));
#73103=CARTESIAN_POINT('Ctrl Pts',(4.07053931528579,1.,-0.131255793548914));
#73104=CARTESIAN_POINT('Ctrl Pts',(4.06333121018476,1.,-0.133972916144225));
#73105=CARTESIAN_POINT('Ctrl Pts',(4.05611873400122,1.,-0.136651205046111));
#73106=CARTESIAN_POINT('Ctrl Pts',(4.04890199238056,1.,-0.13929026718006));
#73107=CARTESIAN_POINT('Ctrl Pts',(4.04168069633842,1.,-0.141889671485508));
#73108=CARTESIAN_POINT('Ctrl Pts',(4.03445411510403,1.,-0.144448947038352));
#73109=CARTESIAN_POINT('Ctrl Pts',(4.02722143147048,1.,-0.146967602878999));
#73110=CARTESIAN_POINT('Ctrl Pts',(4.01998203715588,1.,-0.149445144968708));
#73111=CARTESIAN_POINT('Ctrl Pts',(4.01273584234684,1.,-0.151881094022909));
#73112=CARTESIAN_POINT('Ctrl Pts',(4.00548360245297,1.,-0.15427500487231));
#73113=CARTESIAN_POINT('Ctrl Pts',(3.99822717425869,1.,-0.156626481393736));
#73114=CARTESIAN_POINT('Ctrl Pts',(3.99096873945862,1.,-0.158935123982796));
#73115=CARTESIAN_POINT('Ctrl Pts',(3.98371010319866,1.,-0.161200482186088));
#73116=CARTESIAN_POINT('Ctrl Pts',(3.97645194630944,1.,-0.163422004609999));
#73117=CARTESIAN_POINT('Ctrl Pts',(3.9691931362141,1.,-0.165598992851098));
#73118=CARTESIAN_POINT('Ctrl Pts',(3.96192990160296,1.,-0.167730547023312));
#73119=CARTESIAN_POINT('Ctrl Pts',(3.95465744665263,1.,-0.16981566637413));
#73120=CARTESIAN_POINT('Ctrl Pts',(3.94737164900861,1.,-0.171853355369233));
#73121=CARTESIAN_POINT('Ctrl Pts',(3.94007083096214,1.,-0.173842734974608));
#73122=CARTESIAN_POINT('Ctrl Pts',(3.93275726771049,1.,-0.175783136893873));
#73123=CARTESIAN_POINT('Ctrl Pts',(3.92543942697672,1.,-0.177674246152328));
#73124=CARTESIAN_POINT('Ctrl Pts',(3.91812876180948,1.,-0.179515885822895));
#73125=CARTESIAN_POINT('Ctrl Pts',(3.91083557557193,1.,-0.181307740731796));
#73126=CARTESIAN_POINT('Ctrl Pts',(3.90356488555138,1.,-0.183049081993193));
#73127=CARTESIAN_POINT('Ctrl Pts',(3.89631300742633,1.,-0.184738537728035));
#73128=CARTESIAN_POINT('Ctrl Pts',(3.88906196725817,1.,-0.186373724985263));
#73129=CARTESIAN_POINT('Ctrl Pts',(3.88178563496187,1.,-0.187951632512664));
#73130=CARTESIAN_POINT('Ctrl Pts',(3.87445976418377,1.,-0.189469253358255));
#73131=CARTESIAN_POINT('Ctrl Pts',(3.8670715862477,1.,-0.190924190418613));
#73132=CARTESIAN_POINT('Ctrl Pts',(3.85962774407652,1.,-0.19231515304498));
#73133=CARTESIAN_POINT('Ctrl Pts',(3.85216762264019,1.,-0.193642806777748));
#73134=CARTESIAN_POINT('Ctrl Pts',(3.84475203347052,1.,-0.194909009460255));
#73135=CARTESIAN_POINT('Ctrl Pts',(3.83743910616265,1.,-0.19611519897189));
#73136=CARTESIAN_POINT('Ctrl Pts',(3.83026221776488,1.,-0.197260935827375));
#73137=CARTESIAN_POINT('Ctrl Pts',(3.82321127348981,1.,-0.19834261690047));
#73138=CARTESIAN_POINT('Ctrl Pts',(3.81620203429702,1.,-0.199351525297397));
#73139=CARTESIAN_POINT('Ctrl Pts',(3.80909529318501,1.,-0.20027467943329));
#73140=CARTESIAN_POINT('Ctrl Pts',(3.80175247447171,1.,-0.201097756307252));
#73141=CARTESIAN_POINT('Ctrl Pts',(3.79408354187274,1.,-0.201807533800799));
#73142=CARTESIAN_POINT('Ctrl Pts',(3.78609175019317,1.,-0.202394260512193));
#73143=CARTESIAN_POINT('Ctrl Pts',(3.77793553476879,1.,-0.202854729699197));
#73144=CARTESIAN_POINT('Ctrl Pts',(3.76992071595267,1.,-0.203192390045338));
#73145=CARTESIAN_POINT('Ctrl Pts',(3.76242717937273,1.,-0.203414634707647));
#73146=CARTESIAN_POINT('Ctrl Pts',(3.75585118707924,1.,-0.203530796848404));
#73147=CARTESIAN_POINT('Ctrl Pts',(3.75054693397716,1.,-0.203550035479097));
#73148=CARTESIAN_POINT('Ctrl Pts',(3.74703926501843,1.,-0.203484186269315));
#73149=CARTESIAN_POINT('Ctrl Pts',(3.74535749969262,1.,-0.203375226874332));
#73150=CARTESIAN_POINT('Ctrl Pts',(3.74471097893961,1.,-0.203266610111264));
#73151=CARTESIAN_POINT('Ctrl Pts',(3.74453008995129,1.,-0.203188003947965));
#73152=CARTESIAN_POINT('Ctrl Pts',(3.74449296982994,1.,-0.203156094897896));
#73153=CARTESIAN_POINT('',(4.19931119685982,0.,-0.0760622897878241));
#73154=CARTESIAN_POINT('Origin',(4.19931119685982,0.,0.0760622897878241));
#73155=CARTESIAN_POINT('',(4.19931119685982,1.,-0.0760622897878241));
#73156=CARTESIAN_POINT('Origin',(0.,1.,0.));
#73157=CARTESIAN_POINT('Origin',(0.,1.,0.));
#73158=CARTESIAN_POINT('Origin',(0.,0.,0.));
#73300=UNCERTAINTY_MEASURE_WITH_UNIT(LENGTH_MEASURE(0.001),#73367,
'DISTANCE_ACCURACY_VALUE',
'Maximum model space distance between geometric entities at asserted c
onnectivities');
#73302=UNCERTAINTY_MEASURE_WITH_UNIT(LENGTH_MEASURE(0.001),#73367,
'DISTANCE_ACCURACY_VALUE',
'Maximum model space distance between geometric entities at asserted c
onnectivities');
#73364=(
GEOMETRIC_REPRESENTATION_CONTEXT(3)
GLOBAL_UNCERTAINTY_ASSIGNED_CONTEXT((#73300))
GLOBAL_UNIT_ASSIGNED_CONTEXT((#73367,#73369,#73370))
REPRESENTATION_CONTEXT('','3D')
);
#73366=(
GEOMETRIC_REPRESENTATION_CONTEXT(3)
GLOBAL_UNCERTAINTY_ASSIGNED_CONTEXT((#73302))
GLOBAL_UNIT_ASSIGNED_CONTEXT((#73367,#73369,#73370))
REPRESENTATION_CONTEXT('','3D')
);
#73367=(
LENGTH_UNIT()
NAMED_UNIT(*)
SI_UNIT(.CENTI.,.METRE.)
);
#73369=(
NAMED_UNIT(*)
PLANE_ANGLE_UNIT()
SI_UNIT($,.RADIAN.)
);
#73370=(
NAMED_UNIT(*)
SI_UNIT($,.STERADIAN.)
SOLID_ANGLE_UNIT()
);
#73432=SHAPE_DEFINITION_REPRESENTATION(#73576,#73668);
#73576=PRODUCT_DEFINITION_SHAPE('',$,#73732);
#73668=SHAPE_REPRESENTATION('',(#18245),#73364);
#73670=PRODUCT_DEFINITION_CONTEXT('part definition',#73861,'design');
#73732=PRODUCT_DEFINITION('Spur Gear - Module 2, 40 Teeth, 20 mm Bore',
'Spur Gear - Module 2, 40 Teeth, 20 mm Bore',#73795,#73670);
#73795=PRODUCT_DEFINITION_FORMATION('',$,#73924);
#73861=APPLICATION_CONTEXT(
'Core Data for Automotive Mechanical Design Process');
#73862=PRODUCT_CONTEXT('part definition',#73861,'mechanical');
#73924=PRODUCT('Spur Gear - Module 2, 40 Teeth, 20 mm Bore',
'Spur Gear - Module 2, 40 Teeth, 20 mm Bore',
'Spur Gear - Module 2, 40 Teeth, 20 mm Bore',(#73862));
#73975=COLOUR_RGB('Sky Blue',0.24,0.69,0.87);
#73976=FILL_AREA_STYLE_COLOUR('',#73975);
#73977=FILL_AREA_STYLE('',(#73976));
#73978=SURFACE_STYLE_FILL_AREA(#73977);
#73979=SURFACE_SIDE_STYLE('',(#73978));
#73980=SURFACE_STYLE_USAGE(.BOTH.,#73979);
#73981=PRESENTATION_STYLE_ASSIGNMENT((#73980));
ENDSEC;
END-ISO-10303-21;
